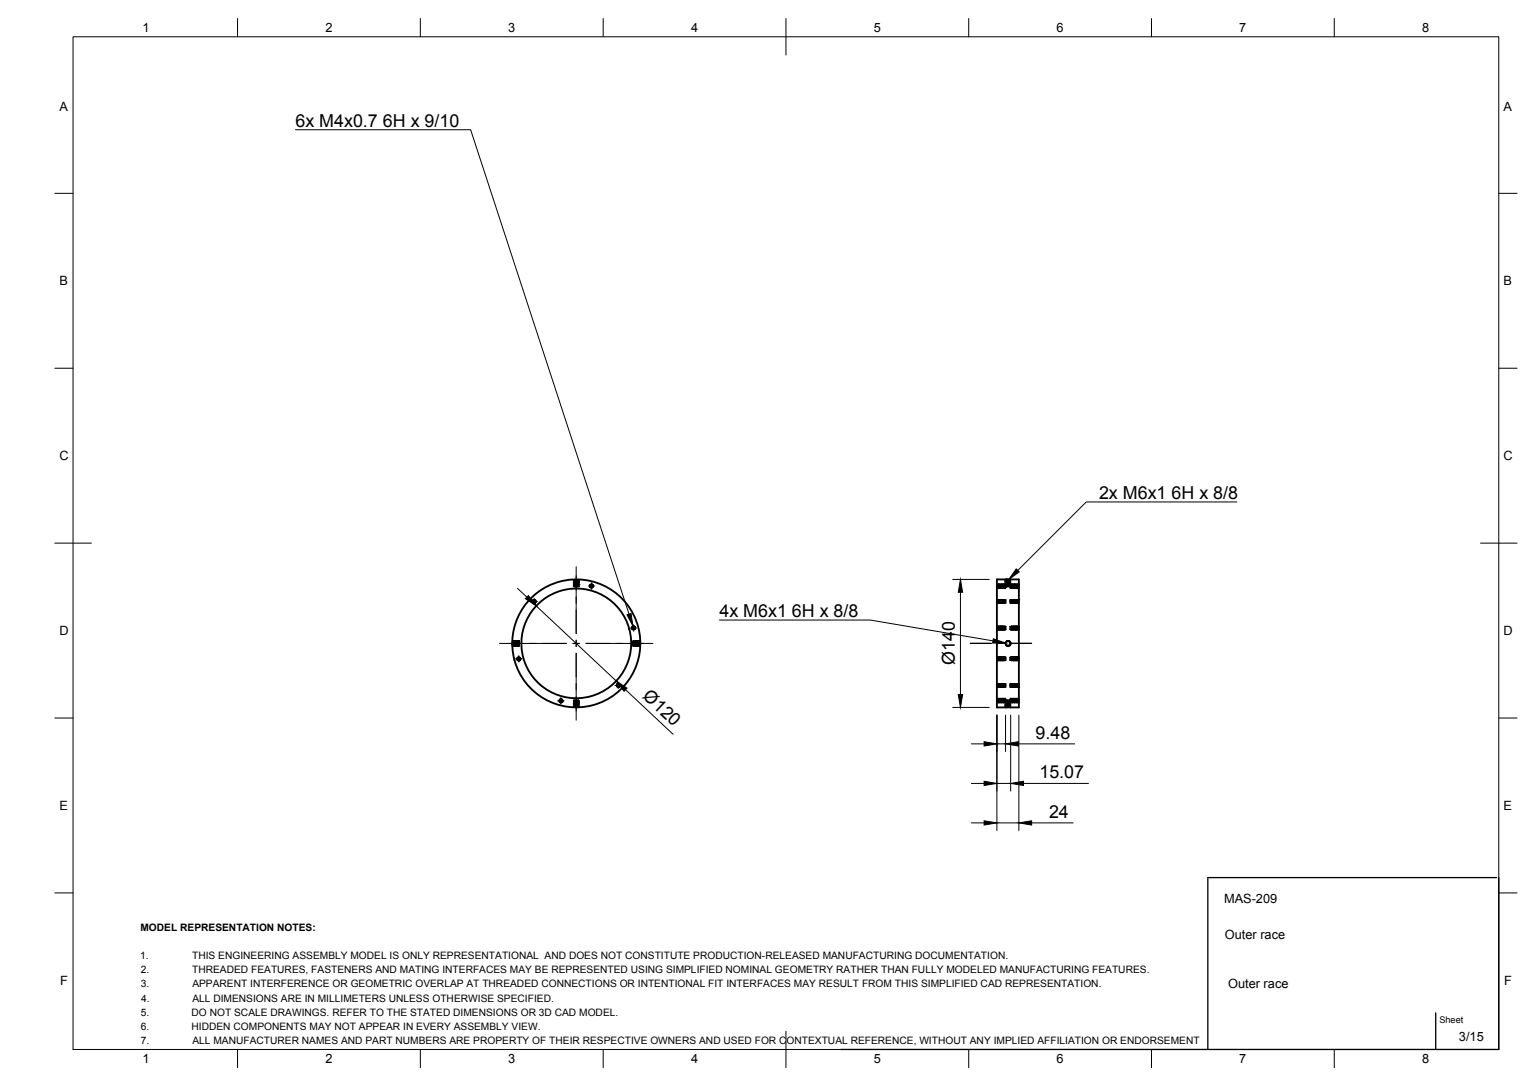
ISO-10303-21;
HEADER;
/* Generated by software containing ST-Developer
 * from STEP Tools, Inc. (www.steptools.com) 
 */

FILE_DESCRIPTION(
/* description */ ('Independent bearing-supported roller-ramp one-way clutch. Six logarit
hmic ramps with plain solid rollers, sprung guided plungers, native Co
il variants, removable shared keepers, rounded parallel key, shaft wit
h complete retaining lips, bronze journal/thrust support and bolted co
vers. Native rotor, roller planar/spin and plunger joints permit manua
l geometric engaged/released inspection. Automatic frictional torque s
witching/contact dynamics are not simulated; no capacity, hardness, fi
t, lubrication, speed, force or life rating. External input driver/cou
pling/anchors outside assembly.'),
/* implementation_level */ '2;1');

FILE_NAME(
/* name */ 'Outer race.step',
/* time_stamp */ '2026-11-08T07:04:38-08:00',
/* author */ (''),
/* organization */ (''),
/* preprocessor_version */ 'ST-DEVELOPER v20.2',
/* originating_system */ 'Autodesk Translation Framework v15.17.0.0',
/* authorisation */ '');

FILE_SCHEMA (('AUTOMOTIVE_DESIGN { 1 0 10303 214 3 1 1 }'));
ENDSEC;

DATA;
#10=MECHANICAL_DESIGN_GEOMETRIC_PRESENTATION_REPRESENTATION('',(#300),#99526);
#268=SHAPE_REPRESENTATION_RELATIONSHIP('SRR','None',#99625,#284);
#284=ADVANCED_BREP_SHAPE_REPRESENTATION('',(#316),#99510);
#300=STYLED_ITEM('',(#99714),#316);
#316=MANIFOLD_SOLID_BREP('Body1',#18270);
#332=FACE_BOUND('',#2130,.T.);
#333=FACE_BOUND('',#2131,.T.);
#334=FACE_BOUND('',#2132,.T.);
#335=FACE_BOUND('',#2133,.T.);
#336=FACE_BOUND('',#2135,.T.);
#337=FACE_BOUND('',#2136,.T.);
#338=FACE_BOUND('',#2137,.T.);
#339=FACE_BOUND('',#2138,.T.);
#340=FACE_BOUND('',#2139,.T.);
#341=FACE_BOUND('',#2140,.T.);
#342=FACE_BOUND('',#2141,.T.);
#343=FACE_BOUND('',#2143,.T.);
#344=FACE_BOUND('',#2144,.T.);
#345=FACE_BOUND('',#2145,.T.);
#346=FACE_BOUND('',#2146,.T.);
#347=FACE_BOUND('',#2147,.T.);
#348=FACE_BOUND('',#2148,.T.);
#349=FACE_BOUND('',#2149,.T.);
#440=PLANE('',#18901);
#441=PLANE('',#18903);
#442=PLANE('',#18905);
#443=PLANE('',#18908);
#444=PLANE('',#18909);
#445=PLANE('',#18912);
#446=PLANE('',#18915);
#447=PLANE('',#18918);
#448=PLANE('',#18921);
#449=PLANE('',#18924);
#450=PLANE('',#18925);
#451=PLANE('',#18926);
#452=PLANE('',#18927);
#453=PLANE('',#18928);
#454=PLANE('',#18929);
#455=PLANE('',#18932);
#456=PLANE('',#18935);
#457=PLANE('',#18938);
#458=PLANE('',#18941);
#459=PLANE('',#18944);
#460=PLANE('',#18945);
#461=PLANE('',#18946);
#462=PLANE('',#18947);
#463=PLANE('',#18948);
#464=PLANE('',#18949);
#465=PLANE('',#18952);
#466=PLANE('',#18953);
#467=PLANE('',#18956);
#468=PLANE('',#18963);
#469=PLANE('',#18964);
#614=B_SPLINE_SURFACE_WITH_KNOTS('',3,3,((#36513,#36514,#36515,#36516,#36517,
#36518,#36519,#36520,#36521,#36522,#36523,#36524,#36525,#36526,#36527,#36528,
#36529,#36530,#36531,#36532,#36533,#36534,#36535,#36536,#36537,#36538,#36539,
#36540,#36541,#36542,#36543,#36544,#36545,#36546,#36547,#36548,#36549,#36550,
#36551,#36552,#36553,#36554,#36555,#36556,#36557,#36558,#36559,#36560,#36561,
#36562,#36563,#36564,#36565,#36566,#36567,#36568),(#36569,#36570,#36571,
#36572,#36573,#36574,#36575,#36576,#36577,#36578,#36579,#36580,#36581,#36582,
#36583,#36584,#36585,#36586,#36587,#36588,#36589,#36590,#36591,#36592,#36593,
#36594,#36595,#36596,#36597,#36598,#36599,#36600,#36601,#36602,#36603,#36604,
#36605,#36606,#36607,#36608,#36609,#36610,#36611,#36612,#36613,#36614,#36615,
#36616,#36617,#36618,#36619,#36620,#36621,#36622,#36623,#36624),(#36625,
#36626,#36627,#36628,#36629,#36630,#36631,#36632,#36633,#36634,#36635,#36636,
#36637,#36638,#36639,#36640,#36641,#36642,#36643,#36644,#36645,#36646,#36647,
#36648,#36649,#36650,#36651,#36652,#36653,#36654,#36655,#36656,#36657,#36658,
#36659,#36660,#36661,#36662,#36663,#36664,#36665,#36666,#36667,#36668,#36669,
#36670,#36671,#36672,#36673,#36674,#36675,#36676,#36677,#36678,#36679,#36680),
(#36681,#36682,#36683,#36684,#36685,#36686,#36687,#36688,#36689,#36690,
#36691,#36692,#36693,#36694,#36695,#36696,#36697,#36698,#36699,#36700,#36701,
#36702,#36703,#36704,#36705,#36706,#36707,#36708,#36709,#36710,#36711,#36712,
#36713,#36714,#36715,#36716,#36717,#36718,#36719,#36720,#36721,#36722,#36723,
#36724,#36725,#36726,#36727,#36728,#36729,#36730,#36731,#36732,#36733,#36734,
#36735,#36736)),.UNSPECIFIED.,.F.,.F.,.F.,(4,4),(4,1,1,1,1,1,1,1,1,1,1,
1,1,1,1,1,1,1,1,1,1,1,1,1,1,1,1,1,1,1,1,1,1,1,1,1,1,1,1,1,1,1,1,1,1,1,1,
1,1,1,1,1,1,4),(0.,0.0642013499338865),(12.0817516052311,13.0640094280149,
14.0462672507987,15.0285250735825,16.0107828963664,16.9930407191502,17.975298541934,
18.9575563647178,19.9398141875016,20.9220720102854,21.9043298330692,22.886587655853,
23.8688454786368,24.8511033014206,25.8333611242044,26.8156189469882,27.797876769772,
28.7801345925559,29.7623924153397,30.7446502381235,31.7269080609073,32.7091658836911,
33.6914237064749,34.6736815292587,35.6559393520425,36.6381971748263,37.6204549976101,
38.6027128203939,39.5849706431777,40.5672284659615,41.5494862887453,42.5317441115292,
43.514001934313,44.4962597570968,45.4785175798806,46.4607754026644,47.4430332254482,
48.425291048232,49.4075488710158,50.3898066937996,51.3720645165834,52.3543223393672,
53.336580162151,54.3188379849348,55.3010958077186,56.2833536305025,57.2656114532863,
58.2478692760701,59.2301270988539,60.2123849216377,61.1946427444215,62.1769005672053,
63.1591583899891,64.1414162127729),.UNSPECIFIED.);
#615=B_SPLINE_SURFACE_WITH_KNOTS('',3,3,((#36890,#36891,#36892,#36893,#36894,
#36895,#36896,#36897,#36898,#36899,#36900,#36901,#36902,#36903,#36904,#36905,
#36906,#36907,#36908,#36909,#36910,#36911,#36912,#36913,#36914,#36915,#36916,
#36917,#36918,#36919,#36920,#36921,#36922,#36923,#36924,#36925,#36926,#36927,
#36928,#36929,#36930,#36931,#36932,#36933,#36934,#36935,#36936,#36937,#36938,
#36939,#36940,#36941,#36942,#36943,#36944,#36945),(#36946,#36947,#36948,
#36949,#36950,#36951,#36952,#36953,#36954,#36955,#36956,#36957,#36958,#36959,
#36960,#36961,#36962,#36963,#36964,#36965,#36966,#36967,#36968,#36969,#36970,
#36971,#36972,#36973,#36974,#36975,#36976,#36977,#36978,#36979,#36980,#36981,
#36982,#36983,#36984,#36985,#36986,#36987,#36988,#36989,#36990,#36991,#36992,
#36993,#36994,#36995,#36996,#36997,#36998,#36999,#37000,#37001),(#37002,
#37003,#37004,#37005,#37006,#37007,#37008,#37009,#37010,#37011,#37012,#37013,
#37014,#37015,#37016,#37017,#37018,#37019,#37020,#37021,#37022,#37023,#37024,
#37025,#37026,#37027,#37028,#37029,#37030,#37031,#37032,#37033,#37034,#37035,
#37036,#37037,#37038,#37039,#37040,#37041,#37042,#37043,#37044,#37045,#37046,
#37047,#37048,#37049,#37050,#37051,#37052,#37053,#37054,#37055,#37056,#37057),
(#37058,#37059,#37060,#37061,#37062,#37063,#37064,#37065,#37066,#37067,
#37068,#37069,#37070,#37071,#37072,#37073,#37074,#37075,#37076,#37077,#37078,
#37079,#37080,#37081,#37082,#37083,#37084,#37085,#37086,#37087,#37088,#37089,
#37090,#37091,#37092,#37093,#37094,#37095,#37096,#37097,#37098,#37099,#37100,
#37101,#37102,#37103,#37104,#37105,#37106,#37107,#37108,#37109,#37110,#37111,
#37112,#37113)),.UNSPECIFIED.,.F.,.F.,.F.,(4,4),(4,1,1,1,1,1,1,1,1,1,1,
1,1,1,1,1,1,1,1,1,1,1,1,1,1,1,1,1,1,1,1,1,1,1,1,1,1,1,1,1,1,1,1,1,1,1,1,
1,1,1,1,1,1,4),(0.,0.0642013499338865),(14.4348810643014,15.4206536381342,
16.4064262119669,17.3921987857997,18.3779713596324,19.3637439334652,20.3495165072979,
21.3352890811306,22.3210616549634,23.3068342287961,24.2926068026289,25.2783793764616,
26.2641519502944,27.2499245241271,28.2356970979599,29.2214696717926,30.2072422456253,
31.1930148194581,32.1787873932908,33.1645599671236,34.1503325409563,35.1361051147891,
36.1218776886218,37.1076502624546,38.0934228362873,39.07919541012,40.0649679839528,
41.0507405577855,42.0365131316183,43.022285705451,44.0080582792838,44.9938308531165,
45.9796034269493,46.965376000782,47.9511485746147,48.9369211484475,49.9226937222802,
50.908466296113,51.8942388699457,52.8800114437785,53.8657840176112,54.851556591444,
55.8373291652767,56.8231017391094,57.8088743129422,58.7946468867749,59.7804194606077,
60.7661920344404,61.7519646082732,62.7377371821059,63.7235097559387,64.7092823297714,
65.6950549036041,66.6808274774369),.UNSPECIFIED.);
#616=B_SPLINE_SURFACE_WITH_KNOTS('',3,3,((#37247,#37248,#37249,#37250,#37251,
#37252,#37253,#37254,#37255,#37256,#37257,#37258,#37259,#37260,#37261,#37262,
#37263,#37264,#37265,#37266,#37267,#37268,#37269,#37270,#37271,#37272,#37273,
#37274,#37275,#37276,#37277,#37278,#37279,#37280,#37281,#37282,#37283,#37284,
#37285,#37286,#37287,#37288,#37289,#37290,#37291,#37292,#37293,#37294,#37295,
#37296,#37297,#37298,#37299,#37300,#37301,#37302),(#37303,#37304,#37305,
#37306,#37307,#37308,#37309,#37310,#37311,#37312,#37313,#37314,#37315,#37316,
#37317,#37318,#37319,#37320,#37321,#37322,#37323,#37324,#37325,#37326,#37327,
#37328,#37329,#37330,#37331,#37332,#37333,#37334,#37335,#37336,#37337,#37338,
#37339,#37340,#37341,#37342,#37343,#37344,#37345,#37346,#37347,#37348,#37349,
#37350,#37351,#37352,#37353,#37354,#37355,#37356,#37357,#37358),(#37359,
#37360,#37361,#37362,#37363,#37364,#37365,#37366,#37367,#37368,#37369,#37370,
#37371,#37372,#37373,#37374,#37375,#37376,#37377,#37378,#37379,#37380,#37381,
#37382,#37383,#37384,#37385,#37386,#37387,#37388,#37389,#37390,#37391,#37392,
#37393,#37394,#37395,#37396,#37397,#37398,#37399,#37400,#37401,#37402,#37403,
#37404,#37405,#37406,#37407,#37408,#37409,#37410,#37411,#37412,#37413,#37414),
(#37415,#37416,#37417,#37418,#37419,#37420,#37421,#37422,#37423,#37424,
#37425,#37426,#37427,#37428,#37429,#37430,#37431,#37432,#37433,#37434,#37435,
#37436,#37437,#37438,#37439,#37440,#37441,#37442,#37443,#37444,#37445,#37446,
#37447,#37448,#37449,#37450,#37451,#37452,#37453,#37454,#37455,#37456,#37457,
#37458,#37459,#37460,#37461,#37462,#37463,#37464,#37465,#37466,#37467,#37468,
#37469,#37470)),.UNSPECIFIED.,.F.,.F.,.F.,(4,4),(4,1,1,1,1,1,1,1,1,1,1,
1,1,1,1,1,1,1,1,1,1,1,1,1,1,1,1,1,1,1,1,1,1,1,1,1,1,1,1,1,1,1,1,1,1,1,1,
1,1,1,1,1,1,4),(0.,0.0642013499338865),(12.0817516052313,13.0640094280151,
14.046267250799,15.0285250735828,16.0107828963666,16.9930407191504,17.9752985419342,
18.957556364718,19.9398141875018,20.9220720102856,21.9043298330694,22.8865876558532,
23.868845478637,24.8511033014208,25.8333611242046,26.8156189469884,27.7978767697722,
28.780134592556,29.7623924153398,30.7446502381237,31.7269080609075,32.7091658836913,
33.6914237064751,34.6736815292589,35.6559393520427,36.6381971748265,37.6204549976103,
38.6027128203941,39.5849706431779,40.5672284659617,41.5494862887455,42.5317441115293,
43.5140019343131,44.4962597570969,45.4785175798807,46.4607754026645,47.4430332254484,
48.4252910482322,49.407548871016,50.3898066937998,51.3720645165836,52.3543223393674,
53.3365801621512,54.318837984935,55.3010958077188,56.2833536305026,57.2656114532864,
58.2478692760702,59.230127098854,60.2123849216378,61.1946427444216,62.1769005672054,
63.1591583899892,64.1414162127731),.UNSPECIFIED.);
#617=B_SPLINE_SURFACE_WITH_KNOTS('',3,3,((#37624,#37625,#37626,#37627,#37628,
#37629,#37630,#37631,#37632,#37633,#37634,#37635,#37636,#37637,#37638,#37639,
#37640,#37641,#37642,#37643,#37644,#37645,#37646,#37647,#37648,#37649,#37650,
#37651,#37652,#37653,#37654,#37655,#37656,#37657,#37658,#37659,#37660,#37661,
#37662,#37663,#37664,#37665,#37666,#37667,#37668,#37669,#37670,#37671,#37672,
#37673,#37674,#37675,#37676,#37677,#37678,#37679),(#37680,#37681,#37682,
#37683,#37684,#37685,#37686,#37687,#37688,#37689,#37690,#37691,#37692,#37693,
#37694,#37695,#37696,#37697,#37698,#37699,#37700,#37701,#37702,#37703,#37704,
#37705,#37706,#37707,#37708,#37709,#37710,#37711,#37712,#37713,#37714,#37715,
#37716,#37717,#37718,#37719,#37720,#37721,#37722,#37723,#37724,#37725,#37726,
#37727,#37728,#37729,#37730,#37731,#37732,#37733,#37734,#37735),(#37736,
#37737,#37738,#37739,#37740,#37741,#37742,#37743,#37744,#37745,#37746,#37747,
#37748,#37749,#37750,#37751,#37752,#37753,#37754,#37755,#37756,#37757,#37758,
#37759,#37760,#37761,#37762,#37763,#37764,#37765,#37766,#37767,#37768,#37769,
#37770,#37771,#37772,#37773,#37774,#37775,#37776,#37777,#37778,#37779,#37780,
#37781,#37782,#37783,#37784,#37785,#37786,#37787,#37788,#37789,#37790,#37791),
(#37792,#37793,#37794,#37795,#37796,#37797,#37798,#37799,#37800,#37801,
#37802,#37803,#37804,#37805,#37806,#37807,#37808,#37809,#37810,#37811,#37812,
#37813,#37814,#37815,#37816,#37817,#37818,#37819,#37820,#37821,#37822,#37823,
#37824,#37825,#37826,#37827,#37828,#37829,#37830,#37831,#37832,#37833,#37834,
#37835,#37836,#37837,#37838,#37839,#37840,#37841,#37842,#37843,#37844,#37845,
#37846,#37847)),.UNSPECIFIED.,.F.,.F.,.F.,(4,4),(4,1,1,1,1,1,1,1,1,1,1,
1,1,1,1,1,1,1,1,1,1,1,1,1,1,1,1,1,1,1,1,1,1,1,1,1,1,1,1,1,1,1,1,1,1,1,1,
1,1,1,1,1,1,4),(0.,0.0642013499338865),(14.4348810643015,15.4206536381343,
16.406426211967,17.3921987857997,18.3779713596325,19.3637439334652,20.349516507298,
21.3352890811307,22.3210616549635,23.3068342287962,24.292606802629,25.2783793764617,
26.2641519502944,27.2499245241272,28.2356970979599,29.2214696717927,30.2072422456254,
31.1930148194582,32.1787873932909,33.1645599671237,34.1503325409564,35.1361051147891,
36.1218776886219,37.1076502624546,38.0934228362874,39.0791954101201,40.0649679839529,
41.0507405577856,42.0365131316183,43.0222857054511,44.0080582792838,44.9938308531166,
45.9796034269493,46.9653760007821,47.9511485746148,48.9369211484476,49.9226937222803,
50.908466296113,51.8942388699458,52.8800114437785,53.8657840176113,54.851556591444,
55.8373291652768,56.8231017391095,57.8088743129423,58.794646886775,59.7804194606078,
60.7661920344405,61.7519646082732,62.737737182106,63.7235097559387,64.7092823297715,
65.6950549036042,66.680827477437),.UNSPECIFIED.);
#618=B_SPLINE_SURFACE_WITH_KNOTS('',3,3,((#37981,#37982,#37983,#37984,#37985,
#37986,#37987,#37988,#37989,#37990,#37991,#37992,#37993,#37994,#37995,#37996,
#37997,#37998,#37999,#38000,#38001,#38002,#38003,#38004,#38005,#38006,#38007,
#38008,#38009,#38010,#38011,#38012,#38013,#38014,#38015,#38016,#38017,#38018,
#38019,#38020,#38021,#38022,#38023,#38024,#38025,#38026,#38027,#38028,#38029,
#38030,#38031,#38032,#38033,#38034,#38035,#38036),(#38037,#38038,#38039,
#38040,#38041,#38042,#38043,#38044,#38045,#38046,#38047,#38048,#38049,#38050,
#38051,#38052,#38053,#38054,#38055,#38056,#38057,#38058,#38059,#38060,#38061,
#38062,#38063,#38064,#38065,#38066,#38067,#38068,#38069,#38070,#38071,#38072,
#38073,#38074,#38075,#38076,#38077,#38078,#38079,#38080,#38081,#38082,#38083,
#38084,#38085,#38086,#38087,#38088,#38089,#38090,#38091,#38092),(#38093,
#38094,#38095,#38096,#38097,#38098,#38099,#38100,#38101,#38102,#38103,#38104,
#38105,#38106,#38107,#38108,#38109,#38110,#38111,#38112,#38113,#38114,#38115,
#38116,#38117,#38118,#38119,#38120,#38121,#38122,#38123,#38124,#38125,#38126,
#38127,#38128,#38129,#38130,#38131,#38132,#38133,#38134,#38135,#38136,#38137,
#38138,#38139,#38140,#38141,#38142,#38143,#38144,#38145,#38146,#38147,#38148),
(#38149,#38150,#38151,#38152,#38153,#38154,#38155,#38156,#38157,#38158,
#38159,#38160,#38161,#38162,#38163,#38164,#38165,#38166,#38167,#38168,#38169,
#38170,#38171,#38172,#38173,#38174,#38175,#38176,#38177,#38178,#38179,#38180,
#38181,#38182,#38183,#38184,#38185,#38186,#38187,#38188,#38189,#38190,#38191,
#38192,#38193,#38194,#38195,#38196,#38197,#38198,#38199,#38200,#38201,#38202,
#38203,#38204)),.UNSPECIFIED.,.F.,.F.,.F.,(4,4),(4,1,1,1,1,1,1,1,1,1,1,
1,1,1,1,1,1,1,1,1,1,1,1,1,1,1,1,1,1,1,1,1,1,1,1,1,1,1,1,1,1,1,1,1,1,1,1,
1,1,1,1,1,1,4),(0.,0.0642013499338865),(12.0817516052311,13.0640094280149,
14.0462672507987,15.0285250735825,16.0107828963663,16.9930407191502,17.975298541934,
18.9575563647178,19.9398141875016,20.9220720102854,21.9043298330692,22.886587655853,
23.8688454786368,24.8511033014206,25.8333611242044,26.8156189469882,27.797876769772,
28.7801345925558,29.7623924153396,30.7446502381234,31.7269080609072,32.709165883691,
33.6914237064749,34.6736815292587,35.6559393520425,36.6381971748263,37.6204549976101,
38.6027128203939,39.5849706431777,40.5672284659615,41.5494862887453,42.5317441115291,
43.5140019343129,44.4962597570967,45.4785175798805,46.4607754026643,47.4430332254481,
48.4252910482319,49.4075488710157,50.3898066937996,51.3720645165834,52.3543223393672,
53.336580162151,54.3188379849348,55.3010958077186,56.2833536305024,57.2656114532862,
58.24786927607,59.2301270988538,60.2123849216376,61.1946427444214,62.1769005672052,
63.159158389989,64.1414162127728),.UNSPECIFIED.);
#619=B_SPLINE_SURFACE_WITH_KNOTS('',3,3,((#38358,#38359,#38360,#38361,#38362,
#38363,#38364,#38365,#38366,#38367,#38368,#38369,#38370,#38371,#38372,#38373,
#38374,#38375,#38376,#38377,#38378,#38379,#38380,#38381,#38382,#38383,#38384,
#38385,#38386,#38387,#38388,#38389,#38390,#38391,#38392,#38393,#38394,#38395,
#38396,#38397,#38398,#38399,#38400,#38401,#38402,#38403,#38404,#38405,#38406,
#38407,#38408,#38409,#38410,#38411,#38412,#38413),(#38414,#38415,#38416,
#38417,#38418,#38419,#38420,#38421,#38422,#38423,#38424,#38425,#38426,#38427,
#38428,#38429,#38430,#38431,#38432,#38433,#38434,#38435,#38436,#38437,#38438,
#38439,#38440,#38441,#38442,#38443,#38444,#38445,#38446,#38447,#38448,#38449,
#38450,#38451,#38452,#38453,#38454,#38455,#38456,#38457,#38458,#38459,#38460,
#38461,#38462,#38463,#38464,#38465,#38466,#38467,#38468,#38469),(#38470,
#38471,#38472,#38473,#38474,#38475,#38476,#38477,#38478,#38479,#38480,#38481,
#38482,#38483,#38484,#38485,#38486,#38487,#38488,#38489,#38490,#38491,#38492,
#38493,#38494,#38495,#38496,#38497,#38498,#38499,#38500,#38501,#38502,#38503,
#38504,#38505,#38506,#38507,#38508,#38509,#38510,#38511,#38512,#38513,#38514,
#38515,#38516,#38517,#38518,#38519,#38520,#38521,#38522,#38523,#38524,#38525),
(#38526,#38527,#38528,#38529,#38530,#38531,#38532,#38533,#38534,#38535,
#38536,#38537,#38538,#38539,#38540,#38541,#38542,#38543,#38544,#38545,#38546,
#38547,#38548,#38549,#38550,#38551,#38552,#38553,#38554,#38555,#38556,#38557,
#38558,#38559,#38560,#38561,#38562,#38563,#38564,#38565,#38566,#38567,#38568,
#38569,#38570,#38571,#38572,#38573,#38574,#38575,#38576,#38577,#38578,#38579,
#38580,#38581)),.UNSPECIFIED.,.F.,.F.,.F.,(4,4),(4,1,1,1,1,1,1,1,1,1,1,
1,1,1,1,1,1,1,1,1,1,1,1,1,1,1,1,1,1,1,1,1,1,1,1,1,1,1,1,1,1,1,1,1,1,1,1,
1,1,1,1,1,1,4),(0.,0.0642013499338865),(14.4348810643012,15.420653638134,
16.4064262119667,17.3921987857995,18.3779713596322,19.363743933465,20.3495165072977,
21.3352890811305,22.3210616549632,23.3068342287959,24.2926068026287,25.2783793764614,
26.2641519502942,27.2499245241269,28.2356970979597,29.2214696717924,30.2072422456252,
31.1930148194579,32.1787873932907,33.1645599671234,34.1503325409562,35.1361051147889,
36.1218776886216,37.1076502624544,38.0934228362871,39.0791954101199,40.0649679839526,
41.0507405577854,42.0365131316181,43.0222857054509,44.0080582792836,44.9938308531164,
45.9796034269491,46.9653760007819,47.9511485746146,48.9369211484474,49.9226937222801,
50.9084662961128,51.8942388699456,52.8800114437783,53.8657840176111,54.8515565914438,
55.8373291652766,56.8231017391093,57.8088743129421,58.7946468867748,59.7804194606076,
60.7661920344403,61.751964608273,62.7377371821058,63.7235097559385,64.7092823297713,
65.695054903604,66.6808274774368),.UNSPECIFIED.);
#620=B_SPLINE_SURFACE_WITH_KNOTS('',3,3,((#38721,#38722,#38723,#38724,#38725,
#38726,#38727,#38728,#38729,#38730,#38731,#38732,#38733,#38734,#38735,#38736,
#38737,#38738,#38739,#38740,#38741,#38742,#38743,#38744,#38745,#38746,#38747,
#38748,#38749,#38750,#38751,#38752,#38753,#38754,#38755,#38756,#38757,#38758,
#38759,#38760,#38761,#38762,#38763,#38764,#38765,#38766,#38767,#38768,#38769,
#38770,#38771,#38772,#38773,#38774,#38775,#38776),(#38777,#38778,#38779,
#38780,#38781,#38782,#38783,#38784,#38785,#38786,#38787,#38788,#38789,#38790,
#38791,#38792,#38793,#38794,#38795,#38796,#38797,#38798,#38799,#38800,#38801,
#38802,#38803,#38804,#38805,#38806,#38807,#38808,#38809,#38810,#38811,#38812,
#38813,#38814,#38815,#38816,#38817,#38818,#38819,#38820,#38821,#38822,#38823,
#38824,#38825,#38826,#38827,#38828,#38829,#38830,#38831,#38832),(#38833,
#38834,#38835,#38836,#38837,#38838,#38839,#38840,#38841,#38842,#38843,#38844,
#38845,#38846,#38847,#38848,#38849,#38850,#38851,#38852,#38853,#38854,#38855,
#38856,#38857,#38858,#38859,#38860,#38861,#38862,#38863,#38864,#38865,#38866,
#38867,#38868,#38869,#38870,#38871,#38872,#38873,#38874,#38875,#38876,#38877,
#38878,#38879,#38880,#38881,#38882,#38883,#38884,#38885,#38886,#38887,#38888),
(#38889,#38890,#38891,#38892,#38893,#38894,#38895,#38896,#38897,#38898,
#38899,#38900,#38901,#38902,#38903,#38904,#38905,#38906,#38907,#38908,#38909,
#38910,#38911,#38912,#38913,#38914,#38915,#38916,#38917,#38918,#38919,#38920,
#38921,#38922,#38923,#38924,#38925,#38926,#38927,#38928,#38929,#38930,#38931,
#38932,#38933,#38934,#38935,#38936,#38937,#38938,#38939,#38940,#38941,#38942,
#38943,#38944)),.UNSPECIFIED.,.F.,.F.,.F.,(4,4),(4,1,1,1,1,1,1,1,1,1,1,
1,1,1,1,1,1,1,1,1,1,1,1,1,1,1,1,1,1,1,1,1,1,1,1,1,1,1,1,1,1,1,1,1,1,1,1,
1,1,1,1,1,1,4),(0.,0.0642013499338865),(12.0817516052311,13.0640094280149,
14.0462672507987,15.0285250735825,16.0107828963663,16.9930407191501,17.9752985419339,
18.9575563647177,19.9398141875016,20.9220720102854,21.9043298330692,22.886587655853,
23.8688454786368,24.8511033014206,25.8333611242044,26.8156189469882,27.797876769772,
28.7801345925558,29.7623924153396,30.7446502381234,31.7269080609072,32.709165883691,
33.6914237064748,34.6736815292587,35.6559393520425,36.6381971748263,37.6204549976101,
38.6027128203939,39.5849706431777,40.5672284659615,41.5494862887453,42.5317441115291,
43.5140019343129,44.4962597570967,45.4785175798805,46.4607754026643,47.4430332254481,
48.4252910482319,49.4075488710157,50.3898066937995,51.3720645165834,52.3543223393672,
53.336580162151,54.3188379849348,55.3010958077186,56.2833536305024,57.2656114532862,
58.24786927607,59.2301270988538,60.2123849216376,61.1946427444214,62.1769005672052,
63.159158389989,64.1414162127728),.UNSPECIFIED.);
#621=B_SPLINE_SURFACE_WITH_KNOTS('',3,3,((#39098,#39099,#39100,#39101,#39102,
#39103,#39104,#39105,#39106,#39107,#39108,#39109,#39110,#39111,#39112,#39113,
#39114,#39115,#39116,#39117,#39118,#39119,#39120,#39121,#39122,#39123,#39124,
#39125,#39126,#39127,#39128,#39129,#39130,#39131,#39132,#39133,#39134,#39135,
#39136,#39137,#39138,#39139,#39140,#39141,#39142,#39143,#39144,#39145,#39146,
#39147,#39148,#39149,#39150,#39151,#39152,#39153),(#39154,#39155,#39156,
#39157,#39158,#39159,#39160,#39161,#39162,#39163,#39164,#39165,#39166,#39167,
#39168,#39169,#39170,#39171,#39172,#39173,#39174,#39175,#39176,#39177,#39178,
#39179,#39180,#39181,#39182,#39183,#39184,#39185,#39186,#39187,#39188,#39189,
#39190,#39191,#39192,#39193,#39194,#39195,#39196,#39197,#39198,#39199,#39200,
#39201,#39202,#39203,#39204,#39205,#39206,#39207,#39208,#39209),(#39210,
#39211,#39212,#39213,#39214,#39215,#39216,#39217,#39218,#39219,#39220,#39221,
#39222,#39223,#39224,#39225,#39226,#39227,#39228,#39229,#39230,#39231,#39232,
#39233,#39234,#39235,#39236,#39237,#39238,#39239,#39240,#39241,#39242,#39243,
#39244,#39245,#39246,#39247,#39248,#39249,#39250,#39251,#39252,#39253,#39254,
#39255,#39256,#39257,#39258,#39259,#39260,#39261,#39262,#39263,#39264,#39265),
(#39266,#39267,#39268,#39269,#39270,#39271,#39272,#39273,#39274,#39275,
#39276,#39277,#39278,#39279,#39280,#39281,#39282,#39283,#39284,#39285,#39286,
#39287,#39288,#39289,#39290,#39291,#39292,#39293,#39294,#39295,#39296,#39297,
#39298,#39299,#39300,#39301,#39302,#39303,#39304,#39305,#39306,#39307,#39308,
#39309,#39310,#39311,#39312,#39313,#39314,#39315,#39316,#39317,#39318,#39319,
#39320,#39321)),.UNSPECIFIED.,.F.,.F.,.F.,(4,4),(4,1,1,1,1,1,1,1,1,1,1,
1,1,1,1,1,1,1,1,1,1,1,1,1,1,1,1,1,1,1,1,1,1,1,1,1,1,1,1,1,1,1,1,1,1,1,1,
1,1,1,1,1,1,4),(0.,0.0642013499338865),(14.4348810643014,15.4206536381342,
16.4064262119669,17.3921987857997,18.3779713596324,19.3637439334652,20.3495165072979,
21.3352890811306,22.3210616549634,23.3068342287961,24.2926068026289,25.2783793764616,
26.2641519502944,27.2499245241271,28.2356970979599,29.2214696717926,30.2072422456253,
31.1930148194581,32.1787873932908,33.1645599671236,34.1503325409563,35.1361051147891,
36.1218776886218,37.1076502624545,38.0934228362873,39.07919541012,40.0649679839528,
41.0507405577855,42.0365131316183,43.022285705451,44.0080582792838,44.9938308531165,
45.9796034269492,46.965376000782,47.9511485746147,48.9369211484475,49.9226937222802,
50.908466296113,51.8942388699457,52.8800114437785,53.8657840176112,54.8515565914439,
55.8373291652767,56.8231017391094,57.8088743129422,58.7946468867749,59.7804194606077,
60.7661920344404,61.7519646082732,62.7377371821059,63.7235097559386,64.7092823297714,
65.6950549036041,66.6808274774369),.UNSPECIFIED.);
#622=B_SPLINE_SURFACE_WITH_KNOTS('',3,3,((#39653,#39654,#39655,#39656,#39657,
#39658,#39659,#39660,#39661,#39662,#39663,#39664,#39665,#39666,#39667,#39668,
#39669,#39670,#39671,#39672,#39673,#39674,#39675,#39676,#39677,#39678,#39679,
#39680,#39681,#39682,#39683,#39684,#39685,#39686,#39687,#39688,#39689,#39690,
#39691,#39692,#39693,#39694,#39695,#39696,#39697,#39698,#39699,#39700,#39701,
#39702,#39703,#39704,#39705,#39706,#39707,#39708,#39709,#39710,#39711,#39712,
#39713,#39714,#39715,#39716,#39717,#39718,#39719,#39720,#39721,#39722,#39723,
#39724,#39725,#39726,#39727,#39728,#39729,#39730,#39731,#39732,#39733,#39734,
#39735,#39736,#39737,#39738),(#39739,#39740,#39741,#39742,#39743,#39744,
#39745,#39746,#39747,#39748,#39749,#39750,#39751,#39752,#39753,#39754,#39755,
#39756,#39757,#39758,#39759,#39760,#39761,#39762,#39763,#39764,#39765,#39766,
#39767,#39768,#39769,#39770,#39771,#39772,#39773,#39774,#39775,#39776,#39777,
#39778,#39779,#39780,#39781,#39782,#39783,#39784,#39785,#39786,#39787,#39788,
#39789,#39790,#39791,#39792,#39793,#39794,#39795,#39796,#39797,#39798,#39799,
#39800,#39801,#39802,#39803,#39804,#39805,#39806,#39807,#39808,#39809,#39810,
#39811,#39812,#39813,#39814,#39815,#39816,#39817,#39818,#39819,#39820,#39821,
#39822,#39823,#39824),(#39825,#39826,#39827,#39828,#39829,#39830,#39831,
#39832,#39833,#39834,#39835,#39836,#39837,#39838,#39839,#39840,#39841,#39842,
#39843,#39844,#39845,#39846,#39847,#39848,#39849,#39850,#39851,#39852,#39853,
#39854,#39855,#39856,#39857,#39858,#39859,#39860,#39861,#39862,#39863,#39864,
#39865,#39866,#39867,#39868,#39869,#39870,#39871,#39872,#39873,#39874,#39875,
#39876,#39877,#39878,#39879,#39880,#39881,#39882,#39883,#39884,#39885,#39886,
#39887,#39888,#39889,#39890,#39891,#39892,#39893,#39894,#39895,#39896,#39897,
#39898,#39899,#39900,#39901,#39902,#39903,#39904,#39905,#39906,#39907,#39908,
#39909,#39910),(#39911,#39912,#39913,#39914,#39915,#39916,#39917,#39918,
#39919,#39920,#39921,#39922,#39923,#39924,#39925,#39926,#39927,#39928,#39929,
#39930,#39931,#39932,#39933,#39934,#39935,#39936,#39937,#39938,#39939,#39940,
#39941,#39942,#39943,#39944,#39945,#39946,#39947,#39948,#39949,#39950,#39951,
#39952,#39953,#39954,#39955,#39956,#39957,#39958,#39959,#39960,#39961,#39962,
#39963,#39964,#39965,#39966,#39967,#39968,#39969,#39970,#39971,#39972,#39973,
#39974,#39975,#39976,#39977,#39978,#39979,#39980,#39981,#39982,#39983,#39984,
#39985,#39986,#39987,#39988,#39989,#39990,#39991,#39992,#39993,#39994,#39995,
#39996)),.UNSPECIFIED.,.F.,.F.,.F.,(4,4),(4,1,1,1,1,1,1,1,1,1,1,1,1,1,1,
1,1,1,1,1,1,1,1,1,1,1,1,1,1,1,1,1,1,1,1,1,1,1,1,1,1,1,1,1,1,1,1,1,1,1,1,
1,1,1,1,1,1,1,1,1,1,1,1,1,1,1,1,1,1,1,1,1,1,1,1,1,1,1,1,1,1,1,1,4),(0.,
0.0448889834294934),(11.8615800042567,12.8591513772396,13.8567227502225,
14.8542941232055,15.8518654961884,16.8494368691713,17.8470082421543,18.8445796151372,
19.8421509881201,20.8397223611031,21.837293734086,22.8348651070689,23.8324364800519,
24.8300078530348,25.8275792260177,26.8251505990007,27.8227219719836,28.8202933449665,
29.8178647179495,30.8154360909324,31.8130074639153,32.8105788368983,33.8081502098812,
34.8057215828641,35.803292955847,36.80086432883,37.7984357018129,38.7960070747958,
39.7935784477788,40.7911498207617,41.7887211937446,42.7862925667276,43.7838639397105,
44.7814353126934,45.7790066856764,46.7765780586593,47.7741494316422,48.7717208046252,
49.7692921776081,50.766863550591,51.764434923574,52.7620062965569,53.7595776695398,
54.7571490425228,55.7547204155057,56.7522917884886,57.7498631614716,58.7474345344545,
59.7450059074374,60.7425772804204,61.7401486534033,62.7377200263862,63.7352913993692,
64.7328627723521,65.730434145335,66.728005518318,67.7255768913009,68.7231482642838,
69.7207196372668,70.7182910102497,71.7158623832326,72.7134337562156,73.7110051291985,
74.7085765021814,75.7061478751643,76.7037192481473,77.7012906211302,78.6988619941132,
79.6964333670961,80.694004740079,81.691576113062,82.6891474860449,83.6867188590278,
84.6842902320108,85.6818616049937,86.6794329779766,87.6770043509595,88.6745757239425,
89.6721470969254,90.6697184699083,91.6672898428913,92.6648612158742,93.6624325888571,
94.6600039618401),.UNSPECIFIED.);
#623=B_SPLINE_SURFACE_WITH_KNOTS('',3,3,((#40104,#40105,#40106,#40107,#40108,
#40109,#40110,#40111,#40112,#40113,#40114,#40115,#40116,#40117,#40118,#40119,
#40120,#40121,#40122,#40123,#40124,#40125,#40126,#40127,#40128,#40129,#40130,
#40131,#40132,#40133,#40134,#40135,#40136,#40137,#40138,#40139,#40140,#40141,
#40142,#40143,#40144,#40145,#40146,#40147,#40148,#40149,#40150,#40151,#40152,
#40153,#40154,#40155,#40156,#40157,#40158,#40159,#40160,#40161,#40162,#40163,
#40164,#40165,#40166,#40167,#40168,#40169,#40170,#40171,#40172,#40173,#40174,
#40175,#40176,#40177,#40178,#40179,#40180,#40181,#40182,#40183,#40184,#40185,
#40186,#40187,#40188,#40189),(#40190,#40191,#40192,#40193,#40194,#40195,
#40196,#40197,#40198,#40199,#40200,#40201,#40202,#40203,#40204,#40205,#40206,
#40207,#40208,#40209,#40210,#40211,#40212,#40213,#40214,#40215,#40216,#40217,
#40218,#40219,#40220,#40221,#40222,#40223,#40224,#40225,#40226,#40227,#40228,
#40229,#40230,#40231,#40232,#40233,#40234,#40235,#40236,#40237,#40238,#40239,
#40240,#40241,#40242,#40243,#40244,#40245,#40246,#40247,#40248,#40249,#40250,
#40251,#40252,#40253,#40254,#40255,#40256,#40257,#40258,#40259,#40260,#40261,
#40262,#40263,#40264,#40265,#40266,#40267,#40268,#40269,#40270,#40271,#40272,
#40273,#40274,#40275),(#40276,#40277,#40278,#40279,#40280,#40281,#40282,
#40283,#40284,#40285,#40286,#40287,#40288,#40289,#40290,#40291,#40292,#40293,
#40294,#40295,#40296,#40297,#40298,#40299,#40300,#40301,#40302,#40303,#40304,
#40305,#40306,#40307,#40308,#40309,#40310,#40311,#40312,#40313,#40314,#40315,
#40316,#40317,#40318,#40319,#40320,#40321,#40322,#40323,#40324,#40325,#40326,
#40327,#40328,#40329,#40330,#40331,#40332,#40333,#40334,#40335,#40336,#40337,
#40338,#40339,#40340,#40341,#40342,#40343,#40344,#40345,#40346,#40347,#40348,
#40349,#40350,#40351,#40352,#40353,#40354,#40355,#40356,#40357,#40358,#40359,
#40360,#40361),(#40362,#40363,#40364,#40365,#40366,#40367,#40368,#40369,
#40370,#40371,#40372,#40373,#40374,#40375,#40376,#40377,#40378,#40379,#40380,
#40381,#40382,#40383,#40384,#40385,#40386,#40387,#40388,#40389,#40390,#40391,
#40392,#40393,#40394,#40395,#40396,#40397,#40398,#40399,#40400,#40401,#40402,
#40403,#40404,#40405,#40406,#40407,#40408,#40409,#40410,#40411,#40412,#40413,
#40414,#40415,#40416,#40417,#40418,#40419,#40420,#40421,#40422,#40423,#40424,
#40425,#40426,#40427,#40428,#40429,#40430,#40431,#40432,#40433,#40434,#40435,
#40436,#40437,#40438,#40439,#40440,#40441,#40442,#40443,#40444,#40445,#40446,
#40447)),.UNSPECIFIED.,.F.,.F.,.F.,(4,4),(4,1,1,1,1,1,1,1,1,1,1,1,1,1,1,
1,1,1,1,1,1,1,1,1,1,1,1,1,1,1,1,1,1,1,1,1,1,1,1,1,1,1,1,1,1,1,1,1,1,1,1,
1,1,1,1,1,1,1,1,1,1,1,1,1,1,1,1,1,1,1,1,1,1,1,1,1,1,1,1,1,1,1,1,4),(0.,
0.0448889834294934),(14.3981410127769,15.3957123857598,16.3932837587428,
17.3908551317257,18.3884265047086,19.3859978776916,20.3835692506745,21.3811406236574,
22.3787119966404,23.3762833696233,24.3738547426062,25.3714261155892,26.3689974885721,
27.366568861555,28.364140234538,29.3617116075209,30.3592829805038,31.3568543534868,
32.3544257264697,33.3519970994526,34.3495684724356,35.3471398454185,36.3447112184014,
37.3422825913844,38.3398539643673,39.3374253373502,40.3349967103332,41.3325680833161,
42.330139456299,43.327710829282,44.3252822022649,45.3228535752478,46.3204249482308,
47.3179963212137,48.3155676941966,49.3131390671795,50.3107104401625,51.3082818131454,
52.3058531861283,53.3034245591113,54.3009959320942,55.2985673050771,56.2961386780601,
57.293710051043,58.2912814240259,59.2888527970089,60.2864241699918,61.2839955429747,
62.2815669159577,63.2791382889406,64.2767096619235,65.2742810349065,66.2718524078894,
67.2694237808723,68.2669951538553,69.2645665268382,70.2621378998211,71.2597092728041,
72.257280645787,73.2548520187699,74.2524233917529,75.2499947647358,76.2475661377187,
77.2451375107017,78.2427088836846,79.2402802566675,80.2378516296505,81.2354230026334,
82.2329943756163,83.2305657485992,84.2281371215822,85.2257084945651,86.2232798675481,
87.220851240531,88.2184226135139,89.2159939864968,90.2135653594798,91.2111367324627,
92.2087081054457,93.2062794784286,94.2038508514115,95.2014222243944,96.1989935973774,
97.1965649703603),.UNSPECIFIED.);
#624=B_SPLINE_SURFACE_WITH_KNOTS('',3,3,((#40752,#40753,#40754,#40755,#40756,
#40757,#40758,#40759,#40760,#40761,#40762,#40763,#40764,#40765,#40766,#40767,
#40768,#40769,#40770,#40771,#40772,#40773,#40774,#40775,#40776,#40777,#40778,
#40779,#40780,#40781,#40782,#40783,#40784,#40785,#40786,#40787,#40788,#40789,
#40790,#40791,#40792,#40793,#40794,#40795,#40796,#40797,#40798,#40799,#40800,
#40801,#40802,#40803,#40804,#40805,#40806,#40807,#40808,#40809,#40810,#40811,
#40812,#40813,#40814,#40815,#40816,#40817,#40818,#40819,#40820,#40821,#40822,
#40823,#40824,#40825,#40826,#40827,#40828,#40829,#40830,#40831,#40832,#40833,
#40834,#40835,#40836,#40837),(#40838,#40839,#40840,#40841,#40842,#40843,
#40844,#40845,#40846,#40847,#40848,#40849,#40850,#40851,#40852,#40853,#40854,
#40855,#40856,#40857,#40858,#40859,#40860,#40861,#40862,#40863,#40864,#40865,
#40866,#40867,#40868,#40869,#40870,#40871,#40872,#40873,#40874,#40875,#40876,
#40877,#40878,#40879,#40880,#40881,#40882,#40883,#40884,#40885,#40886,#40887,
#40888,#40889,#40890,#40891,#40892,#40893,#40894,#40895,#40896,#40897,#40898,
#40899,#40900,#40901,#40902,#40903,#40904,#40905,#40906,#40907,#40908,#40909,
#40910,#40911,#40912,#40913,#40914,#40915,#40916,#40917,#40918,#40919,#40920,
#40921,#40922,#40923),(#40924,#40925,#40926,#40927,#40928,#40929,#40930,
#40931,#40932,#40933,#40934,#40935,#40936,#40937,#40938,#40939,#40940,#40941,
#40942,#40943,#40944,#40945,#40946,#40947,#40948,#40949,#40950,#40951,#40952,
#40953,#40954,#40955,#40956,#40957,#40958,#40959,#40960,#40961,#40962,#40963,
#40964,#40965,#40966,#40967,#40968,#40969,#40970,#40971,#40972,#40973,#40974,
#40975,#40976,#40977,#40978,#40979,#40980,#40981,#40982,#40983,#40984,#40985,
#40986,#40987,#40988,#40989,#40990,#40991,#40992,#40993,#40994,#40995,#40996,
#40997,#40998,#40999,#41000,#41001,#41002,#41003,#41004,#41005,#41006,#41007,
#41008,#41009),(#41010,#41011,#41012,#41013,#41014,#41015,#41016,#41017,
#41018,#41019,#41020,#41021,#41022,#41023,#41024,#41025,#41026,#41027,#41028,
#41029,#41030,#41031,#41032,#41033,#41034,#41035,#41036,#41037,#41038,#41039,
#41040,#41041,#41042,#41043,#41044,#41045,#41046,#41047,#41048,#41049,#41050,
#41051,#41052,#41053,#41054,#41055,#41056,#41057,#41058,#41059,#41060,#41061,
#41062,#41063,#41064,#41065,#41066,#41067,#41068,#41069,#41070,#41071,#41072,
#41073,#41074,#41075,#41076,#41077,#41078,#41079,#41080,#41081,#41082,#41083,
#41084,#41085,#41086,#41087,#41088,#41089,#41090,#41091,#41092,#41093,#41094,
#41095)),.UNSPECIFIED.,.F.,.F.,.F.,(4,4),(4,1,1,1,1,1,1,1,1,1,1,1,1,1,1,
1,1,1,1,1,1,1,1,1,1,1,1,1,1,1,1,1,1,1,1,1,1,1,1,1,1,1,1,1,1,1,1,1,1,1,1,
1,1,1,1,1,1,1,1,1,1,1,1,1,1,1,1,1,1,1,1,1,1,1,1,1,1,1,1,1,1,1,1,4),(0.,
0.0448889834294934),(11.8615800042567,12.8591513772396,13.8567227502225,
14.8542941232055,15.8518654961884,16.8494368691713,17.8470082421543,18.8445796151372,
19.8421509881201,20.8397223611031,21.837293734086,22.8348651070689,23.8324364800519,
24.8300078530348,25.8275792260177,26.8251505990007,27.8227219719836,28.8202933449665,
29.8178647179495,30.8154360909324,31.8130074639153,32.8105788368983,33.8081502098812,
34.8057215828641,35.803292955847,36.80086432883,37.7984357018129,38.7960070747959,
39.7935784477788,40.7911498207617,41.7887211937446,42.7862925667276,43.7838639397105,
44.7814353126934,45.7790066856764,46.7765780586593,47.7741494316422,48.7717208046252,
49.7692921776081,50.766863550591,51.764434923574,52.7620062965569,53.7595776695398,
54.7571490425228,55.7547204155057,56.7522917884886,57.7498631614716,58.7474345344545,
59.7450059074374,60.7425772804204,61.7401486534033,62.7377200263862,63.7352913993692,
64.7328627723521,65.730434145335,66.728005518318,67.7255768913009,68.7231482642838,
69.7207196372668,70.7182910102497,71.7158623832326,72.7134337562156,73.7110051291985,
74.7085765021814,75.7061478751644,76.7037192481473,77.7012906211302,78.6988619941132,
79.6964333670961,80.694004740079,81.691576113062,82.6891474860449,83.6867188590278,
84.6842902320108,85.6818616049937,86.6794329779766,87.6770043509595,88.6745757239425,
89.6721470969254,90.6697184699083,91.6672898428913,92.6648612158742,93.6624325888571,
94.6600039618401),.UNSPECIFIED.);
#625=B_SPLINE_SURFACE_WITH_KNOTS('',3,3,((#41203,#41204,#41205,#41206,#41207,
#41208,#41209,#41210,#41211,#41212,#41213,#41214,#41215,#41216,#41217,#41218,
#41219,#41220,#41221,#41222,#41223,#41224,#41225,#41226,#41227,#41228,#41229,
#41230,#41231,#41232,#41233,#41234,#41235,#41236,#41237,#41238,#41239,#41240,
#41241,#41242,#41243,#41244,#41245,#41246,#41247,#41248,#41249,#41250,#41251,
#41252,#41253,#41254,#41255,#41256,#41257,#41258,#41259,#41260,#41261,#41262,
#41263,#41264,#41265,#41266,#41267,#41268,#41269,#41270,#41271,#41272,#41273,
#41274,#41275,#41276,#41277,#41278,#41279,#41280,#41281,#41282,#41283,#41284,
#41285,#41286,#41287,#41288),(#41289,#41290,#41291,#41292,#41293,#41294,
#41295,#41296,#41297,#41298,#41299,#41300,#41301,#41302,#41303,#41304,#41305,
#41306,#41307,#41308,#41309,#41310,#41311,#41312,#41313,#41314,#41315,#41316,
#41317,#41318,#41319,#41320,#41321,#41322,#41323,#41324,#41325,#41326,#41327,
#41328,#41329,#41330,#41331,#41332,#41333,#41334,#41335,#41336,#41337,#41338,
#41339,#41340,#41341,#41342,#41343,#41344,#41345,#41346,#41347,#41348,#41349,
#41350,#41351,#41352,#41353,#41354,#41355,#41356,#41357,#41358,#41359,#41360,
#41361,#41362,#41363,#41364,#41365,#41366,#41367,#41368,#41369,#41370,#41371,
#41372,#41373,#41374),(#41375,#41376,#41377,#41378,#41379,#41380,#41381,
#41382,#41383,#41384,#41385,#41386,#41387,#41388,#41389,#41390,#41391,#41392,
#41393,#41394,#41395,#41396,#41397,#41398,#41399,#41400,#41401,#41402,#41403,
#41404,#41405,#41406,#41407,#41408,#41409,#41410,#41411,#41412,#41413,#41414,
#41415,#41416,#41417,#41418,#41419,#41420,#41421,#41422,#41423,#41424,#41425,
#41426,#41427,#41428,#41429,#41430,#41431,#41432,#41433,#41434,#41435,#41436,
#41437,#41438,#41439,#41440,#41441,#41442,#41443,#41444,#41445,#41446,#41447,
#41448,#41449,#41450,#41451,#41452,#41453,#41454,#41455,#41456,#41457,#41458,
#41459,#41460),(#41461,#41462,#41463,#41464,#41465,#41466,#41467,#41468,
#41469,#41470,#41471,#41472,#41473,#41474,#41475,#41476,#41477,#41478,#41479,
#41480,#41481,#41482,#41483,#41484,#41485,#41486,#41487,#41488,#41489,#41490,
#41491,#41492,#41493,#41494,#41495,#41496,#41497,#41498,#41499,#41500,#41501,
#41502,#41503,#41504,#41505,#41506,#41507,#41508,#41509,#41510,#41511,#41512,
#41513,#41514,#41515,#41516,#41517,#41518,#41519,#41520,#41521,#41522,#41523,
#41524,#41525,#41526,#41527,#41528,#41529,#41530,#41531,#41532,#41533,#41534,
#41535,#41536,#41537,#41538,#41539,#41540,#41541,#41542,#41543,#41544,#41545,
#41546)),.UNSPECIFIED.,.F.,.F.,.F.,(4,4),(4,1,1,1,1,1,1,1,1,1,1,1,1,1,1,
1,1,1,1,1,1,1,1,1,1,1,1,1,1,1,1,1,1,1,1,1,1,1,1,1,1,1,1,1,1,1,1,1,1,1,1,
1,1,1,1,1,1,1,1,1,1,1,1,1,1,1,1,1,1,1,1,1,1,1,1,1,1,1,1,1,1,1,1,4),(0.,
0.0448889834294934),(14.3981410127769,15.3957123857599,16.3932837587428,
17.3908551317257,18.3884265047086,19.3859978776916,20.3835692506745,21.3811406236574,
22.3787119966404,23.3762833696233,24.3738547426062,25.3714261155892,26.3689974885721,
27.366568861555,28.364140234538,29.3617116075209,30.3592829805038,31.3568543534868,
32.3544257264697,33.3519970994526,34.3495684724356,35.3471398454185,36.3447112184014,
37.3422825913844,38.3398539643673,39.3374253373502,40.3349967103332,41.3325680833161,
42.330139456299,43.327710829282,44.3252822022649,45.3228535752478,46.3204249482308,
47.3179963212137,48.3155676941966,49.3131390671796,50.3107104401625,51.3082818131454,
52.3058531861284,53.3034245591113,54.3009959320942,55.2985673050772,56.2961386780601,
57.293710051043,58.291281424026,59.2888527970089,60.2864241699918,61.2839955429748,
62.2815669159577,63.2791382889406,64.2767096619235,65.2742810349065,66.2718524078894,
67.2694237808723,68.2669951538553,69.2645665268382,70.2621378998211,71.2597092728041,
72.257280645787,73.25485201877,74.2524233917529,75.2499947647358,76.2475661377187,
77.2451375107017,78.2427088836846,79.2402802566675,80.2378516296505,81.2354230026334,
82.2329943756163,83.2305657485993,84.2281371215822,85.2257084945651,86.2232798675481,
87.220851240531,88.2184226135139,89.2159939864969,90.2135653594798,91.2111367324627,
92.2087081054457,93.2062794784286,94.2038508514115,95.2014222243945,96.1989935973774,
97.1965649703603),.UNSPECIFIED.);
#626=B_SPLINE_SURFACE_WITH_KNOTS('',3,3,((#41851,#41852,#41853,#41854,#41855,
#41856,#41857,#41858,#41859,#41860,#41861,#41862,#41863,#41864,#41865,#41866,
#41867,#41868,#41869,#41870,#41871,#41872,#41873,#41874,#41875,#41876,#41877,
#41878,#41879,#41880,#41881,#41882,#41883,#41884,#41885,#41886,#41887,#41888,
#41889,#41890,#41891,#41892,#41893,#41894,#41895,#41896,#41897,#41898,#41899,
#41900,#41901,#41902,#41903,#41904,#41905,#41906,#41907,#41908,#41909,#41910,
#41911,#41912,#41913,#41914,#41915,#41916,#41917,#41918,#41919,#41920,#41921,
#41922,#41923,#41924,#41925,#41926,#41927,#41928,#41929,#41930,#41931,#41932,
#41933,#41934,#41935,#41936),(#41937,#41938,#41939,#41940,#41941,#41942,
#41943,#41944,#41945,#41946,#41947,#41948,#41949,#41950,#41951,#41952,#41953,
#41954,#41955,#41956,#41957,#41958,#41959,#41960,#41961,#41962,#41963,#41964,
#41965,#41966,#41967,#41968,#41969,#41970,#41971,#41972,#41973,#41974,#41975,
#41976,#41977,#41978,#41979,#41980,#41981,#41982,#41983,#41984,#41985,#41986,
#41987,#41988,#41989,#41990,#41991,#41992,#41993,#41994,#41995,#41996,#41997,
#41998,#41999,#42000,#42001,#42002,#42003,#42004,#42005,#42006,#42007,#42008,
#42009,#42010,#42011,#42012,#42013,#42014,#42015,#42016,#42017,#42018,#42019,
#42020,#42021,#42022),(#42023,#42024,#42025,#42026,#42027,#42028,#42029,
#42030,#42031,#42032,#42033,#42034,#42035,#42036,#42037,#42038,#42039,#42040,
#42041,#42042,#42043,#42044,#42045,#42046,#42047,#42048,#42049,#42050,#42051,
#42052,#42053,#42054,#42055,#42056,#42057,#42058,#42059,#42060,#42061,#42062,
#42063,#42064,#42065,#42066,#42067,#42068,#42069,#42070,#42071,#42072,#42073,
#42074,#42075,#42076,#42077,#42078,#42079,#42080,#42081,#42082,#42083,#42084,
#42085,#42086,#42087,#42088,#42089,#42090,#42091,#42092,#42093,#42094,#42095,
#42096,#42097,#42098,#42099,#42100,#42101,#42102,#42103,#42104,#42105,#42106,
#42107,#42108),(#42109,#42110,#42111,#42112,#42113,#42114,#42115,#42116,
#42117,#42118,#42119,#42120,#42121,#42122,#42123,#42124,#42125,#42126,#42127,
#42128,#42129,#42130,#42131,#42132,#42133,#42134,#42135,#42136,#42137,#42138,
#42139,#42140,#42141,#42142,#42143,#42144,#42145,#42146,#42147,#42148,#42149,
#42150,#42151,#42152,#42153,#42154,#42155,#42156,#42157,#42158,#42159,#42160,
#42161,#42162,#42163,#42164,#42165,#42166,#42167,#42168,#42169,#42170,#42171,
#42172,#42173,#42174,#42175,#42176,#42177,#42178,#42179,#42180,#42181,#42182,
#42183,#42184,#42185,#42186,#42187,#42188,#42189,#42190,#42191,#42192,#42193,
#42194)),.UNSPECIFIED.,.F.,.F.,.F.,(4,4),(4,1,1,1,1,1,1,1,1,1,1,1,1,1,1,
1,1,1,1,1,1,1,1,1,1,1,1,1,1,1,1,1,1,1,1,1,1,1,1,1,1,1,1,1,1,1,1,1,1,1,1,
1,1,1,1,1,1,1,1,1,1,1,1,1,1,1,1,1,1,1,1,1,1,1,1,1,1,1,1,1,1,1,1,4),(0.,
0.0448889834294934),(11.8615800042567,12.8591513772396,13.8567227502225,
14.8542941232055,15.8518654961884,16.8494368691713,17.8470082421543,18.8445796151372,
19.8421509881201,20.8397223611031,21.837293734086,22.8348651070689,23.8324364800519,
24.8300078530348,25.8275792260177,26.8251505990007,27.8227219719836,28.8202933449665,
29.8178647179495,30.8154360909324,31.8130074639153,32.8105788368983,33.8081502098812,
34.8057215828641,35.8032929558471,36.80086432883,37.7984357018129,38.7960070747959,
39.7935784477788,40.7911498207617,41.7887211937447,42.7862925667276,43.7838639397105,
44.7814353126935,45.7790066856764,46.7765780586593,47.7741494316423,48.7717208046252,
49.7692921776081,50.7668635505911,51.764434923574,52.7620062965569,53.7595776695399,
54.7571490425228,55.7547204155057,56.7522917884886,57.7498631614716,58.7474345344545,
59.7450059074374,60.7425772804204,61.7401486534033,62.7377200263862,63.7352913993692,
64.7328627723521,65.730434145335,66.728005518318,67.7255768913009,68.7231482642838,
69.7207196372668,70.7182910102497,71.7158623832326,72.7134337562156,73.7110051291985,
74.7085765021814,75.7061478751644,76.7037192481473,77.7012906211302,78.6988619941132,
79.6964333670961,80.694004740079,81.691576113062,82.6891474860449,83.6867188590278,
84.6842902320108,85.6818616049937,86.6794329779766,87.6770043509596,88.6745757239425,
89.6721470969254,90.6697184699084,91.6672898428913,92.6648612158742,93.6624325888572,
94.6600039618401),.UNSPECIFIED.);
#627=B_SPLINE_SURFACE_WITH_KNOTS('',3,3,((#42302,#42303,#42304,#42305,#42306,
#42307,#42308,#42309,#42310,#42311,#42312,#42313,#42314,#42315,#42316,#42317,
#42318,#42319,#42320,#42321,#42322,#42323,#42324,#42325,#42326,#42327,#42328,
#42329,#42330,#42331,#42332,#42333,#42334,#42335,#42336,#42337,#42338,#42339,
#42340,#42341,#42342,#42343,#42344,#42345,#42346,#42347,#42348,#42349,#42350,
#42351,#42352,#42353,#42354,#42355,#42356,#42357,#42358,#42359,#42360,#42361,
#42362,#42363,#42364,#42365,#42366,#42367,#42368,#42369,#42370,#42371,#42372,
#42373,#42374,#42375,#42376,#42377,#42378,#42379,#42380,#42381,#42382,#42383,
#42384,#42385,#42386,#42387),(#42388,#42389,#42390,#42391,#42392,#42393,
#42394,#42395,#42396,#42397,#42398,#42399,#42400,#42401,#42402,#42403,#42404,
#42405,#42406,#42407,#42408,#42409,#42410,#42411,#42412,#42413,#42414,#42415,
#42416,#42417,#42418,#42419,#42420,#42421,#42422,#42423,#42424,#42425,#42426,
#42427,#42428,#42429,#42430,#42431,#42432,#42433,#42434,#42435,#42436,#42437,
#42438,#42439,#42440,#42441,#42442,#42443,#42444,#42445,#42446,#42447,#42448,
#42449,#42450,#42451,#42452,#42453,#42454,#42455,#42456,#42457,#42458,#42459,
#42460,#42461,#42462,#42463,#42464,#42465,#42466,#42467,#42468,#42469,#42470,
#42471,#42472,#42473),(#42474,#42475,#42476,#42477,#42478,#42479,#42480,
#42481,#42482,#42483,#42484,#42485,#42486,#42487,#42488,#42489,#42490,#42491,
#42492,#42493,#42494,#42495,#42496,#42497,#42498,#42499,#42500,#42501,#42502,
#42503,#42504,#42505,#42506,#42507,#42508,#42509,#42510,#42511,#42512,#42513,
#42514,#42515,#42516,#42517,#42518,#42519,#42520,#42521,#42522,#42523,#42524,
#42525,#42526,#42527,#42528,#42529,#42530,#42531,#42532,#42533,#42534,#42535,
#42536,#42537,#42538,#42539,#42540,#42541,#42542,#42543,#42544,#42545,#42546,
#42547,#42548,#42549,#42550,#42551,#42552,#42553,#42554,#42555,#42556,#42557,
#42558,#42559),(#42560,#42561,#42562,#42563,#42564,#42565,#42566,#42567,
#42568,#42569,#42570,#42571,#42572,#42573,#42574,#42575,#42576,#42577,#42578,
#42579,#42580,#42581,#42582,#42583,#42584,#42585,#42586,#42587,#42588,#42589,
#42590,#42591,#42592,#42593,#42594,#42595,#42596,#42597,#42598,#42599,#42600,
#42601,#42602,#42603,#42604,#42605,#42606,#42607,#42608,#42609,#42610,#42611,
#42612,#42613,#42614,#42615,#42616,#42617,#42618,#42619,#42620,#42621,#42622,
#42623,#42624,#42625,#42626,#42627,#42628,#42629,#42630,#42631,#42632,#42633,
#42634,#42635,#42636,#42637,#42638,#42639,#42640,#42641,#42642,#42643,#42644,
#42645)),.UNSPECIFIED.,.F.,.F.,.F.,(4,4),(4,1,1,1,1,1,1,1,1,1,1,1,1,1,1,
1,1,1,1,1,1,1,1,1,1,1,1,1,1,1,1,1,1,1,1,1,1,1,1,1,1,1,1,1,1,1,1,1,1,1,1,
1,1,1,1,1,1,1,1,1,1,1,1,1,1,1,1,1,1,1,1,1,1,1,1,1,1,1,1,1,1,1,1,4),(0.,
0.0448889834294934),(14.3981410127769,15.3957123857599,16.3932837587428,
17.3908551317257,18.3884265047087,19.3859978776916,20.3835692506745,21.3811406236575,
22.3787119966404,23.3762833696233,24.3738547426063,25.3714261155892,26.3689974885721,
27.3665688615551,28.364140234538,29.3617116075209,30.3592829805038,31.3568543534868,
32.3544257264697,33.3519970994526,34.3495684724356,35.3471398454185,36.3447112184014,
37.3422825913844,38.3398539643673,39.3374253373502,40.3349967103332,41.3325680833161,
42.330139456299,43.327710829282,44.3252822022649,45.3228535752478,46.3204249482308,
47.3179963212137,48.3155676941966,49.3131390671796,50.3107104401625,51.3082818131454,
52.3058531861284,53.3034245591113,54.3009959320942,55.2985673050772,56.2961386780601,
57.293710051043,58.291281424026,59.2888527970089,60.2864241699918,61.2839955429748,
62.2815669159577,63.2791382889406,64.2767096619236,65.2742810349065,66.2718524078894,
67.2694237808724,68.2669951538553,69.2645665268382,70.2621378998212,71.2597092728041,
72.257280645787,73.25485201877,74.2524233917529,75.2499947647358,76.2475661377187,
77.2451375107017,78.2427088836846,79.2402802566675,80.2378516296505,81.2354230026334,
82.2329943756163,83.2305657485993,84.2281371215822,85.2257084945651,86.2232798675481,
87.220851240531,88.2184226135139,89.2159939864969,90.2135653594798,91.2111367324627,
92.2087081054457,93.2062794784286,94.2038508514115,95.2014222243945,96.1989935973774,
97.1965649703603),.UNSPECIFIED.);
#628=B_SPLINE_SURFACE_WITH_KNOTS('',3,3,((#42950,#42951,#42952,#42953,#42954,
#42955,#42956,#42957,#42958,#42959,#42960,#42961,#42962,#42963,#42964,#42965,
#42966,#42967,#42968,#42969,#42970,#42971,#42972,#42973,#42974,#42975,#42976,
#42977,#42978,#42979,#42980,#42981,#42982,#42983,#42984,#42985,#42986,#42987,
#42988,#42989,#42990,#42991,#42992,#42993,#42994,#42995,#42996,#42997,#42998,
#42999,#43000,#43001,#43002,#43003,#43004,#43005,#43006,#43007,#43008,#43009,
#43010,#43011,#43012,#43013,#43014,#43015,#43016,#43017,#43018,#43019,#43020,
#43021,#43022,#43023,#43024,#43025,#43026,#43027,#43028,#43029,#43030,#43031,
#43032,#43033,#43034,#43035),(#43036,#43037,#43038,#43039,#43040,#43041,
#43042,#43043,#43044,#43045,#43046,#43047,#43048,#43049,#43050,#43051,#43052,
#43053,#43054,#43055,#43056,#43057,#43058,#43059,#43060,#43061,#43062,#43063,
#43064,#43065,#43066,#43067,#43068,#43069,#43070,#43071,#43072,#43073,#43074,
#43075,#43076,#43077,#43078,#43079,#43080,#43081,#43082,#43083,#43084,#43085,
#43086,#43087,#43088,#43089,#43090,#43091,#43092,#43093,#43094,#43095,#43096,
#43097,#43098,#43099,#43100,#43101,#43102,#43103,#43104,#43105,#43106,#43107,
#43108,#43109,#43110,#43111,#43112,#43113,#43114,#43115,#43116,#43117,#43118,
#43119,#43120,#43121),(#43122,#43123,#43124,#43125,#43126,#43127,#43128,
#43129,#43130,#43131,#43132,#43133,#43134,#43135,#43136,#43137,#43138,#43139,
#43140,#43141,#43142,#43143,#43144,#43145,#43146,#43147,#43148,#43149,#43150,
#43151,#43152,#43153,#43154,#43155,#43156,#43157,#43158,#43159,#43160,#43161,
#43162,#43163,#43164,#43165,#43166,#43167,#43168,#43169,#43170,#43171,#43172,
#43173,#43174,#43175,#43176,#43177,#43178,#43179,#43180,#43181,#43182,#43183,
#43184,#43185,#43186,#43187,#43188,#43189,#43190,#43191,#43192,#43193,#43194,
#43195,#43196,#43197,#43198,#43199,#43200,#43201,#43202,#43203,#43204,#43205,
#43206,#43207),(#43208,#43209,#43210,#43211,#43212,#43213,#43214,#43215,
#43216,#43217,#43218,#43219,#43220,#43221,#43222,#43223,#43224,#43225,#43226,
#43227,#43228,#43229,#43230,#43231,#43232,#43233,#43234,#43235,#43236,#43237,
#43238,#43239,#43240,#43241,#43242,#43243,#43244,#43245,#43246,#43247,#43248,
#43249,#43250,#43251,#43252,#43253,#43254,#43255,#43256,#43257,#43258,#43259,
#43260,#43261,#43262,#43263,#43264,#43265,#43266,#43267,#43268,#43269,#43270,
#43271,#43272,#43273,#43274,#43275,#43276,#43277,#43278,#43279,#43280,#43281,
#43282,#43283,#43284,#43285,#43286,#43287,#43288,#43289,#43290,#43291,#43292,
#43293)),.UNSPECIFIED.,.F.,.F.,.F.,(4,4),(4,1,1,1,1,1,1,1,1,1,1,1,1,1,1,
1,1,1,1,1,1,1,1,1,1,1,1,1,1,1,1,1,1,1,1,1,1,1,1,1,1,1,1,1,1,1,1,1,1,1,1,
1,1,1,1,1,1,1,1,1,1,1,1,1,1,1,1,1,1,1,1,1,1,1,1,1,1,1,1,1,1,1,1,4),(0.,
0.0448889834294934),(11.8615800042567,12.8591513772396,13.8567227502225,
14.8542941232055,15.8518654961884,16.8494368691713,17.8470082421543,18.8445796151372,
19.8421509881201,20.8397223611031,21.837293734086,22.8348651070689,23.8324364800519,
24.8300078530348,25.8275792260177,26.8251505990007,27.8227219719836,28.8202933449665,
29.8178647179495,30.8154360909324,31.8130074639153,32.8105788368983,33.8081502098812,
34.8057215828641,35.8032929558471,36.80086432883,37.7984357018129,38.7960070747959,
39.7935784477788,40.7911498207617,41.7887211937447,42.7862925667276,43.7838639397105,
44.7814353126935,45.7790066856764,46.7765780586593,47.7741494316423,48.7717208046252,
49.7692921776081,50.7668635505911,51.764434923574,52.7620062965569,53.7595776695399,
54.7571490425228,55.7547204155057,56.7522917884886,57.7498631614716,58.7474345344545,
59.7450059074374,60.7425772804204,61.7401486534033,62.7377200263862,63.7352913993692,
64.7328627723521,65.730434145335,66.728005518318,67.7255768913009,68.7231482642838,
69.7207196372668,70.7182910102497,71.7158623832326,72.7134337562156,73.7110051291985,
74.7085765021814,75.7061478751644,76.7037192481473,77.7012906211302,78.6988619941132,
79.6964333670961,80.694004740079,81.691576113062,82.6891474860449,83.6867188590278,
84.6842902320108,85.6818616049937,86.6794329779766,87.6770043509596,88.6745757239425,
89.6721470969254,90.6697184699084,91.6672898428913,92.6648612158742,93.6624325888572,
94.6600039618401),.UNSPECIFIED.);
#629=B_SPLINE_SURFACE_WITH_KNOTS('',3,3,((#43401,#43402,#43403,#43404,#43405,
#43406,#43407,#43408,#43409,#43410,#43411,#43412,#43413,#43414,#43415,#43416,
#43417,#43418,#43419,#43420,#43421,#43422,#43423,#43424,#43425,#43426,#43427,
#43428,#43429,#43430,#43431,#43432,#43433,#43434,#43435,#43436,#43437,#43438,
#43439,#43440,#43441,#43442,#43443,#43444,#43445,#43446,#43447,#43448,#43449,
#43450,#43451,#43452,#43453,#43454,#43455,#43456,#43457,#43458,#43459,#43460,
#43461,#43462,#43463,#43464,#43465,#43466,#43467,#43468,#43469,#43470,#43471,
#43472,#43473,#43474,#43475,#43476,#43477,#43478,#43479,#43480,#43481,#43482,
#43483,#43484,#43485,#43486),(#43487,#43488,#43489,#43490,#43491,#43492,
#43493,#43494,#43495,#43496,#43497,#43498,#43499,#43500,#43501,#43502,#43503,
#43504,#43505,#43506,#43507,#43508,#43509,#43510,#43511,#43512,#43513,#43514,
#43515,#43516,#43517,#43518,#43519,#43520,#43521,#43522,#43523,#43524,#43525,
#43526,#43527,#43528,#43529,#43530,#43531,#43532,#43533,#43534,#43535,#43536,
#43537,#43538,#43539,#43540,#43541,#43542,#43543,#43544,#43545,#43546,#43547,
#43548,#43549,#43550,#43551,#43552,#43553,#43554,#43555,#43556,#43557,#43558,
#43559,#43560,#43561,#43562,#43563,#43564,#43565,#43566,#43567,#43568,#43569,
#43570,#43571,#43572),(#43573,#43574,#43575,#43576,#43577,#43578,#43579,
#43580,#43581,#43582,#43583,#43584,#43585,#43586,#43587,#43588,#43589,#43590,
#43591,#43592,#43593,#43594,#43595,#43596,#43597,#43598,#43599,#43600,#43601,
#43602,#43603,#43604,#43605,#43606,#43607,#43608,#43609,#43610,#43611,#43612,
#43613,#43614,#43615,#43616,#43617,#43618,#43619,#43620,#43621,#43622,#43623,
#43624,#43625,#43626,#43627,#43628,#43629,#43630,#43631,#43632,#43633,#43634,
#43635,#43636,#43637,#43638,#43639,#43640,#43641,#43642,#43643,#43644,#43645,
#43646,#43647,#43648,#43649,#43650,#43651,#43652,#43653,#43654,#43655,#43656,
#43657,#43658),(#43659,#43660,#43661,#43662,#43663,#43664,#43665,#43666,
#43667,#43668,#43669,#43670,#43671,#43672,#43673,#43674,#43675,#43676,#43677,
#43678,#43679,#43680,#43681,#43682,#43683,#43684,#43685,#43686,#43687,#43688,
#43689,#43690,#43691,#43692,#43693,#43694,#43695,#43696,#43697,#43698,#43699,
#43700,#43701,#43702,#43703,#43704,#43705,#43706,#43707,#43708,#43709,#43710,
#43711,#43712,#43713,#43714,#43715,#43716,#43717,#43718,#43719,#43720,#43721,
#43722,#43723,#43724,#43725,#43726,#43727,#43728,#43729,#43730,#43731,#43732,
#43733,#43734,#43735,#43736,#43737,#43738,#43739,#43740,#43741,#43742,#43743,
#43744)),.UNSPECIFIED.,.F.,.F.,.F.,(4,4),(4,1,1,1,1,1,1,1,1,1,1,1,1,1,1,
1,1,1,1,1,1,1,1,1,1,1,1,1,1,1,1,1,1,1,1,1,1,1,1,1,1,1,1,1,1,1,1,1,1,1,1,
1,1,1,1,1,1,1,1,1,1,1,1,1,1,1,1,1,1,1,1,1,1,1,1,1,1,1,1,1,1,1,1,4),(0.,
0.0448889834294934),(14.3981410127769,15.3957123857599,16.3932837587428,
17.3908551317257,18.3884265047087,19.3859978776916,20.3835692506745,21.3811406236575,
22.3787119966404,23.3762833696233,24.3738547426063,25.3714261155892,26.3689974885721,
27.3665688615551,28.364140234538,29.3617116075209,30.3592829805038,31.3568543534868,
32.3544257264697,33.3519970994526,34.3495684724356,35.3471398454185,36.3447112184014,
37.3422825913844,38.3398539643673,39.3374253373502,40.3349967103332,41.3325680833161,
42.330139456299,43.327710829282,44.3252822022649,45.3228535752478,46.3204249482308,
47.3179963212137,48.3155676941966,49.3131390671796,50.3107104401625,51.3082818131454,
52.3058531861284,53.3034245591113,54.3009959320942,55.2985673050772,56.2961386780601,
57.293710051043,58.291281424026,59.2888527970089,60.2864241699918,61.2839955429748,
62.2815669159577,63.2791382889406,64.2767096619236,65.2742810349065,66.2718524078894,
67.2694237808724,68.2669951538553,69.2645665268382,70.2621378998212,71.2597092728041,
72.257280645787,73.25485201877,74.2524233917529,75.2499947647358,76.2475661377187,
77.2451375107017,78.2427088836846,79.2402802566675,80.2378516296505,81.2354230026334,
82.2329943756163,83.2305657485993,84.2281371215822,85.2257084945651,86.2232798675481,
87.220851240531,88.2184226135139,89.2159939864969,90.2135653594798,91.2111367324627,
92.2087081054457,93.2062794784286,94.2038508514115,95.2014222243945,96.1989935973774,
97.1965649703603),.UNSPECIFIED.);
#630=B_SPLINE_SURFACE_WITH_KNOTS('',3,3,((#44049,#44050,#44051,#44052,#44053,
#44054,#44055,#44056,#44057,#44058,#44059,#44060,#44061,#44062,#44063,#44064,
#44065,#44066,#44067,#44068,#44069,#44070,#44071,#44072,#44073,#44074,#44075,
#44076,#44077,#44078,#44079,#44080,#44081,#44082,#44083,#44084,#44085,#44086,
#44087,#44088,#44089,#44090,#44091,#44092,#44093,#44094,#44095,#44096,#44097,
#44098,#44099,#44100,#44101,#44102,#44103,#44104,#44105,#44106,#44107,#44108,
#44109,#44110,#44111,#44112,#44113,#44114,#44115,#44116,#44117,#44118,#44119,
#44120,#44121,#44122,#44123,#44124,#44125,#44126,#44127,#44128,#44129,#44130,
#44131,#44132,#44133,#44134),(#44135,#44136,#44137,#44138,#44139,#44140,
#44141,#44142,#44143,#44144,#44145,#44146,#44147,#44148,#44149,#44150,#44151,
#44152,#44153,#44154,#44155,#44156,#44157,#44158,#44159,#44160,#44161,#44162,
#44163,#44164,#44165,#44166,#44167,#44168,#44169,#44170,#44171,#44172,#44173,
#44174,#44175,#44176,#44177,#44178,#44179,#44180,#44181,#44182,#44183,#44184,
#44185,#44186,#44187,#44188,#44189,#44190,#44191,#44192,#44193,#44194,#44195,
#44196,#44197,#44198,#44199,#44200,#44201,#44202,#44203,#44204,#44205,#44206,
#44207,#44208,#44209,#44210,#44211,#44212,#44213,#44214,#44215,#44216,#44217,
#44218,#44219,#44220),(#44221,#44222,#44223,#44224,#44225,#44226,#44227,
#44228,#44229,#44230,#44231,#44232,#44233,#44234,#44235,#44236,#44237,#44238,
#44239,#44240,#44241,#44242,#44243,#44244,#44245,#44246,#44247,#44248,#44249,
#44250,#44251,#44252,#44253,#44254,#44255,#44256,#44257,#44258,#44259,#44260,
#44261,#44262,#44263,#44264,#44265,#44266,#44267,#44268,#44269,#44270,#44271,
#44272,#44273,#44274,#44275,#44276,#44277,#44278,#44279,#44280,#44281,#44282,
#44283,#44284,#44285,#44286,#44287,#44288,#44289,#44290,#44291,#44292,#44293,
#44294,#44295,#44296,#44297,#44298,#44299,#44300,#44301,#44302,#44303,#44304,
#44305,#44306),(#44307,#44308,#44309,#44310,#44311,#44312,#44313,#44314,
#44315,#44316,#44317,#44318,#44319,#44320,#44321,#44322,#44323,#44324,#44325,
#44326,#44327,#44328,#44329,#44330,#44331,#44332,#44333,#44334,#44335,#44336,
#44337,#44338,#44339,#44340,#44341,#44342,#44343,#44344,#44345,#44346,#44347,
#44348,#44349,#44350,#44351,#44352,#44353,#44354,#44355,#44356,#44357,#44358,
#44359,#44360,#44361,#44362,#44363,#44364,#44365,#44366,#44367,#44368,#44369,
#44370,#44371,#44372,#44373,#44374,#44375,#44376,#44377,#44378,#44379,#44380,
#44381,#44382,#44383,#44384,#44385,#44386,#44387,#44388,#44389,#44390,#44391,
#44392)),.UNSPECIFIED.,.F.,.F.,.F.,(4,4),(4,1,1,1,1,1,1,1,1,1,1,1,1,1,1,
1,1,1,1,1,1,1,1,1,1,1,1,1,1,1,1,1,1,1,1,1,1,1,1,1,1,1,1,1,1,1,1,1,1,1,1,
1,1,1,1,1,1,1,1,1,1,1,1,1,1,1,1,1,1,1,1,1,1,1,1,1,1,1,1,1,1,1,1,4),(0.,
0.0448889834294934),(11.8615800042567,12.8591513772396,13.8567227502225,
14.8542941232055,15.8518654961884,16.8494368691713,17.8470082421543,18.8445796151372,
19.8421509881201,20.8397223611031,21.837293734086,22.8348651070689,23.8324364800519,
24.8300078530348,25.8275792260177,26.8251505990007,27.8227219719836,28.8202933449665,
29.8178647179495,30.8154360909324,31.8130074639153,32.8105788368983,33.8081502098812,
34.8057215828641,35.8032929558471,36.80086432883,37.7984357018129,38.7960070747959,
39.7935784477788,40.7911498207617,41.7887211937447,42.7862925667276,43.7838639397105,
44.7814353126935,45.7790066856764,46.7765780586593,47.7741494316423,48.7717208046252,
49.7692921776081,50.7668635505911,51.764434923574,52.7620062965569,53.7595776695399,
54.7571490425228,55.7547204155057,56.7522917884886,57.7498631614716,58.7474345344545,
59.7450059074374,60.7425772804204,61.7401486534033,62.7377200263862,63.7352913993692,
64.7328627723521,65.7304341453351,66.728005518318,67.7255768913009,68.7231482642839,
69.7207196372668,70.7182910102497,71.7158623832326,72.7134337562156,73.7110051291985,
74.7085765021814,75.7061478751644,76.7037192481473,77.7012906211302,78.6988619941132,
79.6964333670961,80.694004740079,81.691576113062,82.6891474860449,83.6867188590278,
84.6842902320108,85.6818616049937,86.6794329779766,87.6770043509596,88.6745757239425,
89.6721470969254,90.6697184699084,91.6672898428913,92.6648612158742,93.6624325888572,
94.6600039618401),.UNSPECIFIED.);
#631=B_SPLINE_SURFACE_WITH_KNOTS('',3,3,((#44500,#44501,#44502,#44503,#44504,
#44505,#44506,#44507,#44508,#44509,#44510,#44511,#44512,#44513,#44514,#44515,
#44516,#44517,#44518,#44519,#44520,#44521,#44522,#44523,#44524,#44525,#44526,
#44527,#44528,#44529,#44530,#44531,#44532,#44533,#44534,#44535,#44536,#44537,
#44538,#44539,#44540,#44541,#44542,#44543,#44544,#44545,#44546,#44547,#44548,
#44549,#44550,#44551,#44552,#44553,#44554,#44555,#44556,#44557,#44558,#44559,
#44560,#44561,#44562,#44563,#44564,#44565,#44566,#44567,#44568,#44569,#44570,
#44571,#44572,#44573,#44574,#44575,#44576,#44577,#44578,#44579,#44580,#44581,
#44582,#44583,#44584,#44585),(#44586,#44587,#44588,#44589,#44590,#44591,
#44592,#44593,#44594,#44595,#44596,#44597,#44598,#44599,#44600,#44601,#44602,
#44603,#44604,#44605,#44606,#44607,#44608,#44609,#44610,#44611,#44612,#44613,
#44614,#44615,#44616,#44617,#44618,#44619,#44620,#44621,#44622,#44623,#44624,
#44625,#44626,#44627,#44628,#44629,#44630,#44631,#44632,#44633,#44634,#44635,
#44636,#44637,#44638,#44639,#44640,#44641,#44642,#44643,#44644,#44645,#44646,
#44647,#44648,#44649,#44650,#44651,#44652,#44653,#44654,#44655,#44656,#44657,
#44658,#44659,#44660,#44661,#44662,#44663,#44664,#44665,#44666,#44667,#44668,
#44669,#44670,#44671),(#44672,#44673,#44674,#44675,#44676,#44677,#44678,
#44679,#44680,#44681,#44682,#44683,#44684,#44685,#44686,#44687,#44688,#44689,
#44690,#44691,#44692,#44693,#44694,#44695,#44696,#44697,#44698,#44699,#44700,
#44701,#44702,#44703,#44704,#44705,#44706,#44707,#44708,#44709,#44710,#44711,
#44712,#44713,#44714,#44715,#44716,#44717,#44718,#44719,#44720,#44721,#44722,
#44723,#44724,#44725,#44726,#44727,#44728,#44729,#44730,#44731,#44732,#44733,
#44734,#44735,#44736,#44737,#44738,#44739,#44740,#44741,#44742,#44743,#44744,
#44745,#44746,#44747,#44748,#44749,#44750,#44751,#44752,#44753,#44754,#44755,
#44756,#44757),(#44758,#44759,#44760,#44761,#44762,#44763,#44764,#44765,
#44766,#44767,#44768,#44769,#44770,#44771,#44772,#44773,#44774,#44775,#44776,
#44777,#44778,#44779,#44780,#44781,#44782,#44783,#44784,#44785,#44786,#44787,
#44788,#44789,#44790,#44791,#44792,#44793,#44794,#44795,#44796,#44797,#44798,
#44799,#44800,#44801,#44802,#44803,#44804,#44805,#44806,#44807,#44808,#44809,
#44810,#44811,#44812,#44813,#44814,#44815,#44816,#44817,#44818,#44819,#44820,
#44821,#44822,#44823,#44824,#44825,#44826,#44827,#44828,#44829,#44830,#44831,
#44832,#44833,#44834,#44835,#44836,#44837,#44838,#44839,#44840,#44841,#44842,
#44843)),.UNSPECIFIED.,.F.,.F.,.F.,(4,4),(4,1,1,1,1,1,1,1,1,1,1,1,1,1,1,
1,1,1,1,1,1,1,1,1,1,1,1,1,1,1,1,1,1,1,1,1,1,1,1,1,1,1,1,1,1,1,1,1,1,1,1,
1,1,1,1,1,1,1,1,1,1,1,1,1,1,1,1,1,1,1,1,1,1,1,1,1,1,1,1,1,1,1,1,4),(0.,
0.0448889834294934),(14.3981410127769,15.3957123857599,16.3932837587428,
17.3908551317257,18.3884265047087,19.3859978776916,20.3835692506745,21.3811406236575,
22.3787119966404,23.3762833696233,24.3738547426063,25.3714261155892,26.3689974885721,
27.3665688615551,28.364140234538,29.3617116075209,30.3592829805038,31.3568543534868,
32.3544257264697,33.3519970994526,34.3495684724356,35.3471398454185,36.3447112184014,
37.3422825913844,38.3398539643673,39.3374253373502,40.3349967103332,41.3325680833161,
42.330139456299,43.327710829282,44.3252822022649,45.3228535752478,46.3204249482308,
47.3179963212137,48.3155676941966,49.3131390671796,50.3107104401625,51.3082818131454,
52.3058531861284,53.3034245591113,54.3009959320942,55.2985673050772,56.2961386780601,
57.293710051043,58.291281424026,59.2888527970089,60.2864241699918,61.2839955429748,
62.2815669159577,63.2791382889406,64.2767096619236,65.2742810349065,66.2718524078894,
67.2694237808724,68.2669951538553,69.2645665268382,70.2621378998212,71.2597092728041,
72.257280645787,73.25485201877,74.2524233917529,75.2499947647358,76.2475661377187,
77.2451375107017,78.2427088836846,79.2402802566675,80.2378516296505,81.2354230026334,
82.2329943756163,83.2305657485993,84.2281371215822,85.2257084945651,86.2232798675481,
87.220851240531,88.2184226135139,89.2159939864969,90.2135653594798,91.2111367324627,
92.2087081054457,93.2062794784286,94.2038508514115,95.2014222243945,96.1989935973774,
97.1965649703603),.UNSPECIFIED.);
#632=B_SPLINE_SURFACE_WITH_KNOTS('',3,3,((#45153,#45154,#45155,#45156,#45157,
#45158,#45159,#45160,#45161,#45162,#45163,#45164,#45165,#45166,#45167,#45168,
#45169,#45170,#45171,#45172,#45173,#45174,#45175,#45176,#45177,#45178,#45179,
#45180,#45181,#45182,#45183,#45184,#45185,#45186,#45187,#45188,#45189,#45190,
#45191,#45192,#45193,#45194,#45195,#45196,#45197,#45198,#45199,#45200,#45201,
#45202,#45203,#45204,#45205,#45206,#45207,#45208,#45209,#45210,#45211,#45212,
#45213,#45214,#45215,#45216,#45217,#45218,#45219,#45220,#45221,#45222,#45223,
#45224,#45225,#45226,#45227,#45228,#45229,#45230,#45231,#45232,#45233,#45234,
#45235,#45236,#45237,#45238),(#45239,#45240,#45241,#45242,#45243,#45244,
#45245,#45246,#45247,#45248,#45249,#45250,#45251,#45252,#45253,#45254,#45255,
#45256,#45257,#45258,#45259,#45260,#45261,#45262,#45263,#45264,#45265,#45266,
#45267,#45268,#45269,#45270,#45271,#45272,#45273,#45274,#45275,#45276,#45277,
#45278,#45279,#45280,#45281,#45282,#45283,#45284,#45285,#45286,#45287,#45288,
#45289,#45290,#45291,#45292,#45293,#45294,#45295,#45296,#45297,#45298,#45299,
#45300,#45301,#45302,#45303,#45304,#45305,#45306,#45307,#45308,#45309,#45310,
#45311,#45312,#45313,#45314,#45315,#45316,#45317,#45318,#45319,#45320,#45321,
#45322,#45323,#45324),(#45325,#45326,#45327,#45328,#45329,#45330,#45331,
#45332,#45333,#45334,#45335,#45336,#45337,#45338,#45339,#45340,#45341,#45342,
#45343,#45344,#45345,#45346,#45347,#45348,#45349,#45350,#45351,#45352,#45353,
#45354,#45355,#45356,#45357,#45358,#45359,#45360,#45361,#45362,#45363,#45364,
#45365,#45366,#45367,#45368,#45369,#45370,#45371,#45372,#45373,#45374,#45375,
#45376,#45377,#45378,#45379,#45380,#45381,#45382,#45383,#45384,#45385,#45386,
#45387,#45388,#45389,#45390,#45391,#45392,#45393,#45394,#45395,#45396,#45397,
#45398,#45399,#45400,#45401,#45402,#45403,#45404,#45405,#45406,#45407,#45408,
#45409,#45410),(#45411,#45412,#45413,#45414,#45415,#45416,#45417,#45418,
#45419,#45420,#45421,#45422,#45423,#45424,#45425,#45426,#45427,#45428,#45429,
#45430,#45431,#45432,#45433,#45434,#45435,#45436,#45437,#45438,#45439,#45440,
#45441,#45442,#45443,#45444,#45445,#45446,#45447,#45448,#45449,#45450,#45451,
#45452,#45453,#45454,#45455,#45456,#45457,#45458,#45459,#45460,#45461,#45462,
#45463,#45464,#45465,#45466,#45467,#45468,#45469,#45470,#45471,#45472,#45473,
#45474,#45475,#45476,#45477,#45478,#45479,#45480,#45481,#45482,#45483,#45484,
#45485,#45486,#45487,#45488,#45489,#45490,#45491,#45492,#45493,#45494,#45495,
#45496)),.UNSPECIFIED.,.F.,.F.,.F.,(4,4),(4,1,1,1,1,1,1,1,1,1,1,1,1,1,1,
1,1,1,1,1,1,1,1,1,1,1,1,1,1,1,1,1,1,1,1,1,1,1,1,1,1,1,1,1,1,1,1,1,1,1,1,
1,1,1,1,1,1,1,1,1,1,1,1,1,1,1,1,1,1,1,1,1,1,1,1,1,1,1,1,1,1,1,1,4),(0.,
0.0448889834294934),(11.8615800042566,12.8591513772395,13.8567227502225,
14.8542941232054,15.8518654961883,16.8494368691713,17.8470082421542,18.8445796151371,
19.8421509881201,20.839722361103,21.8372937340859,22.8348651070689,23.8324364800518,
24.8300078530347,25.8275792260177,26.8251505990006,27.8227219719835,28.8202933449665,
29.8178647179494,30.8154360909323,31.8130074639152,32.8105788368982,33.8081502098811,
34.805721582864,35.803292955847,36.8008643288299,37.7984357018128,38.7960070747958,
39.7935784477787,40.7911498207616,41.7887211937446,42.7862925667275,43.7838639397104,
44.7814353126934,45.7790066856763,46.7765780586592,47.7741494316422,48.7717208046251,
49.769292177608,50.766863550591,51.7644349235739,52.7620062965568,53.7595776695398,
54.7571490425227,55.7547204155056,56.7522917884886,57.7498631614715,58.7474345344544,
59.7450059074374,60.7425772804203,61.7401486534032,62.7377200263862,63.7352913993691,
64.732862772352,65.730434145335,66.7280055183179,67.7255768913008,68.7231482642838,
69.7207196372667,70.7182910102496,71.7158623832325,72.7134337562155,73.7110051291984,
74.7085765021813,75.7061478751643,76.7037192481472,77.7012906211301,78.6988619941131,
79.696433367096,80.6940047400789,81.6915761130619,82.6891474860448,83.6867188590277,
84.6842902320107,85.6818616049936,86.6794329779765,87.6770043509595,88.6745757239424,
89.6721470969253,90.6697184699083,91.6672898428912,92.6648612158741,93.6624325888571,
94.66000396184),.UNSPECIFIED.);
#633=B_SPLINE_SURFACE_WITH_KNOTS('',3,3,((#45604,#45605,#45606,#45607,#45608,
#45609,#45610,#45611,#45612,#45613,#45614,#45615,#45616,#45617,#45618,#45619,
#45620,#45621,#45622,#45623,#45624,#45625,#45626,#45627,#45628,#45629,#45630,
#45631,#45632,#45633,#45634,#45635,#45636,#45637,#45638,#45639,#45640,#45641,
#45642,#45643,#45644,#45645,#45646,#45647,#45648,#45649,#45650,#45651,#45652,
#45653,#45654,#45655,#45656,#45657,#45658,#45659,#45660,#45661,#45662,#45663,
#45664,#45665,#45666,#45667,#45668,#45669,#45670,#45671,#45672,#45673,#45674,
#45675,#45676,#45677,#45678,#45679,#45680,#45681,#45682,#45683,#45684,#45685,
#45686,#45687,#45688,#45689),(#45690,#45691,#45692,#45693,#45694,#45695,
#45696,#45697,#45698,#45699,#45700,#45701,#45702,#45703,#45704,#45705,#45706,
#45707,#45708,#45709,#45710,#45711,#45712,#45713,#45714,#45715,#45716,#45717,
#45718,#45719,#45720,#45721,#45722,#45723,#45724,#45725,#45726,#45727,#45728,
#45729,#45730,#45731,#45732,#45733,#45734,#45735,#45736,#45737,#45738,#45739,
#45740,#45741,#45742,#45743,#45744,#45745,#45746,#45747,#45748,#45749,#45750,
#45751,#45752,#45753,#45754,#45755,#45756,#45757,#45758,#45759,#45760,#45761,
#45762,#45763,#45764,#45765,#45766,#45767,#45768,#45769,#45770,#45771,#45772,
#45773,#45774,#45775),(#45776,#45777,#45778,#45779,#45780,#45781,#45782,
#45783,#45784,#45785,#45786,#45787,#45788,#45789,#45790,#45791,#45792,#45793,
#45794,#45795,#45796,#45797,#45798,#45799,#45800,#45801,#45802,#45803,#45804,
#45805,#45806,#45807,#45808,#45809,#45810,#45811,#45812,#45813,#45814,#45815,
#45816,#45817,#45818,#45819,#45820,#45821,#45822,#45823,#45824,#45825,#45826,
#45827,#45828,#45829,#45830,#45831,#45832,#45833,#45834,#45835,#45836,#45837,
#45838,#45839,#45840,#45841,#45842,#45843,#45844,#45845,#45846,#45847,#45848,
#45849,#45850,#45851,#45852,#45853,#45854,#45855,#45856,#45857,#45858,#45859,
#45860,#45861),(#45862,#45863,#45864,#45865,#45866,#45867,#45868,#45869,
#45870,#45871,#45872,#45873,#45874,#45875,#45876,#45877,#45878,#45879,#45880,
#45881,#45882,#45883,#45884,#45885,#45886,#45887,#45888,#45889,#45890,#45891,
#45892,#45893,#45894,#45895,#45896,#45897,#45898,#45899,#45900,#45901,#45902,
#45903,#45904,#45905,#45906,#45907,#45908,#45909,#45910,#45911,#45912,#45913,
#45914,#45915,#45916,#45917,#45918,#45919,#45920,#45921,#45922,#45923,#45924,
#45925,#45926,#45927,#45928,#45929,#45930,#45931,#45932,#45933,#45934,#45935,
#45936,#45937,#45938,#45939,#45940,#45941,#45942,#45943,#45944,#45945,#45946,
#45947)),.UNSPECIFIED.,.F.,.F.,.F.,(4,4),(4,1,1,1,1,1,1,1,1,1,1,1,1,1,1,
1,1,1,1,1,1,1,1,1,1,1,1,1,1,1,1,1,1,1,1,1,1,1,1,1,1,1,1,1,1,1,1,1,1,1,1,
1,1,1,1,1,1,1,1,1,1,1,1,1,1,1,1,1,1,1,1,1,1,1,1,1,1,1,1,1,1,1,1,4),(0.,
0.0448889834294934),(14.3981410127769,15.3957123857598,16.3932837587427,
17.3908551317257,18.3884265047086,19.3859978776915,20.3835692506745,21.3811406236574,
22.3787119966403,23.3762833696233,24.3738547426062,25.3714261155891,26.3689974885721,
27.366568861555,28.3641402345379,29.3617116075208,30.3592829805038,31.3568543534867,
32.3544257264696,33.3519970994526,34.3495684724355,35.3471398454184,36.3447112184014,
37.3422825913843,38.3398539643672,39.3374253373502,40.3349967103331,41.332568083316,
42.330139456299,43.3277108292819,44.3252822022648,45.3228535752478,46.3204249482307,
47.3179963212136,48.3155676941966,49.3131390671795,50.3107104401624,51.3082818131454,
52.3058531861283,53.3034245591112,54.3009959320942,55.2985673050771,56.29613867806,
57.293710051043,58.2912814240259,59.2888527970088,60.2864241699918,61.2839955429747,
62.2815669159576,63.2791382889406,64.2767096619235,65.2742810349064,66.2718524078894,
67.2694237808723,68.2669951538552,69.2645665268382,70.2621378998211,71.259709272804,
72.2572806457869,73.2548520187699,74.2524233917528,75.2499947647357,76.2475661377187,
77.2451375107016,78.2427088836845,79.2402802566675,80.2378516296504,81.2354230026333,
82.2329943756163,83.2305657485992,84.2281371215821,85.2257084945651,86.223279867548,
87.2208512405309,88.2184226135139,89.2159939864968,90.2135653594797,91.2111367324627,
92.2087081054456,93.2062794784285,94.2038508514115,95.2014222243944,96.1989935973773,
97.1965649703603),.UNSPECIFIED.);
#634=B_SPLINE_SURFACE_WITH_KNOTS('',3,3,((#46252,#46253,#46254,#46255,#46256,
#46257,#46258,#46259,#46260,#46261,#46262,#46263,#46264,#46265,#46266,#46267,
#46268,#46269,#46270,#46271,#46272,#46273,#46274,#46275,#46276,#46277,#46278,
#46279,#46280,#46281,#46282,#46283,#46284,#46285,#46286,#46287,#46288,#46289,
#46290,#46291,#46292,#46293,#46294,#46295,#46296,#46297,#46298,#46299,#46300,
#46301,#46302,#46303,#46304,#46305,#46306,#46307,#46308,#46309,#46310,#46311,
#46312,#46313,#46314,#46315,#46316,#46317,#46318,#46319,#46320,#46321,#46322,
#46323,#46324,#46325,#46326,#46327,#46328,#46329,#46330,#46331,#46332,#46333,
#46334,#46335,#46336,#46337),(#46338,#46339,#46340,#46341,#46342,#46343,
#46344,#46345,#46346,#46347,#46348,#46349,#46350,#46351,#46352,#46353,#46354,
#46355,#46356,#46357,#46358,#46359,#46360,#46361,#46362,#46363,#46364,#46365,
#46366,#46367,#46368,#46369,#46370,#46371,#46372,#46373,#46374,#46375,#46376,
#46377,#46378,#46379,#46380,#46381,#46382,#46383,#46384,#46385,#46386,#46387,
#46388,#46389,#46390,#46391,#46392,#46393,#46394,#46395,#46396,#46397,#46398,
#46399,#46400,#46401,#46402,#46403,#46404,#46405,#46406,#46407,#46408,#46409,
#46410,#46411,#46412,#46413,#46414,#46415,#46416,#46417,#46418,#46419,#46420,
#46421,#46422,#46423),(#46424,#46425,#46426,#46427,#46428,#46429,#46430,
#46431,#46432,#46433,#46434,#46435,#46436,#46437,#46438,#46439,#46440,#46441,
#46442,#46443,#46444,#46445,#46446,#46447,#46448,#46449,#46450,#46451,#46452,
#46453,#46454,#46455,#46456,#46457,#46458,#46459,#46460,#46461,#46462,#46463,
#46464,#46465,#46466,#46467,#46468,#46469,#46470,#46471,#46472,#46473,#46474,
#46475,#46476,#46477,#46478,#46479,#46480,#46481,#46482,#46483,#46484,#46485,
#46486,#46487,#46488,#46489,#46490,#46491,#46492,#46493,#46494,#46495,#46496,
#46497,#46498,#46499,#46500,#46501,#46502,#46503,#46504,#46505,#46506,#46507,
#46508,#46509),(#46510,#46511,#46512,#46513,#46514,#46515,#46516,#46517,
#46518,#46519,#46520,#46521,#46522,#46523,#46524,#46525,#46526,#46527,#46528,
#46529,#46530,#46531,#46532,#46533,#46534,#46535,#46536,#46537,#46538,#46539,
#46540,#46541,#46542,#46543,#46544,#46545,#46546,#46547,#46548,#46549,#46550,
#46551,#46552,#46553,#46554,#46555,#46556,#46557,#46558,#46559,#46560,#46561,
#46562,#46563,#46564,#46565,#46566,#46567,#46568,#46569,#46570,#46571,#46572,
#46573,#46574,#46575,#46576,#46577,#46578,#46579,#46580,#46581,#46582,#46583,
#46584,#46585,#46586,#46587,#46588,#46589,#46590,#46591,#46592,#46593,#46594,
#46595)),.UNSPECIFIED.,.F.,.F.,.F.,(4,4),(4,1,1,1,1,1,1,1,1,1,1,1,1,1,1,
1,1,1,1,1,1,1,1,1,1,1,1,1,1,1,1,1,1,1,1,1,1,1,1,1,1,1,1,1,1,1,1,1,1,1,1,
1,1,1,1,1,1,1,1,1,1,1,1,1,1,1,1,1,1,1,1,1,1,1,1,1,1,1,1,1,1,1,1,4),(0.,
0.0448889834294934),(11.8615800042566,12.8591513772395,13.8567227502225,
14.8542941232054,15.8518654961883,16.8494368691713,17.8470082421542,18.8445796151371,
19.8421509881201,20.839722361103,21.8372937340859,22.8348651070689,23.8324364800518,
24.8300078530347,25.8275792260177,26.8251505990006,27.8227219719835,28.8202933449665,
29.8178647179494,30.8154360909323,31.8130074639152,32.8105788368982,33.8081502098811,
34.805721582864,35.803292955847,36.8008643288299,37.7984357018128,38.7960070747958,
39.7935784477787,40.7911498207616,41.7887211937446,42.7862925667275,43.7838639397104,
44.7814353126934,45.7790066856763,46.7765780586592,47.7741494316422,48.7717208046251,
49.769292177608,50.766863550591,51.7644349235739,52.7620062965568,53.7595776695398,
54.7571490425227,55.7547204155056,56.7522917884886,57.7498631614715,58.7474345344544,
59.7450059074374,60.7425772804203,61.7401486534032,62.7377200263862,63.7352913993691,
64.732862772352,65.730434145335,66.7280055183179,67.7255768913008,68.7231482642838,
69.7207196372667,70.7182910102496,71.7158623832325,72.7134337562155,73.7110051291984,
74.7085765021813,75.7061478751643,76.7037192481472,77.7012906211301,78.6988619941131,
79.696433367096,80.6940047400789,81.6915761130619,82.6891474860448,83.6867188590277,
84.6842902320107,85.6818616049936,86.6794329779765,87.6770043509595,88.6745757239424,
89.6721470969253,90.6697184699083,91.6672898428912,92.6648612158741,93.6624325888571,
94.66000396184),.UNSPECIFIED.);
#635=B_SPLINE_SURFACE_WITH_KNOTS('',3,3,((#46703,#46704,#46705,#46706,#46707,
#46708,#46709,#46710,#46711,#46712,#46713,#46714,#46715,#46716,#46717,#46718,
#46719,#46720,#46721,#46722,#46723,#46724,#46725,#46726,#46727,#46728,#46729,
#46730,#46731,#46732,#46733,#46734,#46735,#46736,#46737,#46738,#46739,#46740,
#46741,#46742,#46743,#46744,#46745,#46746,#46747,#46748,#46749,#46750,#46751,
#46752,#46753,#46754,#46755,#46756,#46757,#46758,#46759,#46760,#46761,#46762,
#46763,#46764,#46765,#46766,#46767,#46768,#46769,#46770,#46771,#46772,#46773,
#46774,#46775,#46776,#46777,#46778,#46779,#46780,#46781,#46782,#46783,#46784,
#46785,#46786,#46787,#46788),(#46789,#46790,#46791,#46792,#46793,#46794,
#46795,#46796,#46797,#46798,#46799,#46800,#46801,#46802,#46803,#46804,#46805,
#46806,#46807,#46808,#46809,#46810,#46811,#46812,#46813,#46814,#46815,#46816,
#46817,#46818,#46819,#46820,#46821,#46822,#46823,#46824,#46825,#46826,#46827,
#46828,#46829,#46830,#46831,#46832,#46833,#46834,#46835,#46836,#46837,#46838,
#46839,#46840,#46841,#46842,#46843,#46844,#46845,#46846,#46847,#46848,#46849,
#46850,#46851,#46852,#46853,#46854,#46855,#46856,#46857,#46858,#46859,#46860,
#46861,#46862,#46863,#46864,#46865,#46866,#46867,#46868,#46869,#46870,#46871,
#46872,#46873,#46874),(#46875,#46876,#46877,#46878,#46879,#46880,#46881,
#46882,#46883,#46884,#46885,#46886,#46887,#46888,#46889,#46890,#46891,#46892,
#46893,#46894,#46895,#46896,#46897,#46898,#46899,#46900,#46901,#46902,#46903,
#46904,#46905,#46906,#46907,#46908,#46909,#46910,#46911,#46912,#46913,#46914,
#46915,#46916,#46917,#46918,#46919,#46920,#46921,#46922,#46923,#46924,#46925,
#46926,#46927,#46928,#46929,#46930,#46931,#46932,#46933,#46934,#46935,#46936,
#46937,#46938,#46939,#46940,#46941,#46942,#46943,#46944,#46945,#46946,#46947,
#46948,#46949,#46950,#46951,#46952,#46953,#46954,#46955,#46956,#46957,#46958,
#46959,#46960),(#46961,#46962,#46963,#46964,#46965,#46966,#46967,#46968,
#46969,#46970,#46971,#46972,#46973,#46974,#46975,#46976,#46977,#46978,#46979,
#46980,#46981,#46982,#46983,#46984,#46985,#46986,#46987,#46988,#46989,#46990,
#46991,#46992,#46993,#46994,#46995,#46996,#46997,#46998,#46999,#47000,#47001,
#47002,#47003,#47004,#47005,#47006,#47007,#47008,#47009,#47010,#47011,#47012,
#47013,#47014,#47015,#47016,#47017,#47018,#47019,#47020,#47021,#47022,#47023,
#47024,#47025,#47026,#47027,#47028,#47029,#47030,#47031,#47032,#47033,#47034,
#47035,#47036,#47037,#47038,#47039,#47040,#47041,#47042,#47043,#47044,#47045,
#47046)),.UNSPECIFIED.,.F.,.F.,.F.,(4,4),(4,1,1,1,1,1,1,1,1,1,1,1,1,1,1,
1,1,1,1,1,1,1,1,1,1,1,1,1,1,1,1,1,1,1,1,1,1,1,1,1,1,1,1,1,1,1,1,1,1,1,1,
1,1,1,1,1,1,1,1,1,1,1,1,1,1,1,1,1,1,1,1,1,1,1,1,1,1,1,1,1,1,1,1,4),(0.,
0.0448889834294934),(14.3981410127769,15.3957123857598,16.3932837587427,
17.3908551317257,18.3884265047086,19.3859978776915,20.3835692506745,21.3811406236574,
22.3787119966403,23.3762833696233,24.3738547426062,25.3714261155891,26.3689974885721,
27.366568861555,28.3641402345379,29.3617116075209,30.3592829805038,31.3568543534867,
32.3544257264696,33.3519970994526,34.3495684724355,35.3471398454184,36.3447112184014,
37.3422825913843,38.3398539643673,39.3374253373502,40.3349967103331,41.332568083316,
42.330139456299,43.3277108292819,44.3252822022648,45.3228535752478,46.3204249482307,
47.3179963212136,48.3155676941966,49.3131390671795,50.3107104401624,51.3082818131454,
52.3058531861283,53.3034245591112,54.3009959320942,55.2985673050771,56.29613867806,
57.293710051043,58.2912814240259,59.2888527970088,60.2864241699918,61.2839955429747,
62.2815669159576,63.2791382889406,64.2767096619235,65.2742810349064,66.2718524078894,
67.2694237808723,68.2669951538552,69.2645665268382,70.2621378998211,71.259709272804,
72.2572806457869,73.2548520187699,74.2524233917528,75.2499947647357,76.2475661377187,
77.2451375107016,78.2427088836845,79.2402802566675,80.2378516296504,81.2354230026333,
82.2329943756163,83.2305657485992,84.2281371215821,85.2257084945651,86.223279867548,
87.2208512405309,88.2184226135139,89.2159939864968,90.2135653594797,91.2111367324627,
92.2087081054456,93.2062794784285,94.2038508514115,95.2014222243944,96.1989935973773,
97.1965649703603),.UNSPECIFIED.);
#636=B_SPLINE_SURFACE_WITH_KNOTS('',3,3,((#47351,#47352,#47353,#47354,#47355,
#47356,#47357,#47358,#47359,#47360,#47361,#47362,#47363,#47364,#47365,#47366,
#47367,#47368,#47369,#47370,#47371,#47372,#47373,#47374,#47375,#47376,#47377,
#47378,#47379,#47380,#47381,#47382,#47383,#47384,#47385,#47386,#47387,#47388,
#47389,#47390,#47391,#47392,#47393,#47394,#47395,#47396,#47397,#47398,#47399,
#47400,#47401,#47402,#47403,#47404,#47405,#47406,#47407,#47408,#47409,#47410,
#47411,#47412,#47413,#47414,#47415,#47416,#47417,#47418,#47419,#47420,#47421,
#47422,#47423,#47424,#47425,#47426,#47427,#47428,#47429,#47430,#47431,#47432,
#47433,#47434,#47435,#47436),(#47437,#47438,#47439,#47440,#47441,#47442,
#47443,#47444,#47445,#47446,#47447,#47448,#47449,#47450,#47451,#47452,#47453,
#47454,#47455,#47456,#47457,#47458,#47459,#47460,#47461,#47462,#47463,#47464,
#47465,#47466,#47467,#47468,#47469,#47470,#47471,#47472,#47473,#47474,#47475,
#47476,#47477,#47478,#47479,#47480,#47481,#47482,#47483,#47484,#47485,#47486,
#47487,#47488,#47489,#47490,#47491,#47492,#47493,#47494,#47495,#47496,#47497,
#47498,#47499,#47500,#47501,#47502,#47503,#47504,#47505,#47506,#47507,#47508,
#47509,#47510,#47511,#47512,#47513,#47514,#47515,#47516,#47517,#47518,#47519,
#47520,#47521,#47522),(#47523,#47524,#47525,#47526,#47527,#47528,#47529,
#47530,#47531,#47532,#47533,#47534,#47535,#47536,#47537,#47538,#47539,#47540,
#47541,#47542,#47543,#47544,#47545,#47546,#47547,#47548,#47549,#47550,#47551,
#47552,#47553,#47554,#47555,#47556,#47557,#47558,#47559,#47560,#47561,#47562,
#47563,#47564,#47565,#47566,#47567,#47568,#47569,#47570,#47571,#47572,#47573,
#47574,#47575,#47576,#47577,#47578,#47579,#47580,#47581,#47582,#47583,#47584,
#47585,#47586,#47587,#47588,#47589,#47590,#47591,#47592,#47593,#47594,#47595,
#47596,#47597,#47598,#47599,#47600,#47601,#47602,#47603,#47604,#47605,#47606,
#47607,#47608),(#47609,#47610,#47611,#47612,#47613,#47614,#47615,#47616,
#47617,#47618,#47619,#47620,#47621,#47622,#47623,#47624,#47625,#47626,#47627,
#47628,#47629,#47630,#47631,#47632,#47633,#47634,#47635,#47636,#47637,#47638,
#47639,#47640,#47641,#47642,#47643,#47644,#47645,#47646,#47647,#47648,#47649,
#47650,#47651,#47652,#47653,#47654,#47655,#47656,#47657,#47658,#47659,#47660,
#47661,#47662,#47663,#47664,#47665,#47666,#47667,#47668,#47669,#47670,#47671,
#47672,#47673,#47674,#47675,#47676,#47677,#47678,#47679,#47680,#47681,#47682,
#47683,#47684,#47685,#47686,#47687,#47688,#47689,#47690,#47691,#47692,#47693,
#47694)),.UNSPECIFIED.,.F.,.F.,.F.,(4,4),(4,1,1,1,1,1,1,1,1,1,1,1,1,1,1,
1,1,1,1,1,1,1,1,1,1,1,1,1,1,1,1,1,1,1,1,1,1,1,1,1,1,1,1,1,1,1,1,1,1,1,1,
1,1,1,1,1,1,1,1,1,1,1,1,1,1,1,1,1,1,1,1,1,1,1,1,1,1,1,1,1,1,1,1,4),(0.,
0.0448889834294935),(11.8615800042566,12.8591513772396,13.8567227502225,
14.8542941232054,15.8518654961884,16.8494368691713,17.8470082421542,18.8445796151372,
19.8421509881201,20.839722361103,21.837293734086,22.8348651070689,23.8324364800518,
24.8300078530348,25.8275792260177,26.8251505990006,27.8227219719836,28.8202933449665,
29.8178647179494,30.8154360909324,31.8130074639153,32.8105788368982,33.8081502098811,
34.8057215828641,35.803292955847,36.80086432883,37.7984357018129,38.7960070747958,
39.7935784477787,40.7911498207617,41.7887211937446,42.7862925667275,43.7838639397105,
44.7814353126934,45.7790066856763,46.7765780586593,47.7741494316422,48.7717208046251,
49.7692921776081,50.766863550591,51.7644349235739,52.7620062965569,53.7595776695398,
54.7571490425227,55.7547204155057,56.7522917884886,57.7498631614715,58.7474345344545,
59.7450059074374,60.7425772804203,61.7401486534033,62.7377200263862,63.7352913993691,
64.7328627723521,65.730434145335,66.7280055183179,67.7255768913009,68.7231482642838,
69.7207196372667,70.7182910102497,71.7158623832326,72.7134337562155,73.7110051291985,
74.7085765021814,75.7061478751643,76.7037192481473,77.7012906211302,78.6988619941131,
79.696433367096,80.694004740079,81.6915761130619,82.6891474860448,83.6867188590278,
84.6842902320107,85.6818616049936,86.6794329779766,87.6770043509595,88.6745757239424,
89.6721470969254,90.6697184699083,91.6672898428912,92.6648612158742,93.6624325888571,
94.66000396184),.UNSPECIFIED.);
#637=B_SPLINE_SURFACE_WITH_KNOTS('',3,3,((#47802,#47803,#47804,#47805,#47806,
#47807,#47808,#47809,#47810,#47811,#47812,#47813,#47814,#47815,#47816,#47817,
#47818,#47819,#47820,#47821,#47822,#47823,#47824,#47825,#47826,#47827,#47828,
#47829,#47830,#47831,#47832,#47833,#47834,#47835,#47836,#47837,#47838,#47839,
#47840,#47841,#47842,#47843,#47844,#47845,#47846,#47847,#47848,#47849,#47850,
#47851,#47852,#47853,#47854,#47855,#47856,#47857,#47858,#47859,#47860,#47861,
#47862,#47863,#47864,#47865,#47866,#47867,#47868,#47869,#47870,#47871,#47872,
#47873,#47874,#47875,#47876,#47877,#47878,#47879,#47880,#47881,#47882,#47883,
#47884,#47885,#47886,#47887),(#47888,#47889,#47890,#47891,#47892,#47893,
#47894,#47895,#47896,#47897,#47898,#47899,#47900,#47901,#47902,#47903,#47904,
#47905,#47906,#47907,#47908,#47909,#47910,#47911,#47912,#47913,#47914,#47915,
#47916,#47917,#47918,#47919,#47920,#47921,#47922,#47923,#47924,#47925,#47926,
#47927,#47928,#47929,#47930,#47931,#47932,#47933,#47934,#47935,#47936,#47937,
#47938,#47939,#47940,#47941,#47942,#47943,#47944,#47945,#47946,#47947,#47948,
#47949,#47950,#47951,#47952,#47953,#47954,#47955,#47956,#47957,#47958,#47959,
#47960,#47961,#47962,#47963,#47964,#47965,#47966,#47967,#47968,#47969,#47970,
#47971,#47972,#47973),(#47974,#47975,#47976,#47977,#47978,#47979,#47980,
#47981,#47982,#47983,#47984,#47985,#47986,#47987,#47988,#47989,#47990,#47991,
#47992,#47993,#47994,#47995,#47996,#47997,#47998,#47999,#48000,#48001,#48002,
#48003,#48004,#48005,#48006,#48007,#48008,#48009,#48010,#48011,#48012,#48013,
#48014,#48015,#48016,#48017,#48018,#48019,#48020,#48021,#48022,#48023,#48024,
#48025,#48026,#48027,#48028,#48029,#48030,#48031,#48032,#48033,#48034,#48035,
#48036,#48037,#48038,#48039,#48040,#48041,#48042,#48043,#48044,#48045,#48046,
#48047,#48048,#48049,#48050,#48051,#48052,#48053,#48054,#48055,#48056,#48057,
#48058,#48059),(#48060,#48061,#48062,#48063,#48064,#48065,#48066,#48067,
#48068,#48069,#48070,#48071,#48072,#48073,#48074,#48075,#48076,#48077,#48078,
#48079,#48080,#48081,#48082,#48083,#48084,#48085,#48086,#48087,#48088,#48089,
#48090,#48091,#48092,#48093,#48094,#48095,#48096,#48097,#48098,#48099,#48100,
#48101,#48102,#48103,#48104,#48105,#48106,#48107,#48108,#48109,#48110,#48111,
#48112,#48113,#48114,#48115,#48116,#48117,#48118,#48119,#48120,#48121,#48122,
#48123,#48124,#48125,#48126,#48127,#48128,#48129,#48130,#48131,#48132,#48133,
#48134,#48135,#48136,#48137,#48138,#48139,#48140,#48141,#48142,#48143,#48144,
#48145)),.UNSPECIFIED.,.F.,.F.,.F.,(4,4),(4,1,1,1,1,1,1,1,1,1,1,1,1,1,1,
1,1,1,1,1,1,1,1,1,1,1,1,1,1,1,1,1,1,1,1,1,1,1,1,1,1,1,1,1,1,1,1,1,1,1,1,
1,1,1,1,1,1,1,1,1,1,1,1,1,1,1,1,1,1,1,1,1,1,1,1,1,1,1,1,1,1,1,1,4),(0.,
0.0448889834294935),(14.3981410127769,15.3957123857598,16.3932837587428,
17.3908551317257,18.3884265047086,19.3859978776916,20.3835692506745,21.3811406236574,
22.3787119966404,23.3762833696233,24.3738547426062,25.3714261155892,26.3689974885721,
27.366568861555,28.364140234538,29.3617116075209,30.3592829805038,31.3568543534868,
32.3544257264697,33.3519970994526,34.3495684724355,35.3471398454185,36.3447112184014,
37.3422825913843,38.3398539643673,39.3374253373502,40.3349967103332,41.3325680833161,
42.330139456299,43.3277108292819,44.3252822022649,45.3228535752478,46.3204249482307,
47.3179963212137,48.3155676941966,49.3131390671795,50.3107104401625,51.3082818131454,
52.3058531861283,53.3034245591113,54.3009959320942,55.2985673050771,56.2961386780601,
57.293710051043,58.2912814240259,59.2888527970089,60.2864241699918,61.2839955429747,
62.2815669159577,63.2791382889406,64.2767096619235,65.2742810349065,66.2718524078894,
67.2694237808723,68.2669951538553,69.2645665268382,70.2621378998211,71.2597092728041,
72.257280645787,73.2548520187699,74.2524233917529,75.2499947647358,76.2475661377187,
77.2451375107017,78.2427088836846,79.2402802566675,80.2378516296505,81.2354230026334,
82.2329943756163,83.2305657485992,84.2281371215822,85.2257084945651,86.223279867548,
87.220851240531,88.2184226135139,89.2159939864968,90.2135653594798,91.2111367324627,
92.2087081054456,93.2062794784286,94.2038508514115,95.2014222243944,96.1989935973774,
97.1965649703603),.UNSPECIFIED.);
#638=B_SPLINE_SURFACE_WITH_KNOTS('',3,3,((#48450,#48451,#48452,#48453,#48454,
#48455,#48456,#48457,#48458,#48459,#48460,#48461,#48462,#48463,#48464,#48465,
#48466,#48467,#48468,#48469,#48470,#48471,#48472,#48473,#48474,#48475,#48476,
#48477,#48478,#48479,#48480,#48481,#48482,#48483,#48484,#48485,#48486,#48487,
#48488,#48489,#48490,#48491,#48492,#48493,#48494,#48495,#48496,#48497,#48498,
#48499,#48500,#48501,#48502,#48503,#48504,#48505,#48506,#48507,#48508,#48509,
#48510,#48511,#48512,#48513,#48514,#48515,#48516,#48517,#48518,#48519,#48520,
#48521,#48522,#48523,#48524,#48525,#48526,#48527,#48528,#48529,#48530,#48531,
#48532,#48533,#48534,#48535),(#48536,#48537,#48538,#48539,#48540,#48541,
#48542,#48543,#48544,#48545,#48546,#48547,#48548,#48549,#48550,#48551,#48552,
#48553,#48554,#48555,#48556,#48557,#48558,#48559,#48560,#48561,#48562,#48563,
#48564,#48565,#48566,#48567,#48568,#48569,#48570,#48571,#48572,#48573,#48574,
#48575,#48576,#48577,#48578,#48579,#48580,#48581,#48582,#48583,#48584,#48585,
#48586,#48587,#48588,#48589,#48590,#48591,#48592,#48593,#48594,#48595,#48596,
#48597,#48598,#48599,#48600,#48601,#48602,#48603,#48604,#48605,#48606,#48607,
#48608,#48609,#48610,#48611,#48612,#48613,#48614,#48615,#48616,#48617,#48618,
#48619,#48620,#48621),(#48622,#48623,#48624,#48625,#48626,#48627,#48628,
#48629,#48630,#48631,#48632,#48633,#48634,#48635,#48636,#48637,#48638,#48639,
#48640,#48641,#48642,#48643,#48644,#48645,#48646,#48647,#48648,#48649,#48650,
#48651,#48652,#48653,#48654,#48655,#48656,#48657,#48658,#48659,#48660,#48661,
#48662,#48663,#48664,#48665,#48666,#48667,#48668,#48669,#48670,#48671,#48672,
#48673,#48674,#48675,#48676,#48677,#48678,#48679,#48680,#48681,#48682,#48683,
#48684,#48685,#48686,#48687,#48688,#48689,#48690,#48691,#48692,#48693,#48694,
#48695,#48696,#48697,#48698,#48699,#48700,#48701,#48702,#48703,#48704,#48705,
#48706,#48707),(#48708,#48709,#48710,#48711,#48712,#48713,#48714,#48715,
#48716,#48717,#48718,#48719,#48720,#48721,#48722,#48723,#48724,#48725,#48726,
#48727,#48728,#48729,#48730,#48731,#48732,#48733,#48734,#48735,#48736,#48737,
#48738,#48739,#48740,#48741,#48742,#48743,#48744,#48745,#48746,#48747,#48748,
#48749,#48750,#48751,#48752,#48753,#48754,#48755,#48756,#48757,#48758,#48759,
#48760,#48761,#48762,#48763,#48764,#48765,#48766,#48767,#48768,#48769,#48770,
#48771,#48772,#48773,#48774,#48775,#48776,#48777,#48778,#48779,#48780,#48781,
#48782,#48783,#48784,#48785,#48786,#48787,#48788,#48789,#48790,#48791,#48792,
#48793)),.UNSPECIFIED.,.F.,.F.,.F.,(4,4),(4,1,1,1,1,1,1,1,1,1,1,1,1,1,1,
1,1,1,1,1,1,1,1,1,1,1,1,1,1,1,1,1,1,1,1,1,1,1,1,1,1,1,1,1,1,1,1,1,1,1,1,
1,1,1,1,1,1,1,1,1,1,1,1,1,1,1,1,1,1,1,1,1,1,1,1,1,1,1,1,1,1,1,1,4),(0.,
0.0448889834294934),(11.8615800042566,12.8591513772395,13.8567227502225,
14.8542941232054,15.8518654961883,16.8494368691713,17.8470082421542,18.8445796151371,
19.8421509881201,20.839722361103,21.8372937340859,22.8348651070689,23.8324364800518,
24.8300078530347,25.8275792260177,26.8251505990006,27.8227219719835,28.8202933449664,
29.8178647179494,30.8154360909323,31.8130074639152,32.8105788368982,33.8081502098811,
34.805721582864,35.803292955847,36.8008643288299,37.7984357018128,38.7960070747958,
39.7935784477787,40.7911498207616,41.7887211937446,42.7862925667275,43.7838639397104,
44.7814353126934,45.7790066856763,46.7765780586592,47.7741494316422,48.7717208046251,
49.769292177608,50.766863550591,51.7644349235739,52.7620062965568,53.7595776695398,
54.7571490425227,55.7547204155056,56.7522917884886,57.7498631614715,58.7474345344544,
59.7450059074374,60.7425772804203,61.7401486534032,62.7377200263862,63.7352913993691,
64.732862772352,65.730434145335,66.7280055183179,67.7255768913008,68.7231482642838,
69.7207196372667,70.7182910102496,71.7158623832325,72.7134337562155,73.7110051291984,
74.7085765021813,75.7061478751643,76.7037192481472,77.7012906211301,78.6988619941131,
79.696433367096,80.6940047400789,81.6915761130619,82.6891474860448,83.6867188590277,
84.6842902320107,85.6818616049936,86.6794329779765,87.6770043509595,88.6745757239424,
89.6721470969253,90.6697184699083,91.6672898428912,92.6648612158741,93.6624325888571,
94.66000396184),.UNSPECIFIED.);
#639=B_SPLINE_SURFACE_WITH_KNOTS('',3,3,((#48901,#48902,#48903,#48904,#48905,
#48906,#48907,#48908,#48909,#48910,#48911,#48912,#48913,#48914,#48915,#48916,
#48917,#48918,#48919,#48920,#48921,#48922,#48923,#48924,#48925,#48926,#48927,
#48928,#48929,#48930,#48931,#48932,#48933,#48934,#48935,#48936,#48937,#48938,
#48939,#48940,#48941,#48942,#48943,#48944,#48945,#48946,#48947,#48948,#48949,
#48950,#48951,#48952,#48953,#48954,#48955,#48956,#48957,#48958,#48959,#48960,
#48961,#48962,#48963,#48964,#48965,#48966,#48967,#48968,#48969,#48970,#48971,
#48972,#48973,#48974,#48975,#48976,#48977,#48978,#48979,#48980,#48981,#48982,
#48983,#48984,#48985,#48986),(#48987,#48988,#48989,#48990,#48991,#48992,
#48993,#48994,#48995,#48996,#48997,#48998,#48999,#49000,#49001,#49002,#49003,
#49004,#49005,#49006,#49007,#49008,#49009,#49010,#49011,#49012,#49013,#49014,
#49015,#49016,#49017,#49018,#49019,#49020,#49021,#49022,#49023,#49024,#49025,
#49026,#49027,#49028,#49029,#49030,#49031,#49032,#49033,#49034,#49035,#49036,
#49037,#49038,#49039,#49040,#49041,#49042,#49043,#49044,#49045,#49046,#49047,
#49048,#49049,#49050,#49051,#49052,#49053,#49054,#49055,#49056,#49057,#49058,
#49059,#49060,#49061,#49062,#49063,#49064,#49065,#49066,#49067,#49068,#49069,
#49070,#49071,#49072),(#49073,#49074,#49075,#49076,#49077,#49078,#49079,
#49080,#49081,#49082,#49083,#49084,#49085,#49086,#49087,#49088,#49089,#49090,
#49091,#49092,#49093,#49094,#49095,#49096,#49097,#49098,#49099,#49100,#49101,
#49102,#49103,#49104,#49105,#49106,#49107,#49108,#49109,#49110,#49111,#49112,
#49113,#49114,#49115,#49116,#49117,#49118,#49119,#49120,#49121,#49122,#49123,
#49124,#49125,#49126,#49127,#49128,#49129,#49130,#49131,#49132,#49133,#49134,
#49135,#49136,#49137,#49138,#49139,#49140,#49141,#49142,#49143,#49144,#49145,
#49146,#49147,#49148,#49149,#49150,#49151,#49152,#49153,#49154,#49155,#49156,
#49157,#49158),(#49159,#49160,#49161,#49162,#49163,#49164,#49165,#49166,
#49167,#49168,#49169,#49170,#49171,#49172,#49173,#49174,#49175,#49176,#49177,
#49178,#49179,#49180,#49181,#49182,#49183,#49184,#49185,#49186,#49187,#49188,
#49189,#49190,#49191,#49192,#49193,#49194,#49195,#49196,#49197,#49198,#49199,
#49200,#49201,#49202,#49203,#49204,#49205,#49206,#49207,#49208,#49209,#49210,
#49211,#49212,#49213,#49214,#49215,#49216,#49217,#49218,#49219,#49220,#49221,
#49222,#49223,#49224,#49225,#49226,#49227,#49228,#49229,#49230,#49231,#49232,
#49233,#49234,#49235,#49236,#49237,#49238,#49239,#49240,#49241,#49242,#49243,
#49244)),.UNSPECIFIED.,.F.,.F.,.F.,(4,4),(4,1,1,1,1,1,1,1,1,1,1,1,1,1,1,
1,1,1,1,1,1,1,1,1,1,1,1,1,1,1,1,1,1,1,1,1,1,1,1,1,1,1,1,1,1,1,1,1,1,1,1,
1,1,1,1,1,1,1,1,1,1,1,1,1,1,1,1,1,1,1,1,1,1,1,1,1,1,1,1,1,1,1,1,4),(0.,
0.0448889834294934),(14.3981410127769,15.3957123857598,16.3932837587427,
17.3908551317257,18.3884265047086,19.3859978776915,20.3835692506745,21.3811406236574,
22.3787119966403,23.3762833696233,24.3738547426062,25.3714261155891,26.3689974885721,
27.366568861555,28.3641402345379,29.3617116075209,30.3592829805038,31.3568543534867,
32.3544257264696,33.3519970994526,34.3495684724355,35.3471398454184,36.3447112184014,
37.3422825913843,38.3398539643673,39.3374253373502,40.3349967103331,41.332568083316,
42.330139456299,43.3277108292819,44.3252822022648,45.3228535752478,46.3204249482307,
47.3179963212136,48.3155676941966,49.3131390671795,50.3107104401624,51.3082818131454,
52.3058531861283,53.3034245591112,54.3009959320942,55.2985673050771,56.29613867806,
57.293710051043,58.2912814240259,59.2888527970088,60.2864241699918,61.2839955429747,
62.2815669159576,63.2791382889406,64.2767096619235,65.2742810349064,66.2718524078894,
67.2694237808723,68.2669951538552,69.2645665268382,70.2621378998211,71.259709272804,
72.2572806457869,73.2548520187699,74.2524233917528,75.2499947647357,76.2475661377187,
77.2451375107016,78.2427088836845,79.2402802566675,80.2378516296504,81.2354230026333,
82.2329943756163,83.2305657485992,84.2281371215821,85.2257084945651,86.223279867548,
87.2208512405309,88.2184226135139,89.2159939864968,90.2135653594797,91.2111367324627,
92.2087081054456,93.2062794784285,94.2038508514115,95.2014222243944,96.1989935973773,
97.1965649703603),.UNSPECIFIED.);
#640=B_SPLINE_SURFACE_WITH_KNOTS('',3,3,((#49549,#49550,#49551,#49552,#49553,
#49554,#49555,#49556,#49557,#49558,#49559,#49560,#49561,#49562,#49563,#49564,
#49565,#49566,#49567,#49568,#49569,#49570,#49571,#49572,#49573,#49574,#49575,
#49576,#49577,#49578,#49579,#49580,#49581,#49582,#49583,#49584,#49585,#49586,
#49587,#49588,#49589,#49590,#49591,#49592,#49593,#49594,#49595,#49596,#49597,
#49598,#49599,#49600,#49601,#49602,#49603,#49604,#49605,#49606,#49607,#49608,
#49609,#49610,#49611,#49612,#49613,#49614,#49615,#49616,#49617,#49618,#49619,
#49620,#49621,#49622,#49623,#49624,#49625,#49626,#49627,#49628,#49629,#49630,
#49631,#49632,#49633,#49634),(#49635,#49636,#49637,#49638,#49639,#49640,
#49641,#49642,#49643,#49644,#49645,#49646,#49647,#49648,#49649,#49650,#49651,
#49652,#49653,#49654,#49655,#49656,#49657,#49658,#49659,#49660,#49661,#49662,
#49663,#49664,#49665,#49666,#49667,#49668,#49669,#49670,#49671,#49672,#49673,
#49674,#49675,#49676,#49677,#49678,#49679,#49680,#49681,#49682,#49683,#49684,
#49685,#49686,#49687,#49688,#49689,#49690,#49691,#49692,#49693,#49694,#49695,
#49696,#49697,#49698,#49699,#49700,#49701,#49702,#49703,#49704,#49705,#49706,
#49707,#49708,#49709,#49710,#49711,#49712,#49713,#49714,#49715,#49716,#49717,
#49718,#49719,#49720),(#49721,#49722,#49723,#49724,#49725,#49726,#49727,
#49728,#49729,#49730,#49731,#49732,#49733,#49734,#49735,#49736,#49737,#49738,
#49739,#49740,#49741,#49742,#49743,#49744,#49745,#49746,#49747,#49748,#49749,
#49750,#49751,#49752,#49753,#49754,#49755,#49756,#49757,#49758,#49759,#49760,
#49761,#49762,#49763,#49764,#49765,#49766,#49767,#49768,#49769,#49770,#49771,
#49772,#49773,#49774,#49775,#49776,#49777,#49778,#49779,#49780,#49781,#49782,
#49783,#49784,#49785,#49786,#49787,#49788,#49789,#49790,#49791,#49792,#49793,
#49794,#49795,#49796,#49797,#49798,#49799,#49800,#49801,#49802,#49803,#49804,
#49805,#49806),(#49807,#49808,#49809,#49810,#49811,#49812,#49813,#49814,
#49815,#49816,#49817,#49818,#49819,#49820,#49821,#49822,#49823,#49824,#49825,
#49826,#49827,#49828,#49829,#49830,#49831,#49832,#49833,#49834,#49835,#49836,
#49837,#49838,#49839,#49840,#49841,#49842,#49843,#49844,#49845,#49846,#49847,
#49848,#49849,#49850,#49851,#49852,#49853,#49854,#49855,#49856,#49857,#49858,
#49859,#49860,#49861,#49862,#49863,#49864,#49865,#49866,#49867,#49868,#49869,
#49870,#49871,#49872,#49873,#49874,#49875,#49876,#49877,#49878,#49879,#49880,
#49881,#49882,#49883,#49884,#49885,#49886,#49887,#49888,#49889,#49890,#49891,
#49892)),.UNSPECIFIED.,.F.,.F.,.F.,(4,4),(4,1,1,1,1,1,1,1,1,1,1,1,1,1,1,
1,1,1,1,1,1,1,1,1,1,1,1,1,1,1,1,1,1,1,1,1,1,1,1,1,1,1,1,1,1,1,1,1,1,1,1,
1,1,1,1,1,1,1,1,1,1,1,1,1,1,1,1,1,1,1,1,1,1,1,1,1,1,1,1,1,1,1,1,4),(0.,
0.0448889834294934),(11.8615800042566,12.8591513772395,13.8567227502225,
14.8542941232054,15.8518654961883,16.8494368691713,17.8470082421542,18.8445796151371,
19.8421509881201,20.839722361103,21.8372937340859,22.8348651070689,23.8324364800518,
24.8300078530347,25.8275792260177,26.8251505990006,27.8227219719835,28.8202933449665,
29.8178647179494,30.8154360909323,31.8130074639152,32.8105788368982,33.8081502098811,
34.805721582864,35.803292955847,36.8008643288299,37.7984357018128,38.7960070747958,
39.7935784477787,40.7911498207616,41.7887211937446,42.7862925667275,43.7838639397104,
44.7814353126934,45.7790066856763,46.7765780586592,47.7741494316422,48.7717208046251,
49.769292177608,50.766863550591,51.7644349235739,52.7620062965568,53.7595776695398,
54.7571490425227,55.7547204155056,56.7522917884886,57.7498631614715,58.7474345344544,
59.7450059074374,60.7425772804203,61.7401486534032,62.7377200263862,63.7352913993691,
64.732862772352,65.730434145335,66.7280055183179,67.7255768913008,68.7231482642838,
69.7207196372667,70.7182910102496,71.7158623832325,72.7134337562155,73.7110051291984,
74.7085765021813,75.7061478751643,76.7037192481472,77.7012906211301,78.6988619941131,
79.696433367096,80.6940047400789,81.6915761130619,82.6891474860448,83.6867188590277,
84.6842902320107,85.6818616049936,86.6794329779765,87.6770043509595,88.6745757239424,
89.6721470969253,90.6697184699083,91.6672898428912,92.6648612158741,93.6624325888571,
94.66000396184),.UNSPECIFIED.);
#641=B_SPLINE_SURFACE_WITH_KNOTS('',3,3,((#50000,#50001,#50002,#50003,#50004,
#50005,#50006,#50007,#50008,#50009,#50010,#50011,#50012,#50013,#50014,#50015,
#50016,#50017,#50018,#50019,#50020,#50021,#50022,#50023,#50024,#50025,#50026,
#50027,#50028,#50029,#50030,#50031,#50032,#50033,#50034,#50035,#50036,#50037,
#50038,#50039,#50040,#50041,#50042,#50043,#50044,#50045,#50046,#50047,#50048,
#50049,#50050,#50051,#50052,#50053,#50054,#50055,#50056,#50057,#50058,#50059,
#50060,#50061,#50062,#50063,#50064,#50065,#50066,#50067,#50068,#50069,#50070,
#50071,#50072,#50073,#50074,#50075,#50076,#50077,#50078,#50079,#50080,#50081,
#50082,#50083,#50084,#50085),(#50086,#50087,#50088,#50089,#50090,#50091,
#50092,#50093,#50094,#50095,#50096,#50097,#50098,#50099,#50100,#50101,#50102,
#50103,#50104,#50105,#50106,#50107,#50108,#50109,#50110,#50111,#50112,#50113,
#50114,#50115,#50116,#50117,#50118,#50119,#50120,#50121,#50122,#50123,#50124,
#50125,#50126,#50127,#50128,#50129,#50130,#50131,#50132,#50133,#50134,#50135,
#50136,#50137,#50138,#50139,#50140,#50141,#50142,#50143,#50144,#50145,#50146,
#50147,#50148,#50149,#50150,#50151,#50152,#50153,#50154,#50155,#50156,#50157,
#50158,#50159,#50160,#50161,#50162,#50163,#50164,#50165,#50166,#50167,#50168,
#50169,#50170,#50171),(#50172,#50173,#50174,#50175,#50176,#50177,#50178,
#50179,#50180,#50181,#50182,#50183,#50184,#50185,#50186,#50187,#50188,#50189,
#50190,#50191,#50192,#50193,#50194,#50195,#50196,#50197,#50198,#50199,#50200,
#50201,#50202,#50203,#50204,#50205,#50206,#50207,#50208,#50209,#50210,#50211,
#50212,#50213,#50214,#50215,#50216,#50217,#50218,#50219,#50220,#50221,#50222,
#50223,#50224,#50225,#50226,#50227,#50228,#50229,#50230,#50231,#50232,#50233,
#50234,#50235,#50236,#50237,#50238,#50239,#50240,#50241,#50242,#50243,#50244,
#50245,#50246,#50247,#50248,#50249,#50250,#50251,#50252,#50253,#50254,#50255,
#50256,#50257),(#50258,#50259,#50260,#50261,#50262,#50263,#50264,#50265,
#50266,#50267,#50268,#50269,#50270,#50271,#50272,#50273,#50274,#50275,#50276,
#50277,#50278,#50279,#50280,#50281,#50282,#50283,#50284,#50285,#50286,#50287,
#50288,#50289,#50290,#50291,#50292,#50293,#50294,#50295,#50296,#50297,#50298,
#50299,#50300,#50301,#50302,#50303,#50304,#50305,#50306,#50307,#50308,#50309,
#50310,#50311,#50312,#50313,#50314,#50315,#50316,#50317,#50318,#50319,#50320,
#50321,#50322,#50323,#50324,#50325,#50326,#50327,#50328,#50329,#50330,#50331,
#50332,#50333,#50334,#50335,#50336,#50337,#50338,#50339,#50340,#50341,#50342,
#50343)),.UNSPECIFIED.,.F.,.F.,.F.,(4,4),(4,1,1,1,1,1,1,1,1,1,1,1,1,1,1,
1,1,1,1,1,1,1,1,1,1,1,1,1,1,1,1,1,1,1,1,1,1,1,1,1,1,1,1,1,1,1,1,1,1,1,1,
1,1,1,1,1,1,1,1,1,1,1,1,1,1,1,1,1,1,1,1,1,1,1,1,1,1,1,1,1,1,1,1,4),(0.,
0.0448889834294934),(14.3981410127769,15.3957123857598,16.3932837587427,
17.3908551317257,18.3884265047086,19.3859978776915,20.3835692506745,21.3811406236574,
22.3787119966403,23.3762833696233,24.3738547426062,25.3714261155891,26.3689974885721,
27.366568861555,28.3641402345379,29.3617116075209,30.3592829805038,31.3568543534867,
32.3544257264696,33.3519970994526,34.3495684724355,35.3471398454184,36.3447112184014,
37.3422825913843,38.3398539643672,39.3374253373502,40.3349967103331,41.332568083316,
42.330139456299,43.3277108292819,44.3252822022648,45.3228535752478,46.3204249482307,
47.3179963212136,48.3155676941966,49.3131390671795,50.3107104401624,51.3082818131454,
52.3058531861283,53.3034245591112,54.3009959320942,55.2985673050771,56.29613867806,
57.293710051043,58.2912814240259,59.2888527970088,60.2864241699918,61.2839955429747,
62.2815669159576,63.2791382889406,64.2767096619235,65.2742810349064,66.2718524078894,
67.2694237808723,68.2669951538552,69.2645665268382,70.2621378998211,71.259709272804,
72.2572806457869,73.2548520187699,74.2524233917528,75.2499947647357,76.2475661377187,
77.2451375107016,78.2427088836845,79.2402802566675,80.2378516296504,81.2354230026333,
82.2329943756163,83.2305657485992,84.2281371215821,85.2257084945651,86.223279867548,
87.2208512405309,88.2184226135139,89.2159939864968,90.2135653594797,91.2111367324627,
92.2087081054456,93.2062794784285,94.2038508514115,95.2014222243944,96.1989935973773,
97.1965649703603),.UNSPECIFIED.);
#642=B_SPLINE_SURFACE_WITH_KNOTS('',3,3,((#50653,#50654,#50655,#50656,#50657,
#50658,#50659,#50660,#50661,#50662,#50663,#50664,#50665,#50666,#50667,#50668,
#50669,#50670,#50671,#50672,#50673,#50674,#50675,#50676,#50677,#50678,#50679,
#50680,#50681,#50682,#50683,#50684,#50685,#50686,#50687,#50688,#50689,#50690,
#50691,#50692,#50693,#50694,#50695,#50696,#50697,#50698,#50699,#50700,#50701,
#50702,#50703,#50704,#50705,#50706,#50707,#50708,#50709,#50710,#50711,#50712,
#50713,#50714,#50715,#50716,#50717,#50718,#50719,#50720,#50721,#50722,#50723,
#50724,#50725,#50726,#50727,#50728,#50729,#50730,#50731,#50732,#50733,#50734,
#50735,#50736,#50737,#50738),(#50739,#50740,#50741,#50742,#50743,#50744,
#50745,#50746,#50747,#50748,#50749,#50750,#50751,#50752,#50753,#50754,#50755,
#50756,#50757,#50758,#50759,#50760,#50761,#50762,#50763,#50764,#50765,#50766,
#50767,#50768,#50769,#50770,#50771,#50772,#50773,#50774,#50775,#50776,#50777,
#50778,#50779,#50780,#50781,#50782,#50783,#50784,#50785,#50786,#50787,#50788,
#50789,#50790,#50791,#50792,#50793,#50794,#50795,#50796,#50797,#50798,#50799,
#50800,#50801,#50802,#50803,#50804,#50805,#50806,#50807,#50808,#50809,#50810,
#50811,#50812,#50813,#50814,#50815,#50816,#50817,#50818,#50819,#50820,#50821,
#50822,#50823,#50824),(#50825,#50826,#50827,#50828,#50829,#50830,#50831,
#50832,#50833,#50834,#50835,#50836,#50837,#50838,#50839,#50840,#50841,#50842,
#50843,#50844,#50845,#50846,#50847,#50848,#50849,#50850,#50851,#50852,#50853,
#50854,#50855,#50856,#50857,#50858,#50859,#50860,#50861,#50862,#50863,#50864,
#50865,#50866,#50867,#50868,#50869,#50870,#50871,#50872,#50873,#50874,#50875,
#50876,#50877,#50878,#50879,#50880,#50881,#50882,#50883,#50884,#50885,#50886,
#50887,#50888,#50889,#50890,#50891,#50892,#50893,#50894,#50895,#50896,#50897,
#50898,#50899,#50900,#50901,#50902,#50903,#50904,#50905,#50906,#50907,#50908,
#50909,#50910),(#50911,#50912,#50913,#50914,#50915,#50916,#50917,#50918,
#50919,#50920,#50921,#50922,#50923,#50924,#50925,#50926,#50927,#50928,#50929,
#50930,#50931,#50932,#50933,#50934,#50935,#50936,#50937,#50938,#50939,#50940,
#50941,#50942,#50943,#50944,#50945,#50946,#50947,#50948,#50949,#50950,#50951,
#50952,#50953,#50954,#50955,#50956,#50957,#50958,#50959,#50960,#50961,#50962,
#50963,#50964,#50965,#50966,#50967,#50968,#50969,#50970,#50971,#50972,#50973,
#50974,#50975,#50976,#50977,#50978,#50979,#50980,#50981,#50982,#50983,#50984,
#50985,#50986,#50987,#50988,#50989,#50990,#50991,#50992,#50993,#50994,#50995,
#50996)),.UNSPECIFIED.,.F.,.F.,.F.,(4,4),(4,1,1,1,1,1,1,1,1,1,1,1,1,1,1,
1,1,1,1,1,1,1,1,1,1,1,1,1,1,1,1,1,1,1,1,1,1,1,1,1,1,1,1,1,1,1,1,1,1,1,1,
1,1,1,1,1,1,1,1,1,1,1,1,1,1,1,1,1,1,1,1,1,1,1,1,1,1,1,1,1,1,1,1,4),(0.,
0.0448889834294934),(11.8615800042567,12.8591513772396,13.8567227502225,
14.8542941232055,15.8518654961884,16.8494368691713,17.8470082421543,18.8445796151372,
19.8421509881201,20.8397223611031,21.837293734086,22.8348651070689,23.8324364800519,
24.8300078530348,25.8275792260177,26.8251505990007,27.8227219719836,28.8202933449665,
29.8178647179495,30.8154360909324,31.8130074639153,32.8105788368983,33.8081502098812,
34.8057215828641,35.8032929558471,36.80086432883,37.7984357018129,38.7960070747959,
39.7935784477788,40.7911498207617,41.7887211937447,42.7862925667276,43.7838639397105,
44.7814353126935,45.7790066856764,46.7765780586593,47.7741494316423,48.7717208046252,
49.7692921776081,50.7668635505911,51.764434923574,52.7620062965569,53.7595776695399,
54.7571490425228,55.7547204155057,56.7522917884886,57.7498631614716,58.7474345344545,
59.7450059074374,60.7425772804204,61.7401486534033,62.7377200263862,63.7352913993692,
64.7328627723521,65.730434145335,66.728005518318,67.7255768913009,68.7231482642838,
69.7207196372668,70.7182910102497,71.7158623832326,72.7134337562156,73.7110051291985,
74.7085765021814,75.7061478751644,76.7037192481473,77.7012906211302,78.6988619941132,
79.6964333670961,80.694004740079,81.691576113062,82.6891474860449,83.6867188590278,
84.6842902320108,85.6818616049937,86.6794329779766,87.6770043509596,88.6745757239425,
89.6721470969254,90.6697184699084,91.6672898428913,92.6648612158742,93.6624325888572,
94.6600039618401),.UNSPECIFIED.);
#643=B_SPLINE_SURFACE_WITH_KNOTS('',3,3,((#51104,#51105,#51106,#51107,#51108,
#51109,#51110,#51111,#51112,#51113,#51114,#51115,#51116,#51117,#51118,#51119,
#51120,#51121,#51122,#51123,#51124,#51125,#51126,#51127,#51128,#51129,#51130,
#51131,#51132,#51133,#51134,#51135,#51136,#51137,#51138,#51139,#51140,#51141,
#51142,#51143,#51144,#51145,#51146,#51147,#51148,#51149,#51150,#51151,#51152,
#51153,#51154,#51155,#51156,#51157,#51158,#51159,#51160,#51161,#51162,#51163,
#51164,#51165,#51166,#51167,#51168,#51169,#51170,#51171,#51172,#51173,#51174,
#51175,#51176,#51177,#51178,#51179,#51180,#51181,#51182,#51183,#51184,#51185,
#51186,#51187,#51188,#51189),(#51190,#51191,#51192,#51193,#51194,#51195,
#51196,#51197,#51198,#51199,#51200,#51201,#51202,#51203,#51204,#51205,#51206,
#51207,#51208,#51209,#51210,#51211,#51212,#51213,#51214,#51215,#51216,#51217,
#51218,#51219,#51220,#51221,#51222,#51223,#51224,#51225,#51226,#51227,#51228,
#51229,#51230,#51231,#51232,#51233,#51234,#51235,#51236,#51237,#51238,#51239,
#51240,#51241,#51242,#51243,#51244,#51245,#51246,#51247,#51248,#51249,#51250,
#51251,#51252,#51253,#51254,#51255,#51256,#51257,#51258,#51259,#51260,#51261,
#51262,#51263,#51264,#51265,#51266,#51267,#51268,#51269,#51270,#51271,#51272,
#51273,#51274,#51275),(#51276,#51277,#51278,#51279,#51280,#51281,#51282,
#51283,#51284,#51285,#51286,#51287,#51288,#51289,#51290,#51291,#51292,#51293,
#51294,#51295,#51296,#51297,#51298,#51299,#51300,#51301,#51302,#51303,#51304,
#51305,#51306,#51307,#51308,#51309,#51310,#51311,#51312,#51313,#51314,#51315,
#51316,#51317,#51318,#51319,#51320,#51321,#51322,#51323,#51324,#51325,#51326,
#51327,#51328,#51329,#51330,#51331,#51332,#51333,#51334,#51335,#51336,#51337,
#51338,#51339,#51340,#51341,#51342,#51343,#51344,#51345,#51346,#51347,#51348,
#51349,#51350,#51351,#51352,#51353,#51354,#51355,#51356,#51357,#51358,#51359,
#51360,#51361),(#51362,#51363,#51364,#51365,#51366,#51367,#51368,#51369,
#51370,#51371,#51372,#51373,#51374,#51375,#51376,#51377,#51378,#51379,#51380,
#51381,#51382,#51383,#51384,#51385,#51386,#51387,#51388,#51389,#51390,#51391,
#51392,#51393,#51394,#51395,#51396,#51397,#51398,#51399,#51400,#51401,#51402,
#51403,#51404,#51405,#51406,#51407,#51408,#51409,#51410,#51411,#51412,#51413,
#51414,#51415,#51416,#51417,#51418,#51419,#51420,#51421,#51422,#51423,#51424,
#51425,#51426,#51427,#51428,#51429,#51430,#51431,#51432,#51433,#51434,#51435,
#51436,#51437,#51438,#51439,#51440,#51441,#51442,#51443,#51444,#51445,#51446,
#51447)),.UNSPECIFIED.,.F.,.F.,.F.,(4,4),(4,1,1,1,1,1,1,1,1,1,1,1,1,1,1,
1,1,1,1,1,1,1,1,1,1,1,1,1,1,1,1,1,1,1,1,1,1,1,1,1,1,1,1,1,1,1,1,1,1,1,1,
1,1,1,1,1,1,1,1,1,1,1,1,1,1,1,1,1,1,1,1,1,1,1,1,1,1,1,1,1,1,1,1,4),(0.,
0.0448889834294934),(14.3981410127769,15.3957123857599,16.3932837587428,
17.3908551317257,18.3884265047087,19.3859978776916,20.3835692506745,21.3811406236575,
22.3787119966404,23.3762833696233,24.3738547426063,25.3714261155892,26.3689974885721,
27.3665688615551,28.364140234538,29.3617116075209,30.3592829805038,31.3568543534868,
32.3544257264697,33.3519970994526,34.3495684724356,35.3471398454185,36.3447112184014,
37.3422825913844,38.3398539643673,39.3374253373502,40.3349967103332,41.3325680833161,
42.330139456299,43.327710829282,44.3252822022649,45.3228535752478,46.3204249482308,
47.3179963212137,48.3155676941966,49.3131390671796,50.3107104401625,51.3082818131454,
52.3058531861284,53.3034245591113,54.3009959320942,55.2985673050772,56.2961386780601,
57.293710051043,58.291281424026,59.2888527970089,60.2864241699918,61.2839955429748,
62.2815669159577,63.2791382889406,64.2767096619236,65.2742810349065,66.2718524078894,
67.2694237808724,68.2669951538553,69.2645665268382,70.2621378998212,71.2597092728041,
72.257280645787,73.25485201877,74.2524233917529,75.2499947647358,76.2475661377187,
77.2451375107017,78.2427088836846,79.2402802566675,80.2378516296505,81.2354230026334,
82.2329943756163,83.2305657485993,84.2281371215822,85.2257084945651,86.2232798675481,
87.220851240531,88.2184226135139,89.2159939864969,90.2135653594798,91.2111367324627,
92.2087081054457,93.2062794784286,94.2038508514115,95.2014222243945,96.1989935973774,
97.1965649703603),.UNSPECIFIED.);
#644=B_SPLINE_SURFACE_WITH_KNOTS('',3,3,((#51753,#51754,#51755,#51756,#51757,
#51758,#51759,#51760,#51761,#51762,#51763,#51764,#51765,#51766,#51767,#51768,
#51769,#51770,#51771,#51772,#51773,#51774,#51775,#51776,#51777,#51778,#51779,
#51780,#51781,#51782,#51783,#51784,#51785,#51786,#51787,#51788,#51789,#51790,
#51791,#51792,#51793,#51794,#51795,#51796,#51797,#51798,#51799,#51800,#51801,
#51802,#51803,#51804,#51805,#51806,#51807,#51808,#51809,#51810,#51811,#51812,
#51813,#51814,#51815,#51816,#51817,#51818,#51819,#51820,#51821,#51822,#51823,
#51824,#51825,#51826,#51827,#51828,#51829,#51830,#51831,#51832,#51833,#51834,
#51835,#51836,#51837,#51838),(#51839,#51840,#51841,#51842,#51843,#51844,
#51845,#51846,#51847,#51848,#51849,#51850,#51851,#51852,#51853,#51854,#51855,
#51856,#51857,#51858,#51859,#51860,#51861,#51862,#51863,#51864,#51865,#51866,
#51867,#51868,#51869,#51870,#51871,#51872,#51873,#51874,#51875,#51876,#51877,
#51878,#51879,#51880,#51881,#51882,#51883,#51884,#51885,#51886,#51887,#51888,
#51889,#51890,#51891,#51892,#51893,#51894,#51895,#51896,#51897,#51898,#51899,
#51900,#51901,#51902,#51903,#51904,#51905,#51906,#51907,#51908,#51909,#51910,
#51911,#51912,#51913,#51914,#51915,#51916,#51917,#51918,#51919,#51920,#51921,
#51922,#51923,#51924),(#51925,#51926,#51927,#51928,#51929,#51930,#51931,
#51932,#51933,#51934,#51935,#51936,#51937,#51938,#51939,#51940,#51941,#51942,
#51943,#51944,#51945,#51946,#51947,#51948,#51949,#51950,#51951,#51952,#51953,
#51954,#51955,#51956,#51957,#51958,#51959,#51960,#51961,#51962,#51963,#51964,
#51965,#51966,#51967,#51968,#51969,#51970,#51971,#51972,#51973,#51974,#51975,
#51976,#51977,#51978,#51979,#51980,#51981,#51982,#51983,#51984,#51985,#51986,
#51987,#51988,#51989,#51990,#51991,#51992,#51993,#51994,#51995,#51996,#51997,
#51998,#51999,#52000,#52001,#52002,#52003,#52004,#52005,#52006,#52007,#52008,
#52009,#52010),(#52011,#52012,#52013,#52014,#52015,#52016,#52017,#52018,
#52019,#52020,#52021,#52022,#52023,#52024,#52025,#52026,#52027,#52028,#52029,
#52030,#52031,#52032,#52033,#52034,#52035,#52036,#52037,#52038,#52039,#52040,
#52041,#52042,#52043,#52044,#52045,#52046,#52047,#52048,#52049,#52050,#52051,
#52052,#52053,#52054,#52055,#52056,#52057,#52058,#52059,#52060,#52061,#52062,
#52063,#52064,#52065,#52066,#52067,#52068,#52069,#52070,#52071,#52072,#52073,
#52074,#52075,#52076,#52077,#52078,#52079,#52080,#52081,#52082,#52083,#52084,
#52085,#52086,#52087,#52088,#52089,#52090,#52091,#52092,#52093,#52094,#52095,
#52096)),.UNSPECIFIED.,.F.,.F.,.F.,(4,4),(4,1,1,1,1,1,1,1,1,1,1,1,1,1,1,
1,1,1,1,1,1,1,1,1,1,1,1,1,1,1,1,1,1,1,1,1,1,1,1,1,1,1,1,1,1,1,1,1,1,1,1,
1,1,1,1,1,1,1,1,1,1,1,1,1,1,1,1,1,1,1,1,1,1,1,1,1,1,1,1,1,1,1,1,4),(0.,
0.0448889834294935),(11.8615800042566,12.8591513772396,13.8567227502225,
14.8542941232054,15.8518654961884,16.8494368691713,17.8470082421542,18.8445796151372,
19.8421509881201,20.839722361103,21.837293734086,22.8348651070689,23.8324364800518,
24.8300078530348,25.8275792260177,26.8251505990006,27.8227219719836,28.8202933449665,
29.8178647179494,30.8154360909324,31.8130074639153,32.8105788368982,33.8081502098811,
34.8057215828641,35.803292955847,36.80086432883,37.7984357018129,38.7960070747958,
39.7935784477787,40.7911498207617,41.7887211937446,42.7862925667275,43.7838639397105,
44.7814353126934,45.7790066856763,46.7765780586593,47.7741494316422,48.7717208046251,
49.7692921776081,50.766863550591,51.7644349235739,52.7620062965569,53.7595776695398,
54.7571490425227,55.7547204155057,56.7522917884886,57.7498631614715,58.7474345344545,
59.7450059074374,60.7425772804203,61.7401486534033,62.7377200263862,63.7352913993691,
64.7328627723521,65.730434145335,66.7280055183179,67.7255768913009,68.7231482642838,
69.7207196372667,70.7182910102497,71.7158623832326,72.7134337562155,73.7110051291985,
74.7085765021814,75.7061478751643,76.7037192481473,77.7012906211302,78.6988619941131,
79.696433367096,80.694004740079,81.6915761130619,82.6891474860448,83.6867188590278,
84.6842902320107,85.6818616049936,86.6794329779766,87.6770043509595,88.6745757239424,
89.6721470969254,90.6697184699083,91.6672898428912,92.6648612158742,93.6624325888571,
94.66000396184),.UNSPECIFIED.);
#645=B_SPLINE_SURFACE_WITH_KNOTS('',3,3,((#52204,#52205,#52206,#52207,#52208,
#52209,#52210,#52211,#52212,#52213,#52214,#52215,#52216,#52217,#52218,#52219,
#52220,#52221,#52222,#52223,#52224,#52225,#52226,#52227,#52228,#52229,#52230,
#52231,#52232,#52233,#52234,#52235,#52236,#52237,#52238,#52239,#52240,#52241,
#52242,#52243,#52244,#52245,#52246,#52247,#52248,#52249,#52250,#52251,#52252,
#52253,#52254,#52255,#52256,#52257,#52258,#52259,#52260,#52261,#52262,#52263,
#52264,#52265,#52266,#52267,#52268,#52269,#52270,#52271,#52272,#52273,#52274,
#52275,#52276,#52277,#52278,#52279,#52280,#52281,#52282,#52283,#52284,#52285,
#52286,#52287,#52288,#52289),(#52290,#52291,#52292,#52293,#52294,#52295,
#52296,#52297,#52298,#52299,#52300,#52301,#52302,#52303,#52304,#52305,#52306,
#52307,#52308,#52309,#52310,#52311,#52312,#52313,#52314,#52315,#52316,#52317,
#52318,#52319,#52320,#52321,#52322,#52323,#52324,#52325,#52326,#52327,#52328,
#52329,#52330,#52331,#52332,#52333,#52334,#52335,#52336,#52337,#52338,#52339,
#52340,#52341,#52342,#52343,#52344,#52345,#52346,#52347,#52348,#52349,#52350,
#52351,#52352,#52353,#52354,#52355,#52356,#52357,#52358,#52359,#52360,#52361,
#52362,#52363,#52364,#52365,#52366,#52367,#52368,#52369,#52370,#52371,#52372,
#52373,#52374,#52375),(#52376,#52377,#52378,#52379,#52380,#52381,#52382,
#52383,#52384,#52385,#52386,#52387,#52388,#52389,#52390,#52391,#52392,#52393,
#52394,#52395,#52396,#52397,#52398,#52399,#52400,#52401,#52402,#52403,#52404,
#52405,#52406,#52407,#52408,#52409,#52410,#52411,#52412,#52413,#52414,#52415,
#52416,#52417,#52418,#52419,#52420,#52421,#52422,#52423,#52424,#52425,#52426,
#52427,#52428,#52429,#52430,#52431,#52432,#52433,#52434,#52435,#52436,#52437,
#52438,#52439,#52440,#52441,#52442,#52443,#52444,#52445,#52446,#52447,#52448,
#52449,#52450,#52451,#52452,#52453,#52454,#52455,#52456,#52457,#52458,#52459,
#52460,#52461),(#52462,#52463,#52464,#52465,#52466,#52467,#52468,#52469,
#52470,#52471,#52472,#52473,#52474,#52475,#52476,#52477,#52478,#52479,#52480,
#52481,#52482,#52483,#52484,#52485,#52486,#52487,#52488,#52489,#52490,#52491,
#52492,#52493,#52494,#52495,#52496,#52497,#52498,#52499,#52500,#52501,#52502,
#52503,#52504,#52505,#52506,#52507,#52508,#52509,#52510,#52511,#52512,#52513,
#52514,#52515,#52516,#52517,#52518,#52519,#52520,#52521,#52522,#52523,#52524,
#52525,#52526,#52527,#52528,#52529,#52530,#52531,#52532,#52533,#52534,#52535,
#52536,#52537,#52538,#52539,#52540,#52541,#52542,#52543,#52544,#52545,#52546,
#52547)),.UNSPECIFIED.,.F.,.F.,.F.,(4,4),(4,1,1,1,1,1,1,1,1,1,1,1,1,1,1,
1,1,1,1,1,1,1,1,1,1,1,1,1,1,1,1,1,1,1,1,1,1,1,1,1,1,1,1,1,1,1,1,1,1,1,1,
1,1,1,1,1,1,1,1,1,1,1,1,1,1,1,1,1,1,1,1,1,1,1,1,1,1,1,1,1,1,1,1,4),(0.,
0.0448889834294935),(14.3981410127769,15.3957123857598,16.3932837587428,
17.3908551317257,18.3884265047086,19.3859978776916,20.3835692506745,21.3811406236574,
22.3787119966404,23.3762833696233,24.3738547426062,25.3714261155892,26.3689974885721,
27.366568861555,28.364140234538,29.3617116075209,30.3592829805038,31.3568543534868,
32.3544257264697,33.3519970994526,34.3495684724355,35.3471398454185,36.3447112184014,
37.3422825913843,38.3398539643673,39.3374253373502,40.3349967103332,41.3325680833161,
42.330139456299,43.3277108292819,44.3252822022649,45.3228535752478,46.3204249482307,
47.3179963212137,48.3155676941966,49.3131390671795,50.3107104401625,51.3082818131454,
52.3058531861283,53.3034245591113,54.3009959320942,55.2985673050771,56.2961386780601,
57.293710051043,58.2912814240259,59.2888527970089,60.2864241699918,61.2839955429747,
62.2815669159577,63.2791382889406,64.2767096619235,65.2742810349065,66.2718524078894,
67.2694237808723,68.2669951538553,69.2645665268382,70.2621378998211,71.2597092728041,
72.257280645787,73.2548520187699,74.2524233917529,75.2499947647358,76.2475661377187,
77.2451375107017,78.2427088836846,79.2402802566675,80.2378516296505,81.2354230026334,
82.2329943756163,83.2305657485992,84.2281371215822,85.2257084945651,86.223279867548,
87.220851240531,88.2184226135139,89.2159939864968,90.2135653594798,91.2111367324627,
92.2087081054456,93.2062794784286,94.2038508514115,95.2014222243944,96.1989935973774,
97.1965649703603),.UNSPECIFIED.);
#675=FACE_OUTER_BOUND('',#1672,.T.);
#676=FACE_OUTER_BOUND('',#1673,.T.);
#677=FACE_OUTER_BOUND('',#1674,.T.);
#678=FACE_OUTER_BOUND('',#1675,.T.);
#679=FACE_OUTER_BOUND('',#1676,.T.);
#680=FACE_OUTER_BOUND('',#1677,.T.);
#681=FACE_OUTER_BOUND('',#1678,.T.);
#682=FACE_OUTER_BOUND('',#1679,.T.);
#683=FACE_OUTER_BOUND('',#1680,.T.);
#684=FACE_OUTER_BOUND('',#1681,.T.);
#685=FACE_OUTER_BOUND('',#1682,.T.);
#686=FACE_OUTER_BOUND('',#1683,.T.);
#687=FACE_OUTER_BOUND('',#1684,.T.);
#688=FACE_OUTER_BOUND('',#1685,.T.);
#689=FACE_OUTER_BOUND('',#1686,.T.);
#690=FACE_OUTER_BOUND('',#1687,.T.);
#691=FACE_OUTER_BOUND('',#1688,.T.);
#692=FACE_OUTER_BOUND('',#1689,.T.);
#693=FACE_OUTER_BOUND('',#1690,.T.);
#694=FACE_OUTER_BOUND('',#1691,.T.);
#695=FACE_OUTER_BOUND('',#1692,.T.);
#696=FACE_OUTER_BOUND('',#1693,.T.);
#697=FACE_OUTER_BOUND('',#1694,.T.);
#698=FACE_OUTER_BOUND('',#1695,.T.);
#699=FACE_OUTER_BOUND('',#1696,.T.);
#700=FACE_OUTER_BOUND('',#1697,.T.);
#701=FACE_OUTER_BOUND('',#1698,.T.);
#702=FACE_OUTER_BOUND('',#1699,.T.);
#703=FACE_OUTER_BOUND('',#1700,.T.);
#704=FACE_OUTER_BOUND('',#1701,.T.);
#705=FACE_OUTER_BOUND('',#1702,.T.);
#706=FACE_OUTER_BOUND('',#1703,.T.);
#707=FACE_OUTER_BOUND('',#1704,.T.);
#708=FACE_OUTER_BOUND('',#1705,.T.);
#709=FACE_OUTER_BOUND('',#1706,.T.);
#710=FACE_OUTER_BOUND('',#1707,.T.);
#711=FACE_OUTER_BOUND('',#1708,.T.);
#712=FACE_OUTER_BOUND('',#1709,.T.);
#713=FACE_OUTER_BOUND('',#1710,.T.);
#714=FACE_OUTER_BOUND('',#1711,.T.);
#715=FACE_OUTER_BOUND('',#1712,.T.);
#716=FACE_OUTER_BOUND('',#1713,.T.);
#717=FACE_OUTER_BOUND('',#1714,.T.);
#718=FACE_OUTER_BOUND('',#1715,.T.);
#719=FACE_OUTER_BOUND('',#1716,.T.);
#720=FACE_OUTER_BOUND('',#1717,.T.);
#721=FACE_OUTER_BOUND('',#1718,.T.);
#722=FACE_OUTER_BOUND('',#1719,.T.);
#723=FACE_OUTER_BOUND('',#1720,.T.);
#724=FACE_OUTER_BOUND('',#1721,.T.);
#725=FACE_OUTER_BOUND('',#1722,.T.);
#726=FACE_OUTER_BOUND('',#1723,.T.);
#727=FACE_OUTER_BOUND('',#1724,.T.);
#728=FACE_OUTER_BOUND('',#1725,.T.);
#729=FACE_OUTER_BOUND('',#1726,.T.);
#730=FACE_OUTER_BOUND('',#1727,.T.);
#731=FACE_OUTER_BOUND('',#1728,.T.);
#732=FACE_OUTER_BOUND('',#1729,.T.);
#733=FACE_OUTER_BOUND('',#1730,.T.);
#734=FACE_OUTER_BOUND('',#1731,.T.);
#735=FACE_OUTER_BOUND('',#1732,.T.);
#736=FACE_OUTER_BOUND('',#1733,.T.);
#737=FACE_OUTER_BOUND('',#1734,.T.);
#738=FACE_OUTER_BOUND('',#1735,.T.);
#739=FACE_OUTER_BOUND('',#1736,.T.);
#740=FACE_OUTER_BOUND('',#1737,.T.);
#741=FACE_OUTER_BOUND('',#1738,.T.);
#742=FACE_OUTER_BOUND('',#1739,.T.);
#743=FACE_OUTER_BOUND('',#1740,.T.);
#744=FACE_OUTER_BOUND('',#1741,.T.);
#745=FACE_OUTER_BOUND('',#1742,.T.);
#746=FACE_OUTER_BOUND('',#1743,.T.);
#747=FACE_OUTER_BOUND('',#1744,.T.);
#748=FACE_OUTER_BOUND('',#1745,.T.);
#749=FACE_OUTER_BOUND('',#1746,.T.);
#750=FACE_OUTER_BOUND('',#1747,.T.);
#751=FACE_OUTER_BOUND('',#1748,.T.);
#752=FACE_OUTER_BOUND('',#1749,.T.);
#753=FACE_OUTER_BOUND('',#1750,.T.);
#754=FACE_OUTER_BOUND('',#1751,.T.);
#755=FACE_OUTER_BOUND('',#1752,.T.);
#756=FACE_OUTER_BOUND('',#1753,.T.);
#757=FACE_OUTER_BOUND('',#1754,.T.);
#758=FACE_OUTER_BOUND('',#1755,.T.);
#759=FACE_OUTER_BOUND('',#1756,.T.);
#760=FACE_OUTER_BOUND('',#1757,.T.);
#761=FACE_OUTER_BOUND('',#1758,.T.);
#762=FACE_OUTER_BOUND('',#1759,.T.);
#763=FACE_OUTER_BOUND('',#1760,.T.);
#764=FACE_OUTER_BOUND('',#1761,.T.);
#765=FACE_OUTER_BOUND('',#1762,.T.);
#766=FACE_OUTER_BOUND('',#1763,.T.);
#767=FACE_OUTER_BOUND('',#1764,.T.);
#768=FACE_OUTER_BOUND('',#1765,.T.);
#769=FACE_OUTER_BOUND('',#1766,.T.);
#770=FACE_OUTER_BOUND('',#1767,.T.);
#771=FACE_OUTER_BOUND('',#1768,.T.);
#772=FACE_OUTER_BOUND('',#1769,.T.);
#773=FACE_OUTER_BOUND('',#1770,.T.);
#774=FACE_OUTER_BOUND('',#1771,.T.);
#775=FACE_OUTER_BOUND('',#1772,.T.);
#776=FACE_OUTER_BOUND('',#1773,.T.);
#777=FACE_OUTER_BOUND('',#1774,.T.);
#778=FACE_OUTER_BOUND('',#1775,.T.);
#779=FACE_OUTER_BOUND('',#1776,.T.);
#780=FACE_OUTER_BOUND('',#1777,.T.);
#781=FACE_OUTER_BOUND('',#1778,.T.);
#782=FACE_OUTER_BOUND('',#1779,.T.);
#783=FACE_OUTER_BOUND('',#1780,.T.);
#784=FACE_OUTER_BOUND('',#1781,.T.);
#785=FACE_OUTER_BOUND('',#1782,.T.);
#786=FACE_OUTER_BOUND('',#1783,.T.);
#787=FACE_OUTER_BOUND('',#1784,.T.);
#788=FACE_OUTER_BOUND('',#1785,.T.);
#789=FACE_OUTER_BOUND('',#1786,.T.);
#790=FACE_OUTER_BOUND('',#1787,.T.);
#791=FACE_OUTER_BOUND('',#1788,.T.);
#792=FACE_OUTER_BOUND('',#1789,.T.);
#793=FACE_OUTER_BOUND('',#1790,.T.);
#794=FACE_OUTER_BOUND('',#1791,.T.);
#795=FACE_OUTER_BOUND('',#1792,.T.);
#796=FACE_OUTER_BOUND('',#1793,.T.);
#797=FACE_OUTER_BOUND('',#1794,.T.);
#798=FACE_OUTER_BOUND('',#1795,.T.);
#799=FACE_OUTER_BOUND('',#1796,.T.);
#800=FACE_OUTER_BOUND('',#1797,.T.);
#801=FACE_OUTER_BOUND('',#1798,.T.);
#802=FACE_OUTER_BOUND('',#1799,.T.);
#803=FACE_OUTER_BOUND('',#1800,.T.);
#804=FACE_OUTER_BOUND('',#1801,.T.);
#805=FACE_OUTER_BOUND('',#1802,.T.);
#806=FACE_OUTER_BOUND('',#1803,.T.);
#807=FACE_OUTER_BOUND('',#1804,.T.);
#808=FACE_OUTER_BOUND('',#1805,.T.);
#809=FACE_OUTER_BOUND('',#1806,.T.);
#810=FACE_OUTER_BOUND('',#1807,.T.);
#811=FACE_OUTER_BOUND('',#1808,.T.);
#812=FACE_OUTER_BOUND('',#1809,.T.);
#813=FACE_OUTER_BOUND('',#1810,.T.);
#814=FACE_OUTER_BOUND('',#1811,.T.);
#815=FACE_OUTER_BOUND('',#1812,.T.);
#816=FACE_OUTER_BOUND('',#1813,.T.);
#817=FACE_OUTER_BOUND('',#1814,.T.);
#818=FACE_OUTER_BOUND('',#1815,.T.);
#819=FACE_OUTER_BOUND('',#1816,.T.);
#820=FACE_OUTER_BOUND('',#1817,.T.);
#821=FACE_OUTER_BOUND('',#1818,.T.);
#822=FACE_OUTER_BOUND('',#1819,.T.);
#823=FACE_OUTER_BOUND('',#1820,.T.);
#824=FACE_OUTER_BOUND('',#1821,.T.);
#825=FACE_OUTER_BOUND('',#1822,.T.);
#826=FACE_OUTER_BOUND('',#1823,.T.);
#827=FACE_OUTER_BOUND('',#1824,.T.);
#828=FACE_OUTER_BOUND('',#1825,.T.);
#829=FACE_OUTER_BOUND('',#1826,.T.);
#830=FACE_OUTER_BOUND('',#1827,.T.);
#831=FACE_OUTER_BOUND('',#1828,.T.);
#832=FACE_OUTER_BOUND('',#1829,.T.);
#833=FACE_OUTER_BOUND('',#1830,.T.);
#834=FACE_OUTER_BOUND('',#1831,.T.);
#835=FACE_OUTER_BOUND('',#1832,.T.);
#836=FACE_OUTER_BOUND('',#1833,.T.);
#837=FACE_OUTER_BOUND('',#1834,.T.);
#838=FACE_OUTER_BOUND('',#1835,.T.);
#839=FACE_OUTER_BOUND('',#1836,.T.);
#840=FACE_OUTER_BOUND('',#1837,.T.);
#841=FACE_OUTER_BOUND('',#1838,.T.);
#842=FACE_OUTER_BOUND('',#1839,.T.);
#843=FACE_OUTER_BOUND('',#1840,.T.);
#844=FACE_OUTER_BOUND('',#1841,.T.);
#845=FACE_OUTER_BOUND('',#1842,.T.);
#846=FACE_OUTER_BOUND('',#1843,.T.);
#847=FACE_OUTER_BOUND('',#1844,.T.);
#848=FACE_OUTER_BOUND('',#1845,.T.);
#849=FACE_OUTER_BOUND('',#1846,.T.);
#850=FACE_OUTER_BOUND('',#1847,.T.);
#851=FACE_OUTER_BOUND('',#1848,.T.);
#852=FACE_OUTER_BOUND('',#1849,.T.);
#853=FACE_OUTER_BOUND('',#1850,.T.);
#854=FACE_OUTER_BOUND('',#1851,.T.);
#855=FACE_OUTER_BOUND('',#1852,.T.);
#856=FACE_OUTER_BOUND('',#1853,.T.);
#857=FACE_OUTER_BOUND('',#1854,.T.);
#858=FACE_OUTER_BOUND('',#1855,.T.);
#859=FACE_OUTER_BOUND('',#1856,.T.);
#860=FACE_OUTER_BOUND('',#1857,.T.);
#861=FACE_OUTER_BOUND('',#1858,.T.);
#862=FACE_OUTER_BOUND('',#1859,.T.);
#863=FACE_OUTER_BOUND('',#1860,.T.);
#864=FACE_OUTER_BOUND('',#1861,.T.);
#865=FACE_OUTER_BOUND('',#1862,.T.);
#866=FACE_OUTER_BOUND('',#1863,.T.);
#867=FACE_OUTER_BOUND('',#1864,.T.);
#868=FACE_OUTER_BOUND('',#1865,.T.);
#869=FACE_OUTER_BOUND('',#1866,.T.);
#870=FACE_OUTER_BOUND('',#1867,.T.);
#871=FACE_OUTER_BOUND('',#1868,.T.);
#872=FACE_OUTER_BOUND('',#1869,.T.);
#873=FACE_OUTER_BOUND('',#1870,.T.);
#874=FACE_OUTER_BOUND('',#1871,.T.);
#875=FACE_OUTER_BOUND('',#1872,.T.);
#876=FACE_OUTER_BOUND('',#1873,.T.);
#877=FACE_OUTER_BOUND('',#1874,.T.);
#878=FACE_OUTER_BOUND('',#1875,.T.);
#879=FACE_OUTER_BOUND('',#1876,.T.);
#880=FACE_OUTER_BOUND('',#1877,.T.);
#881=FACE_OUTER_BOUND('',#1878,.T.);
#882=FACE_OUTER_BOUND('',#1879,.T.);
#883=FACE_OUTER_BOUND('',#1880,.T.);
#884=FACE_OUTER_BOUND('',#1881,.T.);
#885=FACE_OUTER_BOUND('',#1882,.T.);
#886=FACE_OUTER_BOUND('',#1883,.T.);
#887=FACE_OUTER_BOUND('',#1884,.T.);
#888=FACE_OUTER_BOUND('',#1885,.T.);
#889=FACE_OUTER_BOUND('',#1886,.T.);
#890=FACE_OUTER_BOUND('',#1887,.T.);
#891=FACE_OUTER_BOUND('',#1888,.T.);
#892=FACE_OUTER_BOUND('',#1889,.T.);
#893=FACE_OUTER_BOUND('',#1890,.T.);
#894=FACE_OUTER_BOUND('',#1891,.T.);
#895=FACE_OUTER_BOUND('',#1892,.T.);
#896=FACE_OUTER_BOUND('',#1893,.T.);
#897=FACE_OUTER_BOUND('',#1894,.T.);
#898=FACE_OUTER_BOUND('',#1895,.T.);
#899=FACE_OUTER_BOUND('',#1896,.T.);
#900=FACE_OUTER_BOUND('',#1897,.T.);
#901=FACE_OUTER_BOUND('',#1898,.T.);
#902=FACE_OUTER_BOUND('',#1899,.T.);
#903=FACE_OUTER_BOUND('',#1900,.T.);
#904=FACE_OUTER_BOUND('',#1901,.T.);
#905=FACE_OUTER_BOUND('',#1902,.T.);
#906=FACE_OUTER_BOUND('',#1903,.T.);
#907=FACE_OUTER_BOUND('',#1904,.T.);
#908=FACE_OUTER_BOUND('',#1905,.T.);
#909=FACE_OUTER_BOUND('',#1906,.T.);
#910=FACE_OUTER_BOUND('',#1907,.T.);
#911=FACE_OUTER_BOUND('',#1908,.T.);
#912=FACE_OUTER_BOUND('',#1909,.T.);
#913=FACE_OUTER_BOUND('',#1910,.T.);
#914=FACE_OUTER_BOUND('',#1911,.T.);
#915=FACE_OUTER_BOUND('',#1912,.T.);
#916=FACE_OUTER_BOUND('',#1913,.T.);
#917=FACE_OUTER_BOUND('',#1914,.T.);
#918=FACE_OUTER_BOUND('',#1915,.T.);
#919=FACE_OUTER_BOUND('',#1916,.T.);
#920=FACE_OUTER_BOUND('',#1917,.T.);
#921=FACE_OUTER_BOUND('',#1918,.T.);
#922=FACE_OUTER_BOUND('',#1919,.T.);
#923=FACE_OUTER_BOUND('',#1920,.T.);
#924=FACE_OUTER_BOUND('',#1921,.T.);
#925=FACE_OUTER_BOUND('',#1922,.T.);
#926=FACE_OUTER_BOUND('',#1923,.T.);
#927=FACE_OUTER_BOUND('',#1924,.T.);
#928=FACE_OUTER_BOUND('',#1925,.T.);
#929=FACE_OUTER_BOUND('',#1926,.T.);
#930=FACE_OUTER_BOUND('',#1927,.T.);
#931=FACE_OUTER_BOUND('',#1928,.T.);
#932=FACE_OUTER_BOUND('',#1929,.T.);
#933=FACE_OUTER_BOUND('',#1930,.T.);
#934=FACE_OUTER_BOUND('',#1931,.T.);
#935=FACE_OUTER_BOUND('',#1932,.T.);
#936=FACE_OUTER_BOUND('',#1933,.T.);
#937=FACE_OUTER_BOUND('',#1934,.T.);
#938=FACE_OUTER_BOUND('',#1935,.T.);
#939=FACE_OUTER_BOUND('',#1936,.T.);
#940=FACE_OUTER_BOUND('',#1937,.T.);
#941=FACE_OUTER_BOUND('',#1938,.T.);
#942=FACE_OUTER_BOUND('',#1939,.T.);
#943=FACE_OUTER_BOUND('',#1940,.T.);
#944=FACE_OUTER_BOUND('',#1941,.T.);
#945=FACE_OUTER_BOUND('',#1942,.T.);
#946=FACE_OUTER_BOUND('',#1943,.T.);
#947=FACE_OUTER_BOUND('',#1944,.T.);
#948=FACE_OUTER_BOUND('',#1945,.T.);
#949=FACE_OUTER_BOUND('',#1946,.T.);
#950=FACE_OUTER_BOUND('',#1947,.T.);
#951=FACE_OUTER_BOUND('',#1948,.T.);
#952=FACE_OUTER_BOUND('',#1949,.T.);
#953=FACE_OUTER_BOUND('',#1950,.T.);
#954=FACE_OUTER_BOUND('',#1951,.T.);
#955=FACE_OUTER_BOUND('',#1952,.T.);
#956=FACE_OUTER_BOUND('',#1953,.T.);
#957=FACE_OUTER_BOUND('',#1954,.T.);
#958=FACE_OUTER_BOUND('',#1955,.T.);
#959=FACE_OUTER_BOUND('',#1956,.T.);
#960=FACE_OUTER_BOUND('',#1957,.T.);
#961=FACE_OUTER_BOUND('',#1958,.T.);
#962=FACE_OUTER_BOUND('',#1959,.T.);
#963=FACE_OUTER_BOUND('',#1960,.T.);
#964=FACE_OUTER_BOUND('',#1961,.T.);
#965=FACE_OUTER_BOUND('',#1962,.T.);
#966=FACE_OUTER_BOUND('',#1963,.T.);
#967=FACE_OUTER_BOUND('',#1964,.T.);
#968=FACE_OUTER_BOUND('',#1965,.T.);
#969=FACE_OUTER_BOUND('',#1966,.T.);
#970=FACE_OUTER_BOUND('',#1967,.T.);
#971=FACE_OUTER_BOUND('',#1968,.T.);
#972=FACE_OUTER_BOUND('',#1969,.T.);
#973=FACE_OUTER_BOUND('',#1970,.T.);
#974=FACE_OUTER_BOUND('',#1971,.T.);
#975=FACE_OUTER_BOUND('',#1972,.T.);
#976=FACE_OUTER_BOUND('',#1973,.T.);
#977=FACE_OUTER_BOUND('',#1974,.T.);
#978=FACE_OUTER_BOUND('',#1975,.T.);
#979=FACE_OUTER_BOUND('',#1976,.T.);
#980=FACE_OUTER_BOUND('',#1977,.T.);
#981=FACE_OUTER_BOUND('',#1978,.T.);
#982=FACE_OUTER_BOUND('',#1979,.T.);
#983=FACE_OUTER_BOUND('',#1980,.T.);
#984=FACE_OUTER_BOUND('',#1981,.T.);
#985=FACE_OUTER_BOUND('',#1982,.T.);
#986=FACE_OUTER_BOUND('',#1983,.T.);
#987=FACE_OUTER_BOUND('',#1984,.T.);
#988=FACE_OUTER_BOUND('',#1985,.T.);
#989=FACE_OUTER_BOUND('',#1986,.T.);
#990=FACE_OUTER_BOUND('',#1987,.T.);
#991=FACE_OUTER_BOUND('',#1988,.T.);
#992=FACE_OUTER_BOUND('',#1989,.T.);
#993=FACE_OUTER_BOUND('',#1990,.T.);
#994=FACE_OUTER_BOUND('',#1991,.T.);
#995=FACE_OUTER_BOUND('',#1992,.T.);
#996=FACE_OUTER_BOUND('',#1993,.T.);
#997=FACE_OUTER_BOUND('',#1994,.T.);
#998=FACE_OUTER_BOUND('',#1995,.T.);
#999=FACE_OUTER_BOUND('',#1996,.T.);
#1000=FACE_OUTER_BOUND('',#1997,.T.);
#1001=FACE_OUTER_BOUND('',#1998,.T.);
#1002=FACE_OUTER_BOUND('',#1999,.T.);
#1003=FACE_OUTER_BOUND('',#2000,.T.);
#1004=FACE_OUTER_BOUND('',#2001,.T.);
#1005=FACE_OUTER_BOUND('',#2002,.T.);
#1006=FACE_OUTER_BOUND('',#2003,.T.);
#1007=FACE_OUTER_BOUND('',#2004,.T.);
#1008=FACE_OUTER_BOUND('',#2005,.T.);
#1009=FACE_OUTER_BOUND('',#2006,.T.);
#1010=FACE_OUTER_BOUND('',#2007,.T.);
#1011=FACE_OUTER_BOUND('',#2008,.T.);
#1012=FACE_OUTER_BOUND('',#2009,.T.);
#1013=FACE_OUTER_BOUND('',#2010,.T.);
#1014=FACE_OUTER_BOUND('',#2011,.T.);
#1015=FACE_OUTER_BOUND('',#2012,.T.);
#1016=FACE_OUTER_BOUND('',#2013,.T.);
#1017=FACE_OUTER_BOUND('',#2014,.T.);
#1018=FACE_OUTER_BOUND('',#2015,.T.);
#1019=FACE_OUTER_BOUND('',#2016,.T.);
#1020=FACE_OUTER_BOUND('',#2017,.T.);
#1021=FACE_OUTER_BOUND('',#2018,.T.);
#1022=FACE_OUTER_BOUND('',#2019,.T.);
#1023=FACE_OUTER_BOUND('',#2020,.T.);
#1024=FACE_OUTER_BOUND('',#2021,.T.);
#1025=FACE_OUTER_BOUND('',#2022,.T.);
#1026=FACE_OUTER_BOUND('',#2023,.T.);
#1027=FACE_OUTER_BOUND('',#2024,.T.);
#1028=FACE_OUTER_BOUND('',#2025,.T.);
#1029=FACE_OUTER_BOUND('',#2026,.T.);
#1030=FACE_OUTER_BOUND('',#2027,.T.);
#1031=FACE_OUTER_BOUND('',#2028,.T.);
#1032=FACE_OUTER_BOUND('',#2029,.T.);
#1033=FACE_OUTER_BOUND('',#2030,.T.);
#1034=FACE_OUTER_BOUND('',#2031,.T.);
#1035=FACE_OUTER_BOUND('',#2032,.T.);
#1036=FACE_OUTER_BOUND('',#2033,.T.);
#1037=FACE_OUTER_BOUND('',#2034,.T.);
#1038=FACE_OUTER_BOUND('',#2035,.T.);
#1039=FACE_OUTER_BOUND('',#2036,.T.);
#1040=FACE_OUTER_BOUND('',#2037,.T.);
#1041=FACE_OUTER_BOUND('',#2038,.T.);
#1042=FACE_OUTER_BOUND('',#2039,.T.);
#1043=FACE_OUTER_BOUND('',#2040,.T.);
#1044=FACE_OUTER_BOUND('',#2041,.T.);
#1045=FACE_OUTER_BOUND('',#2042,.T.);
#1046=FACE_OUTER_BOUND('',#2043,.T.);
#1047=FACE_OUTER_BOUND('',#2044,.T.);
#1048=FACE_OUTER_BOUND('',#2045,.T.);
#1049=FACE_OUTER_BOUND('',#2046,.T.);
#1050=FACE_OUTER_BOUND('',#2047,.T.);
#1051=FACE_OUTER_BOUND('',#2048,.T.);
#1052=FACE_OUTER_BOUND('',#2049,.T.);
#1053=FACE_OUTER_BOUND('',#2050,.T.);
#1054=FACE_OUTER_BOUND('',#2051,.T.);
#1055=FACE_OUTER_BOUND('',#2052,.T.);
#1056=FACE_OUTER_BOUND('',#2053,.T.);
#1057=FACE_OUTER_BOUND('',#2054,.T.);
#1058=FACE_OUTER_BOUND('',#2055,.T.);
#1059=FACE_OUTER_BOUND('',#2056,.T.);
#1060=FACE_OUTER_BOUND('',#2057,.T.);
#1061=FACE_OUTER_BOUND('',#2058,.T.);
#1062=FACE_OUTER_BOUND('',#2059,.T.);
#1063=FACE_OUTER_BOUND('',#2060,.T.);
#1064=FACE_OUTER_BOUND('',#2061,.T.);
#1065=FACE_OUTER_BOUND('',#2062,.T.);
#1066=FACE_OUTER_BOUND('',#2063,.T.);
#1067=FACE_OUTER_BOUND('',#2064,.T.);
#1068=FACE_OUTER_BOUND('',#2065,.T.);
#1069=FACE_OUTER_BOUND('',#2066,.T.);
#1070=FACE_OUTER_BOUND('',#2067,.T.);
#1071=FACE_OUTER_BOUND('',#2068,.T.);
#1072=FACE_OUTER_BOUND('',#2069,.T.);
#1073=FACE_OUTER_BOUND('',#2070,.T.);
#1074=FACE_OUTER_BOUND('',#2071,.T.);
#1075=FACE_OUTER_BOUND('',#2072,.T.);
#1076=FACE_OUTER_BOUND('',#2073,.T.);
#1077=FACE_OUTER_BOUND('',#2074,.T.);
#1078=FACE_OUTER_BOUND('',#2075,.T.);
#1079=FACE_OUTER_BOUND('',#2076,.T.);
#1080=FACE_OUTER_BOUND('',#2077,.T.);
#1081=FACE_OUTER_BOUND('',#2078,.T.);
#1082=FACE_OUTER_BOUND('',#2079,.T.);
#1083=FACE_OUTER_BOUND('',#2080,.T.);
#1084=FACE_OUTER_BOUND('',#2081,.T.);
#1085=FACE_OUTER_BOUND('',#2082,.T.);
#1086=FACE_OUTER_BOUND('',#2083,.T.);
#1087=FACE_OUTER_BOUND('',#2084,.T.);
#1088=FACE_OUTER_BOUND('',#2085,.T.);
#1089=FACE_OUTER_BOUND('',#2086,.T.);
#1090=FACE_OUTER_BOUND('',#2087,.T.);
#1091=FACE_OUTER_BOUND('',#2088,.T.);
#1092=FACE_OUTER_BOUND('',#2089,.T.);
#1093=FACE_OUTER_BOUND('',#2090,.T.);
#1094=FACE_OUTER_BOUND('',#2091,.T.);
#1095=FACE_OUTER_BOUND('',#2092,.T.);
#1096=FACE_OUTER_BOUND('',#2093,.T.);
#1097=FACE_OUTER_BOUND('',#2094,.T.);
#1098=FACE_OUTER_BOUND('',#2095,.T.);
#1099=FACE_OUTER_BOUND('',#2096,.T.);
#1100=FACE_OUTER_BOUND('',#2097,.T.);
#1101=FACE_OUTER_BOUND('',#2098,.T.);
#1102=FACE_OUTER_BOUND('',#2099,.T.);
#1103=FACE_OUTER_BOUND('',#2100,.T.);
#1104=FACE_OUTER_BOUND('',#2101,.T.);
#1105=FACE_OUTER_BOUND('',#2102,.T.);
#1106=FACE_OUTER_BOUND('',#2103,.T.);
#1107=FACE_OUTER_BOUND('',#2104,.T.);
#1108=FACE_OUTER_BOUND('',#2105,.T.);
#1109=FACE_OUTER_BOUND('',#2106,.T.);
#1110=FACE_OUTER_BOUND('',#2107,.T.);
#1111=FACE_OUTER_BOUND('',#2108,.T.);
#1112=FACE_OUTER_BOUND('',#2109,.T.);
#1113=FACE_OUTER_BOUND('',#2110,.T.);
#1114=FACE_OUTER_BOUND('',#2111,.T.);
#1115=FACE_OUTER_BOUND('',#2112,.T.);
#1116=FACE_OUTER_BOUND('',#2113,.T.);
#1117=FACE_OUTER_BOUND('',#2114,.T.);
#1118=FACE_OUTER_BOUND('',#2115,.T.);
#1119=FACE_OUTER_BOUND('',#2116,.T.);
#1120=FACE_OUTER_BOUND('',#2117,.T.);
#1121=FACE_OUTER_BOUND('',#2118,.T.);
#1122=FACE_OUTER_BOUND('',#2119,.T.);
#1123=FACE_OUTER_BOUND('',#2120,.T.);
#1124=FACE_OUTER_BOUND('',#2121,.T.);
#1125=FACE_OUTER_BOUND('',#2122,.T.);
#1126=FACE_OUTER_BOUND('',#2123,.T.);
#1127=FACE_OUTER_BOUND('',#2124,.T.);
#1128=FACE_OUTER_BOUND('',#2125,.T.);
#1129=FACE_OUTER_BOUND('',#2126,.T.);
#1130=FACE_OUTER_BOUND('',#2127,.T.);
#1131=FACE_OUTER_BOUND('',#2128,.T.);
#1132=FACE_OUTER_BOUND('',#2129,.T.);
#1133=FACE_OUTER_BOUND('',#2134,.T.);
#1134=FACE_OUTER_BOUND('',#2142,.T.);
#1672=EDGE_LOOP('',(#11018,#11019,#11020,#11021,#11022,#11023,#11024,#11025));
#1673=EDGE_LOOP('',(#11026,#11027,#11028,#11029));
#1674=EDGE_LOOP('',(#11030,#11031,#11032,#11033));
#1675=EDGE_LOOP('',(#11034,#11035,#11036,#11037));
#1676=EDGE_LOOP('',(#11038,#11039,#11040,#11041));
#1677=EDGE_LOOP('',(#11042,#11043,#11044,#11045));
#1678=EDGE_LOOP('',(#11046,#11047,#11048,#11049));
#1679=EDGE_LOOP('',(#11050,#11051,#11052,#11053));
#1680=EDGE_LOOP('',(#11054,#11055,#11056,#11057));
#1681=EDGE_LOOP('',(#11058,#11059,#11060,#11061));
#1682=EDGE_LOOP('',(#11062,#11063,#11064,#11065));
#1683=EDGE_LOOP('',(#11066,#11067,#11068,#11069));
#1684=EDGE_LOOP('',(#11070,#11071,#11072,#11073));
#1685=EDGE_LOOP('',(#11074,#11075,#11076,#11077));
#1686=EDGE_LOOP('',(#11078,#11079,#11080,#11081));
#1687=EDGE_LOOP('',(#11082,#11083,#11084,#11085));
#1688=EDGE_LOOP('',(#11086,#11087,#11088,#11089));
#1689=EDGE_LOOP('',(#11090,#11091,#11092,#11093));
#1690=EDGE_LOOP('',(#11094,#11095,#11096,#11097));
#1691=EDGE_LOOP('',(#11098,#11099,#11100,#11101));
#1692=EDGE_LOOP('',(#11102,#11103,#11104,#11105));
#1693=EDGE_LOOP('',(#11106,#11107,#11108,#11109));
#1694=EDGE_LOOP('',(#11110,#11111,#11112,#11113));
#1695=EDGE_LOOP('',(#11114,#11115,#11116,#11117));
#1696=EDGE_LOOP('',(#11118,#11119,#11120,#11121));
#1697=EDGE_LOOP('',(#11122,#11123,#11124,#11125,#11126,#11127,#11128,#11129));
#1698=EDGE_LOOP('',(#11130,#11131,#11132,#11133));
#1699=EDGE_LOOP('',(#11134,#11135,#11136,#11137));
#1700=EDGE_LOOP('',(#11138,#11139,#11140,#11141));
#1701=EDGE_LOOP('',(#11142,#11143,#11144,#11145));
#1702=EDGE_LOOP('',(#11146,#11147,#11148,#11149));
#1703=EDGE_LOOP('',(#11150,#11151,#11152,#11153));
#1704=EDGE_LOOP('',(#11154,#11155,#11156,#11157));
#1705=EDGE_LOOP('',(#11158,#11159,#11160,#11161));
#1706=EDGE_LOOP('',(#11162,#11163,#11164,#11165));
#1707=EDGE_LOOP('',(#11166,#11167,#11168,#11169));
#1708=EDGE_LOOP('',(#11170,#11171,#11172,#11173));
#1709=EDGE_LOOP('',(#11174,#11175,#11176,#11177));
#1710=EDGE_LOOP('',(#11178,#11179,#11180,#11181));
#1711=EDGE_LOOP('',(#11182,#11183,#11184,#11185));
#1712=EDGE_LOOP('',(#11186,#11187,#11188,#11189));
#1713=EDGE_LOOP('',(#11190,#11191,#11192,#11193));
#1714=EDGE_LOOP('',(#11194,#11195,#11196,#11197));
#1715=EDGE_LOOP('',(#11198,#11199,#11200,#11201));
#1716=EDGE_LOOP('',(#11202,#11203,#11204,#11205));
#1717=EDGE_LOOP('',(#11206,#11207,#11208,#11209));
#1718=EDGE_LOOP('',(#11210,#11211,#11212,#11213));
#1719=EDGE_LOOP('',(#11214,#11215,#11216,#11217));
#1720=EDGE_LOOP('',(#11218,#11219,#11220,#11221));
#1721=EDGE_LOOP('',(#11222,#11223,#11224,#11225));
#1722=EDGE_LOOP('',(#11226,#11227,#11228,#11229,#11230,#11231,#11232,#11233));
#1723=EDGE_LOOP('',(#11234,#11235,#11236,#11237));
#1724=EDGE_LOOP('',(#11238,#11239,#11240,#11241));
#1725=EDGE_LOOP('',(#11242,#11243,#11244,#11245));
#1726=EDGE_LOOP('',(#11246,#11247,#11248,#11249));
#1727=EDGE_LOOP('',(#11250,#11251,#11252,#11253));
#1728=EDGE_LOOP('',(#11254,#11255,#11256,#11257));
#1729=EDGE_LOOP('',(#11258,#11259,#11260,#11261));
#1730=EDGE_LOOP('',(#11262,#11263,#11264,#11265));
#1731=EDGE_LOOP('',(#11266,#11267,#11268,#11269));
#1732=EDGE_LOOP('',(#11270,#11271,#11272,#11273));
#1733=EDGE_LOOP('',(#11274,#11275,#11276,#11277));
#1734=EDGE_LOOP('',(#11278,#11279,#11280,#11281));
#1735=EDGE_LOOP('',(#11282,#11283,#11284,#11285));
#1736=EDGE_LOOP('',(#11286,#11287,#11288,#11289));
#1737=EDGE_LOOP('',(#11290,#11291,#11292,#11293));
#1738=EDGE_LOOP('',(#11294,#11295,#11296,#11297));
#1739=EDGE_LOOP('',(#11298,#11299,#11300,#11301));
#1740=EDGE_LOOP('',(#11302,#11303,#11304,#11305));
#1741=EDGE_LOOP('',(#11306,#11307,#11308,#11309));
#1742=EDGE_LOOP('',(#11310,#11311,#11312,#11313));
#1743=EDGE_LOOP('',(#11314,#11315,#11316,#11317));
#1744=EDGE_LOOP('',(#11318,#11319,#11320,#11321));
#1745=EDGE_LOOP('',(#11322,#11323,#11324,#11325));
#1746=EDGE_LOOP('',(#11326,#11327,#11328,#11329));
#1747=EDGE_LOOP('',(#11330,#11331,#11332,#11333,#11334,#11335,#11336,#11337));
#1748=EDGE_LOOP('',(#11338,#11339,#11340,#11341));
#1749=EDGE_LOOP('',(#11342,#11343,#11344,#11345));
#1750=EDGE_LOOP('',(#11346,#11347,#11348,#11349));
#1751=EDGE_LOOP('',(#11350,#11351,#11352,#11353));
#1752=EDGE_LOOP('',(#11354,#11355,#11356,#11357));
#1753=EDGE_LOOP('',(#11358,#11359,#11360,#11361));
#1754=EDGE_LOOP('',(#11362,#11363,#11364,#11365));
#1755=EDGE_LOOP('',(#11366,#11367,#11368,#11369));
#1756=EDGE_LOOP('',(#11370,#11371,#11372,#11373));
#1757=EDGE_LOOP('',(#11374,#11375,#11376,#11377));
#1758=EDGE_LOOP('',(#11378,#11379,#11380,#11381));
#1759=EDGE_LOOP('',(#11382,#11383,#11384,#11385));
#1760=EDGE_LOOP('',(#11386,#11387,#11388,#11389));
#1761=EDGE_LOOP('',(#11390,#11391,#11392,#11393));
#1762=EDGE_LOOP('',(#11394,#11395,#11396,#11397));
#1763=EDGE_LOOP('',(#11398,#11399,#11400,#11401));
#1764=EDGE_LOOP('',(#11402,#11403,#11404,#11405));
#1765=EDGE_LOOP('',(#11406,#11407,#11408,#11409));
#1766=EDGE_LOOP('',(#11410,#11411,#11412,#11413));
#1767=EDGE_LOOP('',(#11414,#11415,#11416,#11417));
#1768=EDGE_LOOP('',(#11418,#11419,#11420,#11421));
#1769=EDGE_LOOP('',(#11422,#11423,#11424,#11425));
#1770=EDGE_LOOP('',(#11426,#11427,#11428,#11429));
#1771=EDGE_LOOP('',(#11430,#11431,#11432,#11433));
#1772=EDGE_LOOP('',(#11434,#11435,#11436,#11437,#11438,#11439,#11440,#11441));
#1773=EDGE_LOOP('',(#11442,#11443,#11444,#11445));
#1774=EDGE_LOOP('',(#11446,#11447,#11448,#11449));
#1775=EDGE_LOOP('',(#11450,#11451,#11452,#11453));
#1776=EDGE_LOOP('',(#11454,#11455,#11456,#11457));
#1777=EDGE_LOOP('',(#11458,#11459,#11460,#11461));
#1778=EDGE_LOOP('',(#11462,#11463,#11464,#11465));
#1779=EDGE_LOOP('',(#11466,#11467,#11468,#11469));
#1780=EDGE_LOOP('',(#11470,#11471,#11472,#11473));
#1781=EDGE_LOOP('',(#11474,#11475,#11476,#11477));
#1782=EDGE_LOOP('',(#11478,#11479,#11480,#11481));
#1783=EDGE_LOOP('',(#11482,#11483,#11484,#11485));
#1784=EDGE_LOOP('',(#11486,#11487,#11488,#11489));
#1785=EDGE_LOOP('',(#11490,#11491,#11492,#11493));
#1786=EDGE_LOOP('',(#11494,#11495,#11496,#11497));
#1787=EDGE_LOOP('',(#11498,#11499,#11500,#11501));
#1788=EDGE_LOOP('',(#11502,#11503,#11504,#11505));
#1789=EDGE_LOOP('',(#11506,#11507,#11508,#11509));
#1790=EDGE_LOOP('',(#11510,#11511,#11512,#11513));
#1791=EDGE_LOOP('',(#11514,#11515,#11516,#11517));
#1792=EDGE_LOOP('',(#11518,#11519,#11520,#11521));
#1793=EDGE_LOOP('',(#11522,#11523,#11524,#11525));
#1794=EDGE_LOOP('',(#11526,#11527,#11528,#11529));
#1795=EDGE_LOOP('',(#11530,#11531,#11532,#11533));
#1796=EDGE_LOOP('',(#11534,#11535,#11536,#11537));
#1797=EDGE_LOOP('',(#11538,#11539,#11540,#11541,#11542,#11543,#11544,#11545));
#1798=EDGE_LOOP('',(#11546,#11547,#11548,#11549));
#1799=EDGE_LOOP('',(#11550,#11551,#11552,#11553));
#1800=EDGE_LOOP('',(#11554,#11555,#11556,#11557));
#1801=EDGE_LOOP('',(#11558,#11559,#11560,#11561));
#1802=EDGE_LOOP('',(#11562,#11563,#11564,#11565));
#1803=EDGE_LOOP('',(#11566,#11567,#11568,#11569));
#1804=EDGE_LOOP('',(#11570,#11571,#11572,#11573));
#1805=EDGE_LOOP('',(#11574,#11575,#11576,#11577));
#1806=EDGE_LOOP('',(#11578,#11579,#11580,#11581));
#1807=EDGE_LOOP('',(#11582,#11583,#11584,#11585));
#1808=EDGE_LOOP('',(#11586,#11587,#11588,#11589));
#1809=EDGE_LOOP('',(#11590,#11591,#11592,#11593));
#1810=EDGE_LOOP('',(#11594,#11595,#11596,#11597));
#1811=EDGE_LOOP('',(#11598,#11599,#11600,#11601));
#1812=EDGE_LOOP('',(#11602,#11603,#11604,#11605));
#1813=EDGE_LOOP('',(#11606,#11607,#11608,#11609));
#1814=EDGE_LOOP('',(#11610,#11611,#11612,#11613));
#1815=EDGE_LOOP('',(#11614,#11615,#11616,#11617));
#1816=EDGE_LOOP('',(#11618,#11619,#11620,#11621));
#1817=EDGE_LOOP('',(#11622,#11623,#11624,#11625));
#1818=EDGE_LOOP('',(#11626,#11627,#11628,#11629));
#1819=EDGE_LOOP('',(#11630,#11631,#11632,#11633));
#1820=EDGE_LOOP('',(#11634,#11635,#11636,#11637));
#1821=EDGE_LOOP('',(#11638,#11639,#11640,#11641));
#1822=EDGE_LOOP('',(#11642,#11643,#11644,#11645,#11646,#11647,#11648,#11649));
#1823=EDGE_LOOP('',(#11650,#11651,#11652,#11653));
#1824=EDGE_LOOP('',(#11654,#11655,#11656,#11657));
#1825=EDGE_LOOP('',(#11658,#11659,#11660,#11661));
#1826=EDGE_LOOP('',(#11662,#11663,#11664,#11665));
#1827=EDGE_LOOP('',(#11666,#11667,#11668,#11669));
#1828=EDGE_LOOP('',(#11670,#11671,#11672,#11673));
#1829=EDGE_LOOP('',(#11674,#11675,#11676,#11677));
#1830=EDGE_LOOP('',(#11678,#11679,#11680,#11681));
#1831=EDGE_LOOP('',(#11682,#11683,#11684,#11685));
#1832=EDGE_LOOP('',(#11686,#11687,#11688,#11689));
#1833=EDGE_LOOP('',(#11690,#11691,#11692,#11693));
#1834=EDGE_LOOP('',(#11694,#11695,#11696,#11697));
#1835=EDGE_LOOP('',(#11698,#11699,#11700,#11701));
#1836=EDGE_LOOP('',(#11702,#11703,#11704,#11705));
#1837=EDGE_LOOP('',(#11706,#11707,#11708,#11709));
#1838=EDGE_LOOP('',(#11710,#11711,#11712,#11713));
#1839=EDGE_LOOP('',(#11714,#11715,#11716,#11717));
#1840=EDGE_LOOP('',(#11718,#11719,#11720,#11721));
#1841=EDGE_LOOP('',(#11722,#11723,#11724,#11725));
#1842=EDGE_LOOP('',(#11726,#11727,#11728,#11729));
#1843=EDGE_LOOP('',(#11730,#11731,#11732,#11733));
#1844=EDGE_LOOP('',(#11734,#11735,#11736,#11737));
#1845=EDGE_LOOP('',(#11738,#11739,#11740,#11741));
#1846=EDGE_LOOP('',(#11742,#11743,#11744,#11745));
#1847=EDGE_LOOP('',(#11746,#11747,#11748,#11749,#11750,#11751,#11752,#11753));
#1848=EDGE_LOOP('',(#11754,#11755,#11756,#11757));
#1849=EDGE_LOOP('',(#11758,#11759,#11760,#11761));
#1850=EDGE_LOOP('',(#11762,#11763,#11764,#11765));
#1851=EDGE_LOOP('',(#11766,#11767,#11768,#11769));
#1852=EDGE_LOOP('',(#11770,#11771,#11772,#11773));
#1853=EDGE_LOOP('',(#11774,#11775,#11776,#11777));
#1854=EDGE_LOOP('',(#11778,#11779,#11780,#11781));
#1855=EDGE_LOOP('',(#11782,#11783,#11784,#11785));
#1856=EDGE_LOOP('',(#11786,#11787,#11788,#11789));
#1857=EDGE_LOOP('',(#11790,#11791,#11792,#11793));
#1858=EDGE_LOOP('',(#11794,#11795,#11796,#11797));
#1859=EDGE_LOOP('',(#11798,#11799,#11800,#11801));
#1860=EDGE_LOOP('',(#11802,#11803,#11804,#11805));
#1861=EDGE_LOOP('',(#11806,#11807,#11808,#11809));
#1862=EDGE_LOOP('',(#11810,#11811,#11812,#11813));
#1863=EDGE_LOOP('',(#11814,#11815,#11816,#11817));
#1864=EDGE_LOOP('',(#11818,#11819,#11820,#11821));
#1865=EDGE_LOOP('',(#11822,#11823,#11824,#11825));
#1866=EDGE_LOOP('',(#11826,#11827,#11828,#11829));
#1867=EDGE_LOOP('',(#11830,#11831,#11832,#11833));
#1868=EDGE_LOOP('',(#11834,#11835,#11836,#11837));
#1869=EDGE_LOOP('',(#11838,#11839,#11840,#11841));
#1870=EDGE_LOOP('',(#11842,#11843,#11844,#11845));
#1871=EDGE_LOOP('',(#11846,#11847,#11848,#11849));
#1872=EDGE_LOOP('',(#11850,#11851,#11852,#11853,#11854,#11855,#11856,#11857));
#1873=EDGE_LOOP('',(#11858,#11859,#11860,#11861));
#1874=EDGE_LOOP('',(#11862,#11863,#11864,#11865));
#1875=EDGE_LOOP('',(#11866,#11867,#11868,#11869));
#1876=EDGE_LOOP('',(#11870,#11871,#11872,#11873));
#1877=EDGE_LOOP('',(#11874,#11875,#11876,#11877));
#1878=EDGE_LOOP('',(#11878,#11879,#11880,#11881));
#1879=EDGE_LOOP('',(#11882,#11883,#11884,#11885));
#1880=EDGE_LOOP('',(#11886,#11887,#11888,#11889));
#1881=EDGE_LOOP('',(#11890,#11891,#11892,#11893));
#1882=EDGE_LOOP('',(#11894,#11895,#11896,#11897));
#1883=EDGE_LOOP('',(#11898,#11899,#11900,#11901));
#1884=EDGE_LOOP('',(#11902,#11903,#11904,#11905));
#1885=EDGE_LOOP('',(#11906,#11907,#11908,#11909));
#1886=EDGE_LOOP('',(#11910,#11911,#11912,#11913));
#1887=EDGE_LOOP('',(#11914,#11915,#11916,#11917));
#1888=EDGE_LOOP('',(#11918,#11919,#11920,#11921));
#1889=EDGE_LOOP('',(#11922,#11923,#11924,#11925));
#1890=EDGE_LOOP('',(#11926,#11927,#11928,#11929));
#1891=EDGE_LOOP('',(#11930,#11931,#11932,#11933));
#1892=EDGE_LOOP('',(#11934,#11935,#11936,#11937));
#1893=EDGE_LOOP('',(#11938,#11939,#11940,#11941));
#1894=EDGE_LOOP('',(#11942,#11943,#11944,#11945));
#1895=EDGE_LOOP('',(#11946,#11947,#11948,#11949));
#1896=EDGE_LOOP('',(#11950,#11951,#11952,#11953));
#1897=EDGE_LOOP('',(#11954,#11955,#11956,#11957,#11958,#11959,#11960,#11961));
#1898=EDGE_LOOP('',(#11962,#11963,#11964,#11965));
#1899=EDGE_LOOP('',(#11966,#11967,#11968,#11969));
#1900=EDGE_LOOP('',(#11970,#11971,#11972,#11973));
#1901=EDGE_LOOP('',(#11974,#11975,#11976,#11977));
#1902=EDGE_LOOP('',(#11978,#11979,#11980,#11981));
#1903=EDGE_LOOP('',(#11982,#11983,#11984,#11985));
#1904=EDGE_LOOP('',(#11986,#11987,#11988,#11989));
#1905=EDGE_LOOP('',(#11990,#11991,#11992,#11993));
#1906=EDGE_LOOP('',(#11994,#11995,#11996,#11997));
#1907=EDGE_LOOP('',(#11998,#11999,#12000,#12001));
#1908=EDGE_LOOP('',(#12002,#12003,#12004,#12005));
#1909=EDGE_LOOP('',(#12006,#12007,#12008,#12009));
#1910=EDGE_LOOP('',(#12010,#12011,#12012,#12013));
#1911=EDGE_LOOP('',(#12014,#12015,#12016,#12017));
#1912=EDGE_LOOP('',(#12018,#12019,#12020,#12021));
#1913=EDGE_LOOP('',(#12022,#12023,#12024,#12025));
#1914=EDGE_LOOP('',(#12026,#12027,#12028,#12029));
#1915=EDGE_LOOP('',(#12030,#12031,#12032,#12033));
#1916=EDGE_LOOP('',(#12034,#12035,#12036,#12037));
#1917=EDGE_LOOP('',(#12038,#12039,#12040,#12041));
#1918=EDGE_LOOP('',(#12042,#12043,#12044,#12045));
#1919=EDGE_LOOP('',(#12046,#12047,#12048,#12049));
#1920=EDGE_LOOP('',(#12050,#12051,#12052,#12053));
#1921=EDGE_LOOP('',(#12054,#12055,#12056,#12057));
#1922=EDGE_LOOP('',(#12058,#12059,#12060,#12061,#12062,#12063,#12064,#12065));
#1923=EDGE_LOOP('',(#12066,#12067,#12068,#12069));
#1924=EDGE_LOOP('',(#12070,#12071,#12072,#12073));
#1925=EDGE_LOOP('',(#12074,#12075,#12076,#12077));
#1926=EDGE_LOOP('',(#12078,#12079,#12080,#12081));
#1927=EDGE_LOOP('',(#12082,#12083,#12084,#12085));
#1928=EDGE_LOOP('',(#12086,#12087,#12088,#12089));
#1929=EDGE_LOOP('',(#12090,#12091,#12092,#12093));
#1930=EDGE_LOOP('',(#12094,#12095,#12096,#12097));
#1931=EDGE_LOOP('',(#12098,#12099,#12100,#12101));
#1932=EDGE_LOOP('',(#12102,#12103,#12104,#12105));
#1933=EDGE_LOOP('',(#12106,#12107,#12108,#12109));
#1934=EDGE_LOOP('',(#12110,#12111,#12112,#12113));
#1935=EDGE_LOOP('',(#12114,#12115,#12116,#12117));
#1936=EDGE_LOOP('',(#12118,#12119,#12120,#12121));
#1937=EDGE_LOOP('',(#12122,#12123,#12124,#12125));
#1938=EDGE_LOOP('',(#12126,#12127,#12128,#12129));
#1939=EDGE_LOOP('',(#12130,#12131,#12132,#12133));
#1940=EDGE_LOOP('',(#12134,#12135,#12136,#12137));
#1941=EDGE_LOOP('',(#12138,#12139,#12140,#12141));
#1942=EDGE_LOOP('',(#12142,#12143,#12144,#12145));
#1943=EDGE_LOOP('',(#12146,#12147,#12148,#12149));
#1944=EDGE_LOOP('',(#12150,#12151,#12152,#12153));
#1945=EDGE_LOOP('',(#12154,#12155,#12156,#12157));
#1946=EDGE_LOOP('',(#12158,#12159,#12160,#12161));
#1947=EDGE_LOOP('',(#12162,#12163,#12164,#12165,#12166,#12167,#12168,#12169));
#1948=EDGE_LOOP('',(#12170,#12171,#12172,#12173));
#1949=EDGE_LOOP('',(#12174,#12175,#12176,#12177));
#1950=EDGE_LOOP('',(#12178,#12179,#12180,#12181));
#1951=EDGE_LOOP('',(#12182,#12183,#12184,#12185));
#1952=EDGE_LOOP('',(#12186,#12187,#12188,#12189));
#1953=EDGE_LOOP('',(#12190,#12191,#12192,#12193));
#1954=EDGE_LOOP('',(#12194,#12195,#12196,#12197));
#1955=EDGE_LOOP('',(#12198,#12199,#12200,#12201));
#1956=EDGE_LOOP('',(#12202,#12203,#12204,#12205));
#1957=EDGE_LOOP('',(#12206,#12207,#12208,#12209));
#1958=EDGE_LOOP('',(#12210,#12211,#12212,#12213));
#1959=EDGE_LOOP('',(#12214,#12215,#12216,#12217));
#1960=EDGE_LOOP('',(#12218,#12219,#12220,#12221));
#1961=EDGE_LOOP('',(#12222,#12223,#12224,#12225));
#1962=EDGE_LOOP('',(#12226,#12227,#12228,#12229));
#1963=EDGE_LOOP('',(#12230,#12231,#12232,#12233));
#1964=EDGE_LOOP('',(#12234,#12235,#12236,#12237));
#1965=EDGE_LOOP('',(#12238,#12239,#12240,#12241));
#1966=EDGE_LOOP('',(#12242,#12243,#12244,#12245));
#1967=EDGE_LOOP('',(#12246,#12247,#12248,#12249));
#1968=EDGE_LOOP('',(#12250,#12251,#12252,#12253));
#1969=EDGE_LOOP('',(#12254,#12255,#12256,#12257));
#1970=EDGE_LOOP('',(#12258,#12259,#12260,#12261));
#1971=EDGE_LOOP('',(#12262,#12263,#12264,#12265));
#1972=EDGE_LOOP('',(#12266,#12267,#12268,#12269));
#1973=EDGE_LOOP('',(#12270,#12271,#12272,#12273));
#1974=EDGE_LOOP('',(#12274,#12275,#12276,#12277));
#1975=EDGE_LOOP('',(#12278,#12279,#12280,#12281));
#1976=EDGE_LOOP('',(#12282,#12283,#12284,#12285));
#1977=EDGE_LOOP('',(#12286,#12287,#12288,#12289));
#1978=EDGE_LOOP('',(#12290,#12291,#12292,#12293));
#1979=EDGE_LOOP('',(#12294,#12295,#12296,#12297));
#1980=EDGE_LOOP('',(#12298,#12299,#12300,#12301));
#1981=EDGE_LOOP('',(#12302,#12303,#12304,#12305));
#1982=EDGE_LOOP('',(#12306,#12307,#12308,#12309));
#1983=EDGE_LOOP('',(#12310,#12311,#12312,#12313));
#1984=EDGE_LOOP('',(#12314,#12315,#12316,#12317));
#1985=EDGE_LOOP('',(#12318,#12319,#12320,#12321));
#1986=EDGE_LOOP('',(#12322,#12323,#12324,#12325));
#1987=EDGE_LOOP('',(#12326,#12327,#12328,#12329,#12330));
#1988=EDGE_LOOP('',(#12331,#12332,#12333,#12334));
#1989=EDGE_LOOP('',(#12335,#12336,#12337,#12338));
#1990=EDGE_LOOP('',(#12339,#12340,#12341,#12342));
#1991=EDGE_LOOP('',(#12343,#12344,#12345,#12346));
#1992=EDGE_LOOP('',(#12347,#12348,#12349,#12350));
#1993=EDGE_LOOP('',(#12351,#12352,#12353,#12354));
#1994=EDGE_LOOP('',(#12355,#12356,#12357,#12358));
#1995=EDGE_LOOP('',(#12359,#12360,#12361,#12362));
#1996=EDGE_LOOP('',(#12363,#12364,#12365,#12366));
#1997=EDGE_LOOP('',(#12367,#12368,#12369,#12370));
#1998=EDGE_LOOP('',(#12371,#12372,#12373,#12374));
#1999=EDGE_LOOP('',(#12375,#12376,#12377,#12378));
#2000=EDGE_LOOP('',(#12379,#12380,#12381,#12382));
#2001=EDGE_LOOP('',(#12383,#12384,#12385,#12386));
#2002=EDGE_LOOP('',(#12387,#12388,#12389,#12390));
#2003=EDGE_LOOP('',(#12391,#12392,#12393,#12394));
#2004=EDGE_LOOP('',(#12395,#12396,#12397,#12398));
#2005=EDGE_LOOP('',(#12399,#12400,#12401,#12402));
#2006=EDGE_LOOP('',(#12403,#12404,#12405,#12406));
#2007=EDGE_LOOP('',(#12407,#12408,#12409,#12410));
#2008=EDGE_LOOP('',(#12411,#12412,#12413,#12414));
#2009=EDGE_LOOP('',(#12415,#12416,#12417,#12418));
#2010=EDGE_LOOP('',(#12419,#12420,#12421,#12422));
#2011=EDGE_LOOP('',(#12423,#12424,#12425,#12426));
#2012=EDGE_LOOP('',(#12427,#12428,#12429,#12430));
#2013=EDGE_LOOP('',(#12431,#12432,#12433,#12434));
#2014=EDGE_LOOP('',(#12435,#12436,#12437,#12438));
#2015=EDGE_LOOP('',(#12439,#12440,#12441,#12442));
#2016=EDGE_LOOP('',(#12443,#12444,#12445,#12446));
#2017=EDGE_LOOP('',(#12447,#12448,#12449,#12450));
#2018=EDGE_LOOP('',(#12451,#12452,#12453,#12454));
#2019=EDGE_LOOP('',(#12455,#12456,#12457,#12458,#12459));
#2020=EDGE_LOOP('',(#12460,#12461,#12462,#12463));
#2021=EDGE_LOOP('',(#12464,#12465,#12466,#12467));
#2022=EDGE_LOOP('',(#12468,#12469,#12470,#12471));
#2023=EDGE_LOOP('',(#12472,#12473,#12474,#12475));
#2024=EDGE_LOOP('',(#12476,#12477,#12478,#12479));
#2025=EDGE_LOOP('',(#12480,#12481,#12482,#12483));
#2026=EDGE_LOOP('',(#12484,#12485,#12486,#12487));
#2027=EDGE_LOOP('',(#12488,#12489,#12490,#12491,#12492));
#2028=EDGE_LOOP('',(#12493,#12494,#12495,#12496));
#2029=EDGE_LOOP('',(#12497,#12498,#12499,#12500));
#2030=EDGE_LOOP('',(#12501,#12502,#12503,#12504));
#2031=EDGE_LOOP('',(#12505,#12506,#12507,#12508));
#2032=EDGE_LOOP('',(#12509,#12510,#12511,#12512));
#2033=EDGE_LOOP('',(#12513,#12514,#12515,#12516));
#2034=EDGE_LOOP('',(#12517,#12518,#12519,#12520));
#2035=EDGE_LOOP('',(#12521,#12522,#12523,#12524,#12525));
#2036=EDGE_LOOP('',(#12526,#12527,#12528,#12529,#12530,#12531,#12532,#12533,
#12534,#12535,#12536,#12537,#12538,#12539,#12540,#12541,#12542,#12543,#12544,
#12545));
#2037=EDGE_LOOP('',(#12546,#12547,#12548,#12549));
#2038=EDGE_LOOP('',(#12550,#12551,#12552,#12553,#12554,#12555,#12556,#12557,
#12558,#12559,#12560,#12561,#12562,#12563,#12564,#12565,#12566,#12567,#12568,
#12569));
#2039=EDGE_LOOP('',(#12570,#12571,#12572,#12573,#12574,#12575,#12576,#12577,
#12578,#12579,#12580,#12581,#12582,#12583,#12584,#12585,#12586,#12587,#12588,
#12589));
#2040=EDGE_LOOP('',(#12590,#12591,#12592,#12593));
#2041=EDGE_LOOP('',(#12594,#12595,#12596,#12597,#12598,#12599,#12600,#12601,
#12602,#12603,#12604,#12605,#12606,#12607,#12608,#12609,#12610,#12611,#12612,
#12613));
#2042=EDGE_LOOP('',(#12614,#12615,#12616,#12617,#12618,#12619,#12620,#12621,
#12622,#12623,#12624,#12625,#12626,#12627,#12628,#12629,#12630,#12631,#12632,
#12633));
#2043=EDGE_LOOP('',(#12634,#12635,#12636,#12637));
#2044=EDGE_LOOP('',(#12638,#12639,#12640,#12641,#12642,#12643,#12644,#12645,
#12646,#12647,#12648,#12649,#12650,#12651,#12652,#12653,#12654,#12655,#12656,
#12657));
#2045=EDGE_LOOP('',(#12658,#12659,#12660,#12661));
#2046=EDGE_LOOP('',(#12662,#12663,#12664,#12665));
#2047=EDGE_LOOP('',(#12666,#12667,#12668,#12669));
#2048=EDGE_LOOP('',(#12670,#12671,#12672,#12673));
#2049=EDGE_LOOP('',(#12674,#12675,#12676,#12677));
#2050=EDGE_LOOP('',(#12678,#12679,#12680,#12681));
#2051=EDGE_LOOP('',(#12682,#12683,#12684,#12685,#12686,#12687,#12688,#12689,
#12690,#12691,#12692,#12693,#12694,#12695,#12696,#12697,#12698,#12699,#12700,
#12701));
#2052=EDGE_LOOP('',(#12702,#12703,#12704,#12705));
#2053=EDGE_LOOP('',(#12706,#12707,#12708,#12709,#12710,#12711,#12712,#12713,
#12714,#12715,#12716,#12717,#12718,#12719,#12720,#12721,#12722,#12723,#12724,
#12725));
#2054=EDGE_LOOP('',(#12726,#12727,#12728,#12729));
#2055=EDGE_LOOP('',(#12730,#12731,#12732,#12733));
#2056=EDGE_LOOP('',(#12734,#12735,#12736,#12737));
#2057=EDGE_LOOP('',(#12738,#12739,#12740,#12741));
#2058=EDGE_LOOP('',(#12742,#12743,#12744,#12745,#12746,#12747,#12748,#12749,
#12750,#12751,#12752,#12753,#12754,#12755,#12756,#12757,#12758,#12759,#12760,
#12761,#12762,#12763,#12764,#12765,#12766,#12767,#12768,#12769,#12770,#12771));
#2059=EDGE_LOOP('',(#12772,#12773,#12774,#12775,#12776,#12777,#12778,#12779,
#12780,#12781,#12782,#12783,#12784,#12785,#12786,#12787,#12788,#12789,#12790,
#12791,#12792,#12793,#12794,#12795,#12796,#12797,#12798,#12799,#12800));
#2060=EDGE_LOOP('',(#12801,#12802,#12803,#12804));
#2061=EDGE_LOOP('',(#12805,#12806,#12807,#12808));
#2062=EDGE_LOOP('',(#12809,#12810,#12811,#12812));
#2063=EDGE_LOOP('',(#12813,#12814,#12815,#12816,#12817,#12818,#12819,#12820,
#12821,#12822,#12823,#12824,#12825,#12826,#12827,#12828,#12829,#12830,#12831,
#12832,#12833,#12834,#12835,#12836,#12837,#12838,#12839,#12840,#12841,#12842));
#2064=EDGE_LOOP('',(#12843,#12844,#12845,#12846,#12847,#12848,#12849,#12850,
#12851,#12852,#12853,#12854,#12855,#12856,#12857,#12858,#12859,#12860,#12861,
#12862,#12863,#12864,#12865,#12866,#12867,#12868,#12869,#12870,#12871));
#2065=EDGE_LOOP('',(#12872,#12873,#12874,#12875));
#2066=EDGE_LOOP('',(#12876,#12877,#12878,#12879));
#2067=EDGE_LOOP('',(#12880,#12881,#12882,#12883));
#2068=EDGE_LOOP('',(#12884,#12885,#12886,#12887,#12888,#12889,#12890,#12891,
#12892,#12893,#12894,#12895,#12896,#12897,#12898,#12899,#12900,#12901,#12902,
#12903,#12904,#12905,#12906,#12907,#12908,#12909,#12910,#12911,#12912,#12913));
#2069=EDGE_LOOP('',(#12914,#12915,#12916,#12917,#12918,#12919,#12920,#12921,
#12922,#12923,#12924,#12925,#12926,#12927,#12928,#12929,#12930,#12931,#12932,
#12933,#12934,#12935,#12936,#12937,#12938,#12939,#12940,#12941,#12942));
#2070=EDGE_LOOP('',(#12943,#12944,#12945,#12946));
#2071=EDGE_LOOP('',(#12947,#12948,#12949,#12950));
#2072=EDGE_LOOP('',(#12951,#12952,#12953,#12954));
#2073=EDGE_LOOP('',(#12955,#12956,#12957,#12958,#12959,#12960,#12961,#12962,
#12963,#12964,#12965,#12966,#12967,#12968,#12969,#12970,#12971,#12972,#12973,
#12974,#12975,#12976,#12977,#12978,#12979,#12980,#12981,#12982,#12983,#12984));
#2074=EDGE_LOOP('',(#12985,#12986,#12987,#12988,#12989,#12990,#12991,#12992,
#12993,#12994,#12995,#12996,#12997,#12998,#12999,#13000,#13001,#13002,#13003,
#13004,#13005,#13006,#13007,#13008,#13009,#13010,#13011,#13012,#13013));
#2075=EDGE_LOOP('',(#13014,#13015,#13016,#13017));
#2076=EDGE_LOOP('',(#13018,#13019,#13020,#13021));
#2077=EDGE_LOOP('',(#13022,#13023,#13024,#13025));
#2078=EDGE_LOOP('',(#13026,#13027,#13028,#13029,#13030,#13031,#13032,#13033,
#13034,#13035,#13036,#13037,#13038,#13039,#13040,#13041,#13042,#13043,#13044,
#13045,#13046,#13047,#13048,#13049,#13050,#13051,#13052,#13053,#13054,#13055));
#2079=EDGE_LOOP('',(#13056,#13057,#13058,#13059,#13060,#13061,#13062,#13063,
#13064,#13065,#13066,#13067,#13068,#13069,#13070,#13071,#13072,#13073,#13074,
#13075,#13076,#13077,#13078,#13079,#13080,#13081,#13082,#13083,#13084));
#2080=EDGE_LOOP('',(#13085,#13086,#13087,#13088));
#2081=EDGE_LOOP('',(#13089));
#2082=EDGE_LOOP('',(#13090));
#2083=EDGE_LOOP('',(#13091));
#2084=EDGE_LOOP('',(#13092));
#2085=EDGE_LOOP('',(#13093));
#2086=EDGE_LOOP('',(#13094,#13095,#13096,#13097));
#2087=EDGE_LOOP('',(#13098,#13099,#13100,#13101));
#2088=EDGE_LOOP('',(#13102,#13103,#13104,#13105,#13106,#13107,#13108,#13109,
#13110,#13111,#13112,#13113,#13114,#13115,#13116,#13117,#13118,#13119,#13120,
#13121,#13122,#13123,#13124,#13125,#13126,#13127,#13128,#13129,#13130,#13131));
#2089=EDGE_LOOP('',(#13132,#13133,#13134,#13135,#13136,#13137,#13138,#13139,
#13140,#13141,#13142,#13143,#13144,#13145,#13146,#13147,#13148,#13149,#13150,
#13151,#13152,#13153,#13154,#13155,#13156,#13157,#13158,#13159,#13160));
#2090=EDGE_LOOP('',(#13161,#13162,#13163,#13164));
#2091=EDGE_LOOP('',(#13165,#13166,#13167,#13168));
#2092=EDGE_LOOP('',(#13169,#13170,#13171,#13172));
#2093=EDGE_LOOP('',(#13173,#13174,#13175,#13176,#13177,#13178,#13179,#13180,
#13181,#13182,#13183,#13184,#13185,#13186,#13187,#13188,#13189,#13190,#13191,
#13192,#13193,#13194,#13195,#13196,#13197,#13198,#13199,#13200,#13201,#13202));
#2094=EDGE_LOOP('',(#13203,#13204,#13205,#13206,#13207,#13208,#13209,#13210,
#13211,#13212,#13213,#13214,#13215,#13216,#13217,#13218,#13219,#13220,#13221,
#13222,#13223,#13224,#13225,#13226,#13227,#13228,#13229,#13230,#13231));
#2095=EDGE_LOOP('',(#13232,#13233,#13234,#13235));
#2096=EDGE_LOOP('',(#13236,#13237,#13238,#13239));
#2097=EDGE_LOOP('',(#13240,#13241,#13242,#13243));
#2098=EDGE_LOOP('',(#13244,#13245,#13246,#13247,#13248,#13249,#13250,#13251,
#13252,#13253,#13254,#13255,#13256,#13257,#13258,#13259,#13260,#13261,#13262,
#13263,#13264,#13265,#13266,#13267,#13268,#13269,#13270,#13271,#13272,#13273));
#2099=EDGE_LOOP('',(#13274,#13275,#13276,#13277,#13278,#13279,#13280,#13281,
#13282,#13283,#13284,#13285,#13286,#13287,#13288,#13289,#13290,#13291,#13292,
#13293,#13294,#13295,#13296,#13297,#13298,#13299,#13300,#13301,#13302));
#2100=EDGE_LOOP('',(#13303,#13304,#13305,#13306));
#2101=EDGE_LOOP('',(#13307,#13308,#13309,#13310));
#2102=EDGE_LOOP('',(#13311,#13312,#13313,#13314));
#2103=EDGE_LOOP('',(#13315,#13316,#13317,#13318,#13319,#13320,#13321,#13322,
#13323,#13324,#13325,#13326,#13327,#13328,#13329,#13330,#13331,#13332,#13333,
#13334,#13335,#13336,#13337,#13338,#13339,#13340,#13341,#13342,#13343,#13344));
#2104=EDGE_LOOP('',(#13345,#13346,#13347,#13348,#13349,#13350,#13351,#13352,
#13353,#13354,#13355,#13356,#13357,#13358,#13359,#13360,#13361,#13362,#13363,
#13364,#13365,#13366,#13367,#13368,#13369,#13370,#13371,#13372,#13373));
#2105=EDGE_LOOP('',(#13374,#13375,#13376,#13377));
#2106=EDGE_LOOP('',(#13378,#13379,#13380,#13381));
#2107=EDGE_LOOP('',(#13382,#13383,#13384,#13385));
#2108=EDGE_LOOP('',(#13386,#13387,#13388,#13389,#13390,#13391,#13392,#13393,
#13394,#13395,#13396,#13397,#13398,#13399,#13400,#13401,#13402,#13403,#13404,
#13405,#13406,#13407,#13408,#13409,#13410,#13411,#13412,#13413,#13414,#13415));
#2109=EDGE_LOOP('',(#13416,#13417,#13418,#13419,#13420,#13421,#13422,#13423,
#13424,#13425,#13426,#13427,#13428,#13429,#13430,#13431,#13432,#13433,#13434,
#13435,#13436,#13437,#13438,#13439,#13440,#13441,#13442,#13443,#13444));
#2110=EDGE_LOOP('',(#13445,#13446,#13447,#13448));
#2111=EDGE_LOOP('',(#13449));
#2112=EDGE_LOOP('',(#13450));
#2113=EDGE_LOOP('',(#13451));
#2114=EDGE_LOOP('',(#13452));
#2115=EDGE_LOOP('',(#13453));
#2116=EDGE_LOOP('',(#13454,#13455,#13456,#13457));
#2117=EDGE_LOOP('',(#13458,#13459,#13460,#13461));
#2118=EDGE_LOOP('',(#13462,#13463,#13464,#13465,#13466,#13467,#13468,#13469,
#13470,#13471,#13472,#13473,#13474,#13475,#13476,#13477,#13478,#13479,#13480,
#13481,#13482,#13483,#13484,#13485,#13486,#13487,#13488,#13489,#13490,#13491));
#2119=EDGE_LOOP('',(#13492,#13493,#13494,#13495,#13496,#13497,#13498,#13499,
#13500,#13501,#13502,#13503,#13504,#13505,#13506,#13507,#13508,#13509,#13510,
#13511,#13512,#13513,#13514,#13515,#13516,#13517,#13518,#13519,#13520));
#2120=EDGE_LOOP('',(#13521,#13522,#13523,#13524));
#2121=EDGE_LOOP('',(#13525));
#2122=EDGE_LOOP('',(#13526,#13527,#13528,#13529));
#2123=EDGE_LOOP('',(#13530,#13531,#13532,#13533));
#2124=EDGE_LOOP('',(#13534,#13535,#13536,#13537,#13538,#13539,#13540,#13541,
#13542,#13543,#13544,#13545,#13546,#13547,#13548,#13549,#13550,#13551,#13552,
#13553,#13554,#13555,#13556,#13557,#13558,#13559,#13560,#13561,#13562,#13563));
#2125=EDGE_LOOP('',(#13564,#13565,#13566,#13567,#13568,#13569,#13570,#13571,
#13572,#13573,#13574,#13575,#13576,#13577,#13578,#13579,#13580,#13581,#13582,
#13583,#13584,#13585,#13586,#13587,#13588,#13589,#13590,#13591,#13592));
#2126=EDGE_LOOP('',(#13593,#13594,#13595,#13596));
#2127=EDGE_LOOP('',(#13597));
#2128=EDGE_LOOP('',(#13598,#13599,#13600,#13601));
#2129=EDGE_LOOP('',(#13602,#13603,#13604,#13605));
#2130=EDGE_LOOP('',(#13606,#13607,#13608,#13609,#13610));
#2131=EDGE_LOOP('',(#13611,#13612,#13613,#13614,#13615));
#2132=EDGE_LOOP('',(#13616,#13617,#13618,#13619,#13620));
#2133=EDGE_LOOP('',(#13621,#13622,#13623,#13624,#13625));
#2134=EDGE_LOOP('',(#13626));
#2135=EDGE_LOOP('',(#13627,#13628,#13629,#13630));
#2136=EDGE_LOOP('',(#13631,#13632,#13633,#13634));
#2137=EDGE_LOOP('',(#13635,#13636,#13637,#13638));
#2138=EDGE_LOOP('',(#13639,#13640,#13641,#13642));
#2139=EDGE_LOOP('',(#13643,#13644,#13645,#13646));
#2140=EDGE_LOOP('',(#13647));
#2141=EDGE_LOOP('',(#13648,#13649,#13650,#13651));
#2142=EDGE_LOOP('',(#13652));
#2143=EDGE_LOOP('',(#13653,#13654,#13655,#13656));
#2144=EDGE_LOOP('',(#13657,#13658,#13659,#13660));
#2145=EDGE_LOOP('',(#13661,#13662,#13663,#13664));
#2146=EDGE_LOOP('',(#13665,#13666,#13667,#13668));
#2147=EDGE_LOOP('',(#13669,#13670,#13671,#13672));
#2148=EDGE_LOOP('',(#13673));
#2149=EDGE_LOOP('',(#13674,#13675,#13676,#13677));
#2777=CIRCLE('',#18466,1.666);
#2778=CIRCLE('',#18467,1.666);
#2779=CIRCLE('',#18479,1.666);
#2780=CIRCLE('',#18481,2.05475);
#2781=CIRCLE('',#18494,2.05475);
#2782=CIRCLE('',#18496,1.666);
#2783=CIRCLE('',#18497,1.666);
#2784=CIRCLE('',#18509,1.666);
#2785=CIRCLE('',#18511,2.05475);
#2786=CIRCLE('',#18524,2.05475);
#2787=CIRCLE('',#18526,1.666);
#2788=CIRCLE('',#18527,1.666);
#2789=CIRCLE('',#18539,1.666);
#2790=CIRCLE('',#18541,2.05475);
#2791=CIRCLE('',#18554,2.05475);
#2792=CIRCLE('',#18556,1.666);
#2793=CIRCLE('',#18557,1.666);
#2794=CIRCLE('',#18569,1.666);
#2795=CIRCLE('',#18571,2.05474999999998);
#2796=CIRCLE('',#18584,2.05474999999998);
#2797=CIRCLE('',#18586,1.666);
#2798=CIRCLE('',#18587,1.666);
#2799=CIRCLE('',#18599,1.666);
#2800=CIRCLE('',#18601,2.05475);
#2801=CIRCLE('',#18614,2.05475);
#2802=CIRCLE('',#18616,1.666);
#2803=CIRCLE('',#18617,1.666);
#2804=CIRCLE('',#18629,1.666);
#2805=CIRCLE('',#18631,2.05474999999998);
#2806=CIRCLE('',#18644,2.05474999999998);
#2807=CIRCLE('',#18646,1.666);
#2808=CIRCLE('',#18647,1.666);
#2809=CIRCLE('',#18659,1.666);
#2810=CIRCLE('',#18661,2.05474999999998);
#2811=CIRCLE('',#18674,2.05474999999998);
#2812=CIRCLE('',#18676,1.666);
#2813=CIRCLE('',#18677,1.666);
#2814=CIRCLE('',#18689,1.666);
#2815=CIRCLE('',#18691,2.05475000000002);
#2816=CIRCLE('',#18704,2.05475000000002);
#2817=CIRCLE('',#18706,1.666);
#2818=CIRCLE('',#18707,1.666);
#2819=CIRCLE('',#18719,1.666);
#2820=CIRCLE('',#18721,2.05474999999998);
#2821=CIRCLE('',#18734,2.05474999999998);
#2822=CIRCLE('',#18736,1.666);
#2823=CIRCLE('',#18737,1.666);
#2824=CIRCLE('',#18749,1.666);
#2825=CIRCLE('',#18751,2.05475);
#2826=CIRCLE('',#18764,2.05475);
#2827=CIRCLE('',#18766,1.666);
#2828=CIRCLE('',#18767,1.666);
#2829=CIRCLE('',#18779,1.666);
#2830=CIRCLE('',#18781,2.05474999999999);
#2831=CIRCLE('',#18794,2.05474999999999);
#2832=CIRCLE('',#18796,1.666);
#2833=CIRCLE('',#18797,1.666);
#2834=CIRCLE('',#18809,1.666);
#2835=CIRCLE('',#18811,2.05475);
#2836=CIRCLE('',#18824,2.05475);
#2837=CIRCLE('',#18826,2.5175);
#2838=CIRCLE('',#18835,3.07350000000007);
#2839=CIRCLE('',#18844,2.5175);
#2840=CIRCLE('',#18853,2.5175);
#2841=CIRCLE('',#18862,2.5175);
#2842=CIRCLE('',#18871,3.07350000000007);
#2843=CIRCLE('',#18880,3.07350000000007);
#2844=CIRCLE('',#18889,3.07350000000007);
#2845=CIRCLE('',#18958,60.);
#2846=CIRCLE('',#18959,60.);
#2847=CIRCLE('',#18961,70.);
#2848=CIRCLE('',#18962,70.);
#3113=B_SPLINE_CURVE_WITH_KNOTS('',3,(#23382,#23383,#23384,#23385,#23386,
#23387,#23388,#23389,#23390,#23391,#23392,#23393,#23394,#23395,#23396,#23397,
#23398,#23399,#23400,#23401,#23402,#23403),.UNSPECIFIED.,.F.,.F.,(4,3,3,
3,3,3,3,4),(76.708045941327,76.8129957196858,77.8105670926687,78.8081384656517,
79.8057098386346,80.8032812116175,81.8008525846005,82.7984239575834),
 .UNSPECIFIED.);
#3114=B_SPLINE_CURVE_WITH_KNOTS('',3,(#23407,#23408,#23409,#23410,#23411,
#23412,#23413),.UNSPECIFIED.,.F.,.F.,(4,3,4),(-80.7838110923089,-79.8057098386346,
-79.2446069498474),.UNSPECIFIED.);
#3115=B_SPLINE_CURVE_WITH_KNOTS('',3,(#23417,#23418,#23419,#23420,#23421,
#23422,#23423,#23424,#23425,#23426,#23427,#23428,#23429,#23430,#23431,#23432,
#23433,#23434,#23435,#23436,#23437,#23438),.UNSPECIFIED.,.F.,.F.,(4,3,3,
3,3,3,3,4),(-79.2446069498474,-78.8081384656517,-77.8105670926687,-76.8129957196858,
-75.8154243467029,-74.8178529737199,-73.820281600737,-72.9614216426678),
 .UNSPECIFIED.);
#3116=B_SPLINE_CURVE_WITH_KNOTS('',3,(#23443,#23444,#23445,#23446,#23447,
#23448,#23449,#23450,#23451,#23452,#23453,#23454,#23455,#23456,#23457,#23458,
#23459,#23460,#23461,#23462,#23463,#23464),.UNSPECIFIED.,.F.,.F.,(4,3,3,
3,3,3,3,4),(70.4248606341474,70.8275674817882,71.8251388547711,72.8227102277541,
73.820281600737,74.8178529737199,75.8154243467029,76.708045941327),
 .UNSPECIFIED.);
#3117=B_SPLINE_CURVE_WITH_KNOTS('',3,(#23465,#23466,#23467,#23468,#23469,
#23470,#23471,#23472,#23473,#23474,#23475,#23476,#23477,#23478,#23479,#23480,
#23481,#23482,#23483,#23484,#23485,#23486,#23487,#23488,#23489),
 .UNSPECIFIED.,.F.,.F.,(4,3,3,3,3,3,3,3,4),(-72.9614216426678,-72.8227102277541,
-71.8251388547712,-70.8275674817882,-69.8299961088053,-68.8324247358223,
-67.8348533628394,-66.8372819898565,-66.6782363354882),.UNSPECIFIED.);
#3118=B_SPLINE_CURVE_WITH_KNOTS('',3,(#23494,#23495,#23496,#23497,#23498,
#23499,#23500,#23501,#23502,#23503,#23504,#23505,#23506,#23507,#23508,#23509,
#23510,#23511,#23512,#23513,#23514,#23515),.UNSPECIFIED.,.F.,.F.,(4,3,3,
3,3,3,3,4),(64.1416753269678,64.8421392438906,65.8397106168735,66.8372819898565,
67.8348533628394,68.8324247358223,69.8299961088053,70.4248606341474),
 .UNSPECIFIED.);
#3119=B_SPLINE_CURVE_WITH_KNOTS('',3,(#23516,#23517,#23518,#23519,#23520,
#23521,#23522,#23523,#23524,#23525,#23526,#23527,#23528,#23529,#23530,#23531,
#23532,#23533,#23534,#23535,#23536,#23537),.UNSPECIFIED.,.F.,.F.,(4,3,3,
3,3,3,3,4),(-66.6782363354882,-65.8397106168735,-64.8421392438906,-63.8445678709077,
-62.8469964979248,-61.8494251249418,-60.8518537519589,-60.3950510283086),
 .UNSPECIFIED.);
#3120=B_SPLINE_CURVE_WITH_KNOTS('',3,(#23542,#23543,#23544,#23545,#23546,
#23547,#23548,#23549,#23550,#23551,#23552,#23553,#23554,#23555,#23556,#23557,
#23558,#23559,#23560,#23561,#23562,#23563),.UNSPECIFIED.,.F.,.F.,(4,3,3,
3,3,3,3,4),(57.8584900197882,58.856711005993,59.854282378976,60.8518537519589,
61.8494251249418,62.8469964979247,63.8445678709077,64.1416753269678),
 .UNSPECIFIED.);
#3121=B_SPLINE_CURVE_WITH_KNOTS('',3,(#23564,#23565,#23566,#23567,#23568,
#23569,#23570,#23571,#23572,#23573,#23574,#23575,#23576,#23577,#23578,#23579,
#23580,#23581,#23582,#23583,#23584,#23585),.UNSPECIFIED.,.F.,.F.,(4,3,3,
3,3,3,3,4),(-60.3950510283086,-59.854282378976,-58.856711005993,-57.8591396330101,
-56.8615682600271,-55.8639968870442,-54.8664255140613,-54.111865721129),
 .UNSPECIFIED.);
#3122=B_SPLINE_CURVE_WITH_KNOTS('',3,(#23590,#23591,#23592,#23593,#23594,
#23595,#23596,#23597,#23598,#23599,#23600,#23601,#23602,#23603,#23604,#23605,
#23606,#23607,#23608,#23609,#23610,#23611),.UNSPECIFIED.,.F.,.F.,(4,3,3,
3,3,3,3,4),(51.5753047126087,51.8737113951125,52.8712827680954,53.8688541410784,
54.8664255140613,55.8639968870442,56.8615682600272,57.8584900197882),
 .UNSPECIFIED.);
#3123=B_SPLINE_CURVE_WITH_KNOTS('',3,(#23612,#23613,#23614,#23615,#23616,
#23617,#23618,#23619,#23620,#23621,#23622,#23623,#23624,#23625,#23626,#23627,
#23628,#23629,#23630,#23631,#23632,#23633,#23634,#23635,#23636),
 .UNSPECIFIED.,.F.,.F.,(4,3,3,3,3,3,3,3,4),(-54.111865721129,-53.8688541410783,
-52.8712827680954,-51.8737113951125,-50.8761400221296,-49.8785686491466,
-48.8809972761637,-47.8834259031808,-47.8286804139494),.UNSPECIFIED.);
#3124=B_SPLINE_CURVE_WITH_KNOTS('',3,(#23641,#23642,#23643,#23644,#23645,
#23646,#23647,#23648,#23649,#23650,#23651,#23652,#23653,#23654,#23655,#23656,
#23657,#23658,#23659,#23660,#23661,#23662),.UNSPECIFIED.,.F.,.F.,(4,3,3,
3,3,3,3,4),(45.2921194054291,45.8882831572149,46.8858545301978,47.8834259031808,
48.8809972761637,49.8785686491466,50.8761400221296,51.5753047126087),
 .UNSPECIFIED.);
#3125=B_SPLINE_CURVE_WITH_KNOTS('',3,(#23663,#23664,#23665,#23666,#23667,
#23668,#23669,#23670,#23671,#23672,#23673,#23674,#23675,#23676,#23677,#23678,
#23679,#23680,#23681,#23682,#23683,#23684),.UNSPECIFIED.,.F.,.F.,(4,3,3,
3,3,3,3,4),(-47.8286804139494,-46.8858545301978,-45.8882831572149,-44.890711784232,
-43.893140411249,-42.8955690382661,-41.8979976652832,-41.5454951067698),
 .UNSPECIFIED.);
#3126=B_SPLINE_CURVE_WITH_KNOTS('',3,(#23689,#23690,#23691,#23692,#23693,
#23694,#23695,#23696,#23697,#23698,#23699,#23700,#23701,#23702,#23703,#23704,
#23705,#23706,#23707,#23708,#23709,#23710),.UNSPECIFIED.,.F.,.F.,(4,3,3,
3,3,3,3,4),(39.0089340982495,39.9028549193173,40.9004262923002,41.8979976652832,
42.8955690382661,43.893140411249,44.890711784232,45.2921194054291),
 .UNSPECIFIED.);
#3127=B_SPLINE_CURVE_WITH_KNOTS('',3,(#23711,#23712,#23713,#23714,#23715,
#23716,#23717,#23718,#23719,#23720,#23721,#23722,#23723,#23724,#23725,#23726,
#23727,#23728,#23729,#23730,#23731,#23732),.UNSPECIFIED.,.F.,.F.,(4,3,3,
3,3,3,3,4),(-41.5454951067698,-40.9004262923002,-39.9028549193173,-38.9052835463344,
-37.9077121733514,-36.9101408003685,-35.9125694273856,-35.2623097995902),
 .UNSPECIFIED.);
#3128=B_SPLINE_CURVE_WITH_KNOTS('',3,(#23737,#23738,#23739,#23740,#23741,
#23742,#23743,#23744,#23745,#23746,#23747,#23748,#23749,#23750,#23751,#23752,
#23753,#23754,#23755,#23756,#23757,#23758,#23759,#23760,#23761),
 .UNSPECIFIED.,.F.,.F.,(4,3,3,3,3,3,3,3,4),(32.7257487910699,32.9198553084368,
33.9174266814197,34.9149980544026,35.9125694273856,36.9101408003685,37.9077121733514,
38.9052835463344,39.0089340982495),.UNSPECIFIED.);
#3129=B_SPLINE_CURVE_WITH_KNOTS('',3,(#23762,#23763,#23764,#23765,#23766,
#23767,#23768,#23769,#23770,#23771,#23772,#23773,#23774,#23775,#23776,#23777,
#23778,#23779,#23780,#23781,#23782,#23783),.UNSPECIFIED.,.F.,.F.,(4,3,3,
3,3,3,3,4),(-35.2623097995902,-34.9149980544026,-33.9174266814197,-32.9198553084368,
-31.9222839354538,-30.9247125624709,-29.927141189488,-28.9791244924106),
 .UNSPECIFIED.);
#3130=B_SPLINE_CURVE_WITH_KNOTS('',3,(#23788,#23789,#23790,#23791,#23792,
#23793,#23794,#23795,#23796,#23797,#23798,#23799,#23800,#23801,#23802,#23803,
#23804,#23805,#23806,#23807,#23808,#23809),.UNSPECIFIED.,.F.,.F.,(4,3,3,
3,3,3,3,4),(26.4425634838903,26.9344270705392,27.9319984435221,28.929569816505,
29.927141189488,30.9247125624709,31.9222839354538,32.7257487910699),
 .UNSPECIFIED.);
#3131=B_SPLINE_CURVE_WITH_KNOTS('',3,(#23810,#23811,#23812,#23813,#23814,
#23815,#23816,#23817,#23818,#23819,#23820,#23821,#23822,#23823,#23824,#23825,
#23826,#23827,#23828,#23829,#23830,#23831,#23832,#23833,#23834),
 .UNSPECIFIED.,.F.,.F.,(4,3,3,3,3,3,3,3,4),(-28.9791244924106,-28.929569816505,
-27.9319984435221,-26.9344270705392,-25.9368556975563,-24.9392843245733,
-23.9417129515904,-22.9441415786074,-22.695939185231),.UNSPECIFIED.);
#3132=B_SPLINE_CURVE_WITH_KNOTS('',3,(#23839,#23840,#23841,#23842,#23843,
#23844,#23845,#23846,#23847,#23848,#23849,#23850,#23851,#23852,#23853,#23854,
#23855,#23856,#23857,#23858,#23859,#23860),.UNSPECIFIED.,.F.,.F.,(4,3,3,
3,3,3,3,4),(20.1593781767107,20.9489988326416,21.9465702056245,22.9441415786074,
23.9417129515904,24.9392843245733,25.9368556975563,26.4425634838903),
 .UNSPECIFIED.);
#3133=B_SPLINE_CURVE_WITH_KNOTS('',3,(#23861,#23862,#23863,#23864,#23865,
#23866,#23867,#23868,#23869,#23870,#23871,#23872,#23873,#23874,#23875,#23876,
#23877,#23878,#23879,#23880,#23881,#23882),.UNSPECIFIED.,.F.,.F.,(4,3,3,
3,3,3,3,4),(-22.695939185231,-21.9465702056245,-20.9489988326416,-19.9514274596586,
-18.9538560866757,-17.9562847136928,-16.9587133407099,-16.4127538780514),
 .UNSPECIFIED.);
#3134=B_SPLINE_CURVE_WITH_KNOTS('',3,(#23887,#23888,#23889,#23890,#23891,
#23892,#23893,#23894,#23895,#23896,#23897,#23898,#23899,#23900,#23901,#23902,
#23903,#23904,#23905,#23906,#23907,#23908,#23909,#23910,#23911),
 .UNSPECIFIED.,.F.,.F.,(4,3,3,3,3,3,3,3,4),(13.8761928695311,13.9659992217611,
14.963570594744,15.9611419677269,16.9587133407099,17.9562847136928,18.9538560866757,
19.9514274596586,20.1593781767107),.UNSPECIFIED.);
#3135=B_SPLINE_CURVE_WITH_KNOTS('',3,(#23912,#23913,#23914,#23915,#23916,
#23917,#23918,#23919,#23920,#23921,#23922,#23923,#23924,#23925,#23926,#23927,
#23928,#23929,#23930,#23931,#23932,#23933),.UNSPECIFIED.,.F.,.F.,(4,3,3,
3,3,3,3,4),(-16.4127538780514,-15.9611419677269,-14.963570594744,-13.9659992217611,
-12.9684278487781,-11.9708564757952,-10.9732851028123,-10.1295685708719),
 .UNSPECIFIED.);
#3136=B_SPLINE_CURVE_WITH_KNOTS('',3,(#23939,#23940,#23941,#23942,#23943,
#23944,#23945,#23946,#23947,#23948,#23949,#23950,#23951),.UNSPECIFIED.,
 .F.,.F.,(4,3,3,3,4),(-3.84638326369226,-2.9927141189488,-1.99514274596587,
-0.997571372982933,0.),.UNSPECIFIED.);
#3137=B_SPLINE_CURVE_WITH_KNOTS('',3,(#23954,#23955,#23956,#23957,#23958,
#23959,#23960,#23961,#23962,#23963,#23964,#23965,#23966,#23967,#23968,#23969,
#23970,#23971,#23972),.UNSPECIFIED.,.F.,.F.,(4,3,3,3,3,3,4),(2.01461286527445,
2.9927141189488,3.99028549193173,4.98785686491466,5.9854282378976,6.98299961088053,
7.59300756235153),.UNSPECIFIED.);
#3138=B_SPLINE_CURVE_WITH_KNOTS('',3,(#23978,#23979,#23980,#23981,#23982,
#23983,#23984),.UNSPECIFIED.,.F.,.F.,(4,1,1,1,4),(91.106186954104,91.6672898428912,
92.6648612158742,93.6624325888571,94.66000396184),.UNSPECIFIED.);
#3139=B_SPLINE_CURVE_WITH_KNOTS('',3,(#23987,#23988,#23989,#23990,#23991,
#23992,#23993,#23994),.UNSPECIFIED.,.F.,.F.,(4,1,1,1,1,4),(91.106186954104,
91.2111367324627,92.2087081054456,93.2062794784286,94.2038508514115,95.1819521050858),
 .UNSPECIFIED.);
#3140=B_SPLINE_CURVE_WITH_KNOTS('',3,(#23999,#24000,#24001,#24002,#24003,
#24004,#24005,#24006,#24007,#24008),.UNSPECIFIED.,.F.,.F.,(4,1,1,1,1,1,
1,4),(84.8230016469244,85.6818616049936,86.6794329779766,87.6770043509595,
88.6745757239424,89.6721470969254,90.6697184699083,91.106186954104),
 .UNSPECIFIED.);
#3141=B_SPLINE_CURVE_WITH_KNOTS('',3,(#24009,#24010,#24011,#24012,#24013,
#24014,#24015,#24016,#24017,#24018),.UNSPECIFIED.,.F.,.F.,(4,1,1,1,1,1,
1,4),(84.8230016469244,85.2257084945651,86.223279867548,87.220851240531,
88.2184226135139,89.2159939864968,90.2135653594798,91.106186954104),
 .UNSPECIFIED.);
#3142=B_SPLINE_CURVE_WITH_KNOTS('',3,(#24023,#24024,#24025,#24026,#24027,
#24028,#24029,#24030,#24031,#24032,#24033),.UNSPECIFIED.,.F.,.F.,(4,1,1,
1,1,1,1,1,4),(78.5398163397448,78.6988619941131,79.696433367096,80.694004740079,
81.6915761130619,82.6891474860448,83.6867188590278,84.6842902320107,84.8230016469244),
 .UNSPECIFIED.);
#3143=B_SPLINE_CURVE_WITH_KNOTS('',3,(#24034,#24035,#24036,#24037,#24038,
#24039,#24040,#24041,#24042,#24043),.UNSPECIFIED.,.F.,.F.,(4,1,1,1,1,1,
1,4),(78.5398163397448,79.2402802566675,80.2378516296505,81.2354230026334,
82.2329943756163,83.2305657485992,84.2281371215822,84.8230016469244),
 .UNSPECIFIED.);
#3144=B_SPLINE_CURVE_WITH_KNOTS('',3,(#24048,#24049,#24050,#24051,#24052,
#24053,#24054,#24055,#24056,#24057),.UNSPECIFIED.,.F.,.F.,(4,1,1,1,1,1,
1,4),(72.2566310325652,72.7134337562155,73.7110051291985,74.7085765021814,
75.7061478751643,76.7037192481473,77.7012906211302,78.5398163397448),
 .UNSPECIFIED.);
#3145=B_SPLINE_CURVE_WITH_KNOTS('',3,(#24058,#24059,#24060,#24061,#24062,
#24063,#24064,#24065,#24066,#24067,#24068),.UNSPECIFIED.,.F.,.F.,(4,1,1,
1,1,1,1,1,4),(72.2566310325652,72.257280645787,73.2548520187699,74.2524233917529,
75.2499947647358,76.2475661377187,77.2451375107017,78.2427088836846,78.5398163397448),
 .UNSPECIFIED.);
#3146=B_SPLINE_CURVE_WITH_KNOTS('',3,(#24073,#24074,#24075,#24076,#24077,
#24078,#24079,#24080,#24081,#24082),.UNSPECIFIED.,.F.,.F.,(4,1,1,1,1,1,
1,4),(65.9734457253856,66.7280055183179,67.7255768913009,68.7231482642838,
69.7207196372667,70.7182910102497,71.7158623832326,72.2566310325652),
 .UNSPECIFIED.);
#3147=B_SPLINE_CURVE_WITH_KNOTS('',3,(#24083,#24084,#24085,#24086,#24087,
#24088,#24089,#24090,#24091,#24092),.UNSPECIFIED.,.F.,.F.,(4,1,1,1,1,1,
1,4),(65.9734457253856,66.2718524078894,67.2694237808723,68.2669951538553,
69.2645665268382,70.2621378998211,71.2597092728041,72.2566310325652),
 .UNSPECIFIED.);
#3148=B_SPLINE_CURVE_WITH_KNOTS('',3,(#24097,#24098,#24099,#24100,#24101,
#24102,#24103,#24104,#24105,#24106,#24107),.UNSPECIFIED.,.F.,.F.,(4,1,1,
1,1,1,1,1,4),(59.690260418206,59.7450059074374,60.7425772804203,61.7401486534033,
62.7377200263862,63.7352913993691,64.7328627723521,65.730434145335,65.9734457253856),
 .UNSPECIFIED.);
#3149=B_SPLINE_CURVE_WITH_KNOTS('',3,(#24108,#24109,#24110,#24111,#24112,
#24113,#24114,#24115,#24116,#24117),.UNSPECIFIED.,.F.,.F.,(4,1,1,1,1,1,
1,4),(59.690260418206,60.2864241699918,61.2839955429747,62.2815669159577,
63.2791382889406,64.2767096619235,65.2742810349065,65.9734457253856),
 .UNSPECIFIED.);
#3150=B_SPLINE_CURVE_WITH_KNOTS('',3,(#24122,#24123,#24124,#24125,#24126,
#24127,#24128,#24129,#24130,#24131),.UNSPECIFIED.,.F.,.F.,(4,1,1,1,1,1,
1,4),(53.4070751110264,53.7595776695398,54.7571490425227,55.7547204155057,
56.7522917884886,57.7498631614715,58.7474345344545,59.690260418206),
 .UNSPECIFIED.);
#3151=B_SPLINE_CURVE_WITH_KNOTS('',3,(#24132,#24133,#24134,#24135,#24136,
#24137,#24138,#24139,#24140,#24141),.UNSPECIFIED.,.F.,.F.,(4,1,1,1,1,1,
1,4),(53.4070751110264,54.3009959320942,55.2985673050771,56.2961386780601,
57.293710051043,58.2912814240259,59.2888527970089,59.690260418206),
 .UNSPECIFIED.);
#3152=B_SPLINE_CURVE_WITH_KNOTS('',3,(#24146,#24147,#24148,#24149,#24150,
#24151,#24152,#24153,#24154,#24155),.UNSPECIFIED.,.F.,.F.,(4,1,1,1,1,1,
1,4),(47.1238898038468,47.7741494316422,48.7717208046251,49.7692921776081,
50.766863550591,51.7644349235739,52.7620062965569,53.4070751110264),
 .UNSPECIFIED.);
#3153=B_SPLINE_CURVE_WITH_KNOTS('',3,(#24156,#24157,#24158,#24159,#24160,
#24161,#24162,#24163,#24164,#24165,#24166),.UNSPECIFIED.,.F.,.F.,(4,1,1,
1,1,1,1,1,4),(47.1238898038468,47.3179963212137,48.3155676941966,49.3131390671795,
50.3107104401625,51.3082818131454,52.3058531861283,53.3034245591113,53.4070751110264),
 .UNSPECIFIED.);
#3154=B_SPLINE_CURVE_WITH_KNOTS('',3,(#24171,#24172,#24173,#24174,#24175,
#24176,#24177,#24178,#24179,#24180),.UNSPECIFIED.,.F.,.F.,(4,1,1,1,1,1,
1,4),(40.8407044966673,41.7887211937446,42.7862925667275,43.7838639397105,
44.7814353126934,45.7790066856763,46.7765780586593,47.1238898038468),
 .UNSPECIFIED.);
#3155=B_SPLINE_CURVE_WITH_KNOTS('',3,(#24181,#24182,#24183,#24184,#24185,
#24186,#24187,#24188,#24189,#24190),.UNSPECIFIED.,.F.,.F.,(4,1,1,1,1,1,
1,4),(40.8407044966673,41.3325680833161,42.330139456299,43.3277108292819,
44.3252822022649,45.3228535752478,46.3204249482307,47.1238898038468),
 .UNSPECIFIED.);
#3156=B_SPLINE_CURVE_WITH_KNOTS('',3,(#24195,#24196,#24197,#24198,#24199,
#24200,#24201,#24202,#24203,#24204,#24205),.UNSPECIFIED.,.F.,.F.,(4,1,1,
1,1,1,1,1,4),(34.5575191894876,34.8057215828641,35.803292955847,36.80086432883,
37.7984357018129,38.7960070747958,39.7935784477787,40.7911498207617,40.8407044966673),
 .UNSPECIFIED.);
#3157=B_SPLINE_CURVE_WITH_KNOTS('',3,(#24206,#24207,#24208,#24209,#24210,
#24211,#24212,#24213,#24214,#24215),.UNSPECIFIED.,.F.,.F.,(4,1,1,1,1,1,
1,4),(34.5575191894876,35.3471398454185,36.3447112184014,37.3422825913843,
38.3398539643673,39.3374253373502,40.3349967103332,40.8407044966673),
 .UNSPECIFIED.);
#3158=B_SPLINE_CURVE_WITH_KNOTS('',3,(#24220,#24221,#24222,#24223,#24224,
#24225,#24226,#24227,#24228,#24229),.UNSPECIFIED.,.F.,.F.,(4,1,1,1,1,1,
1,4),(28.2743338823081,28.8202933449665,29.8178647179494,30.8154360909324,
31.8130074639153,32.8105788368982,33.8081502098811,34.5575191894876),
 .UNSPECIFIED.);
#3159=B_SPLINE_CURVE_WITH_KNOTS('',3,(#24230,#24231,#24232,#24233,#24234,
#24235,#24236,#24237,#24238,#24239,#24240),.UNSPECIFIED.,.F.,.F.,(4,1,1,
1,1,1,1,1,4),(28.2743338823081,28.364140234538,29.3617116075209,30.3592829805038,
31.3568543534868,32.3544257264697,33.3519970994526,34.3495684724355,34.5575191894876),
 .UNSPECIFIED.);
#3160=B_SPLINE_CURVE_WITH_KNOTS('',3,(#24245,#24246,#24247,#24248,#24249,
#24250,#24251,#24252,#24253,#24254),.UNSPECIFIED.,.F.,.F.,(4,1,1,1,1,1,
1,4),(21.9911485751285,22.8348651070689,23.8324364800518,24.8300078530348,
25.8275792260177,26.8251505990006,27.8227219719836,28.2743338823081),
 .UNSPECIFIED.);
#3161=B_SPLINE_CURVE_WITH_KNOTS('',3,(#24255,#24256,#24257,#24258,#24259,
#24260,#24261,#24262,#24263,#24264),.UNSPECIFIED.,.F.,.F.,(4,1,1,1,1,1,
1,4),(21.9911485751285,22.3787119966404,23.3762833696233,24.3738547426062,
25.3714261155892,26.3689974885721,27.366568861555,28.2743338823081),
 .UNSPECIFIED.);
#3162=B_SPLINE_CURVE_WITH_KNOTS('',3,(#24270,#24271,#24272,#24273,#24274),
 .UNSPECIFIED.,.F.,.F.,(4,1,4),(14.3981410127769,15.3957123857598,15.7079632679489),
 .UNSPECIFIED.);
#3163=B_SPLINE_CURVE_WITH_KNOTS('',3,(#24277,#24278,#24279,#24280,#24281),
 .UNSPECIFIED.,.F.,.F.,(4,1,4),(13.8761928695311,14.8542941232054,15.7079632679489),
 .UNSPECIFIED.);
#3164=B_SPLINE_CURVE_WITH_KNOTS('',3,(#24287,#24288,#24289,#24290,#24291,
#24292,#24293,#24294,#24295,#24296,#24297,#24298,#24299,#24300,#24301,#24302,
#24303,#24304,#24305,#24306,#24307,#24308),.UNSPECIFIED.,.F.,.F.,(4,3,3,
3,3,3,3,4),(76.708045941327,76.8129957196858,77.8105670926687,78.8081384656517,
79.8057098386346,80.8032812116175,81.8008525846005,82.7984239575834),
 .UNSPECIFIED.);
#3165=B_SPLINE_CURVE_WITH_KNOTS('',3,(#24312,#24313,#24314,#24315,#24316,
#24317,#24318),.UNSPECIFIED.,.F.,.F.,(4,3,4),(-80.783811092309,-79.8057098386346,
-79.2446069498473),.UNSPECIFIED.);
#3166=B_SPLINE_CURVE_WITH_KNOTS('',3,(#24322,#24323,#24324,#24325,#24326,
#24327,#24328,#24329,#24330,#24331,#24332,#24333,#24334,#24335,#24336,#24337,
#24338,#24339,#24340,#24341,#24342,#24343),.UNSPECIFIED.,.F.,.F.,(4,3,3,
3,3,3,3,4),(-79.2446069498473,-78.8081384656517,-77.8105670926687,-76.8129957196858,
-75.8154243467029,-74.81785297372,-73.820281600737,-72.9614216426677),
 .UNSPECIFIED.);
#3167=B_SPLINE_CURVE_WITH_KNOTS('',3,(#24348,#24349,#24350,#24351,#24352,
#24353,#24354,#24355,#24356,#24357,#24358,#24359,#24360,#24361,#24362,#24363,
#24364,#24365,#24366,#24367,#24368,#24369),.UNSPECIFIED.,.F.,.F.,(4,3,3,
3,3,3,3,4),(70.4248606341474,70.8275674817882,71.8251388547712,72.8227102277541,
73.820281600737,74.81785297372,75.8154243467029,76.708045941327),
 .UNSPECIFIED.);
#3168=B_SPLINE_CURVE_WITH_KNOTS('',3,(#24370,#24371,#24372,#24373,#24374,
#24375,#24376,#24377,#24378,#24379,#24380,#24381,#24382,#24383,#24384,#24385,
#24386,#24387,#24388,#24389,#24390,#24391,#24392,#24393,#24394),
 .UNSPECIFIED.,.F.,.F.,(4,3,3,3,3,3,3,3,4),(-72.9614216426677,-72.8227102277541,
-71.8251388547712,-70.8275674817882,-69.8299961088053,-68.8324247358224,
-67.8348533628394,-66.8372819898565,-66.6782363354881),.UNSPECIFIED.);
#3169=B_SPLINE_CURVE_WITH_KNOTS('',3,(#24399,#24400,#24401,#24402,#24403,
#24404,#24405,#24406,#24407,#24408,#24409,#24410,#24411,#24412,#24413,#24414,
#24415,#24416,#24417,#24418,#24419,#24420),.UNSPECIFIED.,.F.,.F.,(4,3,3,
3,3,3,3,4),(64.1416753269678,64.8421392438906,65.8397106168735,66.8372819898565,
67.8348533628394,68.8324247358223,69.8299961088053,70.4248606341474),
 .UNSPECIFIED.);
#3170=B_SPLINE_CURVE_WITH_KNOTS('',3,(#24421,#24422,#24423,#24424,#24425,
#24426,#24427,#24428,#24429,#24430,#24431,#24432,#24433,#24434,#24435,#24436,
#24437,#24438,#24439,#24440,#24441,#24442),.UNSPECIFIED.,.F.,.F.,(4,3,3,
3,3,3,3,4),(-66.6782363354881,-65.8397106168736,-64.8421392438906,-63.8445678709077,
-62.8469964979248,-61.8494251249418,-60.8518537519589,-60.3950510283085),
 .UNSPECIFIED.);
#3171=B_SPLINE_CURVE_WITH_KNOTS('',3,(#24447,#24448,#24449,#24450,#24451,
#24452,#24453,#24454,#24455,#24456,#24457,#24458,#24459,#24460,#24461,#24462,
#24463,#24464,#24465,#24466,#24467,#24468),.UNSPECIFIED.,.F.,.F.,(4,3,3,
3,3,3,3,4),(57.8584900197882,58.856711005993,59.854282378976,60.8518537519589,
61.8494251249418,62.8469964979248,63.8445678709077,64.1416753269678),
 .UNSPECIFIED.);
#3172=B_SPLINE_CURVE_WITH_KNOTS('',3,(#24469,#24470,#24471,#24472,#24473,
#24474,#24475,#24476,#24477,#24478,#24479,#24480,#24481,#24482,#24483,#24484,
#24485,#24486,#24487,#24488,#24489,#24490),.UNSPECIFIED.,.F.,.F.,(4,3,3,
3,3,3,3,4),(-60.3950510283085,-59.854282378976,-58.856711005993,-57.8591396330101,
-56.8615682600271,-55.8639968870442,-54.8664255140613,-54.111865721129),
 .UNSPECIFIED.);
#3173=B_SPLINE_CURVE_WITH_KNOTS('',3,(#24495,#24496,#24497,#24498,#24499,
#24500,#24501,#24502,#24503,#24504,#24505,#24506,#24507,#24508,#24509,#24510,
#24511,#24512,#24513,#24514,#24515,#24516),.UNSPECIFIED.,.F.,.F.,(4,3,3,
3,3,3,3,4),(51.5753047126087,51.8737113951125,52.8712827680954,53.8688541410784,
54.8664255140613,55.8639968870442,56.8615682600272,57.8584900197882),
 .UNSPECIFIED.);
#3174=B_SPLINE_CURVE_WITH_KNOTS('',3,(#24517,#24518,#24519,#24520,#24521,
#24522,#24523,#24524,#24525,#24526,#24527,#24528,#24529,#24530,#24531,#24532,
#24533,#24534,#24535,#24536,#24537,#24538,#24539,#24540,#24541),
 .UNSPECIFIED.,.F.,.F.,(4,3,3,3,3,3,3,3,4),(-54.111865721129,-53.8688541410784,
-52.8712827680954,-51.8737113951125,-50.8761400221296,-49.8785686491466,
-48.8809972761637,-47.8834259031808,-47.8286804139494),.UNSPECIFIED.);
#3175=B_SPLINE_CURVE_WITH_KNOTS('',3,(#24546,#24547,#24548,#24549,#24550,
#24551,#24552,#24553,#24554,#24555,#24556,#24557,#24558,#24559,#24560,#24561,
#24562,#24563,#24564,#24565,#24566,#24567),.UNSPECIFIED.,.F.,.F.,(4,3,3,
3,3,3,3,4),(45.2921194054291,45.8882831572149,46.8858545301978,47.8834259031808,
48.8809972761637,49.8785686491466,50.8761400221296,51.5753047126087),
 .UNSPECIFIED.);
#3176=B_SPLINE_CURVE_WITH_KNOTS('',3,(#24568,#24569,#24570,#24571,#24572,
#24573,#24574,#24575,#24576,#24577,#24578,#24579,#24580,#24581,#24582,#24583,
#24584,#24585,#24586,#24587,#24588,#24589),.UNSPECIFIED.,.F.,.F.,(4,3,3,
3,3,3,3,4),(-47.8286804139494,-46.8858545301978,-45.8882831572149,-44.890711784232,
-43.893140411249,-42.8955690382661,-41.8979976652832,-41.5454951067698),
 .UNSPECIFIED.);
#3177=B_SPLINE_CURVE_WITH_KNOTS('',3,(#24594,#24595,#24596,#24597,#24598,
#24599,#24600,#24601,#24602,#24603,#24604,#24605,#24606,#24607,#24608,#24609,
#24610,#24611,#24612,#24613,#24614,#24615),.UNSPECIFIED.,.F.,.F.,(4,3,3,
3,3,3,3,4),(39.0089340982495,39.9028549193173,40.9004262923002,41.8979976652832,
42.8955690382661,43.893140411249,44.890711784232,45.2921194054291),
 .UNSPECIFIED.);
#3178=B_SPLINE_CURVE_WITH_KNOTS('',3,(#24616,#24617,#24618,#24619,#24620,
#24621,#24622,#24623,#24624,#24625,#24626,#24627,#24628,#24629,#24630,#24631,
#24632,#24633,#24634,#24635,#24636,#24637),.UNSPECIFIED.,.F.,.F.,(4,3,3,
3,3,3,3,4),(-41.5454951067698,-40.9004262923002,-39.9028549193173,-38.9052835463344,
-37.9077121733514,-36.9101408003685,-35.9125694273856,-35.2623097995902),
 .UNSPECIFIED.);
#3179=B_SPLINE_CURVE_WITH_KNOTS('',3,(#24642,#24643,#24644,#24645,#24646,
#24647,#24648,#24649,#24650,#24651,#24652,#24653,#24654,#24655,#24656,#24657,
#24658,#24659,#24660,#24661,#24662,#24663,#24664,#24665,#24666),
 .UNSPECIFIED.,.F.,.F.,(4,3,3,3,3,3,3,3,4),(32.7257487910699,32.9198553084368,
33.9174266814197,34.9149980544026,35.9125694273856,36.9101408003685,37.9077121733514,
38.9052835463344,39.0089340982495),.UNSPECIFIED.);
#3180=B_SPLINE_CURVE_WITH_KNOTS('',3,(#24667,#24668,#24669,#24670,#24671,
#24672,#24673,#24674,#24675,#24676,#24677,#24678,#24679,#24680,#24681,#24682,
#24683,#24684,#24685,#24686,#24687,#24688),.UNSPECIFIED.,.F.,.F.,(4,3,3,
3,3,3,3,4),(-35.2623097995902,-34.9149980544027,-33.9174266814197,-32.9198553084368,
-31.9222839354538,-30.9247125624709,-29.927141189488,-28.9791244924106),
 .UNSPECIFIED.);
#3181=B_SPLINE_CURVE_WITH_KNOTS('',3,(#24693,#24694,#24695,#24696,#24697,
#24698,#24699,#24700,#24701,#24702,#24703,#24704,#24705,#24706,#24707,#24708,
#24709,#24710,#24711,#24712,#24713,#24714),.UNSPECIFIED.,.F.,.F.,(4,3,3,
3,3,3,3,4),(26.4425634838903,26.9344270705392,27.9319984435221,28.929569816505,
29.927141189488,30.9247125624709,31.9222839354538,32.7257487910699),
 .UNSPECIFIED.);
#3182=B_SPLINE_CURVE_WITH_KNOTS('',3,(#24715,#24716,#24717,#24718,#24719,
#24720,#24721,#24722,#24723,#24724,#24725,#24726,#24727,#24728,#24729,#24730,
#24731,#24732,#24733,#24734,#24735,#24736,#24737,#24738,#24739),
 .UNSPECIFIED.,.F.,.F.,(4,3,3,3,3,3,3,3,4),(-28.9791244924106,-28.929569816505,
-27.9319984435221,-26.9344270705392,-25.9368556975562,-24.9392843245733,
-23.9417129515904,-22.9441415786075,-22.695939185231),.UNSPECIFIED.);
#3183=B_SPLINE_CURVE_WITH_KNOTS('',3,(#24744,#24745,#24746,#24747,#24748,
#24749,#24750,#24751,#24752,#24753,#24754,#24755,#24756,#24757,#24758,#24759,
#24760,#24761,#24762,#24763,#24764,#24765),.UNSPECIFIED.,.F.,.F.,(4,3,3,
3,3,3,3,4),(20.1593781767107,20.9489988326416,21.9465702056245,22.9441415786075,
23.9417129515904,24.9392843245733,25.9368556975563,26.4425634838903),
 .UNSPECIFIED.);
#3184=B_SPLINE_CURVE_WITH_KNOTS('',3,(#24766,#24767,#24768,#24769,#24770,
#24771,#24772,#24773,#24774,#24775,#24776,#24777,#24778,#24779,#24780,#24781,
#24782,#24783,#24784,#24785,#24786,#24787),.UNSPECIFIED.,.F.,.F.,(4,3,3,
3,3,3,3,4),(-22.695939185231,-21.9465702056245,-20.9489988326416,-19.9514274596587,
-18.9538560866757,-17.9562847136928,-16.9587133407099,-16.4127538780514),
 .UNSPECIFIED.);
#3185=B_SPLINE_CURVE_WITH_KNOTS('',3,(#24792,#24793,#24794,#24795,#24796,
#24797,#24798,#24799,#24800,#24801,#24802,#24803,#24804,#24805,#24806,#24807,
#24808,#24809,#24810,#24811,#24812,#24813,#24814,#24815,#24816),
 .UNSPECIFIED.,.F.,.F.,(4,3,3,3,3,3,3,3,4),(13.8761928695311,13.9659992217611,
14.963570594744,15.9611419677269,16.9587133407099,17.9562847136928,18.9538560866757,
19.9514274596586,20.1593781767107),.UNSPECIFIED.);
#3186=B_SPLINE_CURVE_WITH_KNOTS('',3,(#24817,#24818,#24819,#24820,#24821,
#24822,#24823,#24824,#24825,#24826,#24827,#24828,#24829,#24830,#24831,#24832,
#24833,#24834,#24835,#24836,#24837,#24838),.UNSPECIFIED.,.F.,.F.,(4,3,3,
3,3,3,3,4),(-16.4127538780514,-15.9611419677269,-14.963570594744,-13.9659992217611,
-12.9684278487781,-11.9708564757952,-10.9732851028123,-10.1295685708718),
 .UNSPECIFIED.);
#3187=B_SPLINE_CURVE_WITH_KNOTS('',3,(#24844,#24845,#24846,#24847,#24848,
#24849,#24850,#24851,#24852,#24853,#24854,#24855,#24856),.UNSPECIFIED.,
 .F.,.F.,(4,3,3,3,4),(-3.84638326369223,-2.9927141189488,-1.99514274596586,
-0.997571372982929,0.),.UNSPECIFIED.);
#3188=B_SPLINE_CURVE_WITH_KNOTS('',3,(#24859,#24860,#24861,#24862,#24863,
#24864,#24865,#24866,#24867,#24868,#24869,#24870,#24871,#24872,#24873,#24874,
#24875,#24876,#24877),.UNSPECIFIED.,.F.,.F.,(4,3,3,3,3,3,4),(2.01461286527443,
2.9927141189488,3.99028549193173,4.98785686491467,5.9854282378976,6.98299961088053,
7.59300756235153),.UNSPECIFIED.);
#3189=B_SPLINE_CURVE_WITH_KNOTS('',3,(#24883,#24884,#24885,#24886,#24887,
#24888,#24889),.UNSPECIFIED.,.F.,.F.,(4,1,1,1,4),(91.106186954104,91.6672898428913,
92.6648612158742,93.6624325888572,94.6600039618401),.UNSPECIFIED.);
#3190=B_SPLINE_CURVE_WITH_KNOTS('',3,(#24892,#24893,#24894,#24895,#24896,
#24897,#24898,#24899),.UNSPECIFIED.,.F.,.F.,(4,1,1,1,1,4),(91.106186954104,
91.2111367324627,92.2087081054457,93.2062794784286,94.2038508514115,95.1819521050859),
 .UNSPECIFIED.);
#3191=B_SPLINE_CURVE_WITH_KNOTS('',3,(#24904,#24905,#24906,#24907,#24908,
#24909,#24910,#24911,#24912,#24913),.UNSPECIFIED.,.F.,.F.,(4,1,1,1,1,1,
1,4),(84.8230016469244,85.6818616049937,86.6794329779766,87.6770043509596,
88.6745757239425,89.6721470969254,90.6697184699084,91.106186954104),
 .UNSPECIFIED.);
#3192=B_SPLINE_CURVE_WITH_KNOTS('',3,(#24914,#24915,#24916,#24917,#24918,
#24919,#24920,#24921,#24922,#24923),.UNSPECIFIED.,.F.,.F.,(4,1,1,1,1,1,
1,4),(84.8230016469244,85.2257084945651,86.2232798675481,87.220851240531,
88.2184226135139,89.2159939864969,90.2135653594798,91.106186954104),
 .UNSPECIFIED.);
#3193=B_SPLINE_CURVE_WITH_KNOTS('',3,(#24928,#24929,#24930,#24931,#24932,
#24933,#24934,#24935,#24936,#24937,#24938),.UNSPECIFIED.,.F.,.F.,(4,1,1,
1,1,1,1,1,4),(78.5398163397448,78.6988619941132,79.6964333670961,80.694004740079,
81.691576113062,82.6891474860449,83.6867188590278,84.6842902320108,84.8230016469244),
 .UNSPECIFIED.);
#3194=B_SPLINE_CURVE_WITH_KNOTS('',3,(#24939,#24940,#24941,#24942,#24943,
#24944,#24945,#24946,#24947,#24948),.UNSPECIFIED.,.F.,.F.,(4,1,1,1,1,1,
1,4),(78.5398163397448,79.2402802566675,80.2378516296505,81.2354230026334,
82.2329943756163,83.2305657485993,84.2281371215822,84.8230016469244),
 .UNSPECIFIED.);
#3195=B_SPLINE_CURVE_WITH_KNOTS('',3,(#24953,#24954,#24955,#24956,#24957,
#24958,#24959,#24960,#24961,#24962),.UNSPECIFIED.,.F.,.F.,(4,1,1,1,1,1,
1,4),(72.2566310325652,72.7134337562156,73.7110051291985,74.7085765021814,
75.7061478751644,76.7037192481473,77.7012906211302,78.5398163397448),
 .UNSPECIFIED.);
#3196=B_SPLINE_CURVE_WITH_KNOTS('',3,(#24963,#24964,#24965,#24966,#24967,
#24968,#24969,#24970,#24971,#24972,#24973),.UNSPECIFIED.,.F.,.F.,(4,1,1,
1,1,1,1,1,4),(72.2566310325652,72.257280645787,73.25485201877,74.2524233917529,
75.2499947647358,76.2475661377187,77.2451375107017,78.2427088836846,78.5398163397448),
 .UNSPECIFIED.);
#3197=B_SPLINE_CURVE_WITH_KNOTS('',3,(#24978,#24979,#24980,#24981,#24982,
#24983,#24984,#24985,#24986,#24987),.UNSPECIFIED.,.F.,.F.,(4,1,1,1,1,1,
1,4),(65.9734457253856,66.728005518318,67.7255768913009,68.7231482642838,
69.7207196372668,70.7182910102497,71.7158623832326,72.2566310325652),
 .UNSPECIFIED.);
#3198=B_SPLINE_CURVE_WITH_KNOTS('',3,(#24988,#24989,#24990,#24991,#24992,
#24993,#24994,#24995,#24996,#24997),.UNSPECIFIED.,.F.,.F.,(4,1,1,1,1,1,
1,4),(65.9734457253856,66.2718524078894,67.2694237808724,68.2669951538553,
69.2645665268382,70.2621378998212,71.2597092728041,72.2566310325652),
 .UNSPECIFIED.);
#3199=B_SPLINE_CURVE_WITH_KNOTS('',3,(#25002,#25003,#25004,#25005,#25006,
#25007,#25008,#25009,#25010,#25011,#25012),.UNSPECIFIED.,.F.,.F.,(4,1,1,
1,1,1,1,1,4),(59.690260418206,59.7450059074374,60.7425772804204,61.7401486534033,
62.7377200263862,63.7352913993692,64.7328627723521,65.730434145335,65.9734457253856),
 .UNSPECIFIED.);
#3200=B_SPLINE_CURVE_WITH_KNOTS('',3,(#25013,#25014,#25015,#25016,#25017,
#25018,#25019,#25020,#25021,#25022),.UNSPECIFIED.,.F.,.F.,(4,1,1,1,1,1,
1,4),(59.690260418206,60.2864241699918,61.2839955429748,62.2815669159577,
63.2791382889406,64.2767096619236,65.2742810349065,65.9734457253856),
 .UNSPECIFIED.);
#3201=B_SPLINE_CURVE_WITH_KNOTS('',3,(#25027,#25028,#25029,#25030,#25031,
#25032,#25033,#25034,#25035,#25036),.UNSPECIFIED.,.F.,.F.,(4,1,1,1,1,1,
1,4),(53.4070751110264,53.7595776695399,54.7571490425228,55.7547204155057,
56.7522917884886,57.7498631614716,58.7474345344545,59.690260418206),
 .UNSPECIFIED.);
#3202=B_SPLINE_CURVE_WITH_KNOTS('',3,(#25037,#25038,#25039,#25040,#25041,
#25042,#25043,#25044,#25045,#25046),.UNSPECIFIED.,.F.,.F.,(4,1,1,1,1,1,
1,4),(53.4070751110264,54.3009959320942,55.2985673050772,56.2961386780601,
57.293710051043,58.291281424026,59.2888527970089,59.690260418206),
 .UNSPECIFIED.);
#3203=B_SPLINE_CURVE_WITH_KNOTS('',3,(#25051,#25052,#25053,#25054,#25055,
#25056,#25057,#25058,#25059,#25060),.UNSPECIFIED.,.F.,.F.,(4,1,1,1,1,1,
1,4),(47.1238898038468,47.7741494316423,48.7717208046252,49.7692921776081,
50.7668635505911,51.764434923574,52.7620062965569,53.4070751110264),
 .UNSPECIFIED.);
#3204=B_SPLINE_CURVE_WITH_KNOTS('',3,(#25061,#25062,#25063,#25064,#25065,
#25066,#25067,#25068,#25069,#25070,#25071),.UNSPECIFIED.,.F.,.F.,(4,1,1,
1,1,1,1,1,4),(47.1238898038468,47.3179963212137,48.3155676941966,49.3131390671796,
50.3107104401625,51.3082818131454,52.3058531861284,53.3034245591113,53.4070751110264),
 .UNSPECIFIED.);
#3205=B_SPLINE_CURVE_WITH_KNOTS('',3,(#25076,#25077,#25078,#25079,#25080,
#25081,#25082,#25083,#25084,#25085),.UNSPECIFIED.,.F.,.F.,(4,1,1,1,1,1,
1,4),(40.8407044966673,41.7887211937447,42.7862925667276,43.7838639397105,
44.7814353126935,45.7790066856764,46.7765780586593,47.1238898038468),
 .UNSPECIFIED.);
#3206=B_SPLINE_CURVE_WITH_KNOTS('',3,(#25086,#25087,#25088,#25089,#25090,
#25091,#25092,#25093,#25094,#25095),.UNSPECIFIED.,.F.,.F.,(4,1,1,1,1,1,
1,4),(40.8407044966673,41.3325680833161,42.330139456299,43.327710829282,
44.3252822022649,45.3228535752478,46.3204249482308,47.1238898038468),
 .UNSPECIFIED.);
#3207=B_SPLINE_CURVE_WITH_KNOTS('',3,(#25100,#25101,#25102,#25103,#25104,
#25105,#25106,#25107,#25108,#25109,#25110),.UNSPECIFIED.,.F.,.F.,(4,1,1,
1,1,1,1,1,4),(34.5575191894876,34.8057215828641,35.8032929558471,36.80086432883,
37.7984357018129,38.7960070747959,39.7935784477788,40.7911498207617,40.8407044966673),
 .UNSPECIFIED.);
#3208=B_SPLINE_CURVE_WITH_KNOTS('',3,(#25111,#25112,#25113,#25114,#25115,
#25116,#25117,#25118,#25119,#25120),.UNSPECIFIED.,.F.,.F.,(4,1,1,1,1,1,
1,4),(34.5575191894876,35.3471398454185,36.3447112184014,37.3422825913844,
38.3398539643673,39.3374253373502,40.3349967103332,40.8407044966673),
 .UNSPECIFIED.);
#3209=B_SPLINE_CURVE_WITH_KNOTS('',3,(#25125,#25126,#25127,#25128,#25129,
#25130,#25131,#25132,#25133,#25134),.UNSPECIFIED.,.F.,.F.,(4,1,1,1,1,1,
1,4),(28.2743338823081,28.8202933449665,29.8178647179495,30.8154360909324,
31.8130074639153,32.8105788368983,33.8081502098812,34.5575191894876),
 .UNSPECIFIED.);
#3210=B_SPLINE_CURVE_WITH_KNOTS('',3,(#25135,#25136,#25137,#25138,#25139,
#25140,#25141,#25142,#25143,#25144,#25145),.UNSPECIFIED.,.F.,.F.,(4,1,1,
1,1,1,1,1,4),(28.2743338823081,28.364140234538,29.3617116075209,30.3592829805038,
31.3568543534868,32.3544257264697,33.3519970994526,34.3495684724356,34.5575191894876),
 .UNSPECIFIED.);
#3211=B_SPLINE_CURVE_WITH_KNOTS('',3,(#25150,#25151,#25152,#25153,#25154,
#25155,#25156,#25157,#25158,#25159),.UNSPECIFIED.,.F.,.F.,(4,1,1,1,1,1,
1,4),(21.9911485751285,22.8348651070689,23.8324364800519,24.8300078530348,
25.8275792260177,26.8251505990007,27.8227219719836,28.2743338823081),
 .UNSPECIFIED.);
#3212=B_SPLINE_CURVE_WITH_KNOTS('',3,(#25160,#25161,#25162,#25163,#25164,
#25165,#25166,#25167,#25168,#25169),.UNSPECIFIED.,.F.,.F.,(4,1,1,1,1,1,
1,4),(21.9911485751285,22.3787119966404,23.3762833696233,24.3738547426063,
25.3714261155892,26.3689974885721,27.3665688615551,28.2743338823081),
 .UNSPECIFIED.);
#3213=B_SPLINE_CURVE_WITH_KNOTS('',3,(#25175,#25176,#25177,#25178,#25179),
 .UNSPECIFIED.,.F.,.F.,(4,1,4),(14.3981410127769,15.3957123857599,15.7079632679489),
 .UNSPECIFIED.);
#3214=B_SPLINE_CURVE_WITH_KNOTS('',3,(#25182,#25183,#25184,#25185,#25186),
 .UNSPECIFIED.,.F.,.F.,(4,1,4),(13.8761928695311,14.8542941232055,15.7079632679489),
 .UNSPECIFIED.);
#3215=B_SPLINE_CURVE_WITH_KNOTS('',3,(#25192,#25193,#25194,#25195,#25196,
#25197,#25198,#25199,#25200,#25201,#25202,#25203,#25204,#25205,#25206,#25207,
#25208,#25209,#25210,#25211,#25212,#25213),.UNSPECIFIED.,.F.,.F.,(4,3,3,
3,3,3,3,4),(76.7080459413271,76.8129957196858,77.8105670926687,78.8081384656517,
79.8057098386346,80.8032812116175,81.8008525846005,82.7984239575834),
 .UNSPECIFIED.);
#3216=B_SPLINE_CURVE_WITH_KNOTS('',3,(#25217,#25218,#25219,#25220,#25221,
#25222,#25223),.UNSPECIFIED.,.F.,.F.,(4,3,4),(-80.783811092309,-79.8057098386346,
-79.2446069498474),.UNSPECIFIED.);
#3217=B_SPLINE_CURVE_WITH_KNOTS('',3,(#25227,#25228,#25229,#25230,#25231,
#25232,#25233,#25234,#25235,#25236,#25237,#25238,#25239,#25240,#25241,#25242,
#25243,#25244,#25245,#25246,#25247,#25248),.UNSPECIFIED.,.F.,.F.,(4,3,3,
3,3,3,3,4),(-79.2446069498474,-78.8081384656517,-77.8105670926687,-76.8129957196858,
-75.8154243467029,-74.8178529737199,-73.820281600737,-72.9614216426678),
 .UNSPECIFIED.);
#3218=B_SPLINE_CURVE_WITH_KNOTS('',3,(#25253,#25254,#25255,#25256,#25257,
#25258,#25259,#25260,#25261,#25262,#25263,#25264,#25265,#25266,#25267,#25268,
#25269,#25270,#25271,#25272,#25273,#25274),.UNSPECIFIED.,.F.,.F.,(4,3,3,
3,3,3,3,4),(70.4248606341475,70.8275674817882,71.8251388547711,72.8227102277541,
73.820281600737,74.8178529737199,75.8154243467029,76.7080459413271),
 .UNSPECIFIED.);
#3219=B_SPLINE_CURVE_WITH_KNOTS('',3,(#25275,#25276,#25277,#25278,#25279,
#25280,#25281,#25282,#25283,#25284,#25285,#25286,#25287,#25288,#25289,#25290,
#25291,#25292,#25293,#25294,#25295,#25296,#25297,#25298,#25299),
 .UNSPECIFIED.,.F.,.F.,(4,3,3,3,3,3,3,3,4),(-72.9614216426678,-72.8227102277541,
-71.8251388547711,-70.8275674817882,-69.8299961088053,-68.8324247358223,
-67.8348533628394,-66.8372819898565,-66.6782363354882),.UNSPECIFIED.);
#3220=B_SPLINE_CURVE_WITH_KNOTS('',3,(#25304,#25305,#25306,#25307,#25308,
#25309,#25310,#25311,#25312,#25313,#25314,#25315,#25316,#25317,#25318,#25319,
#25320,#25321,#25322,#25323,#25324,#25325),.UNSPECIFIED.,.F.,.F.,(4,3,3,
3,3,3,3,4),(64.1416753269679,64.8421392438906,65.8397106168735,66.8372819898565,
67.8348533628394,68.8324247358223,69.8299961088053,70.4248606341475),
 .UNSPECIFIED.);
#3221=B_SPLINE_CURVE_WITH_KNOTS('',3,(#25326,#25327,#25328,#25329,#25330,
#25331,#25332,#25333,#25334,#25335,#25336,#25337,#25338,#25339,#25340,#25341,
#25342,#25343,#25344,#25345,#25346,#25347),.UNSPECIFIED.,.F.,.F.,(4,3,3,
3,3,3,3,4),(-66.6782363354882,-65.8397106168736,-64.8421392438906,-63.8445678709077,
-62.8469964979247,-61.8494251249418,-60.8518537519589,-60.3950510283086),
 .UNSPECIFIED.);
#3222=B_SPLINE_CURVE_WITH_KNOTS('',3,(#25352,#25353,#25354,#25355,#25356,
#25357,#25358,#25359,#25360,#25361,#25362,#25363,#25364,#25365,#25366,#25367,
#25368,#25369,#25370,#25371,#25372,#25373),.UNSPECIFIED.,.F.,.F.,(4,3,3,
3,3,3,3,4),(57.8584900197883,58.856711005993,59.854282378976,60.8518537519589,
61.8494251249418,62.8469964979248,63.8445678709077,64.1416753269679),
 .UNSPECIFIED.);
#3223=B_SPLINE_CURVE_WITH_KNOTS('',3,(#25374,#25375,#25376,#25377,#25378,
#25379,#25380,#25381,#25382,#25383,#25384,#25385,#25386,#25387,#25388,#25389,
#25390,#25391,#25392,#25393,#25394,#25395),.UNSPECIFIED.,.F.,.F.,(4,3,3,
3,3,3,3,4),(-60.3950510283086,-59.854282378976,-58.856711005993,-57.8591396330101,
-56.8615682600272,-55.8639968870442,-54.8664255140613,-54.111865721129),
 .UNSPECIFIED.);
#3224=B_SPLINE_CURVE_WITH_KNOTS('',3,(#25400,#25401,#25402,#25403,#25404,
#25405,#25406,#25407,#25408,#25409,#25410,#25411,#25412,#25413,#25414,#25415,
#25416,#25417,#25418,#25419,#25420,#25421),.UNSPECIFIED.,.F.,.F.,(4,3,3,
3,3,3,3,4),(51.5753047126087,51.8737113951125,52.8712827680954,53.8688541410784,
54.8664255140613,55.8639968870442,56.8615682600272,57.8584900197883),
 .UNSPECIFIED.);
#3225=B_SPLINE_CURVE_WITH_KNOTS('',3,(#25422,#25423,#25424,#25425,#25426,
#25427,#25428,#25429,#25430,#25431,#25432,#25433,#25434,#25435,#25436,#25437,
#25438,#25439,#25440,#25441,#25442,#25443,#25444,#25445,#25446),
 .UNSPECIFIED.,.F.,.F.,(4,3,3,3,3,3,3,3,4),(-54.111865721129,-53.8688541410784,
-52.8712827680954,-51.8737113951125,-50.8761400221296,-49.8785686491466,
-48.8809972761637,-47.8834259031808,-47.8286804139494),.UNSPECIFIED.);
#3226=B_SPLINE_CURVE_WITH_KNOTS('',3,(#25451,#25452,#25453,#25454,#25455,
#25456,#25457,#25458,#25459,#25460,#25461,#25462,#25463,#25464,#25465,#25466,
#25467,#25468,#25469,#25470,#25471,#25472),.UNSPECIFIED.,.F.,.F.,(4,3,3,
3,3,3,3,4),(45.2921194054291,45.8882831572149,46.8858545301978,47.8834259031808,
48.8809972761637,49.8785686491466,50.8761400221296,51.5753047126087),
 .UNSPECIFIED.);
#3227=B_SPLINE_CURVE_WITH_KNOTS('',3,(#25473,#25474,#25475,#25476,#25477,
#25478,#25479,#25480,#25481,#25482,#25483,#25484,#25485,#25486,#25487,#25488,
#25489,#25490,#25491,#25492,#25493,#25494),.UNSPECIFIED.,.F.,.F.,(4,3,3,
3,3,3,3,4),(-47.8286804139494,-46.8858545301978,-45.8882831572149,-44.890711784232,
-43.893140411249,-42.8955690382661,-41.8979976652832,-41.5454951067698),
 .UNSPECIFIED.);
#3228=B_SPLINE_CURVE_WITH_KNOTS('',3,(#25499,#25500,#25501,#25502,#25503,
#25504,#25505,#25506,#25507,#25508,#25509,#25510,#25511,#25512,#25513,#25514,
#25515,#25516,#25517,#25518,#25519,#25520),.UNSPECIFIED.,.F.,.F.,(4,3,3,
3,3,3,3,4),(39.0089340982495,39.9028549193173,40.9004262923002,41.8979976652832,
42.8955690382661,43.893140411249,44.890711784232,45.2921194054291),
 .UNSPECIFIED.);
#3229=B_SPLINE_CURVE_WITH_KNOTS('',3,(#25521,#25522,#25523,#25524,#25525,
#25526,#25527,#25528,#25529,#25530,#25531,#25532,#25533,#25534,#25535,#25536,
#25537,#25538,#25539,#25540,#25541,#25542),.UNSPECIFIED.,.F.,.F.,(4,3,3,
3,3,3,3,4),(-41.5454951067698,-40.9004262923002,-39.9028549193173,-38.9052835463344,
-37.9077121733514,-36.9101408003685,-35.9125694273856,-35.2623097995902),
 .UNSPECIFIED.);
#3230=B_SPLINE_CURVE_WITH_KNOTS('',3,(#25547,#25548,#25549,#25550,#25551,
#25552,#25553,#25554,#25555,#25556,#25557,#25558,#25559,#25560,#25561,#25562,
#25563,#25564,#25565,#25566,#25567,#25568,#25569,#25570,#25571),
 .UNSPECIFIED.,.F.,.F.,(4,3,3,3,3,3,3,3,4),(32.7257487910699,32.9198553084368,
33.9174266814197,34.9149980544026,35.9125694273856,36.9101408003685,37.9077121733514,
38.9052835463344,39.0089340982495),.UNSPECIFIED.);
#3231=B_SPLINE_CURVE_WITH_KNOTS('',3,(#25572,#25573,#25574,#25575,#25576,
#25577,#25578,#25579,#25580,#25581,#25582,#25583,#25584,#25585,#25586,#25587,
#25588,#25589,#25590,#25591,#25592,#25593),.UNSPECIFIED.,.F.,.F.,(4,3,3,
3,3,3,3,4),(-35.2623097995902,-34.9149980544026,-33.9174266814197,-32.9198553084368,
-31.9222839354538,-30.9247125624709,-29.927141189488,-28.9791244924107),
 .UNSPECIFIED.);
#3232=B_SPLINE_CURVE_WITH_KNOTS('',3,(#25598,#25599,#25600,#25601,#25602,
#25603,#25604,#25605,#25606,#25607,#25608,#25609,#25610,#25611,#25612,#25613,
#25614,#25615,#25616,#25617,#25618,#25619),.UNSPECIFIED.,.F.,.F.,(4,3,3,
3,3,3,3,4),(26.4425634838903,26.9344270705392,27.9319984435221,28.9295698165051,
29.927141189488,30.9247125624709,31.9222839354538,32.7257487910699),
 .UNSPECIFIED.);
#3233=B_SPLINE_CURVE_WITH_KNOTS('',3,(#25620,#25621,#25622,#25623,#25624,
#25625,#25626,#25627,#25628,#25629,#25630,#25631,#25632,#25633,#25634,#25635,
#25636,#25637,#25638,#25639,#25640,#25641,#25642,#25643,#25644),
 .UNSPECIFIED.,.F.,.F.,(4,3,3,3,3,3,3,3,4),(-28.9791244924107,-28.929569816505,
-27.9319984435221,-26.9344270705392,-25.9368556975563,-24.9392843245733,
-23.9417129515904,-22.9441415786074,-22.6959391852311),.UNSPECIFIED.);
#3234=B_SPLINE_CURVE_WITH_KNOTS('',3,(#25649,#25650,#25651,#25652,#25653,
#25654,#25655,#25656,#25657,#25658,#25659,#25660,#25661,#25662,#25663,#25664,
#25665,#25666,#25667,#25668,#25669,#25670),.UNSPECIFIED.,.F.,.F.,(4,3,3,
3,3,3,3,4),(20.1593781767108,20.9489988326416,21.9465702056245,22.9441415786075,
23.9417129515904,24.9392843245733,25.9368556975563,26.4425634838903),
 .UNSPECIFIED.);
#3235=B_SPLINE_CURVE_WITH_KNOTS('',3,(#25671,#25672,#25673,#25674,#25675,
#25676,#25677,#25678,#25679,#25680,#25681,#25682,#25683,#25684,#25685,#25686,
#25687,#25688,#25689,#25690,#25691,#25692),.UNSPECIFIED.,.F.,.F.,(4,3,3,
3,3,3,3,4),(-22.6959391852311,-21.9465702056245,-20.9489988326416,-19.9514274596586,
-18.9538560866757,-17.9562847136928,-16.9587133407099,-16.4127538780515),
 .UNSPECIFIED.);
#3236=B_SPLINE_CURVE_WITH_KNOTS('',3,(#25697,#25698,#25699,#25700,#25701,
#25702,#25703,#25704,#25705,#25706,#25707,#25708,#25709,#25710,#25711,#25712,
#25713,#25714,#25715,#25716,#25717,#25718,#25719,#25720,#25721),
 .UNSPECIFIED.,.F.,.F.,(4,3,3,3,3,3,3,3,4),(13.8761928695312,13.9659992217611,
14.963570594744,15.9611419677269,16.9587133407099,17.9562847136928,18.9538560866757,
19.9514274596587,20.1593781767108),.UNSPECIFIED.);
#3237=B_SPLINE_CURVE_WITH_KNOTS('',3,(#25722,#25723,#25724,#25725,#25726,
#25727,#25728,#25729,#25730,#25731,#25732,#25733,#25734,#25735,#25736,#25737,
#25738,#25739,#25740,#25741,#25742,#25743),.UNSPECIFIED.,.F.,.F.,(4,3,3,
3,3,3,3,4),(-16.4127538780515,-15.9611419677269,-14.963570594744,-13.9659992217611,
-12.9684278487781,-11.9708564757952,-10.9732851028123,-10.1295685708719),
 .UNSPECIFIED.);
#3238=B_SPLINE_CURVE_WITH_KNOTS('',3,(#25749,#25750,#25751,#25752,#25753,
#25754,#25755,#25756,#25757,#25758,#25759,#25760,#25761),.UNSPECIFIED.,
 .F.,.F.,(4,3,3,3,4),(-3.8463832636923,-2.9927141189488,-1.99514274596586,
-0.997571372982932,0.),.UNSPECIFIED.);
#3239=B_SPLINE_CURVE_WITH_KNOTS('',3,(#25764,#25765,#25766,#25767,#25768,
#25769,#25770,#25771,#25772,#25773,#25774,#25775,#25776,#25777,#25778,#25779,
#25780,#25781,#25782),.UNSPECIFIED.,.F.,.F.,(4,3,3,3,3,3,4),(2.01461286527445,
2.9927141189488,3.99028549193173,4.98785686491466,5.98542823789759,6.98299961088053,
7.59300756235161),.UNSPECIFIED.);
#3240=B_SPLINE_CURVE_WITH_KNOTS('',3,(#25788,#25789,#25790,#25791,#25792,
#25793,#25794),.UNSPECIFIED.,.F.,.F.,(4,1,1,1,4),(91.106186954104,91.6672898428912,
92.6648612158741,93.6624325888571,94.66000396184),.UNSPECIFIED.);
#3241=B_SPLINE_CURVE_WITH_KNOTS('',3,(#25797,#25798,#25799,#25800,#25801,
#25802,#25803,#25804),.UNSPECIFIED.,.F.,.F.,(4,1,1,1,1,4),(91.106186954104,
91.2111367324627,92.2087081054456,93.2062794784285,94.2038508514115,95.1819521050858),
 .UNSPECIFIED.);
#3242=B_SPLINE_CURVE_WITH_KNOTS('',3,(#25809,#25810,#25811,#25812,#25813,
#25814,#25815,#25816,#25817,#25818),.UNSPECIFIED.,.F.,.F.,(4,1,1,1,1,1,
1,4),(84.8230016469244,85.6818616049936,86.6794329779765,87.6770043509595,
88.6745757239424,89.6721470969253,90.6697184699083,91.106186954104),
 .UNSPECIFIED.);
#3243=B_SPLINE_CURVE_WITH_KNOTS('',3,(#25819,#25820,#25821,#25822,#25823,
#25824,#25825,#25826,#25827,#25828),.UNSPECIFIED.,.F.,.F.,(4,1,1,1,1,1,
1,4),(84.8230016469244,85.2257084945651,86.223279867548,87.2208512405309,
88.2184226135139,89.2159939864968,90.2135653594797,91.106186954104),
 .UNSPECIFIED.);
#3244=B_SPLINE_CURVE_WITH_KNOTS('',3,(#25833,#25834,#25835,#25836,#25837,
#25838,#25839,#25840,#25841,#25842,#25843),.UNSPECIFIED.,.F.,.F.,(4,1,1,
1,1,1,1,1,4),(78.5398163397448,78.6988619941131,79.696433367096,80.6940047400789,
81.6915761130619,82.6891474860448,83.6867188590277,84.6842902320107,84.8230016469244),
 .UNSPECIFIED.);
#3245=B_SPLINE_CURVE_WITH_KNOTS('',3,(#25844,#25845,#25846,#25847,#25848,
#25849,#25850,#25851,#25852,#25853),.UNSPECIFIED.,.F.,.F.,(4,1,1,1,1,1,
1,4),(78.5398163397448,79.2402802566675,80.2378516296504,81.2354230026333,
82.2329943756163,83.2305657485992,84.2281371215821,84.8230016469244),
 .UNSPECIFIED.);
#3246=B_SPLINE_CURVE_WITH_KNOTS('',3,(#25858,#25859,#25860,#25861,#25862,
#25863,#25864,#25865,#25866,#25867),.UNSPECIFIED.,.F.,.F.,(4,1,1,1,1,1,
1,4),(72.2566310325652,72.7134337562155,73.7110051291984,74.7085765021813,
75.7061478751643,76.7037192481472,77.7012906211301,78.5398163397448),
 .UNSPECIFIED.);
#3247=B_SPLINE_CURVE_WITH_KNOTS('',3,(#25868,#25869,#25870,#25871,#25872,
#25873,#25874,#25875,#25876,#25877,#25878),.UNSPECIFIED.,.F.,.F.,(4,1,1,
1,1,1,1,1,4),(72.2566310325652,72.2572806457869,73.2548520187699,74.2524233917528,
75.2499947647357,76.2475661377187,77.2451375107016,78.2427088836845,78.5398163397448),
 .UNSPECIFIED.);
#3248=B_SPLINE_CURVE_WITH_KNOTS('',3,(#25883,#25884,#25885,#25886,#25887,
#25888,#25889,#25890,#25891,#25892),.UNSPECIFIED.,.F.,.F.,(4,1,1,1,1,1,
1,4),(65.9734457253856,66.7280055183179,67.7255768913008,68.7231482642838,
69.7207196372667,70.7182910102496,71.7158623832325,72.2566310325652),
 .UNSPECIFIED.);
#3249=B_SPLINE_CURVE_WITH_KNOTS('',3,(#25893,#25894,#25895,#25896,#25897,
#25898,#25899,#25900,#25901,#25902),.UNSPECIFIED.,.F.,.F.,(4,1,1,1,1,1,
1,4),(65.9734457253856,66.2718524078894,67.2694237808723,68.2669951538552,
69.2645665268382,70.2621378998211,71.259709272804,72.2566310325652),
 .UNSPECIFIED.);
#3250=B_SPLINE_CURVE_WITH_KNOTS('',3,(#25907,#25908,#25909,#25910,#25911,
#25912,#25913,#25914,#25915,#25916,#25917),.UNSPECIFIED.,.F.,.F.,(4,1,1,
1,1,1,1,1,4),(59.690260418206,59.7450059074374,60.7425772804203,61.7401486534032,
62.7377200263862,63.7352913993691,64.732862772352,65.730434145335,65.9734457253856),
 .UNSPECIFIED.);
#3251=B_SPLINE_CURVE_WITH_KNOTS('',3,(#25918,#25919,#25920,#25921,#25922,
#25923,#25924,#25925,#25926,#25927),.UNSPECIFIED.,.F.,.F.,(4,1,1,1,1,1,
1,4),(59.690260418206,60.2864241699918,61.2839955429747,62.2815669159576,
63.2791382889406,64.2767096619235,65.2742810349064,65.9734457253856),
 .UNSPECIFIED.);
#3252=B_SPLINE_CURVE_WITH_KNOTS('',3,(#25932,#25933,#25934,#25935,#25936,
#25937,#25938,#25939,#25940,#25941),.UNSPECIFIED.,.F.,.F.,(4,1,1,1,1,1,
1,4),(53.4070751110264,53.7595776695398,54.7571490425227,55.7547204155056,
56.7522917884886,57.7498631614715,58.7474345344544,59.690260418206),
 .UNSPECIFIED.);
#3253=B_SPLINE_CURVE_WITH_KNOTS('',3,(#25942,#25943,#25944,#25945,#25946,
#25947,#25948,#25949,#25950,#25951),.UNSPECIFIED.,.F.,.F.,(4,1,1,1,1,1,
1,4),(53.4070751110264,54.3009959320942,55.2985673050771,56.29613867806,
57.293710051043,58.2912814240259,59.2888527970088,59.690260418206),
 .UNSPECIFIED.);
#3254=B_SPLINE_CURVE_WITH_KNOTS('',3,(#25956,#25957,#25958,#25959,#25960,
#25961,#25962,#25963,#25964,#25965),.UNSPECIFIED.,.F.,.F.,(4,1,1,1,1,1,
1,4),(47.1238898038468,47.7741494316422,48.7717208046251,49.769292177608,
50.766863550591,51.7644349235739,52.7620062965568,53.4070751110264),
 .UNSPECIFIED.);
#3255=B_SPLINE_CURVE_WITH_KNOTS('',3,(#25966,#25967,#25968,#25969,#25970,
#25971,#25972,#25973,#25974,#25975,#25976),.UNSPECIFIED.,.F.,.F.,(4,1,1,
1,1,1,1,1,4),(47.1238898038468,47.3179963212136,48.3155676941966,49.3131390671795,
50.3107104401624,51.3082818131454,52.3058531861283,53.3034245591112,53.4070751110264),
 .UNSPECIFIED.);
#3256=B_SPLINE_CURVE_WITH_KNOTS('',3,(#25981,#25982,#25983,#25984,#25985,
#25986,#25987,#25988,#25989,#25990),.UNSPECIFIED.,.F.,.F.,(4,1,1,1,1,1,
1,4),(40.8407044966673,41.7887211937446,42.7862925667275,43.7838639397104,
44.7814353126934,45.7790066856763,46.7765780586592,47.1238898038468),
 .UNSPECIFIED.);
#3257=B_SPLINE_CURVE_WITH_KNOTS('',3,(#25991,#25992,#25993,#25994,#25995,
#25996,#25997,#25998,#25999,#26000),.UNSPECIFIED.,.F.,.F.,(4,1,1,1,1,1,
1,4),(40.8407044966673,41.332568083316,42.330139456299,43.3277108292819,
44.3252822022648,45.3228535752478,46.3204249482307,47.1238898038468),
 .UNSPECIFIED.);
#3258=B_SPLINE_CURVE_WITH_KNOTS('',3,(#26005,#26006,#26007,#26008,#26009,
#26010,#26011,#26012,#26013,#26014,#26015),.UNSPECIFIED.,.F.,.F.,(4,1,1,
1,1,1,1,1,4),(34.5575191894876,34.805721582864,35.803292955847,36.8008643288299,
37.7984357018128,38.7960070747958,39.7935784477787,40.7911498207616,40.8407044966673),
 .UNSPECIFIED.);
#3259=B_SPLINE_CURVE_WITH_KNOTS('',3,(#26016,#26017,#26018,#26019,#26020,
#26021,#26022,#26023,#26024,#26025),.UNSPECIFIED.,.F.,.F.,(4,1,1,1,1,1,
1,4),(34.5575191894876,35.3471398454184,36.3447112184014,37.3422825913843,
38.3398539643672,39.3374253373502,40.3349967103331,40.8407044966673),
 .UNSPECIFIED.);
#3260=B_SPLINE_CURVE_WITH_KNOTS('',3,(#26030,#26031,#26032,#26033,#26034,
#26035,#26036,#26037,#26038,#26039),.UNSPECIFIED.,.F.,.F.,(4,1,1,1,1,1,
1,4),(28.2743338823081,28.8202933449665,29.8178647179494,30.8154360909323,
31.8130074639152,32.8105788368982,33.8081502098811,34.5575191894876),
 .UNSPECIFIED.);
#3261=B_SPLINE_CURVE_WITH_KNOTS('',3,(#26040,#26041,#26042,#26043,#26044,
#26045,#26046,#26047,#26048,#26049,#26050),.UNSPECIFIED.,.F.,.F.,(4,1,1,
1,1,1,1,1,4),(28.2743338823081,28.3641402345379,29.3617116075209,30.3592829805038,
31.3568543534867,32.3544257264696,33.3519970994526,34.3495684724355,34.5575191894876),
 .UNSPECIFIED.);
#3262=B_SPLINE_CURVE_WITH_KNOTS('',3,(#26055,#26056,#26057,#26058,#26059,
#26060,#26061,#26062,#26063,#26064),.UNSPECIFIED.,.F.,.F.,(4,1,1,1,1,1,
1,4),(21.9911485751285,22.8348651070689,23.8324364800518,24.8300078530347,
25.8275792260177,26.8251505990006,27.8227219719835,28.2743338823081),
 .UNSPECIFIED.);
#3263=B_SPLINE_CURVE_WITH_KNOTS('',3,(#26065,#26066,#26067,#26068,#26069,
#26070,#26071,#26072,#26073,#26074),.UNSPECIFIED.,.F.,.F.,(4,1,1,1,1,1,
1,4),(21.9911485751285,22.3787119966403,23.3762833696233,24.3738547426062,
25.3714261155891,26.3689974885721,27.366568861555,28.2743338823081),
 .UNSPECIFIED.);
#3264=B_SPLINE_CURVE_WITH_KNOTS('',3,(#26080,#26081,#26082,#26083,#26084),
 .UNSPECIFIED.,.F.,.F.,(4,1,4),(14.3981410127769,15.3957123857598,15.7079632679489),
 .UNSPECIFIED.);
#3265=B_SPLINE_CURVE_WITH_KNOTS('',3,(#26087,#26088,#26089,#26090,#26091),
 .UNSPECIFIED.,.F.,.F.,(4,1,4),(13.8761928695311,14.8542941232054,15.7079632679489),
 .UNSPECIFIED.);
#3266=B_SPLINE_CURVE_WITH_KNOTS('',3,(#26097,#26098,#26099,#26100,#26101,
#26102,#26103,#26104,#26105,#26106,#26107,#26108,#26109,#26110,#26111,#26112,
#26113,#26114,#26115,#26116,#26117,#26118),.UNSPECIFIED.,.F.,.F.,(4,3,3,
3,3,3,3,4),(76.7080459413271,76.8129957196858,77.8105670926687,78.8081384656517,
79.8057098386346,80.8032812116175,81.8008525846005,82.7984239575834),
 .UNSPECIFIED.);
#3267=B_SPLINE_CURVE_WITH_KNOTS('',3,(#26122,#26123,#26124,#26125,#26126,
#26127,#26128),.UNSPECIFIED.,.F.,.F.,(4,3,4),(-80.783811092309,-79.8057098386346,
-79.2446069498474),.UNSPECIFIED.);
#3268=B_SPLINE_CURVE_WITH_KNOTS('',3,(#26132,#26133,#26134,#26135,#26136,
#26137,#26138,#26139,#26140,#26141,#26142,#26143,#26144,#26145,#26146,#26147,
#26148,#26149,#26150,#26151,#26152,#26153),.UNSPECIFIED.,.F.,.F.,(4,3,3,
3,3,3,3,4),(-79.2446069498474,-78.8081384656517,-77.8105670926687,-76.8129957196858,
-75.8154243467029,-74.8178529737199,-73.820281600737,-72.9614216426678),
 .UNSPECIFIED.);
#3269=B_SPLINE_CURVE_WITH_KNOTS('',3,(#26158,#26159,#26160,#26161,#26162,
#26163,#26164,#26165,#26166,#26167,#26168,#26169,#26170,#26171,#26172,#26173,
#26174,#26175,#26176,#26177,#26178,#26179),.UNSPECIFIED.,.F.,.F.,(4,3,3,
3,3,3,3,4),(70.4248606341475,70.8275674817882,71.8251388547711,72.8227102277541,
73.820281600737,74.81785297372,75.8154243467029,76.7080459413271),
 .UNSPECIFIED.);
#3270=B_SPLINE_CURVE_WITH_KNOTS('',3,(#26180,#26181,#26182,#26183,#26184,
#26185,#26186,#26187,#26188,#26189,#26190,#26191,#26192,#26193,#26194,#26195,
#26196,#26197,#26198,#26199,#26200,#26201,#26202,#26203,#26204),
 .UNSPECIFIED.,.F.,.F.,(4,3,3,3,3,3,3,3,4),(-72.9614216426678,-72.8227102277541,
-71.8251388547711,-70.8275674817882,-69.8299961088053,-68.8324247358223,
-67.8348533628394,-66.8372819898565,-66.6782363354882),.UNSPECIFIED.);
#3271=B_SPLINE_CURVE_WITH_KNOTS('',3,(#26209,#26210,#26211,#26212,#26213,
#26214,#26215,#26216,#26217,#26218,#26219,#26220,#26221,#26222,#26223,#26224,
#26225,#26226,#26227,#26228,#26229,#26230),.UNSPECIFIED.,.F.,.F.,(4,3,3,
3,3,3,3,4),(64.1416753269679,64.8421392438906,65.8397106168735,66.8372819898565,
67.8348533628394,68.8324247358223,69.8299961088053,70.4248606341475),
 .UNSPECIFIED.);
#3272=B_SPLINE_CURVE_WITH_KNOTS('',3,(#26231,#26232,#26233,#26234,#26235,
#26236,#26237,#26238,#26239,#26240,#26241,#26242,#26243,#26244,#26245,#26246,
#26247,#26248,#26249,#26250,#26251,#26252),.UNSPECIFIED.,.F.,.F.,(4,3,3,
3,3,3,3,4),(-66.6782363354882,-65.8397106168736,-64.8421392438906,-63.8445678709077,
-62.8469964979248,-61.8494251249418,-60.8518537519589,-60.3950510283086),
 .UNSPECIFIED.);
#3273=B_SPLINE_CURVE_WITH_KNOTS('',3,(#26257,#26258,#26259,#26260,#26261,
#26262,#26263,#26264,#26265,#26266,#26267,#26268,#26269,#26270,#26271,#26272,
#26273,#26274,#26275,#26276,#26277,#26278),.UNSPECIFIED.,.F.,.F.,(4,3,3,
3,3,3,3,4),(57.8584900197883,58.856711005993,59.854282378976,60.8518537519589,
61.8494251249418,62.8469964979247,63.8445678709077,64.1416753269679),
 .UNSPECIFIED.);
#3274=B_SPLINE_CURVE_WITH_KNOTS('',3,(#26279,#26280,#26281,#26282,#26283,
#26284,#26285,#26286,#26287,#26288,#26289,#26290,#26291,#26292,#26293,#26294,
#26295,#26296,#26297,#26298,#26299,#26300),.UNSPECIFIED.,.F.,.F.,(4,3,3,
3,3,3,3,4),(-60.3950510283086,-59.854282378976,-58.856711005993,-57.8591396330101,
-56.8615682600272,-55.8639968870442,-54.8664255140613,-54.111865721129),
 .UNSPECIFIED.);
#3275=B_SPLINE_CURVE_WITH_KNOTS('',3,(#26305,#26306,#26307,#26308,#26309,
#26310,#26311,#26312,#26313,#26314,#26315,#26316,#26317,#26318,#26319,#26320,
#26321,#26322,#26323,#26324,#26325,#26326),.UNSPECIFIED.,.F.,.F.,(4,3,3,
3,3,3,3,4),(51.5753047126087,51.8737113951125,52.8712827680954,53.8688541410784,
54.8664255140613,55.8639968870442,56.8615682600272,57.8584900197883),
 .UNSPECIFIED.);
#3276=B_SPLINE_CURVE_WITH_KNOTS('',3,(#26327,#26328,#26329,#26330,#26331,
#26332,#26333,#26334,#26335,#26336,#26337,#26338,#26339,#26340,#26341,#26342,
#26343,#26344,#26345,#26346,#26347,#26348,#26349,#26350,#26351),
 .UNSPECIFIED.,.F.,.F.,(4,3,3,3,3,3,3,3,4),(-54.111865721129,-53.8688541410784,
-52.8712827680954,-51.8737113951125,-50.8761400221296,-49.8785686491466,
-48.8809972761637,-47.8834259031808,-47.8286804139494),.UNSPECIFIED.);
#3277=B_SPLINE_CURVE_WITH_KNOTS('',3,(#26356,#26357,#26358,#26359,#26360,
#26361,#26362,#26363,#26364,#26365,#26366,#26367,#26368,#26369,#26370,#26371,
#26372,#26373,#26374,#26375,#26376,#26377),.UNSPECIFIED.,.F.,.F.,(4,3,3,
3,3,3,3,4),(45.2921194054291,45.8882831572149,46.8858545301978,47.8834259031808,
48.8809972761637,49.8785686491466,50.8761400221296,51.5753047126087),
 .UNSPECIFIED.);
#3278=B_SPLINE_CURVE_WITH_KNOTS('',3,(#26378,#26379,#26380,#26381,#26382,
#26383,#26384,#26385,#26386,#26387,#26388,#26389,#26390,#26391,#26392,#26393,
#26394,#26395,#26396,#26397,#26398,#26399),.UNSPECIFIED.,.F.,.F.,(4,3,3,
3,3,3,3,4),(-47.8286804139494,-46.8858545301978,-45.8882831572149,-44.890711784232,
-43.893140411249,-42.8955690382661,-41.8979976652832,-41.5454951067698),
 .UNSPECIFIED.);
#3279=B_SPLINE_CURVE_WITH_KNOTS('',3,(#26404,#26405,#26406,#26407,#26408,
#26409,#26410,#26411,#26412,#26413,#26414,#26415,#26416,#26417,#26418,#26419,
#26420,#26421,#26422,#26423,#26424,#26425),.UNSPECIFIED.,.F.,.F.,(4,3,3,
3,3,3,3,4),(39.0089340982495,39.9028549193173,40.9004262923002,41.8979976652832,
42.8955690382661,43.893140411249,44.890711784232,45.2921194054291),
 .UNSPECIFIED.);
#3280=B_SPLINE_CURVE_WITH_KNOTS('',3,(#26426,#26427,#26428,#26429,#26430,
#26431,#26432,#26433,#26434,#26435,#26436,#26437,#26438,#26439,#26440,#26441,
#26442,#26443,#26444,#26445,#26446,#26447),.UNSPECIFIED.,.F.,.F.,(4,3,3,
3,3,3,3,4),(-41.5454951067698,-40.9004262923002,-39.9028549193173,-38.9052835463344,
-37.9077121733514,-36.9101408003685,-35.9125694273856,-35.2623097995902),
 .UNSPECIFIED.);
#3281=B_SPLINE_CURVE_WITH_KNOTS('',3,(#26452,#26453,#26454,#26455,#26456,
#26457,#26458,#26459,#26460,#26461,#26462,#26463,#26464,#26465,#26466,#26467,
#26468,#26469,#26470,#26471,#26472,#26473,#26474,#26475,#26476),
 .UNSPECIFIED.,.F.,.F.,(4,3,3,3,3,3,3,3,4),(32.7257487910699,32.9198553084368,
33.9174266814197,34.9149980544026,35.9125694273856,36.9101408003685,37.9077121733514,
38.9052835463344,39.0089340982495),.UNSPECIFIED.);
#3282=B_SPLINE_CURVE_WITH_KNOTS('',3,(#26477,#26478,#26479,#26480,#26481,
#26482,#26483,#26484,#26485,#26486,#26487,#26488,#26489,#26490,#26491,#26492,
#26493,#26494,#26495,#26496,#26497,#26498),.UNSPECIFIED.,.F.,.F.,(4,3,3,
3,3,3,3,4),(-35.2623097995902,-34.9149980544026,-33.9174266814197,-32.9198553084368,
-31.9222839354538,-30.9247125624709,-29.927141189488,-28.9791244924107),
 .UNSPECIFIED.);
#3283=B_SPLINE_CURVE_WITH_KNOTS('',3,(#26503,#26504,#26505,#26506,#26507,
#26508,#26509,#26510,#26511,#26512,#26513,#26514,#26515,#26516,#26517,#26518,
#26519,#26520,#26521,#26522,#26523,#26524),.UNSPECIFIED.,.F.,.F.,(4,3,3,
3,3,3,3,4),(26.4425634838903,26.9344270705392,27.9319984435221,28.929569816505,
29.927141189488,30.9247125624709,31.9222839354538,32.7257487910699),
 .UNSPECIFIED.);
#3284=B_SPLINE_CURVE_WITH_KNOTS('',3,(#26525,#26526,#26527,#26528,#26529,
#26530,#26531,#26532,#26533,#26534,#26535,#26536,#26537,#26538,#26539,#26540,
#26541,#26542,#26543,#26544,#26545,#26546,#26547,#26548,#26549),
 .UNSPECIFIED.,.F.,.F.,(4,3,3,3,3,3,3,3,4),(-28.9791244924107,-28.929569816505,
-27.9319984435221,-26.9344270705392,-25.9368556975563,-24.9392843245733,
-23.9417129515904,-22.9441415786074,-22.6959391852311),.UNSPECIFIED.);
#3285=B_SPLINE_CURVE_WITH_KNOTS('',3,(#26554,#26555,#26556,#26557,#26558,
#26559,#26560,#26561,#26562,#26563,#26564,#26565,#26566,#26567,#26568,#26569,
#26570,#26571,#26572,#26573,#26574,#26575),.UNSPECIFIED.,.F.,.F.,(4,3,3,
3,3,3,3,4),(20.1593781767108,20.9489988326416,21.9465702056245,22.9441415786074,
23.9417129515904,24.9392843245733,25.9368556975562,26.4425634838903),
 .UNSPECIFIED.);
#3286=B_SPLINE_CURVE_WITH_KNOTS('',3,(#26576,#26577,#26578,#26579,#26580,
#26581,#26582,#26583,#26584,#26585,#26586,#26587,#26588,#26589,#26590,#26591,
#26592,#26593,#26594,#26595,#26596,#26597),.UNSPECIFIED.,.F.,.F.,(4,3,3,
3,3,3,3,4),(-22.6959391852311,-21.9465702056245,-20.9489988326416,-19.9514274596586,
-18.9538560866757,-17.9562847136928,-16.9587133407099,-16.4127538780515),
 .UNSPECIFIED.);
#3287=B_SPLINE_CURVE_WITH_KNOTS('',3,(#26602,#26603,#26604,#26605,#26606,
#26607,#26608,#26609,#26610,#26611,#26612,#26613,#26614,#26615,#26616,#26617,
#26618,#26619,#26620,#26621,#26622,#26623,#26624,#26625,#26626),
 .UNSPECIFIED.,.F.,.F.,(4,3,3,3,3,3,3,3,4),(13.8761928695312,13.9659992217611,
14.963570594744,15.9611419677269,16.9587133407099,17.9562847136928,18.9538560866757,
19.9514274596587,20.1593781767108),.UNSPECIFIED.);
#3288=B_SPLINE_CURVE_WITH_KNOTS('',3,(#26627,#26628,#26629,#26630,#26631,
#26632,#26633,#26634,#26635,#26636,#26637,#26638,#26639,#26640,#26641,#26642,
#26643,#26644,#26645,#26646,#26647,#26648),.UNSPECIFIED.,.F.,.F.,(4,3,3,
3,3,3,3,4),(-16.4127538780515,-15.9611419677269,-14.963570594744,-13.9659992217611,
-12.9684278487781,-11.9708564757952,-10.9732851028123,-10.1295685708719),
 .UNSPECIFIED.);
#3289=B_SPLINE_CURVE_WITH_KNOTS('',3,(#26654,#26655,#26656,#26657,#26658,
#26659,#26660,#26661,#26662,#26663,#26664,#26665,#26666),.UNSPECIFIED.,
 .F.,.F.,(4,3,3,3,4),(-3.8463832636923,-2.99271411894879,-1.99514274596586,
-0.997571372982931,0.),.UNSPECIFIED.);
#3290=B_SPLINE_CURVE_WITH_KNOTS('',3,(#26669,#26670,#26671,#26672,#26673,
#26674,#26675,#26676,#26677,#26678,#26679,#26680,#26681,#26682,#26683,#26684,
#26685,#26686,#26687),.UNSPECIFIED.,.F.,.F.,(4,3,3,3,3,3,4),(2.01461286527429,
2.99271411894879,3.99028549193173,4.98785686491466,5.9854282378976,6.98299961088053,
7.59300756235157),.UNSPECIFIED.);
#3291=B_SPLINE_CURVE_WITH_KNOTS('',3,(#26693,#26694,#26695,#26696,#26697,
#26698,#26699),.UNSPECIFIED.,.F.,.F.,(4,1,1,1,4),(91.106186954104,91.6672898428912,
92.6648612158741,93.6624325888571,94.66000396184),.UNSPECIFIED.);
#3292=B_SPLINE_CURVE_WITH_KNOTS('',3,(#26702,#26703,#26704,#26705,#26706,
#26707,#26708,#26709),.UNSPECIFIED.,.F.,.F.,(4,1,1,1,1,4),(91.106186954104,
91.2111367324627,92.2087081054456,93.2062794784285,94.2038508514115,95.1819521050858),
 .UNSPECIFIED.);
#3293=B_SPLINE_CURVE_WITH_KNOTS('',3,(#26714,#26715,#26716,#26717,#26718,
#26719,#26720,#26721,#26722,#26723),.UNSPECIFIED.,.F.,.F.,(4,1,1,1,1,1,
1,4),(84.8230016469244,85.6818616049936,86.6794329779765,87.6770043509595,
88.6745757239424,89.6721470969253,90.6697184699083,91.106186954104),
 .UNSPECIFIED.);
#3294=B_SPLINE_CURVE_WITH_KNOTS('',3,(#26724,#26725,#26726,#26727,#26728,
#26729,#26730,#26731,#26732,#26733),.UNSPECIFIED.,.F.,.F.,(4,1,1,1,1,1,
1,4),(84.8230016469244,85.2257084945651,86.223279867548,87.2208512405309,
88.2184226135139,89.2159939864968,90.2135653594797,91.106186954104),
 .UNSPECIFIED.);
#3295=B_SPLINE_CURVE_WITH_KNOTS('',3,(#26738,#26739,#26740,#26741,#26742,
#26743,#26744,#26745,#26746,#26747,#26748),.UNSPECIFIED.,.F.,.F.,(4,1,1,
1,1,1,1,1,4),(78.5398163397448,78.6988619941131,79.696433367096,80.6940047400789,
81.6915761130619,82.6891474860448,83.6867188590277,84.6842902320107,84.8230016469244),
 .UNSPECIFIED.);
#3296=B_SPLINE_CURVE_WITH_KNOTS('',3,(#26749,#26750,#26751,#26752,#26753,
#26754,#26755,#26756,#26757,#26758),.UNSPECIFIED.,.F.,.F.,(4,1,1,1,1,1,
1,4),(78.5398163397448,79.2402802566675,80.2378516296504,81.2354230026333,
82.2329943756163,83.2305657485992,84.2281371215821,84.8230016469244),
 .UNSPECIFIED.);
#3297=B_SPLINE_CURVE_WITH_KNOTS('',3,(#26763,#26764,#26765,#26766,#26767,
#26768,#26769,#26770,#26771,#26772),.UNSPECIFIED.,.F.,.F.,(4,1,1,1,1,1,
1,4),(72.2566310325652,72.7134337562155,73.7110051291984,74.7085765021813,
75.7061478751643,76.7037192481472,77.7012906211301,78.5398163397448),
 .UNSPECIFIED.);
#3298=B_SPLINE_CURVE_WITH_KNOTS('',3,(#26773,#26774,#26775,#26776,#26777,
#26778,#26779,#26780,#26781,#26782,#26783),.UNSPECIFIED.,.F.,.F.,(4,1,1,
1,1,1,1,1,4),(72.2566310325652,72.2572806457869,73.2548520187699,74.2524233917528,
75.2499947647357,76.2475661377187,77.2451375107016,78.2427088836845,78.5398163397448),
 .UNSPECIFIED.);
#3299=B_SPLINE_CURVE_WITH_KNOTS('',3,(#26788,#26789,#26790,#26791,#26792,
#26793,#26794,#26795,#26796,#26797),.UNSPECIFIED.,.F.,.F.,(4,1,1,1,1,1,
1,4),(65.9734457253856,66.7280055183179,67.7255768913008,68.7231482642838,
69.7207196372667,70.7182910102496,71.7158623832325,72.2566310325652),
 .UNSPECIFIED.);
#3300=B_SPLINE_CURVE_WITH_KNOTS('',3,(#26798,#26799,#26800,#26801,#26802,
#26803,#26804,#26805,#26806,#26807),.UNSPECIFIED.,.F.,.F.,(4,1,1,1,1,1,
1,4),(65.9734457253856,66.2718524078894,67.2694237808723,68.2669951538552,
69.2645665268382,70.2621378998211,71.259709272804,72.2566310325652),
 .UNSPECIFIED.);
#3301=B_SPLINE_CURVE_WITH_KNOTS('',3,(#26812,#26813,#26814,#26815,#26816,
#26817,#26818,#26819,#26820,#26821,#26822),.UNSPECIFIED.,.F.,.F.,(4,1,1,
1,1,1,1,1,4),(59.690260418206,59.7450059074374,60.7425772804203,61.7401486534032,
62.7377200263862,63.7352913993691,64.732862772352,65.730434145335,65.9734457253856),
 .UNSPECIFIED.);
#3302=B_SPLINE_CURVE_WITH_KNOTS('',3,(#26823,#26824,#26825,#26826,#26827,
#26828,#26829,#26830,#26831,#26832),.UNSPECIFIED.,.F.,.F.,(4,1,1,1,1,1,
1,4),(59.690260418206,60.2864241699918,61.2839955429747,62.2815669159576,
63.2791382889406,64.2767096619235,65.2742810349064,65.9734457253856),
 .UNSPECIFIED.);
#3303=B_SPLINE_CURVE_WITH_KNOTS('',3,(#26837,#26838,#26839,#26840,#26841,
#26842,#26843,#26844,#26845,#26846),.UNSPECIFIED.,.F.,.F.,(4,1,1,1,1,1,
1,4),(53.4070751110264,53.7595776695398,54.7571490425227,55.7547204155056,
56.7522917884886,57.7498631614715,58.7474345344544,59.690260418206),
 .UNSPECIFIED.);
#3304=B_SPLINE_CURVE_WITH_KNOTS('',3,(#26847,#26848,#26849,#26850,#26851,
#26852,#26853,#26854,#26855,#26856),.UNSPECIFIED.,.F.,.F.,(4,1,1,1,1,1,
1,4),(53.4070751110264,54.3009959320942,55.2985673050771,56.29613867806,
57.293710051043,58.2912814240259,59.2888527970088,59.690260418206),
 .UNSPECIFIED.);
#3305=B_SPLINE_CURVE_WITH_KNOTS('',3,(#26861,#26862,#26863,#26864,#26865,
#26866,#26867,#26868,#26869,#26870),.UNSPECIFIED.,.F.,.F.,(4,1,1,1,1,1,
1,4),(47.1238898038469,47.7741494316422,48.7717208046251,49.769292177608,
50.766863550591,51.7644349235739,52.7620062965568,53.4070751110264),
 .UNSPECIFIED.);
#3306=B_SPLINE_CURVE_WITH_KNOTS('',3,(#26871,#26872,#26873,#26874,#26875,
#26876,#26877,#26878,#26879,#26880,#26881),.UNSPECIFIED.,.F.,.F.,(4,1,1,
1,1,1,1,1,4),(47.1238898038468,47.3179963212136,48.3155676941966,49.3131390671795,
50.3107104401624,51.3082818131454,52.3058531861283,53.3034245591112,53.4070751110264),
 .UNSPECIFIED.);
#3307=B_SPLINE_CURVE_WITH_KNOTS('',3,(#26886,#26887,#26888,#26889,#26890,
#26891,#26892,#26893,#26894,#26895),.UNSPECIFIED.,.F.,.F.,(4,1,1,1,1,1,
1,4),(40.8407044966673,41.7887211937446,42.7862925667275,43.7838639397104,
44.7814353126934,45.7790066856763,46.7765780586592,47.1238898038469),
 .UNSPECIFIED.);
#3308=B_SPLINE_CURVE_WITH_KNOTS('',3,(#26896,#26897,#26898,#26899,#26900,
#26901,#26902,#26903,#26904,#26905),.UNSPECIFIED.,.F.,.F.,(4,1,1,1,1,1,
1,4),(40.8407044966673,41.332568083316,42.330139456299,43.3277108292819,
44.3252822022648,45.3228535752478,46.3204249482307,47.1238898038468),
 .UNSPECIFIED.);
#3309=B_SPLINE_CURVE_WITH_KNOTS('',3,(#26910,#26911,#26912,#26913,#26914,
#26915,#26916,#26917,#26918,#26919,#26920),.UNSPECIFIED.,.F.,.F.,(4,1,1,
1,1,1,1,1,4),(34.5575191894877,34.805721582864,35.803292955847,36.8008643288299,
37.7984357018128,38.7960070747958,39.7935784477787,40.7911498207616,40.8407044966673),
 .UNSPECIFIED.);
#3310=B_SPLINE_CURVE_WITH_KNOTS('',3,(#26921,#26922,#26923,#26924,#26925,
#26926,#26927,#26928,#26929,#26930),.UNSPECIFIED.,.F.,.F.,(4,1,1,1,1,1,
1,4),(34.5575191894876,35.3471398454184,36.3447112184014,37.3422825913843,
38.3398539643673,39.3374253373502,40.3349967103331,40.8407044966673),
 .UNSPECIFIED.);
#3311=B_SPLINE_CURVE_WITH_KNOTS('',3,(#26935,#26936,#26937,#26938,#26939,
#26940,#26941,#26942,#26943,#26944),.UNSPECIFIED.,.F.,.F.,(4,1,1,1,1,1,
1,4),(28.2743338823081,28.8202933449664,29.8178647179494,30.8154360909323,
31.8130074639152,32.8105788368982,33.8081502098811,34.5575191894877),
 .UNSPECIFIED.);
#3312=B_SPLINE_CURVE_WITH_KNOTS('',3,(#26945,#26946,#26947,#26948,#26949,
#26950,#26951,#26952,#26953,#26954,#26955),.UNSPECIFIED.,.F.,.F.,(4,1,1,
1,1,1,1,1,4),(28.2743338823081,28.3641402345379,29.3617116075209,30.3592829805038,
31.3568543534867,32.3544257264696,33.3519970994526,34.3495684724355,34.5575191894876),
 .UNSPECIFIED.);
#3313=B_SPLINE_CURVE_WITH_KNOTS('',3,(#26960,#26961,#26962,#26963,#26964,
#26965,#26966,#26967,#26968,#26969),.UNSPECIFIED.,.F.,.F.,(4,1,1,1,1,1,
1,4),(21.9911485751285,22.8348651070689,23.8324364800518,24.8300078530347,
25.8275792260177,26.8251505990006,27.8227219719835,28.2743338823081),
 .UNSPECIFIED.);
#3314=B_SPLINE_CURVE_WITH_KNOTS('',3,(#26970,#26971,#26972,#26973,#26974,
#26975,#26976,#26977,#26978,#26979),.UNSPECIFIED.,.F.,.F.,(4,1,1,1,1,1,
1,4),(21.9911485751285,22.3787119966403,23.3762833696233,24.3738547426062,
25.3714261155891,26.3689974885721,27.366568861555,28.2743338823081),
 .UNSPECIFIED.);
#3315=B_SPLINE_CURVE_WITH_KNOTS('',3,(#26985,#26986,#26987,#26988,#26989),
 .UNSPECIFIED.,.F.,.F.,(4,1,4),(14.3981410127769,15.3957123857598,15.7079632679489),
 .UNSPECIFIED.);
#3316=B_SPLINE_CURVE_WITH_KNOTS('',3,(#26992,#26993,#26994,#26995,#26996),
 .UNSPECIFIED.,.F.,.F.,(4,1,4),(13.8761928695311,14.8542941232054,15.7079632679489),
 .UNSPECIFIED.);
#3317=B_SPLINE_CURVE_WITH_KNOTS('',3,(#27002,#27003,#27004,#27005,#27006,
#27007,#27008,#27009,#27010,#27011,#27012,#27013,#27014,#27015,#27016,#27017,
#27018,#27019,#27020,#27021,#27022,#27023),.UNSPECIFIED.,.F.,.F.,(4,3,3,
3,3,3,3,4),(76.708045941327,76.8129957196858,77.8105670926687,78.8081384656517,
79.8057098386346,80.8032812116175,81.8008525846005,82.7984239575834),
 .UNSPECIFIED.);
#3318=B_SPLINE_CURVE_WITH_KNOTS('',3,(#27027,#27028,#27029,#27030,#27031,
#27032,#27033),.UNSPECIFIED.,.F.,.F.,(4,3,4),(-80.7838110923089,-79.8057098386346,
-79.2446069498474),.UNSPECIFIED.);
#3319=B_SPLINE_CURVE_WITH_KNOTS('',3,(#27037,#27038,#27039,#27040,#27041,
#27042,#27043,#27044,#27045,#27046,#27047,#27048,#27049,#27050,#27051,#27052,
#27053,#27054,#27055,#27056,#27057,#27058),.UNSPECIFIED.,.F.,.F.,(4,3,3,
3,3,3,3,4),(-79.2446069498474,-78.8081384656517,-77.8105670926687,-76.8129957196858,
-75.8154243467029,-74.8178529737199,-73.820281600737,-72.9614216426678),
 .UNSPECIFIED.);
#3320=B_SPLINE_CURVE_WITH_KNOTS('',3,(#27063,#27064,#27065,#27066,#27067,
#27068,#27069,#27070,#27071,#27072,#27073,#27074,#27075,#27076,#27077,#27078,
#27079,#27080,#27081,#27082,#27083,#27084),.UNSPECIFIED.,.F.,.F.,(4,3,3,
3,3,3,3,4),(70.4248606341474,70.8275674817882,71.8251388547711,72.8227102277541,
73.820281600737,74.8178529737199,75.8154243467029,76.708045941327),
 .UNSPECIFIED.);
#3321=B_SPLINE_CURVE_WITH_KNOTS('',3,(#27085,#27086,#27087,#27088,#27089,
#27090,#27091,#27092,#27093,#27094,#27095,#27096,#27097,#27098,#27099,#27100,
#27101,#27102,#27103,#27104,#27105,#27106,#27107,#27108,#27109),
 .UNSPECIFIED.,.F.,.F.,(4,3,3,3,3,3,3,3,4),(-72.9614216426678,-72.8227102277541,
-71.8251388547712,-70.8275674817882,-69.8299961088053,-68.8324247358223,
-67.8348533628394,-66.8372819898565,-66.6782363354882),.UNSPECIFIED.);
#3322=B_SPLINE_CURVE_WITH_KNOTS('',3,(#27114,#27115,#27116,#27117,#27118,
#27119,#27120,#27121,#27122,#27123,#27124,#27125,#27126,#27127,#27128,#27129,
#27130,#27131,#27132,#27133,#27134,#27135),.UNSPECIFIED.,.F.,.F.,(4,3,3,
3,3,3,3,4),(64.1416753269678,64.8421392438906,65.8397106168735,66.8372819898565,
67.8348533628394,68.8324247358223,69.8299961088053,70.4248606341474),
 .UNSPECIFIED.);
#3323=B_SPLINE_CURVE_WITH_KNOTS('',3,(#27136,#27137,#27138,#27139,#27140,
#27141,#27142,#27143,#27144,#27145,#27146,#27147,#27148,#27149,#27150,#27151,
#27152,#27153,#27154,#27155,#27156,#27157),.UNSPECIFIED.,.F.,.F.,(4,3,3,
3,3,3,3,4),(-66.6782363354882,-65.8397106168735,-64.8421392438906,-63.8445678709077,
-62.8469964979248,-61.8494251249418,-60.8518537519589,-60.3950510283086),
 .UNSPECIFIED.);
#3324=B_SPLINE_CURVE_WITH_KNOTS('',3,(#27162,#27163,#27164,#27165,#27166,
#27167,#27168,#27169,#27170,#27171,#27172,#27173,#27174,#27175,#27176,#27177,
#27178,#27179,#27180,#27181,#27182,#27183),.UNSPECIFIED.,.F.,.F.,(4,3,3,
3,3,3,3,4),(57.8584900197882,58.856711005993,59.854282378976,60.8518537519589,
61.8494251249418,62.8469964979247,63.8445678709077,64.1416753269678),
 .UNSPECIFIED.);
#3325=B_SPLINE_CURVE_WITH_KNOTS('',3,(#27184,#27185,#27186,#27187,#27188,
#27189,#27190,#27191,#27192,#27193,#27194,#27195,#27196,#27197,#27198,#27199,
#27200,#27201,#27202,#27203,#27204,#27205),.UNSPECIFIED.,.F.,.F.,(4,3,3,
3,3,3,3,4),(-60.3950510283086,-59.854282378976,-58.856711005993,-57.8591396330101,
-56.8615682600271,-55.8639968870442,-54.8664255140613,-54.111865721129),
 .UNSPECIFIED.);
#3326=B_SPLINE_CURVE_WITH_KNOTS('',3,(#27210,#27211,#27212,#27213,#27214,
#27215,#27216,#27217,#27218,#27219,#27220,#27221,#27222,#27223,#27224,#27225,
#27226,#27227,#27228,#27229,#27230,#27231),.UNSPECIFIED.,.F.,.F.,(4,3,3,
3,3,3,3,4),(51.5753047126087,51.8737113951125,52.8712827680954,53.8688541410784,
54.8664255140613,55.8639968870442,56.8615682600272,57.8584900197882),
 .UNSPECIFIED.);
#3327=B_SPLINE_CURVE_WITH_KNOTS('',3,(#27232,#27233,#27234,#27235,#27236,
#27237,#27238,#27239,#27240,#27241,#27242,#27243,#27244,#27245,#27246,#27247,
#27248,#27249,#27250,#27251,#27252,#27253,#27254,#27255,#27256),
 .UNSPECIFIED.,.F.,.F.,(4,3,3,3,3,3,3,3,4),(-54.111865721129,-53.8688541410783,
-52.8712827680954,-51.8737113951125,-50.8761400221296,-49.8785686491466,
-48.8809972761637,-47.8834259031808,-47.8286804139494),.UNSPECIFIED.);
#3328=B_SPLINE_CURVE_WITH_KNOTS('',3,(#27261,#27262,#27263,#27264,#27265,
#27266,#27267,#27268,#27269,#27270,#27271,#27272,#27273,#27274,#27275,#27276,
#27277,#27278,#27279,#27280,#27281,#27282),.UNSPECIFIED.,.F.,.F.,(4,3,3,
3,3,3,3,4),(45.2921194054291,45.8882831572149,46.8858545301978,47.8834259031808,
48.8809972761637,49.8785686491466,50.8761400221296,51.5753047126087),
 .UNSPECIFIED.);
#3329=B_SPLINE_CURVE_WITH_KNOTS('',3,(#27283,#27284,#27285,#27286,#27287,
#27288,#27289,#27290,#27291,#27292,#27293,#27294,#27295,#27296,#27297,#27298,
#27299,#27300,#27301,#27302,#27303,#27304),.UNSPECIFIED.,.F.,.F.,(4,3,3,
3,3,3,3,4),(-47.8286804139494,-46.8858545301978,-45.8882831572149,-44.890711784232,
-43.893140411249,-42.8955690382661,-41.8979976652832,-41.5454951067698),
 .UNSPECIFIED.);
#3330=B_SPLINE_CURVE_WITH_KNOTS('',3,(#27309,#27310,#27311,#27312,#27313,
#27314,#27315,#27316,#27317,#27318,#27319,#27320,#27321,#27322,#27323,#27324,
#27325,#27326,#27327,#27328,#27329,#27330),.UNSPECIFIED.,.F.,.F.,(4,3,3,
3,3,3,3,4),(39.0089340982495,39.9028549193173,40.9004262923002,41.8979976652832,
42.8955690382661,43.893140411249,44.890711784232,45.2921194054291),
 .UNSPECIFIED.);
#3331=B_SPLINE_CURVE_WITH_KNOTS('',3,(#27331,#27332,#27333,#27334,#27335,
#27336,#27337,#27338,#27339,#27340,#27341,#27342,#27343,#27344,#27345,#27346,
#27347,#27348,#27349,#27350,#27351,#27352),.UNSPECIFIED.,.F.,.F.,(4,3,3,
3,3,3,3,4),(-41.5454951067698,-40.9004262923002,-39.9028549193173,-38.9052835463344,
-37.9077121733514,-36.9101408003685,-35.9125694273856,-35.2623097995902),
 .UNSPECIFIED.);
#3332=B_SPLINE_CURVE_WITH_KNOTS('',3,(#27357,#27358,#27359,#27360,#27361,
#27362,#27363,#27364,#27365,#27366,#27367,#27368,#27369,#27370,#27371,#27372,
#27373,#27374,#27375,#27376,#27377,#27378,#27379,#27380,#27381),
 .UNSPECIFIED.,.F.,.F.,(4,3,3,3,3,3,3,3,4),(32.7257487910699,32.9198553084368,
33.9174266814197,34.9149980544026,35.9125694273856,36.9101408003685,37.9077121733514,
38.9052835463344,39.0089340982495),.UNSPECIFIED.);
#3333=B_SPLINE_CURVE_WITH_KNOTS('',3,(#27382,#27383,#27384,#27385,#27386,
#27387,#27388,#27389,#27390,#27391,#27392,#27393,#27394,#27395,#27396,#27397,
#27398,#27399,#27400,#27401,#27402,#27403),.UNSPECIFIED.,.F.,.F.,(4,3,3,
3,3,3,3,4),(-35.2623097995902,-34.9149980544026,-33.9174266814197,-32.9198553084368,
-31.9222839354538,-30.9247125624709,-29.927141189488,-28.9791244924106),
 .UNSPECIFIED.);
#3334=B_SPLINE_CURVE_WITH_KNOTS('',3,(#27408,#27409,#27410,#27411,#27412,
#27413,#27414,#27415,#27416,#27417,#27418,#27419,#27420,#27421,#27422,#27423,
#27424,#27425,#27426,#27427,#27428,#27429),.UNSPECIFIED.,.F.,.F.,(4,3,3,
3,3,3,3,4),(26.4425634838903,26.9344270705392,27.9319984435221,28.929569816505,
29.927141189488,30.9247125624709,31.9222839354538,32.7257487910699),
 .UNSPECIFIED.);
#3335=B_SPLINE_CURVE_WITH_KNOTS('',3,(#27430,#27431,#27432,#27433,#27434,
#27435,#27436,#27437,#27438,#27439,#27440,#27441,#27442,#27443,#27444,#27445,
#27446,#27447,#27448,#27449,#27450,#27451,#27452,#27453,#27454),
 .UNSPECIFIED.,.F.,.F.,(4,3,3,3,3,3,3,3,4),(-28.9791244924106,-28.929569816505,
-27.9319984435221,-26.9344270705392,-25.9368556975563,-24.9392843245733,
-23.9417129515904,-22.9441415786074,-22.695939185231),.UNSPECIFIED.);
#3336=B_SPLINE_CURVE_WITH_KNOTS('',3,(#27459,#27460,#27461,#27462,#27463,
#27464,#27465,#27466,#27467,#27468,#27469,#27470,#27471,#27472,#27473,#27474,
#27475,#27476,#27477,#27478,#27479,#27480),.UNSPECIFIED.,.F.,.F.,(4,3,3,
3,3,3,3,4),(20.1593781767107,20.9489988326416,21.9465702056245,22.9441415786074,
23.9417129515904,24.9392843245733,25.9368556975563,26.4425634838903),
 .UNSPECIFIED.);
#3337=B_SPLINE_CURVE_WITH_KNOTS('',3,(#27481,#27482,#27483,#27484,#27485,
#27486,#27487,#27488,#27489,#27490,#27491,#27492,#27493,#27494,#27495,#27496,
#27497,#27498,#27499,#27500,#27501,#27502),.UNSPECIFIED.,.F.,.F.,(4,3,3,
3,3,3,3,4),(-22.695939185231,-21.9465702056245,-20.9489988326416,-19.9514274596586,
-18.9538560866757,-17.9562847136928,-16.9587133407099,-16.4127538780514),
 .UNSPECIFIED.);
#3338=B_SPLINE_CURVE_WITH_KNOTS('',3,(#27507,#27508,#27509,#27510,#27511,
#27512,#27513,#27514,#27515,#27516,#27517,#27518,#27519,#27520,#27521,#27522,
#27523,#27524,#27525,#27526,#27527,#27528,#27529,#27530,#27531),
 .UNSPECIFIED.,.F.,.F.,(4,3,3,3,3,3,3,3,4),(13.8761928695311,13.9659992217611,
14.963570594744,15.9611419677269,16.9587133407099,17.9562847136928,18.9538560866757,
19.9514274596586,20.1593781767107),.UNSPECIFIED.);
#3339=B_SPLINE_CURVE_WITH_KNOTS('',3,(#27532,#27533,#27534,#27535,#27536,
#27537,#27538,#27539,#27540,#27541,#27542,#27543,#27544,#27545,#27546,#27547,
#27548,#27549,#27550,#27551,#27552,#27553),.UNSPECIFIED.,.F.,.F.,(4,3,3,
3,3,3,3,4),(-16.4127538780514,-15.9611419677269,-14.963570594744,-13.9659992217611,
-12.9684278487781,-11.9708564757952,-10.9732851028123,-10.1295685708719),
 .UNSPECIFIED.);
#3340=B_SPLINE_CURVE_WITH_KNOTS('',3,(#27559,#27560,#27561,#27562,#27563,
#27564,#27565,#27566,#27567,#27568,#27569,#27570,#27571),.UNSPECIFIED.,
 .F.,.F.,(4,3,3,3,4),(-3.84638326369226,-2.9927141189488,-1.99514274596587,
-0.997571372982933,0.),.UNSPECIFIED.);
#3341=B_SPLINE_CURVE_WITH_KNOTS('',3,(#27574,#27575,#27576,#27577,#27578,
#27579,#27580,#27581,#27582,#27583,#27584,#27585,#27586,#27587,#27588,#27589,
#27590,#27591,#27592),.UNSPECIFIED.,.F.,.F.,(4,3,3,3,3,3,4),(2.01461286527445,
2.9927141189488,3.99028549193173,4.98785686491466,5.9854282378976,6.98299961088053,
7.59300756235153),.UNSPECIFIED.);
#3342=B_SPLINE_CURVE_WITH_KNOTS('',3,(#27598,#27599,#27600,#27601,#27602,
#27603,#27604),.UNSPECIFIED.,.F.,.F.,(4,1,1,1,4),(91.106186954104,91.6672898428912,
92.6648612158742,93.6624325888571,94.66000396184),.UNSPECIFIED.);
#3343=B_SPLINE_CURVE_WITH_KNOTS('',3,(#27607,#27608,#27609,#27610,#27611,
#27612,#27613,#27614),.UNSPECIFIED.,.F.,.F.,(4,1,1,1,1,4),(91.106186954104,
91.2111367324627,92.2087081054456,93.2062794784286,94.2038508514115,95.1819521050858),
 .UNSPECIFIED.);
#3344=B_SPLINE_CURVE_WITH_KNOTS('',3,(#27619,#27620,#27621,#27622,#27623,
#27624,#27625,#27626,#27627,#27628),.UNSPECIFIED.,.F.,.F.,(4,1,1,1,1,1,
1,4),(84.8230016469244,85.6818616049936,86.6794329779766,87.6770043509595,
88.6745757239424,89.6721470969254,90.6697184699083,91.106186954104),
 .UNSPECIFIED.);
#3345=B_SPLINE_CURVE_WITH_KNOTS('',3,(#27629,#27630,#27631,#27632,#27633,
#27634,#27635,#27636,#27637,#27638),.UNSPECIFIED.,.F.,.F.,(4,1,1,1,1,1,
1,4),(84.8230016469244,85.2257084945651,86.223279867548,87.220851240531,
88.2184226135139,89.2159939864968,90.2135653594798,91.106186954104),
 .UNSPECIFIED.);
#3346=B_SPLINE_CURVE_WITH_KNOTS('',3,(#27643,#27644,#27645,#27646,#27647,
#27648,#27649,#27650,#27651,#27652,#27653),.UNSPECIFIED.,.F.,.F.,(4,1,1,
1,1,1,1,1,4),(78.5398163397448,78.6988619941131,79.696433367096,80.694004740079,
81.6915761130619,82.6891474860448,83.6867188590278,84.6842902320107,84.8230016469244),
 .UNSPECIFIED.);
#3347=B_SPLINE_CURVE_WITH_KNOTS('',3,(#27654,#27655,#27656,#27657,#27658,
#27659,#27660,#27661,#27662,#27663),.UNSPECIFIED.,.F.,.F.,(4,1,1,1,1,1,
1,4),(78.5398163397448,79.2402802566675,80.2378516296505,81.2354230026334,
82.2329943756163,83.2305657485992,84.2281371215822,84.8230016469244),
 .UNSPECIFIED.);
#3348=B_SPLINE_CURVE_WITH_KNOTS('',3,(#27668,#27669,#27670,#27671,#27672,
#27673,#27674,#27675,#27676,#27677),.UNSPECIFIED.,.F.,.F.,(4,1,1,1,1,1,
1,4),(72.2566310325652,72.7134337562155,73.7110051291985,74.7085765021814,
75.7061478751643,76.7037192481473,77.7012906211302,78.5398163397448),
 .UNSPECIFIED.);
#3349=B_SPLINE_CURVE_WITH_KNOTS('',3,(#27678,#27679,#27680,#27681,#27682,
#27683,#27684,#27685,#27686,#27687,#27688),.UNSPECIFIED.,.F.,.F.,(4,1,1,
1,1,1,1,1,4),(72.2566310325652,72.257280645787,73.2548520187699,74.2524233917529,
75.2499947647358,76.2475661377187,77.2451375107017,78.2427088836846,78.5398163397448),
 .UNSPECIFIED.);
#3350=B_SPLINE_CURVE_WITH_KNOTS('',3,(#27693,#27694,#27695,#27696,#27697,
#27698,#27699,#27700,#27701,#27702),.UNSPECIFIED.,.F.,.F.,(4,1,1,1,1,1,
1,4),(65.9734457253856,66.7280055183179,67.7255768913009,68.7231482642838,
69.7207196372667,70.7182910102497,71.7158623832326,72.2566310325652),
 .UNSPECIFIED.);
#3351=B_SPLINE_CURVE_WITH_KNOTS('',3,(#27703,#27704,#27705,#27706,#27707,
#27708,#27709,#27710,#27711,#27712),.UNSPECIFIED.,.F.,.F.,(4,1,1,1,1,1,
1,4),(65.9734457253856,66.2718524078894,67.2694237808723,68.2669951538553,
69.2645665268382,70.2621378998211,71.2597092728041,72.2566310325652),
 .UNSPECIFIED.);
#3352=B_SPLINE_CURVE_WITH_KNOTS('',3,(#27717,#27718,#27719,#27720,#27721,
#27722,#27723,#27724,#27725,#27726,#27727),.UNSPECIFIED.,.F.,.F.,(4,1,1,
1,1,1,1,1,4),(59.690260418206,59.7450059074374,60.7425772804203,61.7401486534033,
62.7377200263862,63.7352913993691,64.7328627723521,65.730434145335,65.9734457253856),
 .UNSPECIFIED.);
#3353=B_SPLINE_CURVE_WITH_KNOTS('',3,(#27728,#27729,#27730,#27731,#27732,
#27733,#27734,#27735,#27736,#27737),.UNSPECIFIED.,.F.,.F.,(4,1,1,1,1,1,
1,4),(59.690260418206,60.2864241699918,61.2839955429747,62.2815669159577,
63.2791382889406,64.2767096619235,65.2742810349065,65.9734457253856),
 .UNSPECIFIED.);
#3354=B_SPLINE_CURVE_WITH_KNOTS('',3,(#27742,#27743,#27744,#27745,#27746,
#27747,#27748,#27749,#27750,#27751),.UNSPECIFIED.,.F.,.F.,(4,1,1,1,1,1,
1,4),(53.4070751110264,53.7595776695398,54.7571490425227,55.7547204155057,
56.7522917884886,57.7498631614715,58.7474345344545,59.690260418206),
 .UNSPECIFIED.);
#3355=B_SPLINE_CURVE_WITH_KNOTS('',3,(#27752,#27753,#27754,#27755,#27756,
#27757,#27758,#27759,#27760,#27761),.UNSPECIFIED.,.F.,.F.,(4,1,1,1,1,1,
1,4),(53.4070751110264,54.3009959320942,55.2985673050771,56.2961386780601,
57.293710051043,58.2912814240259,59.2888527970089,59.690260418206),
 .UNSPECIFIED.);
#3356=B_SPLINE_CURVE_WITH_KNOTS('',3,(#27766,#27767,#27768,#27769,#27770,
#27771,#27772,#27773,#27774,#27775),.UNSPECIFIED.,.F.,.F.,(4,1,1,1,1,1,
1,4),(47.1238898038468,47.7741494316422,48.7717208046251,49.7692921776081,
50.766863550591,51.7644349235739,52.7620062965569,53.4070751110264),
 .UNSPECIFIED.);
#3357=B_SPLINE_CURVE_WITH_KNOTS('',3,(#27776,#27777,#27778,#27779,#27780,
#27781,#27782,#27783,#27784,#27785,#27786),.UNSPECIFIED.,.F.,.F.,(4,1,1,
1,1,1,1,1,4),(47.1238898038468,47.3179963212137,48.3155676941966,49.3131390671795,
50.3107104401625,51.3082818131454,52.3058531861283,53.3034245591113,53.4070751110264),
 .UNSPECIFIED.);
#3358=B_SPLINE_CURVE_WITH_KNOTS('',3,(#27791,#27792,#27793,#27794,#27795,
#27796,#27797,#27798,#27799,#27800),.UNSPECIFIED.,.F.,.F.,(4,1,1,1,1,1,
1,4),(40.8407044966673,41.7887211937446,42.7862925667275,43.7838639397105,
44.7814353126934,45.7790066856763,46.7765780586593,47.1238898038468),
 .UNSPECIFIED.);
#3359=B_SPLINE_CURVE_WITH_KNOTS('',3,(#27801,#27802,#27803,#27804,#27805,
#27806,#27807,#27808,#27809,#27810),.UNSPECIFIED.,.F.,.F.,(4,1,1,1,1,1,
1,4),(40.8407044966673,41.3325680833161,42.330139456299,43.3277108292819,
44.3252822022649,45.3228535752478,46.3204249482307,47.1238898038468),
 .UNSPECIFIED.);
#3360=B_SPLINE_CURVE_WITH_KNOTS('',3,(#27815,#27816,#27817,#27818,#27819,
#27820,#27821,#27822,#27823,#27824,#27825),.UNSPECIFIED.,.F.,.F.,(4,1,1,
1,1,1,1,1,4),(34.5575191894876,34.8057215828641,35.803292955847,36.80086432883,
37.7984357018129,38.7960070747958,39.7935784477787,40.7911498207617,40.8407044966673),
 .UNSPECIFIED.);
#3361=B_SPLINE_CURVE_WITH_KNOTS('',3,(#27826,#27827,#27828,#27829,#27830,
#27831,#27832,#27833,#27834,#27835),.UNSPECIFIED.,.F.,.F.,(4,1,1,1,1,1,
1,4),(34.5575191894876,35.3471398454185,36.3447112184014,37.3422825913843,
38.3398539643673,39.3374253373502,40.3349967103332,40.8407044966673),
 .UNSPECIFIED.);
#3362=B_SPLINE_CURVE_WITH_KNOTS('',3,(#27840,#27841,#27842,#27843,#27844,
#27845,#27846,#27847,#27848,#27849),.UNSPECIFIED.,.F.,.F.,(4,1,1,1,1,1,
1,4),(28.2743338823081,28.8202933449665,29.8178647179494,30.8154360909324,
31.8130074639153,32.8105788368982,33.8081502098811,34.5575191894876),
 .UNSPECIFIED.);
#3363=B_SPLINE_CURVE_WITH_KNOTS('',3,(#27850,#27851,#27852,#27853,#27854,
#27855,#27856,#27857,#27858,#27859,#27860),.UNSPECIFIED.,.F.,.F.,(4,1,1,
1,1,1,1,1,4),(28.2743338823081,28.364140234538,29.3617116075209,30.3592829805038,
31.3568543534868,32.3544257264697,33.3519970994526,34.3495684724355,34.5575191894876),
 .UNSPECIFIED.);
#3364=B_SPLINE_CURVE_WITH_KNOTS('',3,(#27865,#27866,#27867,#27868,#27869,
#27870,#27871,#27872,#27873,#27874),.UNSPECIFIED.,.F.,.F.,(4,1,1,1,1,1,
1,4),(21.9911485751285,22.8348651070689,23.8324364800518,24.8300078530348,
25.8275792260177,26.8251505990006,27.8227219719836,28.2743338823081),
 .UNSPECIFIED.);
#3365=B_SPLINE_CURVE_WITH_KNOTS('',3,(#27875,#27876,#27877,#27878,#27879,
#27880,#27881,#27882,#27883,#27884),.UNSPECIFIED.,.F.,.F.,(4,1,1,1,1,1,
1,4),(21.9911485751285,22.3787119966404,23.3762833696233,24.3738547426062,
25.3714261155892,26.3689974885721,27.366568861555,28.2743338823081),
 .UNSPECIFIED.);
#3366=B_SPLINE_CURVE_WITH_KNOTS('',3,(#27890,#27891,#27892,#27893,#27894),
 .UNSPECIFIED.,.F.,.F.,(4,1,4),(14.3981410127769,15.3957123857598,15.7079632679489),
 .UNSPECIFIED.);
#3367=B_SPLINE_CURVE_WITH_KNOTS('',3,(#27897,#27898,#27899,#27900,#27901),
 .UNSPECIFIED.,.F.,.F.,(4,1,4),(13.8761928695311,14.8542941232054,15.7079632679489),
 .UNSPECIFIED.);
#3368=B_SPLINE_CURVE_WITH_KNOTS('',3,(#27907,#27908,#27909,#27910,#27911,
#27912,#27913,#27914,#27915,#27916,#27917,#27918,#27919,#27920,#27921,#27922,
#27923,#27924,#27925,#27926,#27927,#27928),.UNSPECIFIED.,.F.,.F.,(4,3,3,
3,3,3,3,4),(76.7080459413271,76.8129957196858,77.8105670926687,78.8081384656517,
79.8057098386346,80.8032812116175,81.8008525846005,82.7984239575834),
 .UNSPECIFIED.);
#3369=B_SPLINE_CURVE_WITH_KNOTS('',3,(#27932,#27933,#27934,#27935,#27936,
#27937,#27938),.UNSPECIFIED.,.F.,.F.,(4,3,4),(-80.7838110923091,-79.8057098386346,
-79.2446069498474),.UNSPECIFIED.);
#3370=B_SPLINE_CURVE_WITH_KNOTS('',3,(#27942,#27943,#27944,#27945,#27946,
#27947,#27948,#27949,#27950,#27951,#27952,#27953,#27954,#27955,#27956,#27957,
#27958,#27959,#27960,#27961,#27962,#27963),.UNSPECIFIED.,.F.,.F.,(4,3,3,
3,3,3,3,4),(-79.2446069498474,-78.8081384656517,-77.8105670926687,-76.8129957196858,
-75.8154243467029,-74.8178529737199,-73.820281600737,-72.9614216426678),
 .UNSPECIFIED.);
#3371=B_SPLINE_CURVE_WITH_KNOTS('',3,(#27968,#27969,#27970,#27971,#27972,
#27973,#27974,#27975,#27976,#27977,#27978,#27979,#27980,#27981,#27982,#27983,
#27984,#27985,#27986,#27987,#27988,#27989),.UNSPECIFIED.,.F.,.F.,(4,3,3,
3,3,3,3,4),(70.4248606341475,70.8275674817882,71.8251388547711,72.8227102277541,
73.820281600737,74.8178529737199,75.8154243467029,76.7080459413271),
 .UNSPECIFIED.);
#3372=B_SPLINE_CURVE_WITH_KNOTS('',3,(#27990,#27991,#27992,#27993,#27994,
#27995,#27996,#27997,#27998,#27999,#28000,#28001,#28002,#28003,#28004,#28005,
#28006,#28007,#28008,#28009,#28010,#28011,#28012,#28013,#28014),
 .UNSPECIFIED.,.F.,.F.,(4,3,3,3,3,3,3,3,4),(-72.9614216426678,-72.8227102277541,
-71.8251388547711,-70.8275674817882,-69.8299961088053,-68.8324247358223,
-67.8348533628394,-66.8372819898565,-66.6782363354882),.UNSPECIFIED.);
#3373=B_SPLINE_CURVE_WITH_KNOTS('',3,(#28019,#28020,#28021,#28022,#28023,
#28024,#28025,#28026,#28027,#28028,#28029,#28030,#28031,#28032,#28033,#28034,
#28035,#28036,#28037,#28038,#28039,#28040),.UNSPECIFIED.,.F.,.F.,(4,3,3,
3,3,3,3,4),(64.1416753269679,64.8421392438906,65.8397106168735,66.8372819898565,
67.8348533628394,68.8324247358223,69.8299961088053,70.4248606341475),
 .UNSPECIFIED.);
#3374=B_SPLINE_CURVE_WITH_KNOTS('',3,(#28041,#28042,#28043,#28044,#28045,
#28046,#28047,#28048,#28049,#28050,#28051,#28052,#28053,#28054,#28055,#28056,
#28057,#28058,#28059,#28060,#28061,#28062),.UNSPECIFIED.,.F.,.F.,(4,3,3,
3,3,3,3,4),(-66.6782363354882,-65.8397106168736,-64.8421392438906,-63.8445678709077,
-62.8469964979247,-61.8494251249418,-60.8518537519589,-60.3950510283086),
 .UNSPECIFIED.);
#3375=B_SPLINE_CURVE_WITH_KNOTS('',3,(#28067,#28068,#28069,#28070,#28071,
#28072,#28073,#28074,#28075,#28076,#28077,#28078,#28079,#28080,#28081,#28082,
#28083,#28084,#28085,#28086,#28087,#28088),.UNSPECIFIED.,.F.,.F.,(4,3,3,
3,3,3,3,4),(57.8584900197883,58.856711005993,59.854282378976,60.8518537519589,
61.8494251249418,62.8469964979247,63.8445678709077,64.1416753269679),
 .UNSPECIFIED.);
#3376=B_SPLINE_CURVE_WITH_KNOTS('',3,(#28089,#28090,#28091,#28092,#28093,
#28094,#28095,#28096,#28097,#28098,#28099,#28100,#28101,#28102,#28103,#28104,
#28105,#28106,#28107,#28108,#28109,#28110),.UNSPECIFIED.,.F.,.F.,(4,3,3,
3,3,3,3,4),(-60.3950510283086,-59.854282378976,-58.856711005993,-57.8591396330101,
-56.8615682600272,-55.8639968870442,-54.8664255140613,-54.111865721129),
 .UNSPECIFIED.);
#3377=B_SPLINE_CURVE_WITH_KNOTS('',3,(#28115,#28116,#28117,#28118,#28119,
#28120,#28121,#28122,#28123,#28124,#28125,#28126,#28127,#28128,#28129,#28130,
#28131,#28132,#28133,#28134,#28135,#28136),.UNSPECIFIED.,.F.,.F.,(4,3,3,
3,3,3,3,4),(51.5753047126087,51.8737113951125,52.8712827680954,53.8688541410784,
54.8664255140613,55.8639968870442,56.8615682600272,57.8584900197883),
 .UNSPECIFIED.);
#3378=B_SPLINE_CURVE_WITH_KNOTS('',3,(#28137,#28138,#28139,#28140,#28141,
#28142,#28143,#28144,#28145,#28146,#28147,#28148,#28149,#28150,#28151,#28152,
#28153,#28154,#28155,#28156,#28157,#28158,#28159,#28160,#28161),
 .UNSPECIFIED.,.F.,.F.,(4,3,3,3,3,3,3,3,4),(-54.111865721129,-53.8688541410784,
-52.8712827680954,-51.8737113951125,-50.8761400221296,-49.8785686491466,
-48.8809972761637,-47.8834259031808,-47.8286804139494),.UNSPECIFIED.);
#3379=B_SPLINE_CURVE_WITH_KNOTS('',3,(#28166,#28167,#28168,#28169,#28170,
#28171,#28172,#28173,#28174,#28175,#28176,#28177,#28178,#28179,#28180,#28181,
#28182,#28183,#28184,#28185,#28186,#28187),.UNSPECIFIED.,.F.,.F.,(4,3,3,
3,3,3,3,4),(45.2921194054291,45.8882831572149,46.8858545301978,47.8834259031808,
48.8809972761637,49.8785686491466,50.8761400221296,51.5753047126087),
 .UNSPECIFIED.);
#3380=B_SPLINE_CURVE_WITH_KNOTS('',3,(#28188,#28189,#28190,#28191,#28192,
#28193,#28194,#28195,#28196,#28197,#28198,#28199,#28200,#28201,#28202,#28203,
#28204,#28205,#28206,#28207,#28208,#28209),.UNSPECIFIED.,.F.,.F.,(4,3,3,
3,3,3,3,4),(-47.8286804139494,-46.8858545301978,-45.8882831572149,-44.890711784232,
-43.893140411249,-42.8955690382661,-41.8979976652832,-41.5454951067698),
 .UNSPECIFIED.);
#3381=B_SPLINE_CURVE_WITH_KNOTS('',3,(#28214,#28215,#28216,#28217,#28218,
#28219,#28220,#28221,#28222,#28223,#28224,#28225,#28226,#28227,#28228,#28229,
#28230,#28231,#28232,#28233,#28234,#28235),.UNSPECIFIED.,.F.,.F.,(4,3,3,
3,3,3,3,4),(39.0089340982495,39.9028549193173,40.9004262923002,41.8979976652832,
42.8955690382661,43.893140411249,44.890711784232,45.2921194054291),
 .UNSPECIFIED.);
#3382=B_SPLINE_CURVE_WITH_KNOTS('',3,(#28236,#28237,#28238,#28239,#28240,
#28241,#28242,#28243,#28244,#28245,#28246,#28247,#28248,#28249,#28250,#28251,
#28252,#28253,#28254,#28255,#28256,#28257),.UNSPECIFIED.,.F.,.F.,(4,3,3,
3,3,3,3,4),(-41.5454951067698,-40.9004262923002,-39.9028549193173,-38.9052835463344,
-37.9077121733514,-36.9101408003685,-35.9125694273856,-35.2623097995902),
 .UNSPECIFIED.);
#3383=B_SPLINE_CURVE_WITH_KNOTS('',3,(#28262,#28263,#28264,#28265,#28266,
#28267,#28268,#28269,#28270,#28271,#28272,#28273,#28274,#28275,#28276,#28277,
#28278,#28279,#28280,#28281,#28282,#28283,#28284,#28285,#28286),
 .UNSPECIFIED.,.F.,.F.,(4,3,3,3,3,3,3,3,4),(32.7257487910699,32.9198553084368,
33.9174266814197,34.9149980544026,35.9125694273856,36.9101408003685,37.9077121733514,
38.9052835463344,39.0089340982495),.UNSPECIFIED.);
#3384=B_SPLINE_CURVE_WITH_KNOTS('',3,(#28287,#28288,#28289,#28290,#28291,
#28292,#28293,#28294,#28295,#28296,#28297,#28298,#28299,#28300,#28301,#28302,
#28303,#28304,#28305,#28306,#28307,#28308),.UNSPECIFIED.,.F.,.F.,(4,3,3,
3,3,3,3,4),(-35.2623097995902,-34.9149980544026,-33.9174266814197,-32.9198553084368,
-31.9222839354538,-30.9247125624709,-29.927141189488,-28.9791244924107),
 .UNSPECIFIED.);
#3385=B_SPLINE_CURVE_WITH_KNOTS('',3,(#28313,#28314,#28315,#28316,#28317,
#28318,#28319,#28320,#28321,#28322,#28323,#28324,#28325,#28326,#28327,#28328,
#28329,#28330,#28331,#28332,#28333,#28334),.UNSPECIFIED.,.F.,.F.,(4,3,3,
3,3,3,3,4),(26.4425634838903,26.9344270705392,27.9319984435221,28.9295698165051,
29.927141189488,30.9247125624709,31.9222839354538,32.7257487910699),
 .UNSPECIFIED.);
#3386=B_SPLINE_CURVE_WITH_KNOTS('',3,(#28335,#28336,#28337,#28338,#28339,
#28340,#28341,#28342,#28343,#28344,#28345,#28346,#28347,#28348,#28349,#28350,
#28351,#28352,#28353,#28354,#28355,#28356,#28357,#28358,#28359),
 .UNSPECIFIED.,.F.,.F.,(4,3,3,3,3,3,3,3,4),(-28.9791244924107,-28.929569816505,
-27.9319984435221,-26.9344270705392,-25.9368556975563,-24.9392843245733,
-23.9417129515904,-22.9441415786074,-22.6959391852311),.UNSPECIFIED.);
#3387=B_SPLINE_CURVE_WITH_KNOTS('',3,(#28364,#28365,#28366,#28367,#28368,
#28369,#28370,#28371,#28372,#28373,#28374,#28375,#28376,#28377,#28378,#28379,
#28380,#28381,#28382,#28383,#28384,#28385),.UNSPECIFIED.,.F.,.F.,(4,3,3,
3,3,3,3,4),(20.1593781767108,20.9489988326416,21.9465702056245,22.9441415786075,
23.9417129515904,24.9392843245733,25.9368556975563,26.4425634838903),
 .UNSPECIFIED.);
#3388=B_SPLINE_CURVE_WITH_KNOTS('',3,(#28386,#28387,#28388,#28389,#28390,
#28391,#28392,#28393,#28394,#28395,#28396,#28397,#28398,#28399,#28400,#28401,
#28402,#28403,#28404,#28405,#28406,#28407),.UNSPECIFIED.,.F.,.F.,(4,3,3,
3,3,3,3,4),(-22.6959391852311,-21.9465702056245,-20.9489988326416,-19.9514274596586,
-18.9538560866757,-17.9562847136928,-16.9587133407099,-16.4127538780515),
 .UNSPECIFIED.);
#3389=B_SPLINE_CURVE_WITH_KNOTS('',3,(#28412,#28413,#28414,#28415,#28416,
#28417,#28418,#28419,#28420,#28421,#28422,#28423,#28424,#28425,#28426,#28427,
#28428,#28429,#28430,#28431,#28432,#28433,#28434,#28435,#28436),
 .UNSPECIFIED.,.F.,.F.,(4,3,3,3,3,3,3,3,4),(13.8761928695312,13.9659992217611,
14.963570594744,15.9611419677269,16.9587133407099,17.9562847136928,18.9538560866757,
19.9514274596587,20.1593781767108),.UNSPECIFIED.);
#3390=B_SPLINE_CURVE_WITH_KNOTS('',3,(#28437,#28438,#28439,#28440,#28441,
#28442,#28443,#28444,#28445,#28446,#28447,#28448,#28449,#28450,#28451,#28452,
#28453,#28454,#28455,#28456,#28457,#28458),.UNSPECIFIED.,.F.,.F.,(4,3,3,
3,3,3,3,4),(-16.4127538780515,-15.9611419677269,-14.963570594744,-13.9659992217611,
-12.9684278487781,-11.9708564757952,-10.9732851028123,-10.1295685708719),
 .UNSPECIFIED.);
#3391=B_SPLINE_CURVE_WITH_KNOTS('',3,(#28464,#28465,#28466,#28467,#28468,
#28469,#28470,#28471,#28472,#28473,#28474,#28475,#28476),.UNSPECIFIED.,
 .F.,.F.,(4,3,3,3,4),(-3.8463832636923,-2.9927141189488,-1.99514274596586,
-0.997571372982932,0.),.UNSPECIFIED.);
#3392=B_SPLINE_CURVE_WITH_KNOTS('',3,(#28479,#28480,#28481,#28482,#28483,
#28484,#28485,#28486,#28487,#28488,#28489,#28490,#28491,#28492,#28493,#28494,
#28495,#28496,#28497),.UNSPECIFIED.,.F.,.F.,(4,3,3,3,3,3,4),(2.01461286527437,
2.9927141189488,3.99028549193173,4.98785686491466,5.9854282378976,6.98299961088053,
7.59300756235157),.UNSPECIFIED.);
#3393=B_SPLINE_CURVE_WITH_KNOTS('',3,(#28503,#28504,#28505,#28506,#28507,
#28508,#28509),.UNSPECIFIED.,.F.,.F.,(4,1,1,1,4),(91.106186954104,91.6672898428912,
92.6648612158741,93.6624325888571,94.66000396184),.UNSPECIFIED.);
#3394=B_SPLINE_CURVE_WITH_KNOTS('',3,(#28512,#28513,#28514,#28515,#28516,
#28517,#28518,#28519),.UNSPECIFIED.,.F.,.F.,(4,1,1,1,1,4),(91.106186954104,
91.2111367324627,92.2087081054456,93.2062794784285,94.2038508514115,95.1819521050858),
 .UNSPECIFIED.);
#3395=B_SPLINE_CURVE_WITH_KNOTS('',3,(#28524,#28525,#28526,#28527,#28528,
#28529,#28530,#28531,#28532,#28533),.UNSPECIFIED.,.F.,.F.,(4,1,1,1,1,1,
1,4),(84.8230016469244,85.6818616049936,86.6794329779765,87.6770043509595,
88.6745757239424,89.6721470969253,90.6697184699083,91.106186954104),
 .UNSPECIFIED.);
#3396=B_SPLINE_CURVE_WITH_KNOTS('',3,(#28534,#28535,#28536,#28537,#28538,
#28539,#28540,#28541,#28542,#28543),.UNSPECIFIED.,.F.,.F.,(4,1,1,1,1,1,
1,4),(84.8230016469244,85.2257084945651,86.223279867548,87.2208512405309,
88.2184226135139,89.2159939864968,90.2135653594797,91.106186954104),
 .UNSPECIFIED.);
#3397=B_SPLINE_CURVE_WITH_KNOTS('',3,(#28548,#28549,#28550,#28551,#28552,
#28553,#28554,#28555,#28556,#28557,#28558),.UNSPECIFIED.,.F.,.F.,(4,1,1,
1,1,1,1,1,4),(78.5398163397448,78.6988619941131,79.696433367096,80.6940047400789,
81.6915761130619,82.6891474860448,83.6867188590277,84.6842902320107,84.8230016469244),
 .UNSPECIFIED.);
#3398=B_SPLINE_CURVE_WITH_KNOTS('',3,(#28559,#28560,#28561,#28562,#28563,
#28564,#28565,#28566,#28567,#28568),.UNSPECIFIED.,.F.,.F.,(4,1,1,1,1,1,
1,4),(78.5398163397448,79.2402802566675,80.2378516296504,81.2354230026333,
82.2329943756163,83.2305657485992,84.2281371215821,84.8230016469244),
 .UNSPECIFIED.);
#3399=B_SPLINE_CURVE_WITH_KNOTS('',3,(#28573,#28574,#28575,#28576,#28577,
#28578,#28579,#28580,#28581,#28582),.UNSPECIFIED.,.F.,.F.,(4,1,1,1,1,1,
1,4),(72.2566310325652,72.7134337562155,73.7110051291984,74.7085765021813,
75.7061478751643,76.7037192481472,77.7012906211301,78.5398163397448),
 .UNSPECIFIED.);
#3400=B_SPLINE_CURVE_WITH_KNOTS('',3,(#28583,#28584,#28585,#28586,#28587,
#28588,#28589,#28590,#28591,#28592,#28593),.UNSPECIFIED.,.F.,.F.,(4,1,1,
1,1,1,1,1,4),(72.2566310325652,72.2572806457869,73.2548520187699,74.2524233917528,
75.2499947647357,76.2475661377187,77.2451375107016,78.2427088836845,78.5398163397448),
 .UNSPECIFIED.);
#3401=B_SPLINE_CURVE_WITH_KNOTS('',3,(#28598,#28599,#28600,#28601,#28602,
#28603,#28604,#28605,#28606,#28607),.UNSPECIFIED.,.F.,.F.,(4,1,1,1,1,1,
1,4),(65.9734457253856,66.7280055183179,67.7255768913008,68.7231482642838,
69.7207196372667,70.7182910102496,71.7158623832325,72.2566310325652),
 .UNSPECIFIED.);
#3402=B_SPLINE_CURVE_WITH_KNOTS('',3,(#28608,#28609,#28610,#28611,#28612,
#28613,#28614,#28615,#28616,#28617),.UNSPECIFIED.,.F.,.F.,(4,1,1,1,1,1,
1,4),(65.9734457253856,66.2718524078894,67.2694237808723,68.2669951538552,
69.2645665268382,70.2621378998211,71.259709272804,72.2566310325652),
 .UNSPECIFIED.);
#3403=B_SPLINE_CURVE_WITH_KNOTS('',3,(#28622,#28623,#28624,#28625,#28626,
#28627,#28628,#28629,#28630,#28631,#28632),.UNSPECIFIED.,.F.,.F.,(4,1,1,
1,1,1,1,1,4),(59.690260418206,59.7450059074374,60.7425772804203,61.7401486534032,
62.7377200263862,63.7352913993691,64.732862772352,65.730434145335,65.9734457253856),
 .UNSPECIFIED.);
#3404=B_SPLINE_CURVE_WITH_KNOTS('',3,(#28633,#28634,#28635,#28636,#28637,
#28638,#28639,#28640,#28641,#28642),.UNSPECIFIED.,.F.,.F.,(4,1,1,1,1,1,
1,4),(59.690260418206,60.2864241699918,61.2839955429747,62.2815669159576,
63.2791382889406,64.2767096619235,65.2742810349064,65.9734457253856),
 .UNSPECIFIED.);
#3405=B_SPLINE_CURVE_WITH_KNOTS('',3,(#28647,#28648,#28649,#28650,#28651,
#28652,#28653,#28654,#28655,#28656),.UNSPECIFIED.,.F.,.F.,(4,1,1,1,1,1,
1,4),(53.4070751110264,53.7595776695398,54.7571490425227,55.7547204155056,
56.7522917884886,57.7498631614715,58.7474345344544,59.690260418206),
 .UNSPECIFIED.);
#3406=B_SPLINE_CURVE_WITH_KNOTS('',3,(#28657,#28658,#28659,#28660,#28661,
#28662,#28663,#28664,#28665,#28666),.UNSPECIFIED.,.F.,.F.,(4,1,1,1,1,1,
1,4),(53.4070751110264,54.3009959320942,55.2985673050771,56.29613867806,
57.293710051043,58.2912814240259,59.2888527970088,59.690260418206),
 .UNSPECIFIED.);
#3407=B_SPLINE_CURVE_WITH_KNOTS('',3,(#28671,#28672,#28673,#28674,#28675,
#28676,#28677,#28678,#28679,#28680),.UNSPECIFIED.,.F.,.F.,(4,1,1,1,1,1,
1,4),(47.1238898038469,47.7741494316422,48.7717208046251,49.769292177608,
50.766863550591,51.7644349235739,52.7620062965568,53.4070751110264),
 .UNSPECIFIED.);
#3408=B_SPLINE_CURVE_WITH_KNOTS('',3,(#28681,#28682,#28683,#28684,#28685,
#28686,#28687,#28688,#28689,#28690,#28691),.UNSPECIFIED.,.F.,.F.,(4,1,1,
1,1,1,1,1,4),(47.1238898038468,47.3179963212136,48.3155676941966,49.3131390671795,
50.3107104401624,51.3082818131454,52.3058531861283,53.3034245591112,53.4070751110264),
 .UNSPECIFIED.);
#3409=B_SPLINE_CURVE_WITH_KNOTS('',3,(#28696,#28697,#28698,#28699,#28700,
#28701,#28702,#28703,#28704,#28705),.UNSPECIFIED.,.F.,.F.,(4,1,1,1,1,1,
1,4),(40.8407044966673,41.7887211937446,42.7862925667275,43.7838639397104,
44.7814353126934,45.7790066856763,46.7765780586592,47.1238898038469),
 .UNSPECIFIED.);
#3410=B_SPLINE_CURVE_WITH_KNOTS('',3,(#28706,#28707,#28708,#28709,#28710,
#28711,#28712,#28713,#28714,#28715),.UNSPECIFIED.,.F.,.F.,(4,1,1,1,1,1,
1,4),(40.8407044966673,41.332568083316,42.330139456299,43.3277108292819,
44.3252822022648,45.3228535752478,46.3204249482307,47.1238898038468),
 .UNSPECIFIED.);
#3411=B_SPLINE_CURVE_WITH_KNOTS('',3,(#28720,#28721,#28722,#28723,#28724,
#28725,#28726,#28727,#28728,#28729,#28730),.UNSPECIFIED.,.F.,.F.,(4,1,1,
1,1,1,1,1,4),(34.5575191894877,34.805721582864,35.803292955847,36.8008643288299,
37.7984357018128,38.7960070747958,39.7935784477787,40.7911498207616,40.8407044966673),
 .UNSPECIFIED.);
#3412=B_SPLINE_CURVE_WITH_KNOTS('',3,(#28731,#28732,#28733,#28734,#28735,
#28736,#28737,#28738,#28739,#28740),.UNSPECIFIED.,.F.,.F.,(4,1,1,1,1,1,
1,4),(34.5575191894876,35.3471398454184,36.3447112184014,37.3422825913843,
38.3398539643673,39.3374253373502,40.3349967103331,40.8407044966673),
 .UNSPECIFIED.);
#3413=B_SPLINE_CURVE_WITH_KNOTS('',3,(#28745,#28746,#28747,#28748,#28749,
#28750,#28751,#28752,#28753,#28754),.UNSPECIFIED.,.F.,.F.,(4,1,1,1,1,1,
1,4),(28.2743338823081,28.8202933449665,29.8178647179494,30.8154360909323,
31.8130074639152,32.8105788368982,33.8081502098811,34.5575191894877),
 .UNSPECIFIED.);
#3414=B_SPLINE_CURVE_WITH_KNOTS('',3,(#28755,#28756,#28757,#28758,#28759,
#28760,#28761,#28762,#28763,#28764,#28765),.UNSPECIFIED.,.F.,.F.,(4,1,1,
1,1,1,1,1,4),(28.2743338823081,28.3641402345379,29.3617116075209,30.3592829805038,
31.3568543534867,32.3544257264696,33.3519970994526,34.3495684724355,34.5575191894876),
 .UNSPECIFIED.);
#3415=B_SPLINE_CURVE_WITH_KNOTS('',3,(#28770,#28771,#28772,#28773,#28774,
#28775,#28776,#28777,#28778,#28779),.UNSPECIFIED.,.F.,.F.,(4,1,1,1,1,1,
1,4),(21.9911485751285,22.8348651070689,23.8324364800518,24.8300078530347,
25.8275792260177,26.8251505990006,27.8227219719835,28.2743338823081),
 .UNSPECIFIED.);
#3416=B_SPLINE_CURVE_WITH_KNOTS('',3,(#28780,#28781,#28782,#28783,#28784,
#28785,#28786,#28787,#28788,#28789),.UNSPECIFIED.,.F.,.F.,(4,1,1,1,1,1,
1,4),(21.9911485751285,22.3787119966403,23.3762833696233,24.3738547426062,
25.3714261155891,26.3689974885721,27.366568861555,28.2743338823081),
 .UNSPECIFIED.);
#3417=B_SPLINE_CURVE_WITH_KNOTS('',3,(#28795,#28796,#28797,#28798,#28799),
 .UNSPECIFIED.,.F.,.F.,(4,1,4),(14.3981410127769,15.3957123857598,15.7079632679489),
 .UNSPECIFIED.);
#3418=B_SPLINE_CURVE_WITH_KNOTS('',3,(#28802,#28803,#28804,#28805,#28806),
 .UNSPECIFIED.,.F.,.F.,(4,1,4),(13.8761928695311,14.8542941232054,15.7079632679489),
 .UNSPECIFIED.);
#3419=B_SPLINE_CURVE_WITH_KNOTS('',3,(#28812,#28813,#28814,#28815,#28816,
#28817,#28818,#28819,#28820,#28821,#28822,#28823,#28824,#28825,#28826,#28827,
#28828,#28829,#28830,#28831,#28832,#28833),.UNSPECIFIED.,.F.,.F.,(4,3,3,
3,3,3,3,4),(76.7080459413271,76.8129957196858,77.8105670926687,78.8081384656517,
79.8057098386346,80.8032812116175,81.8008525846005,82.7984239575834),
 .UNSPECIFIED.);
#3420=B_SPLINE_CURVE_WITH_KNOTS('',3,(#28837,#28838,#28839,#28840,#28841,
#28842,#28843),.UNSPECIFIED.,.F.,.F.,(4,3,4),(-80.783811092309,-79.8057098386346,
-79.2446069498474),.UNSPECIFIED.);
#3421=B_SPLINE_CURVE_WITH_KNOTS('',3,(#28847,#28848,#28849,#28850,#28851,
#28852,#28853,#28854,#28855,#28856,#28857,#28858,#28859,#28860,#28861,#28862,
#28863,#28864,#28865,#28866,#28867,#28868),.UNSPECIFIED.,.F.,.F.,(4,3,3,
3,3,3,3,4),(-79.2446069498474,-78.8081384656517,-77.8105670926687,-76.8129957196858,
-75.8154243467029,-74.8178529737199,-73.820281600737,-72.9614216426678),
 .UNSPECIFIED.);
#3422=B_SPLINE_CURVE_WITH_KNOTS('',3,(#28873,#28874,#28875,#28876,#28877,
#28878,#28879,#28880,#28881,#28882,#28883,#28884,#28885,#28886,#28887,#28888,
#28889,#28890,#28891,#28892,#28893,#28894),.UNSPECIFIED.,.F.,.F.,(4,3,3,
3,3,3,3,4),(70.4248606341475,70.8275674817882,71.8251388547711,72.8227102277541,
73.820281600737,74.81785297372,75.8154243467029,76.7080459413271),
 .UNSPECIFIED.);
#3423=B_SPLINE_CURVE_WITH_KNOTS('',3,(#28895,#28896,#28897,#28898,#28899,
#28900,#28901,#28902,#28903,#28904,#28905,#28906,#28907,#28908,#28909,#28910,
#28911,#28912,#28913,#28914,#28915,#28916,#28917,#28918,#28919),
 .UNSPECIFIED.,.F.,.F.,(4,3,3,3,3,3,3,3,4),(-72.9614216426678,-72.8227102277541,
-71.8251388547711,-70.8275674817882,-69.8299961088053,-68.8324247358223,
-67.8348533628394,-66.8372819898565,-66.6782363354882),.UNSPECIFIED.);
#3424=B_SPLINE_CURVE_WITH_KNOTS('',3,(#28924,#28925,#28926,#28927,#28928,
#28929,#28930,#28931,#28932,#28933,#28934,#28935,#28936,#28937,#28938,#28939,
#28940,#28941,#28942,#28943,#28944,#28945),.UNSPECIFIED.,.F.,.F.,(4,3,3,
3,3,3,3,4),(64.1416753269679,64.8421392438906,65.8397106168735,66.8372819898565,
67.8348533628394,68.8324247358223,69.8299961088053,70.4248606341475),
 .UNSPECIFIED.);
#3425=B_SPLINE_CURVE_WITH_KNOTS('',3,(#28946,#28947,#28948,#28949,#28950,
#28951,#28952,#28953,#28954,#28955,#28956,#28957,#28958,#28959,#28960,#28961,
#28962,#28963,#28964,#28965,#28966,#28967),.UNSPECIFIED.,.F.,.F.,(4,3,3,
3,3,3,3,4),(-66.6782363354882,-65.8397106168736,-64.8421392438906,-63.8445678709077,
-62.8469964979247,-61.8494251249418,-60.8518537519589,-60.3950510283086),
 .UNSPECIFIED.);
#3426=B_SPLINE_CURVE_WITH_KNOTS('',3,(#28972,#28973,#28974,#28975,#28976,
#28977,#28978,#28979,#28980,#28981,#28982,#28983,#28984,#28985,#28986,#28987,
#28988,#28989,#28990,#28991,#28992,#28993),.UNSPECIFIED.,.F.,.F.,(4,3,3,
3,3,3,3,4),(57.8584900197883,58.856711005993,59.854282378976,60.8518537519589,
61.8494251249418,62.8469964979247,63.8445678709077,64.1416753269679),
 .UNSPECIFIED.);
#3427=B_SPLINE_CURVE_WITH_KNOTS('',3,(#28994,#28995,#28996,#28997,#28998,
#28999,#29000,#29001,#29002,#29003,#29004,#29005,#29006,#29007,#29008,#29009,
#29010,#29011,#29012,#29013,#29014,#29015),.UNSPECIFIED.,.F.,.F.,(4,3,3,
3,3,3,3,4),(-60.3950510283086,-59.854282378976,-58.856711005993,-57.8591396330101,
-56.8615682600271,-55.8639968870442,-54.8664255140613,-54.111865721129),
 .UNSPECIFIED.);
#3428=B_SPLINE_CURVE_WITH_KNOTS('',3,(#29020,#29021,#29022,#29023,#29024,
#29025,#29026,#29027,#29028,#29029,#29030,#29031,#29032,#29033,#29034,#29035,
#29036,#29037,#29038,#29039,#29040,#29041),.UNSPECIFIED.,.F.,.F.,(4,3,3,
3,3,3,3,4),(51.5753047126087,51.8737113951125,52.8712827680954,53.8688541410784,
54.8664255140613,55.8639968870442,56.8615682600272,57.8584900197883),
 .UNSPECIFIED.);
#3429=B_SPLINE_CURVE_WITH_KNOTS('',3,(#29042,#29043,#29044,#29045,#29046,
#29047,#29048,#29049,#29050,#29051,#29052,#29053,#29054,#29055,#29056,#29057,
#29058,#29059,#29060,#29061,#29062,#29063,#29064,#29065,#29066),
 .UNSPECIFIED.,.F.,.F.,(4,3,3,3,3,3,3,3,4),(-54.111865721129,-53.8688541410784,
-52.8712827680954,-51.8737113951125,-50.8761400221296,-49.8785686491466,
-48.8809972761637,-47.8834259031808,-47.8286804139494),.UNSPECIFIED.);
#3430=B_SPLINE_CURVE_WITH_KNOTS('',3,(#29071,#29072,#29073,#29074,#29075,
#29076,#29077,#29078,#29079,#29080,#29081,#29082,#29083,#29084,#29085,#29086,
#29087,#29088,#29089,#29090,#29091,#29092),.UNSPECIFIED.,.F.,.F.,(4,3,3,
3,3,3,3,4),(45.2921194054291,45.8882831572149,46.8858545301978,47.8834259031808,
48.8809972761637,49.8785686491466,50.8761400221296,51.5753047126087),
 .UNSPECIFIED.);
#3431=B_SPLINE_CURVE_WITH_KNOTS('',3,(#29093,#29094,#29095,#29096,#29097,
#29098,#29099,#29100,#29101,#29102,#29103,#29104,#29105,#29106,#29107,#29108,
#29109,#29110,#29111,#29112,#29113,#29114),.UNSPECIFIED.,.F.,.F.,(4,3,3,
3,3,3,3,4),(-47.8286804139494,-46.8858545301978,-45.8882831572149,-44.890711784232,
-43.893140411249,-42.8955690382661,-41.8979976652832,-41.5454951067698),
 .UNSPECIFIED.);
#3432=B_SPLINE_CURVE_WITH_KNOTS('',3,(#29119,#29120,#29121,#29122,#29123,
#29124,#29125,#29126,#29127,#29128,#29129,#29130,#29131,#29132,#29133,#29134,
#29135,#29136,#29137,#29138,#29139,#29140),.UNSPECIFIED.,.F.,.F.,(4,3,3,
3,3,3,3,4),(39.0089340982495,39.9028549193173,40.9004262923002,41.8979976652832,
42.8955690382661,43.893140411249,44.890711784232,45.2921194054291),
 .UNSPECIFIED.);
#3433=B_SPLINE_CURVE_WITH_KNOTS('',3,(#29141,#29142,#29143,#29144,#29145,
#29146,#29147,#29148,#29149,#29150,#29151,#29152,#29153,#29154,#29155,#29156,
#29157,#29158,#29159,#29160,#29161,#29162),.UNSPECIFIED.,.F.,.F.,(4,3,3,
3,3,3,3,4),(-41.5454951067698,-40.9004262923002,-39.9028549193173,-38.9052835463344,
-37.9077121733514,-36.9101408003685,-35.9125694273856,-35.2623097995902),
 .UNSPECIFIED.);
#3434=B_SPLINE_CURVE_WITH_KNOTS('',3,(#29167,#29168,#29169,#29170,#29171,
#29172,#29173,#29174,#29175,#29176,#29177,#29178,#29179,#29180,#29181,#29182,
#29183,#29184,#29185,#29186,#29187,#29188,#29189,#29190,#29191),
 .UNSPECIFIED.,.F.,.F.,(4,3,3,3,3,3,3,3,4),(32.7257487910699,32.9198553084368,
33.9174266814197,34.9149980544026,35.9125694273856,36.9101408003685,37.9077121733514,
38.9052835463344,39.0089340982495),.UNSPECIFIED.);
#3435=B_SPLINE_CURVE_WITH_KNOTS('',3,(#29192,#29193,#29194,#29195,#29196,
#29197,#29198,#29199,#29200,#29201,#29202,#29203,#29204,#29205,#29206,#29207,
#29208,#29209,#29210,#29211,#29212,#29213),.UNSPECIFIED.,.F.,.F.,(4,3,3,
3,3,3,3,4),(-35.2623097995902,-34.9149980544026,-33.9174266814197,-32.9198553084368,
-31.9222839354538,-30.9247125624709,-29.927141189488,-28.9791244924106),
 .UNSPECIFIED.);
#3436=B_SPLINE_CURVE_WITH_KNOTS('',3,(#29218,#29219,#29220,#29221,#29222,
#29223,#29224,#29225,#29226,#29227,#29228,#29229,#29230,#29231,#29232,#29233,
#29234,#29235,#29236,#29237,#29238,#29239),.UNSPECIFIED.,.F.,.F.,(4,3,3,
3,3,3,3,4),(26.4425634838903,26.9344270705392,27.9319984435221,28.929569816505,
29.927141189488,30.9247125624709,31.9222839354538,32.7257487910699),
 .UNSPECIFIED.);
#3437=B_SPLINE_CURVE_WITH_KNOTS('',3,(#29240,#29241,#29242,#29243,#29244,
#29245,#29246,#29247,#29248,#29249,#29250,#29251,#29252,#29253,#29254,#29255,
#29256,#29257,#29258,#29259,#29260,#29261,#29262,#29263,#29264),
 .UNSPECIFIED.,.F.,.F.,(4,3,3,3,3,3,3,3,4),(-28.9791244924106,-28.929569816505,
-27.9319984435221,-26.9344270705392,-25.9368556975562,-24.9392843245733,
-23.9417129515904,-22.9441415786074,-22.6959391852311),.UNSPECIFIED.);
#3438=B_SPLINE_CURVE_WITH_KNOTS('',3,(#29269,#29270,#29271,#29272,#29273,
#29274,#29275,#29276,#29277,#29278,#29279,#29280,#29281,#29282,#29283,#29284,
#29285,#29286,#29287,#29288,#29289,#29290),.UNSPECIFIED.,.F.,.F.,(4,3,3,
3,3,3,3,4),(20.1593781767108,20.9489988326416,21.9465702056245,22.9441415786074,
23.9417129515904,24.9392843245733,25.9368556975562,26.4425634838903),
 .UNSPECIFIED.);
#3439=B_SPLINE_CURVE_WITH_KNOTS('',3,(#29291,#29292,#29293,#29294,#29295,
#29296,#29297,#29298,#29299,#29300,#29301,#29302,#29303,#29304,#29305,#29306,
#29307,#29308,#29309,#29310,#29311,#29312),.UNSPECIFIED.,.F.,.F.,(4,3,3,
3,3,3,3,4),(-22.6959391852311,-21.9465702056245,-20.9489988326416,-19.9514274596586,
-18.9538560866757,-17.9562847136928,-16.9587133407098,-16.4127538780515),
 .UNSPECIFIED.);
#3440=B_SPLINE_CURVE_WITH_KNOTS('',3,(#29317,#29318,#29319,#29320,#29321,
#29322,#29323,#29324,#29325,#29326,#29327,#29328,#29329,#29330,#29331,#29332,
#29333,#29334,#29335,#29336,#29337,#29338,#29339,#29340,#29341),
 .UNSPECIFIED.,.F.,.F.,(4,3,3,3,3,3,3,3,4),(13.8761928695311,13.9659992217611,
14.963570594744,15.9611419677269,16.9587133407098,17.9562847136928,18.9538560866757,
19.9514274596586,20.1593781767108),.UNSPECIFIED.);
#3441=B_SPLINE_CURVE_WITH_KNOTS('',3,(#29342,#29343,#29344,#29345,#29346,
#29347,#29348,#29349,#29350,#29351,#29352,#29353,#29354,#29355,#29356,#29357,
#29358,#29359,#29360,#29361,#29362,#29363),.UNSPECIFIED.,.F.,.F.,(4,3,3,
3,3,3,3,4),(-16.4127538780515,-15.9611419677269,-14.963570594744,-13.9659992217611,
-12.9684278487781,-11.9708564757952,-10.9732851028123,-10.1295685708719),
 .UNSPECIFIED.);
#3442=B_SPLINE_CURVE_WITH_KNOTS('',3,(#29369,#29370,#29371,#29372,#29373,
#29374,#29375,#29376,#29377,#29378,#29379,#29380,#29381),.UNSPECIFIED.,
 .F.,.F.,(4,3,3,3,4),(-3.8463832636923,-2.99271411894879,-1.99514274596586,
-0.997571372982927,0.),.UNSPECIFIED.);
#3443=B_SPLINE_CURVE_WITH_KNOTS('',3,(#29384,#29385,#29386,#29387,#29388,
#29389,#29390,#29391,#29392,#29393,#29394,#29395,#29396,#29397,#29398,#29399,
#29400,#29401,#29402),.UNSPECIFIED.,.F.,.F.,(4,3,3,3,3,3,4),(2.01461286527433,
2.9927141189488,3.99028549193173,4.98785686491466,5.98542823789759,6.98299961088052,
7.59300756235157),.UNSPECIFIED.);
#3444=B_SPLINE_CURVE_WITH_KNOTS('',3,(#29408,#29409,#29410,#29411,#29412,
#29413,#29414),.UNSPECIFIED.,.F.,.F.,(4,1,1,1,4),(91.106186954104,91.6672898428912,
92.6648612158741,93.6624325888571,94.66000396184),.UNSPECIFIED.);
#3445=B_SPLINE_CURVE_WITH_KNOTS('',3,(#29417,#29418,#29419,#29420,#29421,
#29422,#29423,#29424),.UNSPECIFIED.,.F.,.F.,(4,1,1,1,1,4),(91.106186954104,
91.2111367324627,92.2087081054456,93.2062794784285,94.2038508514115,95.1819521050858),
 .UNSPECIFIED.);
#3446=B_SPLINE_CURVE_WITH_KNOTS('',3,(#29429,#29430,#29431,#29432,#29433,
#29434,#29435,#29436,#29437,#29438),.UNSPECIFIED.,.F.,.F.,(4,1,1,1,1,1,
1,4),(84.8230016469244,85.6818616049936,86.6794329779765,87.6770043509595,
88.6745757239424,89.6721470969253,90.6697184699083,91.106186954104),
 .UNSPECIFIED.);
#3447=B_SPLINE_CURVE_WITH_KNOTS('',3,(#29439,#29440,#29441,#29442,#29443,
#29444,#29445,#29446,#29447,#29448),.UNSPECIFIED.,.F.,.F.,(4,1,1,1,1,1,
1,4),(84.8230016469244,85.2257084945651,86.223279867548,87.2208512405309,
88.2184226135139,89.2159939864968,90.2135653594797,91.106186954104),
 .UNSPECIFIED.);
#3448=B_SPLINE_CURVE_WITH_KNOTS('',3,(#29453,#29454,#29455,#29456,#29457,
#29458,#29459,#29460,#29461,#29462,#29463),.UNSPECIFIED.,.F.,.F.,(4,1,1,
1,1,1,1,1,4),(78.5398163397448,78.6988619941131,79.696433367096,80.6940047400789,
81.6915761130619,82.6891474860448,83.6867188590277,84.6842902320107,84.8230016469244),
 .UNSPECIFIED.);
#3449=B_SPLINE_CURVE_WITH_KNOTS('',3,(#29464,#29465,#29466,#29467,#29468,
#29469,#29470,#29471,#29472,#29473),.UNSPECIFIED.,.F.,.F.,(4,1,1,1,1,1,
1,4),(78.5398163397448,79.2402802566675,80.2378516296504,81.2354230026333,
82.2329943756163,83.2305657485992,84.2281371215821,84.8230016469244),
 .UNSPECIFIED.);
#3450=B_SPLINE_CURVE_WITH_KNOTS('',3,(#29478,#29479,#29480,#29481,#29482,
#29483,#29484,#29485,#29486,#29487),.UNSPECIFIED.,.F.,.F.,(4,1,1,1,1,1,
1,4),(72.2566310325652,72.7134337562155,73.7110051291984,74.7085765021813,
75.7061478751643,76.7037192481472,77.7012906211301,78.5398163397448),
 .UNSPECIFIED.);
#3451=B_SPLINE_CURVE_WITH_KNOTS('',3,(#29488,#29489,#29490,#29491,#29492,
#29493,#29494,#29495,#29496,#29497,#29498),.UNSPECIFIED.,.F.,.F.,(4,1,1,
1,1,1,1,1,4),(72.2566310325652,72.2572806457869,73.2548520187699,74.2524233917528,
75.2499947647357,76.2475661377187,77.2451375107016,78.2427088836845,78.5398163397448),
 .UNSPECIFIED.);
#3452=B_SPLINE_CURVE_WITH_KNOTS('',3,(#29503,#29504,#29505,#29506,#29507,
#29508,#29509,#29510,#29511,#29512),.UNSPECIFIED.,.F.,.F.,(4,1,1,1,1,1,
1,4),(65.9734457253856,66.7280055183179,67.7255768913008,68.7231482642838,
69.7207196372667,70.7182910102496,71.7158623832325,72.2566310325652),
 .UNSPECIFIED.);
#3453=B_SPLINE_CURVE_WITH_KNOTS('',3,(#29513,#29514,#29515,#29516,#29517,
#29518,#29519,#29520,#29521,#29522),.UNSPECIFIED.,.F.,.F.,(4,1,1,1,1,1,
1,4),(65.9734457253856,66.2718524078894,67.2694237808723,68.2669951538552,
69.2645665268382,70.2621378998211,71.259709272804,72.2566310325652),
 .UNSPECIFIED.);
#3454=B_SPLINE_CURVE_WITH_KNOTS('',3,(#29527,#29528,#29529,#29530,#29531,
#29532,#29533,#29534,#29535,#29536,#29537),.UNSPECIFIED.,.F.,.F.,(4,1,1,
1,1,1,1,1,4),(59.690260418206,59.7450059074374,60.7425772804203,61.7401486534032,
62.7377200263862,63.7352913993691,64.732862772352,65.730434145335,65.9734457253856),
 .UNSPECIFIED.);
#3455=B_SPLINE_CURVE_WITH_KNOTS('',3,(#29538,#29539,#29540,#29541,#29542,
#29543,#29544,#29545,#29546,#29547),.UNSPECIFIED.,.F.,.F.,(4,1,1,1,1,1,
1,4),(59.690260418206,60.2864241699918,61.2839955429747,62.2815669159576,
63.2791382889406,64.2767096619235,65.2742810349064,65.9734457253856),
 .UNSPECIFIED.);
#3456=B_SPLINE_CURVE_WITH_KNOTS('',3,(#29552,#29553,#29554,#29555,#29556,
#29557,#29558,#29559,#29560,#29561),.UNSPECIFIED.,.F.,.F.,(4,1,1,1,1,1,
1,4),(53.4070751110265,53.7595776695398,54.7571490425227,55.7547204155056,
56.7522917884886,57.7498631614715,58.7474345344544,59.690260418206),
 .UNSPECIFIED.);
#3457=B_SPLINE_CURVE_WITH_KNOTS('',3,(#29562,#29563,#29564,#29565,#29566,
#29567,#29568,#29569,#29570,#29571),.UNSPECIFIED.,.F.,.F.,(4,1,1,1,1,1,
1,4),(53.4070751110264,54.3009959320942,55.2985673050771,56.29613867806,
57.293710051043,58.2912814240259,59.2888527970088,59.690260418206),
 .UNSPECIFIED.);
#3458=B_SPLINE_CURVE_WITH_KNOTS('',3,(#29576,#29577,#29578,#29579,#29580,
#29581,#29582,#29583,#29584,#29585),.UNSPECIFIED.,.F.,.F.,(4,1,1,1,1,1,
1,4),(47.1238898038469,47.7741494316422,48.7717208046251,49.769292177608,
50.766863550591,51.7644349235739,52.7620062965568,53.4070751110265),
 .UNSPECIFIED.);
#3459=B_SPLINE_CURVE_WITH_KNOTS('',3,(#29586,#29587,#29588,#29589,#29590,
#29591,#29592,#29593,#29594,#29595,#29596),.UNSPECIFIED.,.F.,.F.,(4,1,1,
1,1,1,1,1,4),(47.1238898038468,47.3179963212136,48.3155676941966,49.3131390671795,
50.3107104401624,51.3082818131454,52.3058531861283,53.3034245591112,53.4070751110264),
 .UNSPECIFIED.);
#3460=B_SPLINE_CURVE_WITH_KNOTS('',3,(#29601,#29602,#29603,#29604,#29605,
#29606,#29607,#29608,#29609,#29610),.UNSPECIFIED.,.F.,.F.,(4,1,1,1,1,1,
1,4),(40.8407044966673,41.7887211937446,42.7862925667275,43.7838639397104,
44.7814353126934,45.7790066856763,46.7765780586592,47.1238898038469),
 .UNSPECIFIED.);
#3461=B_SPLINE_CURVE_WITH_KNOTS('',3,(#29611,#29612,#29613,#29614,#29615,
#29616,#29617,#29618,#29619,#29620),.UNSPECIFIED.,.F.,.F.,(4,1,1,1,1,1,
1,4),(40.8407044966673,41.332568083316,42.330139456299,43.3277108292819,
44.3252822022648,45.3228535752478,46.3204249482307,47.1238898038468),
 .UNSPECIFIED.);
#3462=B_SPLINE_CURVE_WITH_KNOTS('',3,(#29625,#29626,#29627,#29628,#29629,
#29630,#29631,#29632,#29633,#29634,#29635),.UNSPECIFIED.,.F.,.F.,(4,1,1,
1,1,1,1,1,4),(34.5575191894877,34.805721582864,35.803292955847,36.8008643288299,
37.7984357018128,38.7960070747958,39.7935784477787,40.7911498207616,40.8407044966673),
 .UNSPECIFIED.);
#3463=B_SPLINE_CURVE_WITH_KNOTS('',3,(#29636,#29637,#29638,#29639,#29640,
#29641,#29642,#29643,#29644,#29645),.UNSPECIFIED.,.F.,.F.,(4,1,1,1,1,1,
1,4),(34.5575191894876,35.3471398454184,36.3447112184014,37.3422825913843,
38.3398539643672,39.3374253373502,40.3349967103331,40.8407044966673),
 .UNSPECIFIED.);
#3464=B_SPLINE_CURVE_WITH_KNOTS('',3,(#29650,#29651,#29652,#29653,#29654,
#29655,#29656,#29657,#29658,#29659),.UNSPECIFIED.,.F.,.F.,(4,1,1,1,1,1,
1,4),(28.2743338823081,28.8202933449665,29.8178647179494,30.8154360909323,
31.8130074639152,32.8105788368982,33.8081502098811,34.5575191894877),
 .UNSPECIFIED.);
#3465=B_SPLINE_CURVE_WITH_KNOTS('',3,(#29660,#29661,#29662,#29663,#29664,
#29665,#29666,#29667,#29668,#29669,#29670),.UNSPECIFIED.,.F.,.F.,(4,1,1,
1,1,1,1,1,4),(28.2743338823081,28.3641402345379,29.3617116075208,30.3592829805038,
31.3568543534867,32.3544257264696,33.3519970994526,34.3495684724355,34.5575191894876),
 .UNSPECIFIED.);
#3466=B_SPLINE_CURVE_WITH_KNOTS('',3,(#29675,#29676,#29677,#29678,#29679,
#29680,#29681,#29682,#29683,#29684),.UNSPECIFIED.,.F.,.F.,(4,1,1,1,1,1,
1,4),(21.9911485751285,22.8348651070689,23.8324364800518,24.8300078530347,
25.8275792260177,26.8251505990006,27.8227219719835,28.2743338823081),
 .UNSPECIFIED.);
#3467=B_SPLINE_CURVE_WITH_KNOTS('',3,(#29685,#29686,#29687,#29688,#29689,
#29690,#29691,#29692,#29693,#29694),.UNSPECIFIED.,.F.,.F.,(4,1,1,1,1,1,
1,4),(21.9911485751285,22.3787119966403,23.3762833696233,24.3738547426062,
25.3714261155891,26.3689974885721,27.366568861555,28.2743338823081),
 .UNSPECIFIED.);
#3468=B_SPLINE_CURVE_WITH_KNOTS('',3,(#29700,#29701,#29702,#29703,#29704),
 .UNSPECIFIED.,.F.,.F.,(4,1,4),(14.3981410127769,15.3957123857598,15.7079632679489),
 .UNSPECIFIED.);
#3469=B_SPLINE_CURVE_WITH_KNOTS('',3,(#29707,#29708,#29709,#29710,#29711),
 .UNSPECIFIED.,.F.,.F.,(4,1,4),(13.8761928695311,14.8542941232054,15.7079632679489),
 .UNSPECIFIED.);
#3470=B_SPLINE_CURVE_WITH_KNOTS('',3,(#29717,#29718,#29719,#29720,#29721,
#29722,#29723,#29724,#29725,#29726,#29727,#29728,#29729,#29730,#29731,#29732,
#29733,#29734,#29735,#29736,#29737,#29738),.UNSPECIFIED.,.F.,.F.,(4,3,3,
3,3,3,3,4),(76.708045941327,76.8129957196858,77.8105670926687,78.8081384656517,
79.8057098386346,80.8032812116175,81.8008525846005,82.7984239575834),
 .UNSPECIFIED.);
#3471=B_SPLINE_CURVE_WITH_KNOTS('',3,(#29742,#29743,#29744,#29745,#29746,
#29747,#29748),.UNSPECIFIED.,.F.,.F.,(4,3,4),(-80.7838110923089,-79.8057098386346,
-79.2446069498473),.UNSPECIFIED.);
#3472=B_SPLINE_CURVE_WITH_KNOTS('',3,(#29752,#29753,#29754,#29755,#29756,
#29757,#29758,#29759,#29760,#29761,#29762,#29763,#29764,#29765,#29766,#29767,
#29768,#29769,#29770,#29771,#29772,#29773),.UNSPECIFIED.,.F.,.F.,(4,3,3,
3,3,3,3,4),(-79.2446069498473,-78.8081384656517,-77.8105670926687,-76.8129957196858,
-75.8154243467029,-74.81785297372,-73.820281600737,-72.9614216426677),
 .UNSPECIFIED.);
#3473=B_SPLINE_CURVE_WITH_KNOTS('',3,(#29778,#29779,#29780,#29781,#29782,
#29783,#29784,#29785,#29786,#29787,#29788,#29789,#29790,#29791,#29792,#29793,
#29794,#29795,#29796,#29797,#29798,#29799),.UNSPECIFIED.,.F.,.F.,(4,3,3,
3,3,3,3,4),(70.4248606341474,70.8275674817882,71.8251388547712,72.8227102277541,
73.820281600737,74.81785297372,75.8154243467029,76.708045941327),
 .UNSPECIFIED.);
#3474=B_SPLINE_CURVE_WITH_KNOTS('',3,(#29800,#29801,#29802,#29803,#29804,
#29805,#29806,#29807,#29808,#29809,#29810,#29811,#29812,#29813,#29814,#29815,
#29816,#29817,#29818,#29819,#29820,#29821,#29822,#29823,#29824),
 .UNSPECIFIED.,.F.,.F.,(4,3,3,3,3,3,3,3,4),(-72.9614216426677,-72.8227102277541,
-71.8251388547711,-70.8275674817882,-69.8299961088053,-68.8324247358223,
-67.8348533628394,-66.8372819898565,-66.6782363354881),.UNSPECIFIED.);
#3475=B_SPLINE_CURVE_WITH_KNOTS('',3,(#29829,#29830,#29831,#29832,#29833,
#29834,#29835,#29836,#29837,#29838,#29839,#29840,#29841,#29842,#29843,#29844,
#29845,#29846,#29847,#29848,#29849,#29850),.UNSPECIFIED.,.F.,.F.,(4,3,3,
3,3,3,3,4),(64.1416753269678,64.8421392438906,65.8397106168735,66.8372819898565,
67.8348533628394,68.8324247358223,69.8299961088053,70.4248606341474),
 .UNSPECIFIED.);
#3476=B_SPLINE_CURVE_WITH_KNOTS('',3,(#29851,#29852,#29853,#29854,#29855,
#29856,#29857,#29858,#29859,#29860,#29861,#29862,#29863,#29864,#29865,#29866,
#29867,#29868,#29869,#29870,#29871,#29872),.UNSPECIFIED.,.F.,.F.,(4,3,3,
3,3,3,3,4),(-66.6782363354881,-65.8397106168735,-64.8421392438906,-63.8445678709077,
-62.8469964979248,-61.8494251249418,-60.8518537519589,-60.3950510283085),
 .UNSPECIFIED.);
#3477=B_SPLINE_CURVE_WITH_KNOTS('',3,(#29877,#29878,#29879,#29880,#29881,
#29882,#29883,#29884,#29885,#29886,#29887,#29888,#29889,#29890,#29891,#29892,
#29893,#29894,#29895,#29896,#29897,#29898),.UNSPECIFIED.,.F.,.F.,(4,3,3,
3,3,3,3,4),(57.8584900197882,58.856711005993,59.854282378976,60.8518537519589,
61.8494251249418,62.8469964979248,63.8445678709077,64.1416753269678),
 .UNSPECIFIED.);
#3478=B_SPLINE_CURVE_WITH_KNOTS('',3,(#29899,#29900,#29901,#29902,#29903,
#29904,#29905,#29906,#29907,#29908,#29909,#29910,#29911,#29912,#29913,#29914,
#29915,#29916,#29917,#29918,#29919,#29920),.UNSPECIFIED.,.F.,.F.,(4,3,3,
3,3,3,3,4),(-60.3950510283085,-59.854282378976,-58.856711005993,-57.8591396330101,
-56.8615682600272,-55.8639968870442,-54.8664255140613,-54.111865721129),
 .UNSPECIFIED.);
#3479=B_SPLINE_CURVE_WITH_KNOTS('',3,(#29925,#29926,#29927,#29928,#29929,
#29930,#29931,#29932,#29933,#29934,#29935,#29936,#29937,#29938,#29939,#29940,
#29941,#29942,#29943,#29944,#29945,#29946),.UNSPECIFIED.,.F.,.F.,(4,3,3,
3,3,3,3,4),(51.5753047126087,51.8737113951125,52.8712827680954,53.8688541410784,
54.8664255140613,55.8639968870442,56.8615682600272,57.8584900197882),
 .UNSPECIFIED.);
#3480=B_SPLINE_CURVE_WITH_KNOTS('',3,(#29947,#29948,#29949,#29950,#29951,
#29952,#29953,#29954,#29955,#29956,#29957,#29958,#29959,#29960,#29961,#29962,
#29963,#29964,#29965,#29966,#29967,#29968,#29969,#29970,#29971),
 .UNSPECIFIED.,.F.,.F.,(4,3,3,3,3,3,3,3,4),(-54.111865721129,-53.8688541410784,
-52.8712827680954,-51.8737113951125,-50.8761400221296,-49.8785686491466,
-48.8809972761637,-47.8834259031808,-47.8286804139494),.UNSPECIFIED.);
#3481=B_SPLINE_CURVE_WITH_KNOTS('',3,(#29976,#29977,#29978,#29979,#29980,
#29981,#29982,#29983,#29984,#29985,#29986,#29987,#29988,#29989,#29990,#29991,
#29992,#29993,#29994,#29995,#29996,#29997),.UNSPECIFIED.,.F.,.F.,(4,3,3,
3,3,3,3,4),(45.2921194054291,45.8882831572149,46.8858545301978,47.8834259031808,
48.8809972761637,49.8785686491466,50.8761400221296,51.5753047126087),
 .UNSPECIFIED.);
#3482=B_SPLINE_CURVE_WITH_KNOTS('',3,(#29998,#29999,#30000,#30001,#30002,
#30003,#30004,#30005,#30006,#30007,#30008,#30009,#30010,#30011,#30012,#30013,
#30014,#30015,#30016,#30017,#30018,#30019),.UNSPECIFIED.,.F.,.F.,(4,3,3,
3,3,3,3,4),(-47.8286804139494,-46.8858545301978,-45.8882831572149,-44.890711784232,
-43.893140411249,-42.8955690382661,-41.8979976652832,-41.5454951067698),
 .UNSPECIFIED.);
#3483=B_SPLINE_CURVE_WITH_KNOTS('',3,(#30024,#30025,#30026,#30027,#30028,
#30029,#30030,#30031,#30032,#30033,#30034,#30035,#30036,#30037,#30038,#30039,
#30040,#30041,#30042,#30043,#30044,#30045),.UNSPECIFIED.,.F.,.F.,(4,3,3,
3,3,3,3,4),(39.0089340982495,39.9028549193173,40.9004262923002,41.8979976652832,
42.8955690382661,43.893140411249,44.890711784232,45.2921194054291),
 .UNSPECIFIED.);
#3484=B_SPLINE_CURVE_WITH_KNOTS('',3,(#30046,#30047,#30048,#30049,#30050,
#30051,#30052,#30053,#30054,#30055,#30056,#30057,#30058,#30059,#30060,#30061,
#30062,#30063,#30064,#30065,#30066,#30067),.UNSPECIFIED.,.F.,.F.,(4,3,3,
3,3,3,3,4),(-41.5454951067698,-40.9004262923002,-39.9028549193173,-38.9052835463344,
-37.9077121733514,-36.9101408003685,-35.9125694273856,-35.2623097995902),
 .UNSPECIFIED.);
#3485=B_SPLINE_CURVE_WITH_KNOTS('',3,(#30072,#30073,#30074,#30075,#30076,
#30077,#30078,#30079,#30080,#30081,#30082,#30083,#30084,#30085,#30086,#30087,
#30088,#30089,#30090,#30091,#30092,#30093,#30094,#30095,#30096),
 .UNSPECIFIED.,.F.,.F.,(4,3,3,3,3,3,3,3,4),(32.7257487910699,32.9198553084368,
33.9174266814197,34.9149980544026,35.9125694273856,36.9101408003685,37.9077121733514,
38.9052835463344,39.0089340982495),.UNSPECIFIED.);
#3486=B_SPLINE_CURVE_WITH_KNOTS('',3,(#30097,#30098,#30099,#30100,#30101,
#30102,#30103,#30104,#30105,#30106,#30107,#30108,#30109,#30110,#30111,#30112,
#30113,#30114,#30115,#30116,#30117,#30118),.UNSPECIFIED.,.F.,.F.,(4,3,3,
3,3,3,3,4),(-35.2623097995902,-34.9149980544027,-33.9174266814197,-32.9198553084368,
-31.9222839354539,-30.9247125624709,-29.927141189488,-28.9791244924106),
 .UNSPECIFIED.);
#3487=B_SPLINE_CURVE_WITH_KNOTS('',3,(#30123,#30124,#30125,#30126,#30127,
#30128,#30129,#30130,#30131,#30132,#30133,#30134,#30135,#30136,#30137,#30138,
#30139,#30140,#30141,#30142,#30143,#30144),.UNSPECIFIED.,.F.,.F.,(4,3,3,
3,3,3,3,4),(26.4425634838903,26.9344270705392,27.9319984435221,28.929569816505,
29.927141189488,30.9247125624709,31.9222839354538,32.7257487910699),
 .UNSPECIFIED.);
#3488=B_SPLINE_CURVE_WITH_KNOTS('',3,(#30145,#30146,#30147,#30148,#30149,
#30150,#30151,#30152,#30153,#30154,#30155,#30156,#30157,#30158,#30159,#30160,
#30161,#30162,#30163,#30164,#30165,#30166,#30167,#30168,#30169),
 .UNSPECIFIED.,.F.,.F.,(4,3,3,3,3,3,3,3,4),(-28.9791244924106,-28.9295698165051,
-27.9319984435221,-26.9344270705392,-25.9368556975562,-24.9392843245733,
-23.9417129515904,-22.9441415786075,-22.695939185231),.UNSPECIFIED.);
#3489=B_SPLINE_CURVE_WITH_KNOTS('',3,(#30174,#30175,#30176,#30177,#30178,
#30179,#30180,#30181,#30182,#30183,#30184,#30185,#30186,#30187,#30188,#30189,
#30190,#30191,#30192,#30193,#30194,#30195),.UNSPECIFIED.,.F.,.F.,(4,3,3,
3,3,3,3,4),(20.1593781767107,20.9489988326416,21.9465702056245,22.9441415786074,
23.9417129515904,24.9392843245733,25.9368556975562,26.4425634838903),
 .UNSPECIFIED.);
#3490=B_SPLINE_CURVE_WITH_KNOTS('',3,(#30196,#30197,#30198,#30199,#30200,
#30201,#30202,#30203,#30204,#30205,#30206,#30207,#30208,#30209,#30210,#30211,
#30212,#30213,#30214,#30215,#30216,#30217),.UNSPECIFIED.,.F.,.F.,(4,3,3,
3,3,3,3,4),(-22.695939185231,-21.9465702056245,-20.9489988326416,-19.9514274596587,
-18.9538560866757,-17.9562847136928,-16.9587133407099,-16.4127538780514),
 .UNSPECIFIED.);
#3491=B_SPLINE_CURVE_WITH_KNOTS('',3,(#30222,#30223,#30224,#30225,#30226,
#30227,#30228,#30229,#30230,#30231,#30232,#30233,#30234,#30235,#30236,#30237,
#30238,#30239,#30240,#30241,#30242,#30243,#30244,#30245,#30246),
 .UNSPECIFIED.,.F.,.F.,(4,3,3,3,3,3,3,3,4),(13.8761928695311,13.9659992217611,
14.963570594744,15.9611419677269,16.9587133407099,17.9562847136928,18.9538560866757,
19.9514274596586,20.1593781767107),.UNSPECIFIED.);
#3492=B_SPLINE_CURVE_WITH_KNOTS('',3,(#30247,#30248,#30249,#30250,#30251,
#30252,#30253,#30254,#30255,#30256,#30257,#30258,#30259,#30260,#30261,#30262,
#30263,#30264,#30265,#30266,#30267,#30268),.UNSPECIFIED.,.F.,.F.,(4,3,3,
3,3,3,3,4),(-16.4127538780514,-15.9611419677269,-14.963570594744,-13.9659992217611,
-12.9684278487781,-11.9708564757952,-10.9732851028123,-10.1295685708718),
 .UNSPECIFIED.);
#3493=B_SPLINE_CURVE_WITH_KNOTS('',3,(#30274,#30275,#30276,#30277,#30278,
#30279,#30280,#30281,#30282,#30283,#30284,#30285,#30286),.UNSPECIFIED.,
 .F.,.F.,(4,3,3,3,4),(-3.84638326369223,-2.9927141189488,-1.99514274596587,
-0.997571372982933,0.),.UNSPECIFIED.);
#3494=B_SPLINE_CURVE_WITH_KNOTS('',3,(#30289,#30290,#30291,#30292,#30293,
#30294,#30295,#30296,#30297,#30298,#30299,#30300,#30301,#30302,#30303,#30304,
#30305,#30306,#30307),.UNSPECIFIED.,.F.,.F.,(4,3,3,3,3,3,4),(2.01461286527451,
2.9927141189488,3.99028549193173,4.98785686491466,5.98542823789759,6.98299961088052,
7.59300756235153),.UNSPECIFIED.);
#3495=B_SPLINE_CURVE_WITH_KNOTS('',3,(#30313,#30314,#30315,#30316,#30317,
#30318,#30319),.UNSPECIFIED.,.F.,.F.,(4,1,1,1,4),(91.106186954104,91.6672898428913,
92.6648612158742,93.6624325888572,94.6600039618401),.UNSPECIFIED.);
#3496=B_SPLINE_CURVE_WITH_KNOTS('',3,(#30322,#30323,#30324,#30325,#30326,
#30327,#30328,#30329),.UNSPECIFIED.,.F.,.F.,(4,1,1,1,1,4),(91.106186954104,
91.2111367324627,92.2087081054457,93.2062794784286,94.2038508514115,95.1819521050859),
 .UNSPECIFIED.);
#3497=B_SPLINE_CURVE_WITH_KNOTS('',3,(#30334,#30335,#30336,#30337,#30338,
#30339,#30340,#30341,#30342,#30343),.UNSPECIFIED.,.F.,.F.,(4,1,1,1,1,1,
1,4),(84.8230016469244,85.6818616049937,86.6794329779766,87.6770043509596,
88.6745757239425,89.6721470969254,90.6697184699084,91.106186954104),
 .UNSPECIFIED.);
#3498=B_SPLINE_CURVE_WITH_KNOTS('',3,(#30344,#30345,#30346,#30347,#30348,
#30349,#30350,#30351,#30352,#30353),.UNSPECIFIED.,.F.,.F.,(4,1,1,1,1,1,
1,4),(84.8230016469244,85.2257084945651,86.2232798675481,87.220851240531,
88.2184226135139,89.2159939864969,90.2135653594798,91.106186954104),
 .UNSPECIFIED.);
#3499=B_SPLINE_CURVE_WITH_KNOTS('',3,(#30358,#30359,#30360,#30361,#30362,
#30363,#30364,#30365,#30366,#30367,#30368),.UNSPECIFIED.,.F.,.F.,(4,1,1,
1,1,1,1,1,4),(78.5398163397448,78.6988619941132,79.6964333670961,80.694004740079,
81.691576113062,82.6891474860449,83.6867188590278,84.6842902320108,84.8230016469244),
 .UNSPECIFIED.);
#3500=B_SPLINE_CURVE_WITH_KNOTS('',3,(#30369,#30370,#30371,#30372,#30373,
#30374,#30375,#30376,#30377,#30378),.UNSPECIFIED.,.F.,.F.,(4,1,1,1,1,1,
1,4),(78.5398163397448,79.2402802566675,80.2378516296505,81.2354230026334,
82.2329943756163,83.2305657485993,84.2281371215822,84.8230016469244),
 .UNSPECIFIED.);
#3501=B_SPLINE_CURVE_WITH_KNOTS('',3,(#30383,#30384,#30385,#30386,#30387,
#30388,#30389,#30390,#30391,#30392),.UNSPECIFIED.,.F.,.F.,(4,1,1,1,1,1,
1,4),(72.2566310325652,72.7134337562156,73.7110051291985,74.7085765021814,
75.7061478751644,76.7037192481473,77.7012906211302,78.5398163397448),
 .UNSPECIFIED.);
#3502=B_SPLINE_CURVE_WITH_KNOTS('',3,(#30393,#30394,#30395,#30396,#30397,
#30398,#30399,#30400,#30401,#30402,#30403),.UNSPECIFIED.,.F.,.F.,(4,1,1,
1,1,1,1,1,4),(72.2566310325652,72.257280645787,73.25485201877,74.2524233917529,
75.2499947647358,76.2475661377187,77.2451375107017,78.2427088836846,78.5398163397448),
 .UNSPECIFIED.);
#3503=B_SPLINE_CURVE_WITH_KNOTS('',3,(#30408,#30409,#30410,#30411,#30412,
#30413,#30414,#30415,#30416,#30417),.UNSPECIFIED.,.F.,.F.,(4,1,1,1,1,1,
1,4),(65.9734457253856,66.728005518318,67.7255768913009,68.7231482642839,
69.7207196372668,70.7182910102497,71.7158623832326,72.2566310325652),
 .UNSPECIFIED.);
#3504=B_SPLINE_CURVE_WITH_KNOTS('',3,(#30418,#30419,#30420,#30421,#30422,
#30423,#30424,#30425,#30426,#30427),.UNSPECIFIED.,.F.,.F.,(4,1,1,1,1,1,
1,4),(65.9734457253856,66.2718524078894,67.2694237808724,68.2669951538553,
69.2645665268382,70.2621378998212,71.2597092728041,72.2566310325652),
 .UNSPECIFIED.);
#3505=B_SPLINE_CURVE_WITH_KNOTS('',3,(#30432,#30433,#30434,#30435,#30436,
#30437,#30438,#30439,#30440,#30441,#30442),.UNSPECIFIED.,.F.,.F.,(4,1,1,
1,1,1,1,1,4),(59.690260418206,59.7450059074374,60.7425772804204,61.7401486534033,
62.7377200263862,63.7352913993692,64.7328627723521,65.7304341453351,65.9734457253856),
 .UNSPECIFIED.);
#3506=B_SPLINE_CURVE_WITH_KNOTS('',3,(#30443,#30444,#30445,#30446,#30447,
#30448,#30449,#30450,#30451,#30452),.UNSPECIFIED.,.F.,.F.,(4,1,1,1,1,1,
1,4),(59.690260418206,60.2864241699918,61.2839955429748,62.2815669159577,
63.2791382889406,64.2767096619236,65.2742810349065,65.9734457253856),
 .UNSPECIFIED.);
#3507=B_SPLINE_CURVE_WITH_KNOTS('',3,(#30457,#30458,#30459,#30460,#30461,
#30462,#30463,#30464,#30465,#30466),.UNSPECIFIED.,.F.,.F.,(4,1,1,1,1,1,
1,4),(53.4070751110264,53.7595776695399,54.7571490425228,55.7547204155057,
56.7522917884886,57.7498631614716,58.7474345344545,59.690260418206),
 .UNSPECIFIED.);
#3508=B_SPLINE_CURVE_WITH_KNOTS('',3,(#30467,#30468,#30469,#30470,#30471,
#30472,#30473,#30474,#30475,#30476),.UNSPECIFIED.,.F.,.F.,(4,1,1,1,1,1,
1,4),(53.4070751110264,54.3009959320942,55.2985673050772,56.2961386780601,
57.293710051043,58.291281424026,59.2888527970089,59.690260418206),
 .UNSPECIFIED.);
#3509=B_SPLINE_CURVE_WITH_KNOTS('',3,(#30481,#30482,#30483,#30484,#30485,
#30486,#30487,#30488,#30489,#30490),.UNSPECIFIED.,.F.,.F.,(4,1,1,1,1,1,
1,4),(47.1238898038468,47.7741494316423,48.7717208046252,49.7692921776081,
50.7668635505911,51.764434923574,52.7620062965569,53.4070751110264),
 .UNSPECIFIED.);
#3510=B_SPLINE_CURVE_WITH_KNOTS('',3,(#30491,#30492,#30493,#30494,#30495,
#30496,#30497,#30498,#30499,#30500,#30501),.UNSPECIFIED.,.F.,.F.,(4,1,1,
1,1,1,1,1,4),(47.1238898038468,47.3179963212137,48.3155676941966,49.3131390671796,
50.3107104401625,51.3082818131454,52.3058531861284,53.3034245591113,53.4070751110264),
 .UNSPECIFIED.);
#3511=B_SPLINE_CURVE_WITH_KNOTS('',3,(#30506,#30507,#30508,#30509,#30510,
#30511,#30512,#30513,#30514,#30515),.UNSPECIFIED.,.F.,.F.,(4,1,1,1,1,1,
1,4),(40.8407044966672,41.7887211937447,42.7862925667276,43.7838639397105,
44.7814353126935,45.7790066856764,46.7765780586593,47.1238898038468),
 .UNSPECIFIED.);
#3512=B_SPLINE_CURVE_WITH_KNOTS('',3,(#30516,#30517,#30518,#30519,#30520,
#30521,#30522,#30523,#30524,#30525),.UNSPECIFIED.,.F.,.F.,(4,1,1,1,1,1,
1,4),(40.8407044966673,41.3325680833161,42.330139456299,43.327710829282,
44.3252822022649,45.3228535752478,46.3204249482308,47.1238898038468),
 .UNSPECIFIED.);
#3513=B_SPLINE_CURVE_WITH_KNOTS('',3,(#30530,#30531,#30532,#30533,#30534,
#30535,#30536,#30537,#30538,#30539,#30540),.UNSPECIFIED.,.F.,.F.,(4,1,1,
1,1,1,1,1,4),(34.5575191894876,34.8057215828641,35.8032929558471,36.80086432883,
37.7984357018129,38.7960070747959,39.7935784477788,40.7911498207617,40.8407044966672),
 .UNSPECIFIED.);
#3514=B_SPLINE_CURVE_WITH_KNOTS('',3,(#30541,#30542,#30543,#30544,#30545,
#30546,#30547,#30548,#30549,#30550),.UNSPECIFIED.,.F.,.F.,(4,1,1,1,1,1,
1,4),(34.5575191894876,35.3471398454185,36.3447112184014,37.3422825913844,
38.3398539643673,39.3374253373502,40.3349967103332,40.8407044966673),
 .UNSPECIFIED.);
#3515=B_SPLINE_CURVE_WITH_KNOTS('',3,(#30555,#30556,#30557,#30558,#30559,
#30560,#30561,#30562,#30563,#30564),.UNSPECIFIED.,.F.,.F.,(4,1,1,1,1,1,
1,4),(28.2743338823081,28.8202933449665,29.8178647179495,30.8154360909324,
31.8130074639153,32.8105788368983,33.8081502098812,34.5575191894876),
 .UNSPECIFIED.);
#3516=B_SPLINE_CURVE_WITH_KNOTS('',3,(#30565,#30566,#30567,#30568,#30569,
#30570,#30571,#30572,#30573,#30574,#30575),.UNSPECIFIED.,.F.,.F.,(4,1,1,
1,1,1,1,1,4),(28.2743338823081,28.364140234538,29.3617116075209,30.3592829805038,
31.3568543534868,32.3544257264697,33.3519970994526,34.3495684724356,34.5575191894876),
 .UNSPECIFIED.);
#3517=B_SPLINE_CURVE_WITH_KNOTS('',3,(#30580,#30581,#30582,#30583,#30584,
#30585,#30586,#30587,#30588,#30589),.UNSPECIFIED.,.F.,.F.,(4,1,1,1,1,1,
1,4),(21.9911485751285,22.8348651070689,23.8324364800519,24.8300078530348,
25.8275792260177,26.8251505990007,27.8227219719836,28.2743338823081),
 .UNSPECIFIED.);
#3518=B_SPLINE_CURVE_WITH_KNOTS('',3,(#30590,#30591,#30592,#30593,#30594,
#30595,#30596,#30597,#30598,#30599),.UNSPECIFIED.,.F.,.F.,(4,1,1,1,1,1,
1,4),(21.9911485751285,22.3787119966404,23.3762833696233,24.3738547426063,
25.3714261155892,26.3689974885721,27.3665688615551,28.2743338823081),
 .UNSPECIFIED.);
#3519=B_SPLINE_CURVE_WITH_KNOTS('',3,(#30605,#30606,#30607,#30608,#30609),
 .UNSPECIFIED.,.F.,.F.,(4,1,4),(14.3981410127769,15.3957123857599,15.7079632679489),
 .UNSPECIFIED.);
#3520=B_SPLINE_CURVE_WITH_KNOTS('',3,(#30612,#30613,#30614,#30615,#30616),
 .UNSPECIFIED.,.F.,.F.,(4,1,4),(13.8761928695311,14.8542941232055,15.7079632679489),
 .UNSPECIFIED.);
#3521=B_SPLINE_CURVE_WITH_KNOTS('',3,(#30622,#30623,#30624,#30625,#30626,
#30627,#30628,#30629,#30630,#30631,#30632,#30633,#30634,#30635,#30636,#30637,
#30638,#30639,#30640,#30641,#30642,#30643),.UNSPECIFIED.,.F.,.F.,(4,3,3,
3,3,3,3,4),(76.708045941327,76.8129957196858,77.8105670926687,78.8081384656517,
79.8057098386346,80.8032812116175,81.8008525846005,82.7984239575834),
 .UNSPECIFIED.);
#3522=B_SPLINE_CURVE_WITH_KNOTS('',3,(#30647,#30648,#30649,#30650,#30651,
#30652,#30653),.UNSPECIFIED.,.F.,.F.,(4,3,4),(-80.7838110923091,-79.8057098386346,
-79.2446069498473),.UNSPECIFIED.);
#3523=B_SPLINE_CURVE_WITH_KNOTS('',3,(#30657,#30658,#30659,#30660,#30661,
#30662,#30663,#30664,#30665,#30666,#30667,#30668,#30669,#30670,#30671,#30672,
#30673,#30674,#30675,#30676,#30677,#30678),.UNSPECIFIED.,.F.,.F.,(4,3,3,
3,3,3,3,4),(-79.2446069498473,-78.8081384656517,-77.8105670926688,-76.8129957196858,
-75.8154243467029,-74.81785297372,-73.820281600737,-72.9614216426677),
 .UNSPECIFIED.);
#3524=B_SPLINE_CURVE_WITH_KNOTS('',3,(#30683,#30684,#30685,#30686,#30687,
#30688,#30689,#30690,#30691,#30692,#30693,#30694,#30695,#30696,#30697,#30698,
#30699,#30700,#30701,#30702,#30703,#30704),.UNSPECIFIED.,.F.,.F.,(4,3,3,
3,3,3,3,4),(70.4248606341474,70.8275674817882,71.8251388547712,72.8227102277541,
73.820281600737,74.81785297372,75.8154243467029,76.708045941327),
 .UNSPECIFIED.);
#3525=B_SPLINE_CURVE_WITH_KNOTS('',3,(#30705,#30706,#30707,#30708,#30709,
#30710,#30711,#30712,#30713,#30714,#30715,#30716,#30717,#30718,#30719,#30720,
#30721,#30722,#30723,#30724,#30725,#30726,#30727,#30728,#30729),
 .UNSPECIFIED.,.F.,.F.,(4,3,3,3,3,3,3,3,4),(-72.9614216426677,-72.8227102277541,
-71.8251388547712,-70.8275674817882,-69.8299961088053,-68.8324247358224,
-67.8348533628394,-66.8372819898565,-66.6782363354882),.UNSPECIFIED.);
#3526=B_SPLINE_CURVE_WITH_KNOTS('',3,(#30734,#30735,#30736,#30737,#30738,
#30739,#30740,#30741,#30742,#30743,#30744,#30745,#30746,#30747,#30748,#30749,
#30750,#30751,#30752,#30753,#30754,#30755),.UNSPECIFIED.,.F.,.F.,(4,3,3,
3,3,3,3,4),(64.1416753269678,64.8421392438906,65.8397106168735,66.8372819898565,
67.8348533628394,68.8324247358223,69.8299961088053,70.4248606341474),
 .UNSPECIFIED.);
#3527=B_SPLINE_CURVE_WITH_KNOTS('',3,(#30756,#30757,#30758,#30759,#30760,
#30761,#30762,#30763,#30764,#30765,#30766,#30767,#30768,#30769,#30770,#30771,
#30772,#30773,#30774,#30775,#30776,#30777),.UNSPECIFIED.,.F.,.F.,(4,3,3,
3,3,3,3,4),(-66.6782363354882,-65.8397106168736,-64.8421392438906,-63.8445678709077,
-62.8469964979248,-61.8494251249418,-60.8518537519589,-60.3950510283086),
 .UNSPECIFIED.);
#3528=B_SPLINE_CURVE_WITH_KNOTS('',3,(#30782,#30783,#30784,#30785,#30786,
#30787,#30788,#30789,#30790,#30791,#30792,#30793,#30794,#30795,#30796,#30797,
#30798,#30799,#30800,#30801,#30802,#30803),.UNSPECIFIED.,.F.,.F.,(4,3,3,
3,3,3,3,4),(57.8584900197882,58.856711005993,59.854282378976,60.8518537519589,
61.8494251249418,62.8469964979248,63.8445678709077,64.1416753269678),
 .UNSPECIFIED.);
#3529=B_SPLINE_CURVE_WITH_KNOTS('',3,(#30804,#30805,#30806,#30807,#30808,
#30809,#30810,#30811,#30812,#30813,#30814,#30815,#30816,#30817,#30818,#30819,
#30820,#30821,#30822,#30823,#30824,#30825),.UNSPECIFIED.,.F.,.F.,(4,3,3,
3,3,3,3,4),(-60.3950510283086,-59.854282378976,-58.856711005993,-57.8591396330101,
-56.8615682600272,-55.8639968870442,-54.8664255140613,-54.111865721129),
 .UNSPECIFIED.);
#3530=B_SPLINE_CURVE_WITH_KNOTS('',3,(#30830,#30831,#30832,#30833,#30834,
#30835,#30836,#30837,#30838,#30839,#30840,#30841,#30842,#30843,#30844,#30845,
#30846,#30847,#30848,#30849,#30850,#30851),.UNSPECIFIED.,.F.,.F.,(4,3,3,
3,3,3,3,4),(51.5753047126087,51.8737113951125,52.8712827680954,53.8688541410784,
54.8664255140613,55.8639968870442,56.8615682600272,57.8584900197882),
 .UNSPECIFIED.);
#3531=B_SPLINE_CURVE_WITH_KNOTS('',3,(#30852,#30853,#30854,#30855,#30856,
#30857,#30858,#30859,#30860,#30861,#30862,#30863,#30864,#30865,#30866,#30867,
#30868,#30869,#30870,#30871,#30872,#30873,#30874,#30875,#30876),
 .UNSPECIFIED.,.F.,.F.,(4,3,3,3,3,3,3,3,4),(-54.111865721129,-53.8688541410784,
-52.8712827680954,-51.8737113951125,-50.8761400221296,-49.8785686491466,
-48.8809972761637,-47.8834259031808,-47.8286804139494),.UNSPECIFIED.);
#3532=B_SPLINE_CURVE_WITH_KNOTS('',3,(#30881,#30882,#30883,#30884,#30885,
#30886,#30887,#30888,#30889,#30890,#30891,#30892,#30893,#30894,#30895,#30896,
#30897,#30898,#30899,#30900,#30901,#30902),.UNSPECIFIED.,.F.,.F.,(4,3,3,
3,3,3,3,4),(45.2921194054291,45.8882831572149,46.8858545301978,47.8834259031808,
48.8809972761637,49.8785686491466,50.8761400221296,51.5753047126087),
 .UNSPECIFIED.);
#3533=B_SPLINE_CURVE_WITH_KNOTS('',3,(#30903,#30904,#30905,#30906,#30907,
#30908,#30909,#30910,#30911,#30912,#30913,#30914,#30915,#30916,#30917,#30918,
#30919,#30920,#30921,#30922,#30923,#30924),.UNSPECIFIED.,.F.,.F.,(4,3,3,
3,3,3,3,4),(-47.8286804139494,-46.8858545301978,-45.8882831572149,-44.890711784232,
-43.893140411249,-42.8955690382661,-41.8979976652832,-41.5454951067698),
 .UNSPECIFIED.);
#3534=B_SPLINE_CURVE_WITH_KNOTS('',3,(#30929,#30930,#30931,#30932,#30933,
#30934,#30935,#30936,#30937,#30938,#30939,#30940,#30941,#30942,#30943,#30944,
#30945,#30946,#30947,#30948,#30949,#30950),.UNSPECIFIED.,.F.,.F.,(4,3,3,
3,3,3,3,4),(39.0089340982495,39.9028549193173,40.9004262923002,41.8979976652832,
42.8955690382661,43.893140411249,44.890711784232,45.2921194054291),
 .UNSPECIFIED.);
#3535=B_SPLINE_CURVE_WITH_KNOTS('',3,(#30951,#30952,#30953,#30954,#30955,
#30956,#30957,#30958,#30959,#30960,#30961,#30962,#30963,#30964,#30965,#30966,
#30967,#30968,#30969,#30970,#30971,#30972),.UNSPECIFIED.,.F.,.F.,(4,3,3,
3,3,3,3,4),(-41.5454951067698,-40.9004262923002,-39.9028549193173,-38.9052835463344,
-37.9077121733514,-36.9101408003685,-35.9125694273856,-35.2623097995902),
 .UNSPECIFIED.);
#3536=B_SPLINE_CURVE_WITH_KNOTS('',3,(#30977,#30978,#30979,#30980,#30981,
#30982,#30983,#30984,#30985,#30986,#30987,#30988,#30989,#30990,#30991,#30992,
#30993,#30994,#30995,#30996,#30997,#30998,#30999,#31000,#31001),
 .UNSPECIFIED.,.F.,.F.,(4,3,3,3,3,3,3,3,4),(32.7257487910699,32.9198553084368,
33.9174266814197,34.9149980544026,35.9125694273856,36.9101408003685,37.9077121733514,
38.9052835463344,39.0089340982495),.UNSPECIFIED.);
#3537=B_SPLINE_CURVE_WITH_KNOTS('',3,(#31002,#31003,#31004,#31005,#31006,
#31007,#31008,#31009,#31010,#31011,#31012,#31013,#31014,#31015,#31016,#31017,
#31018,#31019,#31020,#31021,#31022,#31023),.UNSPECIFIED.,.F.,.F.,(4,3,3,
3,3,3,3,4),(-35.2623097995902,-34.9149980544027,-33.9174266814197,-32.9198553084368,
-31.9222839354538,-30.9247125624709,-29.927141189488,-28.9791244924106),
 .UNSPECIFIED.);
#3538=B_SPLINE_CURVE_WITH_KNOTS('',3,(#31028,#31029,#31030,#31031,#31032,
#31033,#31034,#31035,#31036,#31037,#31038,#31039,#31040,#31041,#31042,#31043,
#31044,#31045,#31046,#31047,#31048,#31049),.UNSPECIFIED.,.F.,.F.,(4,3,3,
3,3,3,3,4),(26.4425634838903,26.9344270705392,27.9319984435221,28.929569816505,
29.927141189488,30.9247125624709,31.9222839354538,32.7257487910699),
 .UNSPECIFIED.);
#3539=B_SPLINE_CURVE_WITH_KNOTS('',3,(#31050,#31051,#31052,#31053,#31054,
#31055,#31056,#31057,#31058,#31059,#31060,#31061,#31062,#31063,#31064,#31065,
#31066,#31067,#31068,#31069,#31070,#31071,#31072,#31073,#31074),
 .UNSPECIFIED.,.F.,.F.,(4,3,3,3,3,3,3,3,4),(-28.9791244924106,-28.9295698165051,
-27.9319984435221,-26.9344270705392,-25.9368556975562,-24.9392843245733,
-23.9417129515904,-22.9441415786074,-22.695939185231),.UNSPECIFIED.);
#3540=B_SPLINE_CURVE_WITH_KNOTS('',3,(#31079,#31080,#31081,#31082,#31083,
#31084,#31085,#31086,#31087,#31088,#31089,#31090,#31091,#31092,#31093,#31094,
#31095,#31096,#31097,#31098,#31099,#31100),.UNSPECIFIED.,.F.,.F.,(4,3,3,
3,3,3,3,4),(20.1593781767107,20.9489988326416,21.9465702056245,22.9441415786075,
23.9417129515904,24.9392843245733,25.9368556975563,26.4425634838903),
 .UNSPECIFIED.);
#3541=B_SPLINE_CURVE_WITH_KNOTS('',3,(#31101,#31102,#31103,#31104,#31105,
#31106,#31107,#31108,#31109,#31110,#31111,#31112,#31113,#31114,#31115,#31116,
#31117,#31118,#31119,#31120,#31121,#31122),.UNSPECIFIED.,.F.,.F.,(4,3,3,
3,3,3,3,4),(-22.695939185231,-21.9465702056245,-20.9489988326416,-19.9514274596586,
-18.9538560866757,-17.9562847136928,-16.9587133407099,-16.4127538780514),
 .UNSPECIFIED.);
#3542=B_SPLINE_CURVE_WITH_KNOTS('',3,(#31127,#31128,#31129,#31130,#31131,
#31132,#31133,#31134,#31135,#31136,#31137,#31138,#31139,#31140,#31141,#31142,
#31143,#31144,#31145,#31146,#31147,#31148,#31149,#31150,#31151),
 .UNSPECIFIED.,.F.,.F.,(4,3,3,3,3,3,3,3,4),(13.8761928695311,13.9659992217611,
14.963570594744,15.9611419677269,16.9587133407099,17.9562847136928,18.9538560866757,
19.9514274596586,20.1593781767107),.UNSPECIFIED.);
#3543=B_SPLINE_CURVE_WITH_KNOTS('',3,(#31152,#31153,#31154,#31155,#31156,
#31157,#31158,#31159,#31160,#31161,#31162,#31163,#31164,#31165,#31166,#31167,
#31168,#31169,#31170,#31171,#31172,#31173),.UNSPECIFIED.,.F.,.F.,(4,3,3,
3,3,3,3,4),(-16.4127538780514,-15.9611419677269,-14.963570594744,-13.9659992217611,
-12.9684278487781,-11.9708564757952,-10.9732851028123,-10.1295685708718),
 .UNSPECIFIED.);
#3544=B_SPLINE_CURVE_WITH_KNOTS('',3,(#31179,#31180,#31181,#31182,#31183,
#31184,#31185,#31186,#31187,#31188,#31189,#31190,#31191),.UNSPECIFIED.,
 .F.,.F.,(4,3,3,3,4),(-3.84638326369224,-2.9927141189488,-1.99514274596586,
-0.997571372982933,0.),.UNSPECIFIED.);
#3545=B_SPLINE_CURVE_WITH_KNOTS('',3,(#31194,#31195,#31196,#31197,#31198,
#31199,#31200,#31201,#31202,#31203,#31204,#31205,#31206,#31207,#31208,#31209,
#31210,#31211,#31212),.UNSPECIFIED.,.F.,.F.,(4,3,3,3,3,3,4),(2.01461286527433,
2.9927141189488,3.99028549193173,4.98785686491466,5.9854282378976,6.98299961088053,
7.59300756235153),.UNSPECIFIED.);
#3546=B_SPLINE_CURVE_WITH_KNOTS('',3,(#31218,#31219,#31220,#31221,#31222,
#31223,#31224),.UNSPECIFIED.,.F.,.F.,(4,1,1,1,4),(91.106186954104,91.6672898428913,
92.6648612158742,93.6624325888572,94.6600039618401),.UNSPECIFIED.);
#3547=B_SPLINE_CURVE_WITH_KNOTS('',3,(#31227,#31228,#31229,#31230,#31231,
#31232,#31233,#31234),.UNSPECIFIED.,.F.,.F.,(4,1,1,1,1,4),(91.106186954104,
91.2111367324627,92.2087081054457,93.2062794784286,94.2038508514115,95.1819521050859),
 .UNSPECIFIED.);
#3548=B_SPLINE_CURVE_WITH_KNOTS('',3,(#31239,#31240,#31241,#31242,#31243,
#31244,#31245,#31246,#31247,#31248),.UNSPECIFIED.,.F.,.F.,(4,1,1,1,1,1,
1,4),(84.8230016469244,85.6818616049937,86.6794329779766,87.6770043509596,
88.6745757239425,89.6721470969254,90.6697184699084,91.106186954104),
 .UNSPECIFIED.);
#3549=B_SPLINE_CURVE_WITH_KNOTS('',3,(#31249,#31250,#31251,#31252,#31253,
#31254,#31255,#31256,#31257,#31258),.UNSPECIFIED.,.F.,.F.,(4,1,1,1,1,1,
1,4),(84.8230016469244,85.2257084945651,86.2232798675481,87.220851240531,
88.2184226135139,89.2159939864969,90.2135653594798,91.106186954104),
 .UNSPECIFIED.);
#3550=B_SPLINE_CURVE_WITH_KNOTS('',3,(#31263,#31264,#31265,#31266,#31267,
#31268,#31269,#31270,#31271,#31272,#31273),.UNSPECIFIED.,.F.,.F.,(4,1,1,
1,1,1,1,1,4),(78.5398163397448,78.6988619941132,79.6964333670961,80.694004740079,
81.691576113062,82.6891474860449,83.6867188590278,84.6842902320108,84.8230016469244),
 .UNSPECIFIED.);
#3551=B_SPLINE_CURVE_WITH_KNOTS('',3,(#31274,#31275,#31276,#31277,#31278,
#31279,#31280,#31281,#31282,#31283),.UNSPECIFIED.,.F.,.F.,(4,1,1,1,1,1,
1,4),(78.5398163397448,79.2402802566675,80.2378516296505,81.2354230026334,
82.2329943756163,83.2305657485993,84.2281371215822,84.8230016469244),
 .UNSPECIFIED.);
#3552=B_SPLINE_CURVE_WITH_KNOTS('',3,(#31288,#31289,#31290,#31291,#31292,
#31293,#31294,#31295,#31296,#31297),.UNSPECIFIED.,.F.,.F.,(4,1,1,1,1,1,
1,4),(72.2566310325652,72.7134337562156,73.7110051291985,74.7085765021814,
75.7061478751644,76.7037192481473,77.7012906211302,78.5398163397448),
 .UNSPECIFIED.);
#3553=B_SPLINE_CURVE_WITH_KNOTS('',3,(#31298,#31299,#31300,#31301,#31302,
#31303,#31304,#31305,#31306,#31307,#31308),.UNSPECIFIED.,.F.,.F.,(4,1,1,
1,1,1,1,1,4),(72.2566310325652,72.257280645787,73.25485201877,74.2524233917529,
75.2499947647358,76.2475661377187,77.2451375107017,78.2427088836846,78.5398163397448),
 .UNSPECIFIED.);
#3554=B_SPLINE_CURVE_WITH_KNOTS('',3,(#31313,#31314,#31315,#31316,#31317,
#31318,#31319,#31320,#31321,#31322),.UNSPECIFIED.,.F.,.F.,(4,1,1,1,1,1,
1,4),(65.9734457253856,66.728005518318,67.7255768913009,68.7231482642838,
69.7207196372668,70.7182910102497,71.7158623832326,72.2566310325652),
 .UNSPECIFIED.);
#3555=B_SPLINE_CURVE_WITH_KNOTS('',3,(#31323,#31324,#31325,#31326,#31327,
#31328,#31329,#31330,#31331,#31332),.UNSPECIFIED.,.F.,.F.,(4,1,1,1,1,1,
1,4),(65.9734457253856,66.2718524078894,67.2694237808724,68.2669951538553,
69.2645665268382,70.2621378998212,71.2597092728041,72.2566310325652),
 .UNSPECIFIED.);
#3556=B_SPLINE_CURVE_WITH_KNOTS('',3,(#31337,#31338,#31339,#31340,#31341,
#31342,#31343,#31344,#31345,#31346,#31347),.UNSPECIFIED.,.F.,.F.,(4,1,1,
1,1,1,1,1,4),(59.690260418206,59.7450059074374,60.7425772804204,61.7401486534033,
62.7377200263862,63.7352913993692,64.7328627723521,65.730434145335,65.9734457253856),
 .UNSPECIFIED.);
#3557=B_SPLINE_CURVE_WITH_KNOTS('',3,(#31348,#31349,#31350,#31351,#31352,
#31353,#31354,#31355,#31356,#31357),.UNSPECIFIED.,.F.,.F.,(4,1,1,1,1,1,
1,4),(59.690260418206,60.2864241699918,61.2839955429748,62.2815669159577,
63.2791382889406,64.2767096619236,65.2742810349065,65.9734457253856),
 .UNSPECIFIED.);
#3558=B_SPLINE_CURVE_WITH_KNOTS('',3,(#31362,#31363,#31364,#31365,#31366,
#31367,#31368,#31369,#31370,#31371),.UNSPECIFIED.,.F.,.F.,(4,1,1,1,1,1,
1,4),(53.4070751110264,53.7595776695399,54.7571490425228,55.7547204155057,
56.7522917884886,57.7498631614716,58.7474345344545,59.690260418206),
 .UNSPECIFIED.);
#3559=B_SPLINE_CURVE_WITH_KNOTS('',3,(#31372,#31373,#31374,#31375,#31376,
#31377,#31378,#31379,#31380,#31381),.UNSPECIFIED.,.F.,.F.,(4,1,1,1,1,1,
1,4),(53.4070751110265,54.3009959320942,55.2985673050772,56.2961386780601,
57.293710051043,58.291281424026,59.2888527970089,59.690260418206),
 .UNSPECIFIED.);
#3560=B_SPLINE_CURVE_WITH_KNOTS('',3,(#31386,#31387,#31388,#31389,#31390,
#31391,#31392,#31393,#31394,#31395),.UNSPECIFIED.,.F.,.F.,(4,1,1,1,1,1,
1,4),(47.1238898038468,47.7741494316423,48.7717208046252,49.7692921776081,
50.7668635505911,51.764434923574,52.7620062965569,53.4070751110264),
 .UNSPECIFIED.);
#3561=B_SPLINE_CURVE_WITH_KNOTS('',3,(#31396,#31397,#31398,#31399,#31400,
#31401,#31402,#31403,#31404,#31405,#31406),.UNSPECIFIED.,.F.,.F.,(4,1,1,
1,1,1,1,1,4),(47.1238898038469,47.3179963212137,48.3155676941966,49.3131390671796,
50.3107104401625,51.3082818131454,52.3058531861284,53.3034245591113,53.4070751110265),
 .UNSPECIFIED.);
#3562=B_SPLINE_CURVE_WITH_KNOTS('',3,(#31411,#31412,#31413,#31414,#31415,
#31416,#31417,#31418,#31419,#31420),.UNSPECIFIED.,.F.,.F.,(4,1,1,1,1,1,
1,4),(40.8407044966673,41.7887211937447,42.7862925667276,43.7838639397105,
44.7814353126935,45.7790066856764,46.7765780586593,47.1238898038468),
 .UNSPECIFIED.);
#3563=B_SPLINE_CURVE_WITH_KNOTS('',3,(#31421,#31422,#31423,#31424,#31425,
#31426,#31427,#31428,#31429,#31430),.UNSPECIFIED.,.F.,.F.,(4,1,1,1,1,1,
1,4),(40.8407044966673,41.3325680833161,42.330139456299,43.327710829282,
44.3252822022649,45.3228535752478,46.3204249482308,47.1238898038469),
 .UNSPECIFIED.);
#3564=B_SPLINE_CURVE_WITH_KNOTS('',3,(#31435,#31436,#31437,#31438,#31439,
#31440,#31441,#31442,#31443,#31444,#31445),.UNSPECIFIED.,.F.,.F.,(4,1,1,
1,1,1,1,1,4),(34.5575191894876,34.8057215828641,35.8032929558471,36.80086432883,
37.7984357018129,38.7960070747959,39.7935784477788,40.7911498207617,40.8407044966673),
 .UNSPECIFIED.);
#3565=B_SPLINE_CURVE_WITH_KNOTS('',3,(#31446,#31447,#31448,#31449,#31450,
#31451,#31452,#31453,#31454,#31455),.UNSPECIFIED.,.F.,.F.,(4,1,1,1,1,1,
1,4),(34.5575191894877,35.3471398454185,36.3447112184014,37.3422825913844,
38.3398539643673,39.3374253373502,40.3349967103332,40.8407044966673),
 .UNSPECIFIED.);
#3566=B_SPLINE_CURVE_WITH_KNOTS('',3,(#31460,#31461,#31462,#31463,#31464,
#31465,#31466,#31467,#31468,#31469),.UNSPECIFIED.,.F.,.F.,(4,1,1,1,1,1,
1,4),(28.2743338823081,28.8202933449665,29.8178647179495,30.8154360909324,
31.8130074639153,32.8105788368983,33.8081502098812,34.5575191894876),
 .UNSPECIFIED.);
#3567=B_SPLINE_CURVE_WITH_KNOTS('',3,(#31470,#31471,#31472,#31473,#31474,
#31475,#31476,#31477,#31478,#31479,#31480),.UNSPECIFIED.,.F.,.F.,(4,1,1,
1,1,1,1,1,4),(28.2743338823081,28.364140234538,29.3617116075209,30.3592829805038,
31.3568543534868,32.3544257264697,33.3519970994526,34.3495684724356,34.5575191894877),
 .UNSPECIFIED.);
#3568=B_SPLINE_CURVE_WITH_KNOTS('',3,(#31485,#31486,#31487,#31488,#31489,
#31490,#31491,#31492,#31493,#31494),.UNSPECIFIED.,.F.,.F.,(4,1,1,1,1,1,
1,4),(21.9911485751285,22.8348651070689,23.8324364800519,24.8300078530348,
25.8275792260177,26.8251505990007,27.8227219719836,28.2743338823081),
 .UNSPECIFIED.);
#3569=B_SPLINE_CURVE_WITH_KNOTS('',3,(#31495,#31496,#31497,#31498,#31499,
#31500,#31501,#31502,#31503,#31504),.UNSPECIFIED.,.F.,.F.,(4,1,1,1,1,1,
1,4),(21.9911485751285,22.3787119966404,23.3762833696233,24.3738547426063,
25.3714261155892,26.3689974885721,27.3665688615551,28.2743338823081),
 .UNSPECIFIED.);
#3570=B_SPLINE_CURVE_WITH_KNOTS('',3,(#31510,#31511,#31512,#31513,#31514),
 .UNSPECIFIED.,.F.,.F.,(4,1,4),(14.3981410127769,15.3957123857599,15.7079632679489),
 .UNSPECIFIED.);
#3571=B_SPLINE_CURVE_WITH_KNOTS('',3,(#31517,#31518,#31519,#31520,#31521),
 .UNSPECIFIED.,.F.,.F.,(4,1,4),(13.8761928695311,14.8542941232055,15.7079632679489),
 .UNSPECIFIED.);
#3572=B_SPLINE_CURVE_WITH_KNOTS('',3,(#31527,#31528,#31529,#31530,#31531,
#31532,#31533,#31534,#31535,#31536,#31537,#31538,#31539,#31540,#31541,#31542,
#31543,#31544,#31545,#31546,#31547,#31548),.UNSPECIFIED.,.F.,.F.,(4,3,3,
3,3,3,3,4),(76.708045941327,76.8129957196858,77.8105670926687,78.8081384656517,
79.8057098386346,80.8032812116175,81.8008525846005,82.7984239575834),
 .UNSPECIFIED.);
#3573=B_SPLINE_CURVE_WITH_KNOTS('',3,(#31552,#31553,#31554,#31555,#31556,
#31557,#31558),.UNSPECIFIED.,.F.,.F.,(4,3,4),(-80.783811092309,-79.8057098386346,
-79.2446069498473),.UNSPECIFIED.);
#3574=B_SPLINE_CURVE_WITH_KNOTS('',3,(#31562,#31563,#31564,#31565,#31566,
#31567,#31568,#31569,#31570,#31571,#31572,#31573,#31574,#31575,#31576,#31577,
#31578,#31579,#31580,#31581,#31582,#31583),.UNSPECIFIED.,.F.,.F.,(4,3,3,
3,3,3,3,4),(-79.2446069498473,-78.8081384656517,-77.8105670926687,-76.8129957196858,
-75.8154243467029,-74.81785297372,-73.820281600737,-72.9614216426677),
 .UNSPECIFIED.);
#3575=B_SPLINE_CURVE_WITH_KNOTS('',3,(#31588,#31589,#31590,#31591,#31592,
#31593,#31594,#31595,#31596,#31597,#31598,#31599,#31600,#31601,#31602,#31603,
#31604,#31605,#31606,#31607,#31608,#31609),.UNSPECIFIED.,.F.,.F.,(4,3,3,
3,3,3,3,4),(70.4248606341474,70.8275674817882,71.8251388547712,72.8227102277541,
73.820281600737,74.81785297372,75.8154243467029,76.708045941327),
 .UNSPECIFIED.);
#3576=B_SPLINE_CURVE_WITH_KNOTS('',3,(#31610,#31611,#31612,#31613,#31614,
#31615,#31616,#31617,#31618,#31619,#31620,#31621,#31622,#31623,#31624,#31625,
#31626,#31627,#31628,#31629,#31630,#31631,#31632,#31633,#31634),
 .UNSPECIFIED.,.F.,.F.,(4,3,3,3,3,3,3,3,4),(-72.9614216426677,-72.8227102277541,
-71.8251388547712,-70.8275674817882,-69.8299961088053,-68.8324247358224,
-67.8348533628394,-66.8372819898565,-66.6782363354881),.UNSPECIFIED.);
#3577=B_SPLINE_CURVE_WITH_KNOTS('',3,(#31639,#31640,#31641,#31642,#31643,
#31644,#31645,#31646,#31647,#31648,#31649,#31650,#31651,#31652,#31653,#31654,
#31655,#31656,#31657,#31658,#31659,#31660),.UNSPECIFIED.,.F.,.F.,(4,3,3,
3,3,3,3,4),(64.1416753269678,64.8421392438906,65.8397106168735,66.8372819898565,
67.8348533628394,68.8324247358223,69.8299961088053,70.4248606341474),
 .UNSPECIFIED.);
#3578=B_SPLINE_CURVE_WITH_KNOTS('',3,(#31661,#31662,#31663,#31664,#31665,
#31666,#31667,#31668,#31669,#31670,#31671,#31672,#31673,#31674,#31675,#31676,
#31677,#31678,#31679,#31680,#31681,#31682),.UNSPECIFIED.,.F.,.F.,(4,3,3,
3,3,3,3,4),(-66.6782363354881,-65.8397106168736,-64.8421392438906,-63.8445678709077,
-62.8469964979248,-61.8494251249418,-60.8518537519589,-60.3950510283085),
 .UNSPECIFIED.);
#3579=B_SPLINE_CURVE_WITH_KNOTS('',3,(#31687,#31688,#31689,#31690,#31691,
#31692,#31693,#31694,#31695,#31696,#31697,#31698,#31699,#31700,#31701,#31702,
#31703,#31704,#31705,#31706,#31707,#31708),.UNSPECIFIED.,.F.,.F.,(4,3,3,
3,3,3,3,4),(57.8584900197882,58.856711005993,59.854282378976,60.8518537519589,
61.8494251249418,62.8469964979248,63.8445678709077,64.1416753269678),
 .UNSPECIFIED.);
#3580=B_SPLINE_CURVE_WITH_KNOTS('',3,(#31709,#31710,#31711,#31712,#31713,
#31714,#31715,#31716,#31717,#31718,#31719,#31720,#31721,#31722,#31723,#31724,
#31725,#31726,#31727,#31728,#31729,#31730),.UNSPECIFIED.,.F.,.F.,(4,3,3,
3,3,3,3,4),(-60.3950510283085,-59.854282378976,-58.856711005993,-57.8591396330101,
-56.8615682600271,-55.8639968870442,-54.8664255140613,-54.111865721129),
 .UNSPECIFIED.);
#3581=B_SPLINE_CURVE_WITH_KNOTS('',3,(#31735,#31736,#31737,#31738,#31739,
#31740,#31741,#31742,#31743,#31744,#31745,#31746,#31747,#31748,#31749,#31750,
#31751,#31752,#31753,#31754,#31755,#31756),.UNSPECIFIED.,.F.,.F.,(4,3,3,
3,3,3,3,4),(51.5753047126087,51.8737113951125,52.8712827680954,53.8688541410784,
54.8664255140613,55.8639968870442,56.8615682600272,57.8584900197882),
 .UNSPECIFIED.);
#3582=B_SPLINE_CURVE_WITH_KNOTS('',3,(#31757,#31758,#31759,#31760,#31761,
#31762,#31763,#31764,#31765,#31766,#31767,#31768,#31769,#31770,#31771,#31772,
#31773,#31774,#31775,#31776,#31777,#31778,#31779,#31780,#31781),
 .UNSPECIFIED.,.F.,.F.,(4,3,3,3,3,3,3,3,4),(-54.111865721129,-53.8688541410784,
-52.8712827680954,-51.8737113951125,-50.8761400221296,-49.8785686491466,
-48.8809972761637,-47.8834259031808,-47.8286804139494),.UNSPECIFIED.);
#3583=B_SPLINE_CURVE_WITH_KNOTS('',3,(#31786,#31787,#31788,#31789,#31790,
#31791,#31792,#31793,#31794,#31795,#31796,#31797,#31798,#31799,#31800,#31801,
#31802,#31803,#31804,#31805,#31806,#31807),.UNSPECIFIED.,.F.,.F.,(4,3,3,
3,3,3,3,4),(45.2921194054291,45.8882831572149,46.8858545301978,47.8834259031808,
48.8809972761637,49.8785686491466,50.8761400221296,51.5753047126087),
 .UNSPECIFIED.);
#3584=B_SPLINE_CURVE_WITH_KNOTS('',3,(#31808,#31809,#31810,#31811,#31812,
#31813,#31814,#31815,#31816,#31817,#31818,#31819,#31820,#31821,#31822,#31823,
#31824,#31825,#31826,#31827,#31828,#31829),.UNSPECIFIED.,.F.,.F.,(4,3,3,
3,3,3,3,4),(-47.8286804139494,-46.8858545301978,-45.8882831572149,-44.890711784232,
-43.893140411249,-42.8955690382661,-41.8979976652832,-41.5454951067698),
 .UNSPECIFIED.);
#3585=B_SPLINE_CURVE_WITH_KNOTS('',3,(#31834,#31835,#31836,#31837,#31838,
#31839,#31840,#31841,#31842,#31843,#31844,#31845,#31846,#31847,#31848,#31849,
#31850,#31851,#31852,#31853,#31854,#31855),.UNSPECIFIED.,.F.,.F.,(4,3,3,
3,3,3,3,4),(39.0089340982495,39.9028549193173,40.9004262923002,41.8979976652832,
42.8955690382661,43.893140411249,44.890711784232,45.2921194054291),
 .UNSPECIFIED.);
#3586=B_SPLINE_CURVE_WITH_KNOTS('',3,(#31856,#31857,#31858,#31859,#31860,
#31861,#31862,#31863,#31864,#31865,#31866,#31867,#31868,#31869,#31870,#31871,
#31872,#31873,#31874,#31875,#31876,#31877),.UNSPECIFIED.,.F.,.F.,(4,3,3,
3,3,3,3,4),(-41.5454951067698,-40.9004262923002,-39.9028549193173,-38.9052835463344,
-37.9077121733514,-36.9101408003685,-35.9125694273856,-35.2623097995902),
 .UNSPECIFIED.);
#3587=B_SPLINE_CURVE_WITH_KNOTS('',3,(#31882,#31883,#31884,#31885,#31886,
#31887,#31888,#31889,#31890,#31891,#31892,#31893,#31894,#31895,#31896,#31897,
#31898,#31899,#31900,#31901,#31902,#31903,#31904,#31905,#31906),
 .UNSPECIFIED.,.F.,.F.,(4,3,3,3,3,3,3,3,4),(32.7257487910699,32.9198553084368,
33.9174266814197,34.9149980544026,35.9125694273856,36.9101408003685,37.9077121733514,
38.9052835463344,39.0089340982495),.UNSPECIFIED.);
#3588=B_SPLINE_CURVE_WITH_KNOTS('',3,(#31907,#31908,#31909,#31910,#31911,
#31912,#31913,#31914,#31915,#31916,#31917,#31918,#31919,#31920,#31921,#31922,
#31923,#31924,#31925,#31926,#31927,#31928),.UNSPECIFIED.,.F.,.F.,(4,3,3,
3,3,3,3,4),(-35.2623097995902,-34.9149980544027,-33.9174266814197,-32.9198553084368,
-31.9222839354538,-30.9247125624709,-29.927141189488,-28.9791244924106),
 .UNSPECIFIED.);
#3589=B_SPLINE_CURVE_WITH_KNOTS('',3,(#31933,#31934,#31935,#31936,#31937,
#31938,#31939,#31940,#31941,#31942,#31943,#31944,#31945,#31946,#31947,#31948,
#31949,#31950,#31951,#31952,#31953,#31954),.UNSPECIFIED.,.F.,.F.,(4,3,3,
3,3,3,3,4),(26.4425634838903,26.9344270705392,27.9319984435221,28.929569816505,
29.927141189488,30.9247125624709,31.9222839354538,32.7257487910699),
 .UNSPECIFIED.);
#3590=B_SPLINE_CURVE_WITH_KNOTS('',3,(#31955,#31956,#31957,#31958,#31959,
#31960,#31961,#31962,#31963,#31964,#31965,#31966,#31967,#31968,#31969,#31970,
#31971,#31972,#31973,#31974,#31975,#31976,#31977,#31978,#31979),
 .UNSPECIFIED.,.F.,.F.,(4,3,3,3,3,3,3,3,4),(-28.9791244924106,-28.929569816505,
-27.9319984435221,-26.9344270705392,-25.9368556975562,-24.9392843245733,
-23.9417129515904,-22.9441415786075,-22.695939185231),.UNSPECIFIED.);
#3591=B_SPLINE_CURVE_WITH_KNOTS('',3,(#31984,#31985,#31986,#31987,#31988,
#31989,#31990,#31991,#31992,#31993,#31994,#31995,#31996,#31997,#31998,#31999,
#32000,#32001,#32002,#32003,#32004,#32005),.UNSPECIFIED.,.F.,.F.,(4,3,3,
3,3,3,3,4),(20.1593781767107,20.9489988326416,21.9465702056245,22.9441415786074,
23.9417129515904,24.9392843245733,25.9368556975562,26.4425634838903),
 .UNSPECIFIED.);
#3592=B_SPLINE_CURVE_WITH_KNOTS('',3,(#32006,#32007,#32008,#32009,#32010,
#32011,#32012,#32013,#32014,#32015,#32016,#32017,#32018,#32019,#32020,#32021,
#32022,#32023,#32024,#32025,#32026,#32027),.UNSPECIFIED.,.F.,.F.,(4,3,3,
3,3,3,3,4),(-22.695939185231,-21.9465702056245,-20.9489988326416,-19.9514274596587,
-18.9538560866757,-17.9562847136928,-16.9587133407099,-16.4127538780514),
 .UNSPECIFIED.);
#3593=B_SPLINE_CURVE_WITH_KNOTS('',3,(#32032,#32033,#32034,#32035,#32036,
#32037,#32038,#32039,#32040,#32041,#32042,#32043,#32044,#32045,#32046,#32047,
#32048,#32049,#32050,#32051,#32052,#32053,#32054,#32055,#32056),
 .UNSPECIFIED.,.F.,.F.,(4,3,3,3,3,3,3,3,4),(13.8761928695311,13.9659992217611,
14.963570594744,15.9611419677269,16.9587133407099,17.9562847136928,18.9538560866757,
19.9514274596586,20.1593781767107),.UNSPECIFIED.);
#3594=B_SPLINE_CURVE_WITH_KNOTS('',3,(#32057,#32058,#32059,#32060,#32061,
#32062,#32063,#32064,#32065,#32066,#32067,#32068,#32069,#32070,#32071,#32072,
#32073,#32074,#32075,#32076,#32077,#32078),.UNSPECIFIED.,.F.,.F.,(4,3,3,
3,3,3,3,4),(-16.4127538780514,-15.9611419677269,-14.963570594744,-13.9659992217611,
-12.9684278487781,-11.9708564757952,-10.9732851028123,-10.1295685708718),
 .UNSPECIFIED.);
#3595=B_SPLINE_CURVE_WITH_KNOTS('',3,(#32084,#32085,#32086,#32087,#32088,
#32089,#32090,#32091,#32092,#32093,#32094,#32095,#32096),.UNSPECIFIED.,
 .F.,.F.,(4,3,3,3,4),(-3.84638326369223,-2.9927141189488,-1.99514274596586,
-0.997571372982929,0.),.UNSPECIFIED.);
#3596=B_SPLINE_CURVE_WITH_KNOTS('',3,(#32099,#32100,#32101,#32102,#32103,
#32104,#32105,#32106,#32107,#32108,#32109,#32110,#32111,#32112,#32113,#32114,
#32115,#32116,#32117),.UNSPECIFIED.,.F.,.F.,(4,3,3,3,3,3,4),(2.01461286527443,
2.9927141189488,3.99028549193173,4.98785686491467,5.9854282378976,6.98299961088053,
7.59300756235153),.UNSPECIFIED.);
#3597=B_SPLINE_CURVE_WITH_KNOTS('',3,(#32123,#32124,#32125,#32126,#32127,
#32128,#32129),.UNSPECIFIED.,.F.,.F.,(4,1,1,1,4),(91.106186954104,91.6672898428913,
92.6648612158742,93.6624325888572,94.6600039618401),.UNSPECIFIED.);
#3598=B_SPLINE_CURVE_WITH_KNOTS('',3,(#32132,#32133,#32134,#32135,#32136,
#32137,#32138,#32139),.UNSPECIFIED.,.F.,.F.,(4,1,1,1,1,4),(91.106186954104,
91.2111367324627,92.2087081054457,93.2062794784286,94.2038508514115,95.1819521050859),
 .UNSPECIFIED.);
#3599=B_SPLINE_CURVE_WITH_KNOTS('',3,(#32144,#32145,#32146,#32147,#32148,
#32149,#32150,#32151,#32152,#32153),.UNSPECIFIED.,.F.,.F.,(4,1,1,1,1,1,
1,4),(84.8230016469244,85.6818616049937,86.6794329779766,87.6770043509596,
88.6745757239425,89.6721470969254,90.6697184699084,91.106186954104),
 .UNSPECIFIED.);
#3600=B_SPLINE_CURVE_WITH_KNOTS('',3,(#32154,#32155,#32156,#32157,#32158,
#32159,#32160,#32161,#32162,#32163),.UNSPECIFIED.,.F.,.F.,(4,1,1,1,1,1,
1,4),(84.8230016469244,85.2257084945651,86.2232798675481,87.220851240531,
88.2184226135139,89.2159939864969,90.2135653594798,91.106186954104),
 .UNSPECIFIED.);
#3601=B_SPLINE_CURVE_WITH_KNOTS('',3,(#32168,#32169,#32170,#32171,#32172,
#32173,#32174,#32175,#32176,#32177,#32178),.UNSPECIFIED.,.F.,.F.,(4,1,1,
1,1,1,1,1,4),(78.5398163397448,78.6988619941132,79.6964333670961,80.694004740079,
81.691576113062,82.6891474860449,83.6867188590278,84.6842902320108,84.8230016469244),
 .UNSPECIFIED.);
#3602=B_SPLINE_CURVE_WITH_KNOTS('',3,(#32179,#32180,#32181,#32182,#32183,
#32184,#32185,#32186,#32187,#32188),.UNSPECIFIED.,.F.,.F.,(4,1,1,1,1,1,
1,4),(78.5398163397448,79.2402802566675,80.2378516296505,81.2354230026334,
82.2329943756163,83.2305657485993,84.2281371215822,84.8230016469244),
 .UNSPECIFIED.);
#3603=B_SPLINE_CURVE_WITH_KNOTS('',3,(#32193,#32194,#32195,#32196,#32197,
#32198,#32199,#32200,#32201,#32202),.UNSPECIFIED.,.F.,.F.,(4,1,1,1,1,1,
1,4),(72.2566310325652,72.7134337562156,73.7110051291985,74.7085765021814,
75.7061478751644,76.7037192481473,77.7012906211302,78.5398163397448),
 .UNSPECIFIED.);
#3604=B_SPLINE_CURVE_WITH_KNOTS('',3,(#32203,#32204,#32205,#32206,#32207,
#32208,#32209,#32210,#32211,#32212,#32213),.UNSPECIFIED.,.F.,.F.,(4,1,1,
1,1,1,1,1,4),(72.2566310325652,72.257280645787,73.25485201877,74.2524233917529,
75.2499947647358,76.2475661377187,77.2451375107017,78.2427088836846,78.5398163397448),
 .UNSPECIFIED.);
#3605=B_SPLINE_CURVE_WITH_KNOTS('',3,(#32218,#32219,#32220,#32221,#32222,
#32223,#32224,#32225,#32226,#32227),.UNSPECIFIED.,.F.,.F.,(4,1,1,1,1,1,
1,4),(65.9734457253856,66.728005518318,67.7255768913009,68.7231482642838,
69.7207196372668,70.7182910102497,71.7158623832326,72.2566310325652),
 .UNSPECIFIED.);
#3606=B_SPLINE_CURVE_WITH_KNOTS('',3,(#32228,#32229,#32230,#32231,#32232,
#32233,#32234,#32235,#32236,#32237),.UNSPECIFIED.,.F.,.F.,(4,1,1,1,1,1,
1,4),(65.9734457253856,66.2718524078894,67.2694237808724,68.2669951538553,
69.2645665268382,70.2621378998212,71.2597092728041,72.2566310325652),
 .UNSPECIFIED.);
#3607=B_SPLINE_CURVE_WITH_KNOTS('',3,(#32242,#32243,#32244,#32245,#32246,
#32247,#32248,#32249,#32250,#32251,#32252),.UNSPECIFIED.,.F.,.F.,(4,1,1,
1,1,1,1,1,4),(59.690260418206,59.7450059074374,60.7425772804204,61.7401486534033,
62.7377200263862,63.7352913993692,64.7328627723521,65.730434145335,65.9734457253856),
 .UNSPECIFIED.);
#3608=B_SPLINE_CURVE_WITH_KNOTS('',3,(#32253,#32254,#32255,#32256,#32257,
#32258,#32259,#32260,#32261,#32262),.UNSPECIFIED.,.F.,.F.,(4,1,1,1,1,1,
1,4),(59.690260418206,60.2864241699918,61.2839955429748,62.2815669159577,
63.2791382889406,64.2767096619236,65.2742810349065,65.9734457253856),
 .UNSPECIFIED.);
#3609=B_SPLINE_CURVE_WITH_KNOTS('',3,(#32267,#32268,#32269,#32270,#32271,
#32272,#32273,#32274,#32275,#32276),.UNSPECIFIED.,.F.,.F.,(4,1,1,1,1,1,
1,4),(53.4070751110264,53.7595776695399,54.7571490425228,55.7547204155057,
56.7522917884886,57.7498631614716,58.7474345344545,59.690260418206),
 .UNSPECIFIED.);
#3610=B_SPLINE_CURVE_WITH_KNOTS('',3,(#32277,#32278,#32279,#32280,#32281,
#32282,#32283,#32284,#32285,#32286),.UNSPECIFIED.,.F.,.F.,(4,1,1,1,1,1,
1,4),(53.4070751110264,54.3009959320942,55.2985673050772,56.2961386780601,
57.293710051043,58.291281424026,59.2888527970089,59.690260418206),
 .UNSPECIFIED.);
#3611=B_SPLINE_CURVE_WITH_KNOTS('',3,(#32291,#32292,#32293,#32294,#32295,
#32296,#32297,#32298,#32299,#32300),.UNSPECIFIED.,.F.,.F.,(4,1,1,1,1,1,
1,4),(47.1238898038468,47.7741494316423,48.7717208046252,49.7692921776081,
50.7668635505911,51.764434923574,52.7620062965569,53.4070751110264),
 .UNSPECIFIED.);
#3612=B_SPLINE_CURVE_WITH_KNOTS('',3,(#32301,#32302,#32303,#32304,#32305,
#32306,#32307,#32308,#32309,#32310,#32311),.UNSPECIFIED.,.F.,.F.,(4,1,1,
1,1,1,1,1,4),(47.1238898038468,47.3179963212137,48.3155676941966,49.3131390671796,
50.3107104401625,51.3082818131454,52.3058531861284,53.3034245591113,53.4070751110264),
 .UNSPECIFIED.);
#3613=B_SPLINE_CURVE_WITH_KNOTS('',3,(#32316,#32317,#32318,#32319,#32320,
#32321,#32322,#32323,#32324,#32325),.UNSPECIFIED.,.F.,.F.,(4,1,1,1,1,1,
1,4),(40.8407044966673,41.7887211937447,42.7862925667276,43.7838639397105,
44.7814353126935,45.7790066856764,46.7765780586593,47.1238898038468),
 .UNSPECIFIED.);
#3614=B_SPLINE_CURVE_WITH_KNOTS('',3,(#32326,#32327,#32328,#32329,#32330,
#32331,#32332,#32333,#32334,#32335),.UNSPECIFIED.,.F.,.F.,(4,1,1,1,1,1,
1,4),(40.8407044966673,41.3325680833161,42.330139456299,43.327710829282,
44.3252822022649,45.3228535752478,46.3204249482308,47.1238898038468),
 .UNSPECIFIED.);
#3615=B_SPLINE_CURVE_WITH_KNOTS('',3,(#32340,#32341,#32342,#32343,#32344,
#32345,#32346,#32347,#32348,#32349,#32350),.UNSPECIFIED.,.F.,.F.,(4,1,1,
1,1,1,1,1,4),(34.5575191894876,34.8057215828641,35.8032929558471,36.80086432883,
37.7984357018129,38.7960070747959,39.7935784477788,40.7911498207617,40.8407044966673),
 .UNSPECIFIED.);
#3616=B_SPLINE_CURVE_WITH_KNOTS('',3,(#32351,#32352,#32353,#32354,#32355,
#32356,#32357,#32358,#32359,#32360),.UNSPECIFIED.,.F.,.F.,(4,1,1,1,1,1,
1,4),(34.5575191894876,35.3471398454185,36.3447112184014,37.3422825913844,
38.3398539643673,39.3374253373502,40.3349967103332,40.8407044966673),
 .UNSPECIFIED.);
#3617=B_SPLINE_CURVE_WITH_KNOTS('',3,(#32365,#32366,#32367,#32368,#32369,
#32370,#32371,#32372,#32373,#32374),.UNSPECIFIED.,.F.,.F.,(4,1,1,1,1,1,
1,4),(28.2743338823081,28.8202933449665,29.8178647179495,30.8154360909324,
31.8130074639153,32.8105788368983,33.8081502098812,34.5575191894876),
 .UNSPECIFIED.);
#3618=B_SPLINE_CURVE_WITH_KNOTS('',3,(#32375,#32376,#32377,#32378,#32379,
#32380,#32381,#32382,#32383,#32384,#32385),.UNSPECIFIED.,.F.,.F.,(4,1,1,
1,1,1,1,1,4),(28.2743338823081,28.364140234538,29.3617116075209,30.3592829805038,
31.3568543534868,32.3544257264697,33.3519970994526,34.3495684724356,34.5575191894876),
 .UNSPECIFIED.);
#3619=B_SPLINE_CURVE_WITH_KNOTS('',3,(#32390,#32391,#32392,#32393,#32394,
#32395,#32396,#32397,#32398,#32399),.UNSPECIFIED.,.F.,.F.,(4,1,1,1,1,1,
1,4),(21.9911485751285,22.8348651070689,23.8324364800519,24.8300078530348,
25.8275792260177,26.8251505990007,27.8227219719836,28.2743338823081),
 .UNSPECIFIED.);
#3620=B_SPLINE_CURVE_WITH_KNOTS('',3,(#32400,#32401,#32402,#32403,#32404,
#32405,#32406,#32407,#32408,#32409),.UNSPECIFIED.,.F.,.F.,(4,1,1,1,1,1,
1,4),(21.9911485751285,22.3787119966404,23.3762833696233,24.3738547426063,
25.3714261155892,26.3689974885721,27.3665688615551,28.2743338823081),
 .UNSPECIFIED.);
#3621=B_SPLINE_CURVE_WITH_KNOTS('',3,(#32415,#32416,#32417,#32418,#32419),
 .UNSPECIFIED.,.F.,.F.,(4,1,4),(14.3981410127769,15.3957123857599,15.7079632679489),
 .UNSPECIFIED.);
#3622=B_SPLINE_CURVE_WITH_KNOTS('',3,(#32422,#32423,#32424,#32425,#32426),
 .UNSPECIFIED.,.F.,.F.,(4,1,4),(13.8761928695311,14.8542941232055,15.7079632679489),
 .UNSPECIFIED.);
#3623=B_SPLINE_CURVE_WITH_KNOTS('',3,(#32432,#32433,#32434,#32435,#32436,
#32437,#32438,#32439,#32440,#32441,#32442,#32443,#32444,#32445,#32446,#32447,
#32448,#32449,#32450,#32451,#32452,#32453),.UNSPECIFIED.,.F.,.F.,(4,3,3,
3,3,3,3,4),(76.708045941327,76.8129957196858,77.8105670926687,78.8081384656517,
79.8057098386346,80.8032812116175,81.8008525846005,82.7984239575834),
 .UNSPECIFIED.);
#3624=B_SPLINE_CURVE_WITH_KNOTS('',3,(#32457,#32458,#32459,#32460,#32461,
#32462,#32463),.UNSPECIFIED.,.F.,.F.,(4,3,4),(-80.783811092309,-79.8057098386346,
-79.2446069498473),.UNSPECIFIED.);
#3625=B_SPLINE_CURVE_WITH_KNOTS('',3,(#32467,#32468,#32469,#32470,#32471,
#32472,#32473,#32474,#32475,#32476,#32477,#32478,#32479,#32480,#32481,#32482,
#32483,#32484,#32485,#32486,#32487,#32488),.UNSPECIFIED.,.F.,.F.,(4,3,3,
3,3,3,3,4),(-79.2446069498473,-78.8081384656517,-77.8105670926687,-76.8129957196858,
-75.8154243467029,-74.81785297372,-73.820281600737,-72.9614216426677),
 .UNSPECIFIED.);
#3626=B_SPLINE_CURVE_WITH_KNOTS('',3,(#32493,#32494,#32495,#32496,#32497,
#32498,#32499,#32500,#32501,#32502,#32503,#32504,#32505,#32506,#32507,#32508,
#32509,#32510,#32511,#32512,#32513,#32514),.UNSPECIFIED.,.F.,.F.,(4,3,3,
3,3,3,3,4),(70.4248606341474,70.8275674817882,71.8251388547712,72.8227102277541,
73.820281600737,74.81785297372,75.8154243467029,76.708045941327),
 .UNSPECIFIED.);
#3627=B_SPLINE_CURVE_WITH_KNOTS('',3,(#32515,#32516,#32517,#32518,#32519,
#32520,#32521,#32522,#32523,#32524,#32525,#32526,#32527,#32528,#32529,#32530,
#32531,#32532,#32533,#32534,#32535,#32536,#32537,#32538,#32539),
 .UNSPECIFIED.,.F.,.F.,(4,3,3,3,3,3,3,3,4),(-72.9614216426677,-72.8227102277541,
-71.8251388547712,-70.8275674817882,-69.8299961088053,-68.8324247358224,
-67.8348533628394,-66.8372819898565,-66.6782363354882),.UNSPECIFIED.);
#3628=B_SPLINE_CURVE_WITH_KNOTS('',3,(#32544,#32545,#32546,#32547,#32548,
#32549,#32550,#32551,#32552,#32553,#32554,#32555,#32556,#32557,#32558,#32559,
#32560,#32561,#32562,#32563,#32564,#32565),.UNSPECIFIED.,.F.,.F.,(4,3,3,
3,3,3,3,4),(64.1416753269678,64.8421392438906,65.8397106168736,66.8372819898565,
67.8348533628394,68.8324247358224,69.8299961088053,70.4248606341474),
 .UNSPECIFIED.);
#3629=B_SPLINE_CURVE_WITH_KNOTS('',3,(#32566,#32567,#32568,#32569,#32570,
#32571,#32572,#32573,#32574,#32575,#32576,#32577,#32578,#32579,#32580,#32581,
#32582,#32583,#32584,#32585,#32586,#32587),.UNSPECIFIED.,.F.,.F.,(4,3,3,
3,3,3,3,4),(-66.6782363354882,-65.8397106168736,-64.8421392438906,-63.8445678709077,
-62.8469964979248,-61.8494251249418,-60.8518537519589,-60.3950510283085),
 .UNSPECIFIED.);
#3630=B_SPLINE_CURVE_WITH_KNOTS('',3,(#32592,#32593,#32594,#32595,#32596,
#32597,#32598,#32599,#32600,#32601,#32602,#32603,#32604,#32605,#32606,#32607,
#32608,#32609,#32610,#32611,#32612,#32613),.UNSPECIFIED.,.F.,.F.,(4,3,3,
3,3,3,3,4),(57.8584900197882,58.856711005993,59.854282378976,60.8518537519589,
61.8494251249418,62.8469964979248,63.8445678709077,64.1416753269678),
 .UNSPECIFIED.);
#3631=B_SPLINE_CURVE_WITH_KNOTS('',3,(#32614,#32615,#32616,#32617,#32618,
#32619,#32620,#32621,#32622,#32623,#32624,#32625,#32626,#32627,#32628,#32629,
#32630,#32631,#32632,#32633,#32634,#32635),.UNSPECIFIED.,.F.,.F.,(4,3,3,
3,3,3,3,4),(-60.3950510283085,-59.854282378976,-58.856711005993,-57.8591396330101,
-56.8615682600272,-55.8639968870442,-54.8664255140613,-54.111865721129),
 .UNSPECIFIED.);
#3632=B_SPLINE_CURVE_WITH_KNOTS('',3,(#32640,#32641,#32642,#32643,#32644,
#32645,#32646,#32647,#32648,#32649,#32650,#32651,#32652,#32653,#32654,#32655,
#32656,#32657,#32658,#32659,#32660,#32661),.UNSPECIFIED.,.F.,.F.,(4,3,3,
3,3,3,3,4),(51.5753047126086,51.8737113951125,52.8712827680954,53.8688541410784,
54.8664255140613,55.8639968870442,56.8615682600272,57.8584900197882),
 .UNSPECIFIED.);
#3633=B_SPLINE_CURVE_WITH_KNOTS('',3,(#32662,#32663,#32664,#32665,#32666,
#32667,#32668,#32669,#32670,#32671,#32672,#32673,#32674,#32675,#32676,#32677,
#32678,#32679,#32680,#32681,#32682,#32683,#32684,#32685,#32686),
 .UNSPECIFIED.,.F.,.F.,(4,3,3,3,3,3,3,3,4),(-54.111865721129,-53.8688541410784,
-52.8712827680954,-51.8737113951125,-50.8761400221296,-49.8785686491466,
-48.8809972761637,-47.8834259031808,-47.8286804139494),.UNSPECIFIED.);
#3634=B_SPLINE_CURVE_WITH_KNOTS('',3,(#32691,#32692,#32693,#32694,#32695,
#32696,#32697,#32698,#32699,#32700,#32701,#32702,#32703,#32704,#32705,#32706,
#32707,#32708,#32709,#32710,#32711,#32712),.UNSPECIFIED.,.F.,.F.,(4,3,3,
3,3,3,3,4),(45.2921194054291,45.8882831572149,46.8858545301978,47.8834259031808,
48.8809972761637,49.8785686491466,50.8761400221296,51.5753047126086),
 .UNSPECIFIED.);
#3635=B_SPLINE_CURVE_WITH_KNOTS('',3,(#32713,#32714,#32715,#32716,#32717,
#32718,#32719,#32720,#32721,#32722,#32723,#32724,#32725,#32726,#32727,#32728,
#32729,#32730,#32731,#32732,#32733,#32734),.UNSPECIFIED.,.F.,.F.,(4,3,3,
3,3,3,3,4),(-47.8286804139494,-46.8858545301978,-45.8882831572149,-44.890711784232,
-43.893140411249,-42.8955690382661,-41.8979976652832,-41.5454951067698),
 .UNSPECIFIED.);
#3636=B_SPLINE_CURVE_WITH_KNOTS('',3,(#32739,#32740,#32741,#32742,#32743,
#32744,#32745,#32746,#32747,#32748,#32749,#32750,#32751,#32752,#32753,#32754,
#32755,#32756,#32757,#32758,#32759,#32760),.UNSPECIFIED.,.F.,.F.,(4,3,3,
3,3,3,3,4),(39.0089340982495,39.9028549193173,40.9004262923002,41.8979976652832,
42.8955690382661,43.893140411249,44.890711784232,45.2921194054291),
 .UNSPECIFIED.);
#3637=B_SPLINE_CURVE_WITH_KNOTS('',3,(#32761,#32762,#32763,#32764,#32765,
#32766,#32767,#32768,#32769,#32770,#32771,#32772,#32773,#32774,#32775,#32776,
#32777,#32778,#32779,#32780,#32781,#32782),.UNSPECIFIED.,.F.,.F.,(4,3,3,
3,3,3,3,4),(-41.5454951067698,-40.9004262923002,-39.9028549193173,-38.9052835463344,
-37.9077121733514,-36.9101408003685,-35.9125694273856,-35.2623097995902),
 .UNSPECIFIED.);
#3638=B_SPLINE_CURVE_WITH_KNOTS('',3,(#32787,#32788,#32789,#32790,#32791,
#32792,#32793,#32794,#32795,#32796,#32797,#32798,#32799,#32800,#32801,#32802,
#32803,#32804,#32805,#32806,#32807,#32808,#32809,#32810,#32811),
 .UNSPECIFIED.,.F.,.F.,(4,3,3,3,3,3,3,3,4),(32.7257487910699,32.9198553084368,
33.9174266814197,34.9149980544027,35.9125694273856,36.9101408003685,37.9077121733514,
38.9052835463344,39.0089340982495),.UNSPECIFIED.);
#3639=B_SPLINE_CURVE_WITH_KNOTS('',3,(#32812,#32813,#32814,#32815,#32816,
#32817,#32818,#32819,#32820,#32821,#32822,#32823,#32824,#32825,#32826,#32827,
#32828,#32829,#32830,#32831,#32832,#32833),.UNSPECIFIED.,.F.,.F.,(4,3,3,
3,3,3,3,4),(-35.2623097995902,-34.9149980544026,-33.9174266814197,-32.9198553084368,
-31.9222839354538,-30.9247125624709,-29.927141189488,-28.9791244924106),
 .UNSPECIFIED.);
#3640=B_SPLINE_CURVE_WITH_KNOTS('',3,(#32838,#32839,#32840,#32841,#32842,
#32843,#32844,#32845,#32846,#32847,#32848,#32849,#32850,#32851,#32852,#32853,
#32854,#32855,#32856,#32857,#32858,#32859),.UNSPECIFIED.,.F.,.F.,(4,3,3,
3,3,3,3,4),(26.4425634838903,26.9344270705392,27.9319984435221,28.9295698165051,
29.927141189488,30.9247125624709,31.9222839354539,32.7257487910699),
 .UNSPECIFIED.);
#3641=B_SPLINE_CURVE_WITH_KNOTS('',3,(#32860,#32861,#32862,#32863,#32864,
#32865,#32866,#32867,#32868,#32869,#32870,#32871,#32872,#32873,#32874,#32875,
#32876,#32877,#32878,#32879,#32880,#32881,#32882,#32883,#32884),
 .UNSPECIFIED.,.F.,.F.,(4,3,3,3,3,3,3,3,4),(-28.9791244924106,-28.9295698165051,
-27.9319984435221,-26.9344270705392,-25.9368556975562,-24.9392843245733,
-23.9417129515904,-22.9441415786074,-22.695939185231),.UNSPECIFIED.);
#3642=B_SPLINE_CURVE_WITH_KNOTS('',3,(#32889,#32890,#32891,#32892,#32893,
#32894,#32895,#32896,#32897,#32898,#32899,#32900,#32901,#32902,#32903,#32904,
#32905,#32906,#32907,#32908,#32909,#32910),.UNSPECIFIED.,.F.,.F.,(4,3,3,
3,3,3,3,4),(20.1593781767107,20.9489988326416,21.9465702056245,22.9441415786075,
23.9417129515904,24.9392843245733,25.9368556975563,26.4425634838903),
 .UNSPECIFIED.);
#3643=B_SPLINE_CURVE_WITH_KNOTS('',3,(#32911,#32912,#32913,#32914,#32915,
#32916,#32917,#32918,#32919,#32920,#32921,#32922,#32923,#32924,#32925,#32926,
#32927,#32928,#32929,#32930,#32931,#32932),.UNSPECIFIED.,.F.,.F.,(4,3,3,
3,3,3,3,4),(-22.695939185231,-21.9465702056245,-20.9489988326416,-19.9514274596587,
-18.9538560866757,-17.9562847136928,-16.9587133407099,-16.4127538780514),
 .UNSPECIFIED.);
#3644=B_SPLINE_CURVE_WITH_KNOTS('',3,(#32937,#32938,#32939,#32940,#32941,
#32942,#32943,#32944,#32945,#32946,#32947,#32948,#32949,#32950,#32951,#32952,
#32953,#32954,#32955,#32956,#32957,#32958,#32959,#32960,#32961),
 .UNSPECIFIED.,.F.,.F.,(4,3,3,3,3,3,3,3,4),(13.8761928695311,13.9659992217611,
14.963570594744,15.9611419677269,16.9587133407099,17.9562847136928,18.9538560866757,
19.9514274596587,20.1593781767107),.UNSPECIFIED.);
#3645=B_SPLINE_CURVE_WITH_KNOTS('',3,(#32962,#32963,#32964,#32965,#32966,
#32967,#32968,#32969,#32970,#32971,#32972,#32973,#32974,#32975,#32976,#32977,
#32978,#32979,#32980,#32981,#32982,#32983),.UNSPECIFIED.,.F.,.F.,(4,3,3,
3,3,3,3,4),(-16.4127538780514,-15.9611419677269,-14.963570594744,-13.9659992217611,
-12.9684278487781,-11.9708564757952,-10.9732851028123,-10.1295685708718),
 .UNSPECIFIED.);
#3646=B_SPLINE_CURVE_WITH_KNOTS('',3,(#32989,#32990,#32991,#32992,#32993,
#32994,#32995,#32996,#32997,#32998,#32999,#33000,#33001),.UNSPECIFIED.,
 .F.,.F.,(4,3,3,3,4),(-3.84638326369223,-2.9927141189488,-1.99514274596586,
-0.997571372982932,0.),.UNSPECIFIED.);
#3647=B_SPLINE_CURVE_WITH_KNOTS('',3,(#33004,#33005,#33006,#33007,#33008,
#33009,#33010,#33011,#33012,#33013,#33014,#33015,#33016,#33017,#33018,#33019,
#33020,#33021,#33022),.UNSPECIFIED.,.F.,.F.,(4,3,3,3,3,3,4),(2.01461286527439,
2.9927141189488,3.99028549193173,4.98785686491467,5.9854282378976,6.98299961088053,
7.59300756235152),.UNSPECIFIED.);
#3648=B_SPLINE_CURVE_WITH_KNOTS('',3,(#33028,#33029,#33030,#33031,#33032,
#33033,#33034),.UNSPECIFIED.,.F.,.F.,(4,1,1,1,4),(91.106186954104,91.6672898428913,
92.6648612158742,93.6624325888571,94.6600039618401),.UNSPECIFIED.);
#3649=B_SPLINE_CURVE_WITH_KNOTS('',3,(#33037,#33038,#33039,#33040,#33041,
#33042,#33043,#33044),.UNSPECIFIED.,.F.,.F.,(4,1,1,1,1,4),(91.106186954104,
91.2111367324627,92.2087081054457,93.2062794784286,94.2038508514115,95.1819521050859),
 .UNSPECIFIED.);
#3650=B_SPLINE_CURVE_WITH_KNOTS('',3,(#33049,#33050,#33051,#33052,#33053,
#33054,#33055,#33056,#33057,#33058),.UNSPECIFIED.,.F.,.F.,(4,1,1,1,1,1,
1,4),(84.8230016469244,85.6818616049937,86.6794329779766,87.6770043509595,
88.6745757239425,89.6721470969254,90.6697184699083,91.106186954104),
 .UNSPECIFIED.);
#3651=B_SPLINE_CURVE_WITH_KNOTS('',3,(#33059,#33060,#33061,#33062,#33063,
#33064,#33065,#33066,#33067,#33068),.UNSPECIFIED.,.F.,.F.,(4,1,1,1,1,1,
1,4),(84.8230016469244,85.2257084945651,86.2232798675481,87.220851240531,
88.2184226135139,89.2159939864969,90.2135653594798,91.106186954104),
 .UNSPECIFIED.);
#3652=B_SPLINE_CURVE_WITH_KNOTS('',3,(#33073,#33074,#33075,#33076,#33077,
#33078,#33079,#33080,#33081,#33082,#33083),.UNSPECIFIED.,.F.,.F.,(4,1,1,
1,1,1,1,1,4),(78.5398163397448,78.6988619941132,79.6964333670961,80.694004740079,
81.691576113062,82.6891474860449,83.6867188590278,84.6842902320108,84.8230016469244),
 .UNSPECIFIED.);
#3653=B_SPLINE_CURVE_WITH_KNOTS('',3,(#33084,#33085,#33086,#33087,#33088,
#33089,#33090,#33091,#33092,#33093),.UNSPECIFIED.,.F.,.F.,(4,1,1,1,1,1,
1,4),(78.5398163397448,79.2402802566675,80.2378516296505,81.2354230026334,
82.2329943756163,83.2305657485993,84.2281371215822,84.8230016469244),
 .UNSPECIFIED.);
#3654=B_SPLINE_CURVE_WITH_KNOTS('',3,(#33098,#33099,#33100,#33101,#33102,
#33103,#33104,#33105,#33106,#33107),.UNSPECIFIED.,.F.,.F.,(4,1,1,1,1,1,
1,4),(72.2566310325652,72.7134337562156,73.7110051291985,74.7085765021814,
75.7061478751644,76.7037192481473,77.7012906211302,78.5398163397448),
 .UNSPECIFIED.);
#3655=B_SPLINE_CURVE_WITH_KNOTS('',3,(#33108,#33109,#33110,#33111,#33112,
#33113,#33114,#33115,#33116,#33117,#33118),.UNSPECIFIED.,.F.,.F.,(4,1,1,
1,1,1,1,1,4),(72.2566310325652,72.257280645787,73.25485201877,74.2524233917529,
75.2499947647358,76.2475661377187,77.2451375107017,78.2427088836846,78.5398163397448),
 .UNSPECIFIED.);
#3656=B_SPLINE_CURVE_WITH_KNOTS('',3,(#33123,#33124,#33125,#33126,#33127,
#33128,#33129,#33130,#33131,#33132),.UNSPECIFIED.,.F.,.F.,(4,1,1,1,1,1,
1,4),(65.9734457253856,66.728005518318,67.7255768913009,68.7231482642838,
69.7207196372668,70.7182910102497,71.7158623832326,72.2566310325652),
 .UNSPECIFIED.);
#3657=B_SPLINE_CURVE_WITH_KNOTS('',3,(#33133,#33134,#33135,#33136,#33137,
#33138,#33139,#33140,#33141,#33142),.UNSPECIFIED.,.F.,.F.,(4,1,1,1,1,1,
1,4),(65.9734457253856,66.2718524078894,67.2694237808723,68.2669951538553,
69.2645665268382,70.2621378998211,71.2597092728041,72.2566310325652),
 .UNSPECIFIED.);
#3658=B_SPLINE_CURVE_WITH_KNOTS('',3,(#33147,#33148,#33149,#33150,#33151,
#33152,#33153,#33154,#33155,#33156,#33157),.UNSPECIFIED.,.F.,.F.,(4,1,1,
1,1,1,1,1,4),(59.690260418206,59.7450059074374,60.7425772804204,61.7401486534033,
62.7377200263862,63.7352913993692,64.7328627723521,65.730434145335,65.9734457253856),
 .UNSPECIFIED.);
#3659=B_SPLINE_CURVE_WITH_KNOTS('',3,(#33158,#33159,#33160,#33161,#33162,
#33163,#33164,#33165,#33166,#33167),.UNSPECIFIED.,.F.,.F.,(4,1,1,1,1,1,
1,4),(59.690260418206,60.2864241699918,61.2839955429748,62.2815669159577,
63.2791382889406,64.2767096619235,65.2742810349065,65.9734457253856),
 .UNSPECIFIED.);
#3660=B_SPLINE_CURVE_WITH_KNOTS('',3,(#33172,#33173,#33174,#33175,#33176,
#33177,#33178,#33179,#33180,#33181),.UNSPECIFIED.,.F.,.F.,(4,1,1,1,1,1,
1,4),(53.4070751110265,53.7595776695398,54.7571490425228,55.7547204155057,
56.7522917884886,57.7498631614716,58.7474345344545,59.690260418206),
 .UNSPECIFIED.);
#3661=B_SPLINE_CURVE_WITH_KNOTS('',3,(#33182,#33183,#33184,#33185,#33186,
#33187,#33188,#33189,#33190,#33191),.UNSPECIFIED.,.F.,.F.,(4,1,1,1,1,1,
1,4),(53.4070751110264,54.3009959320942,55.2985673050772,56.2961386780601,
57.293710051043,58.291281424026,59.2888527970089,59.690260418206),
 .UNSPECIFIED.);
#3662=B_SPLINE_CURVE_WITH_KNOTS('',3,(#33196,#33197,#33198,#33199,#33200,
#33201,#33202,#33203,#33204,#33205),.UNSPECIFIED.,.F.,.F.,(4,1,1,1,1,1,
1,4),(47.1238898038469,47.7741494316422,48.7717208046252,49.7692921776081,
50.766863550591,51.764434923574,52.7620062965569,53.4070751110265),
 .UNSPECIFIED.);
#3663=B_SPLINE_CURVE_WITH_KNOTS('',3,(#33206,#33207,#33208,#33209,#33210,
#33211,#33212,#33213,#33214,#33215,#33216),.UNSPECIFIED.,.F.,.F.,(4,1,1,
1,1,1,1,1,4),(47.1238898038468,47.3179963212137,48.3155676941966,49.3131390671796,
50.3107104401625,51.3082818131454,52.3058531861284,53.3034245591113,53.4070751110264),
 .UNSPECIFIED.);
#3664=B_SPLINE_CURVE_WITH_KNOTS('',3,(#33221,#33222,#33223,#33224,#33225,
#33226,#33227,#33228,#33229,#33230),.UNSPECIFIED.,.F.,.F.,(4,1,1,1,1,1,
1,4),(40.8407044966673,41.7887211937446,42.7862925667276,43.7838639397105,
44.7814353126934,45.7790066856764,46.7765780586593,47.1238898038469),
 .UNSPECIFIED.);
#3665=B_SPLINE_CURVE_WITH_KNOTS('',3,(#33231,#33232,#33233,#33234,#33235,
#33236,#33237,#33238,#33239,#33240),.UNSPECIFIED.,.F.,.F.,(4,1,1,1,1,1,
1,4),(40.8407044966673,41.3325680833161,42.330139456299,43.327710829282,
44.3252822022649,45.3228535752478,46.3204249482308,47.1238898038468),
 .UNSPECIFIED.);
#3666=B_SPLINE_CURVE_WITH_KNOTS('',3,(#33245,#33246,#33247,#33248,#33249,
#33250,#33251,#33252,#33253,#33254,#33255),.UNSPECIFIED.,.F.,.F.,(4,1,1,
1,1,1,1,1,4),(34.5575191894877,34.8057215828641,35.803292955847,36.80086432883,
37.7984357018129,38.7960070747959,39.7935784477788,40.7911498207617,40.8407044966673),
 .UNSPECIFIED.);
#3667=B_SPLINE_CURVE_WITH_KNOTS('',3,(#33256,#33257,#33258,#33259,#33260,
#33261,#33262,#33263,#33264,#33265),.UNSPECIFIED.,.F.,.F.,(4,1,1,1,1,1,
1,4),(34.5575191894876,35.3471398454185,36.3447112184014,37.3422825913844,
38.3398539643673,39.3374253373502,40.3349967103332,40.8407044966673),
 .UNSPECIFIED.);
#3668=B_SPLINE_CURVE_WITH_KNOTS('',3,(#33270,#33271,#33272,#33273,#33274,
#33275,#33276,#33277,#33278,#33279),.UNSPECIFIED.,.F.,.F.,(4,1,1,1,1,1,
1,4),(28.2743338823081,28.8202933449665,29.8178647179495,30.8154360909324,
31.8130074639153,32.8105788368983,33.8081502098812,34.5575191894877),
 .UNSPECIFIED.);
#3669=B_SPLINE_CURVE_WITH_KNOTS('',3,(#33280,#33281,#33282,#33283,#33284,
#33285,#33286,#33287,#33288,#33289,#33290),.UNSPECIFIED.,.F.,.F.,(4,1,1,
1,1,1,1,1,4),(28.2743338823081,28.364140234538,29.3617116075209,30.3592829805038,
31.3568543534868,32.3544257264697,33.3519970994526,34.3495684724356,34.5575191894876),
 .UNSPECIFIED.);
#3670=B_SPLINE_CURVE_WITH_KNOTS('',3,(#33295,#33296,#33297,#33298,#33299,
#33300,#33301,#33302,#33303,#33304),.UNSPECIFIED.,.F.,.F.,(4,1,1,1,1,1,
1,4),(21.9911485751285,22.8348651070689,23.8324364800519,24.8300078530348,
25.8275792260177,26.8251505990007,27.8227219719836,28.2743338823081),
 .UNSPECIFIED.);
#3671=B_SPLINE_CURVE_WITH_KNOTS('',3,(#33305,#33306,#33307,#33308,#33309,
#33310,#33311,#33312,#33313,#33314),.UNSPECIFIED.,.F.,.F.,(4,1,1,1,1,1,
1,4),(21.9911485751285,22.3787119966404,23.3762833696233,24.3738547426062,
25.3714261155892,26.3689974885721,27.366568861555,28.2743338823081),
 .UNSPECIFIED.);
#3672=B_SPLINE_CURVE_WITH_KNOTS('',3,(#33320,#33321,#33322,#33323,#33324),
 .UNSPECIFIED.,.F.,.F.,(4,1,4),(14.3981410127769,15.3957123857599,15.7079632679489),
 .UNSPECIFIED.);
#3673=B_SPLINE_CURVE_WITH_KNOTS('',3,(#33327,#33328,#33329,#33330,#33331),
 .UNSPECIFIED.,.F.,.F.,(4,1,4),(13.8761928695311,14.8542941232055,15.7079632679489),
 .UNSPECIFIED.);
#3674=B_SPLINE_CURVE_WITH_KNOTS('',3,(#33337,#33338,#33339,#33340,#33341,
#33342,#33343,#33344,#33345,#33346,#33347,#33348,#33349,#33350,#33351,#33352,
#33353,#33354,#33355,#33356,#33357,#33358),.UNSPECIFIED.,.F.,.F.,(4,3,3,
3,3,3,3,4),(76.708045941327,76.8129957196858,77.8105670926687,78.8081384656517,
79.8057098386346,80.8032812116175,81.8008525846005,82.7984239575834),
 .UNSPECIFIED.);
#3675=B_SPLINE_CURVE_WITH_KNOTS('',3,(#33362,#33363,#33364,#33365,#33366,
#33367,#33368),.UNSPECIFIED.,.F.,.F.,(4,3,4),(-80.783811092309,-79.8057098386346,
-79.2446069498473),.UNSPECIFIED.);
#3676=B_SPLINE_CURVE_WITH_KNOTS('',3,(#33372,#33373,#33374,#33375,#33376,
#33377,#33378,#33379,#33380,#33381,#33382,#33383,#33384,#33385,#33386,#33387,
#33388,#33389,#33390,#33391,#33392,#33393),.UNSPECIFIED.,.F.,.F.,(4,3,3,
3,3,3,3,4),(-79.2446069498473,-78.8081384656517,-77.8105670926688,-76.8129957196858,
-75.8154243467029,-74.81785297372,-73.820281600737,-72.9614216426677),
 .UNSPECIFIED.);
#3677=B_SPLINE_CURVE_WITH_KNOTS('',3,(#33398,#33399,#33400,#33401,#33402,
#33403,#33404,#33405,#33406,#33407,#33408,#33409,#33410,#33411,#33412,#33413,
#33414,#33415,#33416,#33417,#33418,#33419),.UNSPECIFIED.,.F.,.F.,(4,3,3,
3,3,3,3,4),(70.4248606341474,70.8275674817882,71.8251388547711,72.8227102277541,
73.820281600737,74.8178529737199,75.8154243467029,76.708045941327),
 .UNSPECIFIED.);
#3678=B_SPLINE_CURVE_WITH_KNOTS('',3,(#33420,#33421,#33422,#33423,#33424,
#33425,#33426,#33427,#33428,#33429,#33430,#33431,#33432,#33433,#33434,#33435,
#33436,#33437,#33438,#33439,#33440,#33441,#33442,#33443,#33444),
 .UNSPECIFIED.,.F.,.F.,(4,3,3,3,3,3,3,3,4),(-72.9614216426677,-72.8227102277541,
-71.8251388547712,-70.8275674817882,-69.8299961088053,-68.8324247358224,
-67.8348533628394,-66.8372819898565,-66.6782363354882),.UNSPECIFIED.);
#3679=B_SPLINE_CURVE_WITH_KNOTS('',3,(#33449,#33450,#33451,#33452,#33453,
#33454,#33455,#33456,#33457,#33458,#33459,#33460,#33461,#33462,#33463,#33464,
#33465,#33466,#33467,#33468,#33469,#33470),.UNSPECIFIED.,.F.,.F.,(4,3,3,
3,3,3,3,4),(64.1416753269678,64.8421392438906,65.8397106168736,66.8372819898565,
67.8348533628394,68.8324247358223,69.8299961088053,70.4248606341474),
 .UNSPECIFIED.);
#3680=B_SPLINE_CURVE_WITH_KNOTS('',3,(#33471,#33472,#33473,#33474,#33475,
#33476,#33477,#33478,#33479,#33480,#33481,#33482,#33483,#33484,#33485,#33486,
#33487,#33488,#33489,#33490,#33491,#33492),.UNSPECIFIED.,.F.,.F.,(4,3,3,
3,3,3,3,4),(-66.6782363354882,-65.8397106168736,-64.8421392438906,-63.8445678709077,
-62.8469964979248,-61.8494251249418,-60.8518537519589,-60.3950510283085),
 .UNSPECIFIED.);
#3681=B_SPLINE_CURVE_WITH_KNOTS('',3,(#33497,#33498,#33499,#33500,#33501,
#33502,#33503,#33504,#33505,#33506,#33507,#33508,#33509,#33510,#33511,#33512,
#33513,#33514,#33515,#33516,#33517,#33518),.UNSPECIFIED.,.F.,.F.,(4,3,3,
3,3,3,3,4),(57.8584900197882,58.856711005993,59.854282378976,60.8518537519589,
61.8494251249418,62.8469964979247,63.8445678709077,64.1416753269678),
 .UNSPECIFIED.);
#3682=B_SPLINE_CURVE_WITH_KNOTS('',3,(#33519,#33520,#33521,#33522,#33523,
#33524,#33525,#33526,#33527,#33528,#33529,#33530,#33531,#33532,#33533,#33534,
#33535,#33536,#33537,#33538,#33539,#33540),.UNSPECIFIED.,.F.,.F.,(4,3,3,
3,3,3,3,4),(-60.3950510283085,-59.854282378976,-58.856711005993,-57.8591396330101,
-56.8615682600272,-55.8639968870442,-54.8664255140613,-54.111865721129),
 .UNSPECIFIED.);
#3683=B_SPLINE_CURVE_WITH_KNOTS('',3,(#33545,#33546,#33547,#33548,#33549,
#33550,#33551,#33552,#33553,#33554,#33555,#33556,#33557,#33558,#33559,#33560,
#33561,#33562,#33563,#33564,#33565,#33566),.UNSPECIFIED.,.F.,.F.,(4,3,3,
3,3,3,3,4),(51.5753047126087,51.8737113951125,52.8712827680954,53.8688541410784,
54.8664255140613,55.8639968870442,56.8615682600272,57.8584900197882),
 .UNSPECIFIED.);
#3684=B_SPLINE_CURVE_WITH_KNOTS('',3,(#33567,#33568,#33569,#33570,#33571,
#33572,#33573,#33574,#33575,#33576,#33577,#33578,#33579,#33580,#33581,#33582,
#33583,#33584,#33585,#33586,#33587,#33588,#33589,#33590,#33591),
 .UNSPECIFIED.,.F.,.F.,(4,3,3,3,3,3,3,3,4),(-54.111865721129,-53.8688541410784,
-52.8712827680954,-51.8737113951125,-50.8761400221296,-49.8785686491466,
-48.8809972761637,-47.8834259031808,-47.8286804139494),.UNSPECIFIED.);
#3685=B_SPLINE_CURVE_WITH_KNOTS('',3,(#33596,#33597,#33598,#33599,#33600,
#33601,#33602,#33603,#33604,#33605,#33606,#33607,#33608,#33609,#33610,#33611,
#33612,#33613,#33614,#33615,#33616,#33617),.UNSPECIFIED.,.F.,.F.,(4,3,3,
3,3,3,3,4),(45.2921194054291,45.8882831572149,46.8858545301978,47.8834259031808,
48.8809972761637,49.8785686491466,50.8761400221295,51.5753047126087),
 .UNSPECIFIED.);
#3686=B_SPLINE_CURVE_WITH_KNOTS('',3,(#33618,#33619,#33620,#33621,#33622,
#33623,#33624,#33625,#33626,#33627,#33628,#33629,#33630,#33631,#33632,#33633,
#33634,#33635,#33636,#33637,#33638,#33639),.UNSPECIFIED.,.F.,.F.,(4,3,3,
3,3,3,3,4),(-47.8286804139494,-46.8858545301978,-45.8882831572149,-44.890711784232,
-43.893140411249,-42.8955690382661,-41.8979976652832,-41.5454951067698),
 .UNSPECIFIED.);
#3687=B_SPLINE_CURVE_WITH_KNOTS('',3,(#33644,#33645,#33646,#33647,#33648,
#33649,#33650,#33651,#33652,#33653,#33654,#33655,#33656,#33657,#33658,#33659,
#33660,#33661,#33662,#33663,#33664,#33665),.UNSPECIFIED.,.F.,.F.,(4,3,3,
3,3,3,3,4),(39.0089340982495,39.9028549193173,40.9004262923002,41.8979976652832,
42.8955690382661,43.893140411249,44.890711784232,45.2921194054291),
 .UNSPECIFIED.);
#3688=B_SPLINE_CURVE_WITH_KNOTS('',3,(#33666,#33667,#33668,#33669,#33670,
#33671,#33672,#33673,#33674,#33675,#33676,#33677,#33678,#33679,#33680,#33681,
#33682,#33683,#33684,#33685,#33686,#33687),.UNSPECIFIED.,.F.,.F.,(4,3,3,
3,3,3,3,4),(-41.5454951067698,-40.9004262923002,-39.9028549193173,-38.9052835463344,
-37.9077121733514,-36.9101408003685,-35.9125694273856,-35.2623097995902),
 .UNSPECIFIED.);
#3689=B_SPLINE_CURVE_WITH_KNOTS('',3,(#33692,#33693,#33694,#33695,#33696,
#33697,#33698,#33699,#33700,#33701,#33702,#33703,#33704,#33705,#33706,#33707,
#33708,#33709,#33710,#33711,#33712,#33713,#33714,#33715,#33716),
 .UNSPECIFIED.,.F.,.F.,(4,3,3,3,3,3,3,3,4),(32.7257487910699,32.9198553084368,
33.9174266814197,34.9149980544026,35.9125694273856,36.9101408003685,37.9077121733514,
38.9052835463344,39.0089340982495),.UNSPECIFIED.);
#3690=B_SPLINE_CURVE_WITH_KNOTS('',3,(#33717,#33718,#33719,#33720,#33721,
#33722,#33723,#33724,#33725,#33726,#33727,#33728,#33729,#33730,#33731,#33732,
#33733,#33734,#33735,#33736,#33737,#33738),.UNSPECIFIED.,.F.,.F.,(4,3,3,
3,3,3,3,4),(-35.2623097995902,-34.9149980544027,-33.9174266814197,-32.9198553084368,
-31.9222839354538,-30.9247125624709,-29.927141189488,-28.9791244924106),
 .UNSPECIFIED.);
#3691=B_SPLINE_CURVE_WITH_KNOTS('',3,(#33743,#33744,#33745,#33746,#33747,
#33748,#33749,#33750,#33751,#33752,#33753,#33754,#33755,#33756,#33757,#33758,
#33759,#33760,#33761,#33762,#33763,#33764),.UNSPECIFIED.,.F.,.F.,(4,3,3,
3,3,3,3,4),(26.4425634838903,26.9344270705392,27.9319984435221,28.929569816505,
29.927141189488,30.9247125624709,31.9222839354538,32.7257487910699),
 .UNSPECIFIED.);
#3692=B_SPLINE_CURVE_WITH_KNOTS('',3,(#33765,#33766,#33767,#33768,#33769,
#33770,#33771,#33772,#33773,#33774,#33775,#33776,#33777,#33778,#33779,#33780,
#33781,#33782,#33783,#33784,#33785,#33786,#33787,#33788,#33789),
 .UNSPECIFIED.,.F.,.F.,(4,3,3,3,3,3,3,3,4),(-28.9791244924106,-28.929569816505,
-27.9319984435221,-26.9344270705392,-25.9368556975563,-24.9392843245733,
-23.9417129515904,-22.9441415786075,-22.695939185231),.UNSPECIFIED.);
#3693=B_SPLINE_CURVE_WITH_KNOTS('',3,(#33794,#33795,#33796,#33797,#33798,
#33799,#33800,#33801,#33802,#33803,#33804,#33805,#33806,#33807,#33808,#33809,
#33810,#33811,#33812,#33813,#33814,#33815),.UNSPECIFIED.,.F.,.F.,(4,3,3,
3,3,3,3,4),(20.1593781767107,20.9489988326416,21.9465702056245,22.9441415786075,
23.9417129515904,24.9392843245733,25.9368556975563,26.4425634838903),
 .UNSPECIFIED.);
#3694=B_SPLINE_CURVE_WITH_KNOTS('',3,(#33816,#33817,#33818,#33819,#33820,
#33821,#33822,#33823,#33824,#33825,#33826,#33827,#33828,#33829,#33830,#33831,
#33832,#33833,#33834,#33835,#33836,#33837),.UNSPECIFIED.,.F.,.F.,(4,3,3,
3,3,3,3,4),(-22.695939185231,-21.9465702056245,-20.9489988326416,-19.9514274596587,
-18.9538560866757,-17.9562847136928,-16.9587133407099,-16.4127538780514),
 .UNSPECIFIED.);
#3695=B_SPLINE_CURVE_WITH_KNOTS('',3,(#33842,#33843,#33844,#33845,#33846,
#33847,#33848,#33849,#33850,#33851,#33852,#33853,#33854,#33855,#33856,#33857,
#33858,#33859,#33860,#33861,#33862,#33863,#33864,#33865,#33866),
 .UNSPECIFIED.,.F.,.F.,(4,3,3,3,3,3,3,3,4),(13.8761928695311,13.9659992217611,
14.963570594744,15.9611419677269,16.9587133407099,17.9562847136928,18.9538560866757,
19.9514274596586,20.1593781767107),.UNSPECIFIED.);
#3696=B_SPLINE_CURVE_WITH_KNOTS('',3,(#33867,#33868,#33869,#33870,#33871,
#33872,#33873,#33874,#33875,#33876,#33877,#33878,#33879,#33880,#33881,#33882,
#33883,#33884,#33885,#33886,#33887,#33888),.UNSPECIFIED.,.F.,.F.,(4,3,3,
3,3,3,3,4),(-16.4127538780514,-15.9611419677269,-14.963570594744,-13.9659992217611,
-12.9684278487781,-11.9708564757952,-10.9732851028123,-10.1295685708718),
 .UNSPECIFIED.);
#3697=B_SPLINE_CURVE_WITH_KNOTS('',3,(#33894,#33895,#33896,#33897,#33898,
#33899,#33900,#33901,#33902,#33903,#33904,#33905,#33906),.UNSPECIFIED.,
 .F.,.F.,(4,3,3,3,4),(-3.84638326369224,-2.9927141189488,-1.99514274596586,
-0.997571372982931,0.),.UNSPECIFIED.);
#3698=B_SPLINE_CURVE_WITH_KNOTS('',3,(#33909,#33910,#33911,#33912,#33913,
#33914,#33915,#33916,#33917,#33918,#33919,#33920,#33921,#33922,#33923,#33924,
#33925,#33926,#33927),.UNSPECIFIED.,.F.,.F.,(4,3,3,3,3,3,4),(2.01461286527446,
2.99271411894879,3.99028549193172,4.98785686491466,5.98542823789759,6.98299961088052,
7.59300756235153),.UNSPECIFIED.);
#3699=B_SPLINE_CURVE_WITH_KNOTS('',3,(#33933,#33934,#33935,#33936,#33937,
#33938,#33939),.UNSPECIFIED.,.F.,.F.,(4,1,1,1,4),(91.106186954104,91.6672898428913,
92.6648612158742,93.6624325888571,94.6600039618401),.UNSPECIFIED.);
#3700=B_SPLINE_CURVE_WITH_KNOTS('',3,(#33942,#33943,#33944,#33945,#33946,
#33947,#33948,#33949),.UNSPECIFIED.,.F.,.F.,(4,1,1,1,1,4),(91.106186954104,
91.2111367324627,92.2087081054457,93.2062794784286,94.2038508514115,95.1819521050859),
 .UNSPECIFIED.);
#3701=B_SPLINE_CURVE_WITH_KNOTS('',3,(#33954,#33955,#33956,#33957,#33958,
#33959,#33960,#33961,#33962,#33963),.UNSPECIFIED.,.F.,.F.,(4,1,1,1,1,1,
1,4),(84.8230016469244,85.6818616049937,86.6794329779766,87.6770043509595,
88.6745757239425,89.6721470969254,90.6697184699083,91.106186954104),
 .UNSPECIFIED.);
#3702=B_SPLINE_CURVE_WITH_KNOTS('',3,(#33964,#33965,#33966,#33967,#33968,
#33969,#33970,#33971,#33972,#33973),.UNSPECIFIED.,.F.,.F.,(4,1,1,1,1,1,
1,4),(84.8230016469244,85.2257084945651,86.2232798675481,87.220851240531,
88.2184226135139,89.2159939864968,90.2135653594798,91.106186954104),
 .UNSPECIFIED.);
#3703=B_SPLINE_CURVE_WITH_KNOTS('',3,(#33978,#33979,#33980,#33981,#33982,
#33983,#33984,#33985,#33986,#33987,#33988),.UNSPECIFIED.,.F.,.F.,(4,1,1,
1,1,1,1,1,4),(78.5398163397448,78.6988619941132,79.6964333670961,80.694004740079,
81.691576113062,82.6891474860449,83.6867188590278,84.6842902320108,84.8230016469244),
 .UNSPECIFIED.);
#3704=B_SPLINE_CURVE_WITH_KNOTS('',3,(#33989,#33990,#33991,#33992,#33993,
#33994,#33995,#33996,#33997,#33998),.UNSPECIFIED.,.F.,.F.,(4,1,1,1,1,1,
1,4),(78.5398163397448,79.2402802566675,80.2378516296505,81.2354230026334,
82.2329943756163,83.2305657485992,84.2281371215822,84.8230016469244),
 .UNSPECIFIED.);
#3705=B_SPLINE_CURVE_WITH_KNOTS('',3,(#34003,#34004,#34005,#34006,#34007,
#34008,#34009,#34010,#34011,#34012),.UNSPECIFIED.,.F.,.F.,(4,1,1,1,1,1,
1,4),(72.2566310325652,72.7134337562156,73.7110051291985,74.7085765021814,
75.7061478751643,76.7037192481473,77.7012906211302,78.5398163397448),
 .UNSPECIFIED.);
#3706=B_SPLINE_CURVE_WITH_KNOTS('',3,(#34013,#34014,#34015,#34016,#34017,
#34018,#34019,#34020,#34021,#34022,#34023),.UNSPECIFIED.,.F.,.F.,(4,1,1,
1,1,1,1,1,4),(72.2566310325652,72.257280645787,73.2548520187699,74.2524233917529,
75.2499947647358,76.2475661377187,77.2451375107017,78.2427088836846,78.5398163397448),
 .UNSPECIFIED.);
#3707=B_SPLINE_CURVE_WITH_KNOTS('',3,(#34028,#34029,#34030,#34031,#34032,
#34033,#34034,#34035,#34036,#34037),.UNSPECIFIED.,.F.,.F.,(4,1,1,1,1,1,
1,4),(65.9734457253856,66.728005518318,67.7255768913009,68.7231482642838,
69.7207196372668,70.7182910102497,71.7158623832326,72.2566310325652),
 .UNSPECIFIED.);
#3708=B_SPLINE_CURVE_WITH_KNOTS('',3,(#34038,#34039,#34040,#34041,#34042,
#34043,#34044,#34045,#34046,#34047),.UNSPECIFIED.,.F.,.F.,(4,1,1,1,1,1,
1,4),(65.9734457253856,66.2718524078894,67.2694237808723,68.2669951538553,
69.2645665268382,70.2621378998211,71.2597092728041,72.2566310325652),
 .UNSPECIFIED.);
#3709=B_SPLINE_CURVE_WITH_KNOTS('',3,(#34052,#34053,#34054,#34055,#34056,
#34057,#34058,#34059,#34060,#34061,#34062),.UNSPECIFIED.,.F.,.F.,(4,1,1,
1,1,1,1,1,4),(59.690260418206,59.7450059074374,60.7425772804204,61.7401486534033,
62.7377200263862,63.7352913993692,64.7328627723521,65.730434145335,65.9734457253856),
 .UNSPECIFIED.);
#3710=B_SPLINE_CURVE_WITH_KNOTS('',3,(#34063,#34064,#34065,#34066,#34067,
#34068,#34069,#34070,#34071,#34072),.UNSPECIFIED.,.F.,.F.,(4,1,1,1,1,1,
1,4),(59.690260418206,60.2864241699918,61.2839955429747,62.2815669159577,
63.2791382889406,64.2767096619235,65.2742810349065,65.9734457253856),
 .UNSPECIFIED.);
#3711=B_SPLINE_CURVE_WITH_KNOTS('',3,(#34077,#34078,#34079,#34080,#34081,
#34082,#34083,#34084,#34085,#34086),.UNSPECIFIED.,.F.,.F.,(4,1,1,1,1,1,
1,4),(53.4070751110265,53.7595776695398,54.7571490425228,55.7547204155057,
56.7522917884886,57.7498631614716,58.7474345344545,59.690260418206),
 .UNSPECIFIED.);
#3712=B_SPLINE_CURVE_WITH_KNOTS('',3,(#34087,#34088,#34089,#34090,#34091,
#34092,#34093,#34094,#34095,#34096),.UNSPECIFIED.,.F.,.F.,(4,1,1,1,1,1,
1,4),(53.4070751110264,54.3009959320942,55.2985673050771,56.2961386780601,
57.293710051043,58.2912814240259,59.2888527970089,59.690260418206),
 .UNSPECIFIED.);
#3713=B_SPLINE_CURVE_WITH_KNOTS('',3,(#34101,#34102,#34103,#34104,#34105,
#34106,#34107,#34108,#34109,#34110),.UNSPECIFIED.,.F.,.F.,(4,1,1,1,1,1,
1,4),(47.1238898038469,47.7741494316422,48.7717208046252,49.7692921776081,
50.766863550591,51.764434923574,52.7620062965569,53.4070751110265),
 .UNSPECIFIED.);
#3714=B_SPLINE_CURVE_WITH_KNOTS('',3,(#34111,#34112,#34113,#34114,#34115,
#34116,#34117,#34118,#34119,#34120,#34121),.UNSPECIFIED.,.F.,.F.,(4,1,1,
1,1,1,1,1,4),(47.1238898038468,47.3179963212137,48.3155676941966,49.3131390671795,
50.3107104401625,51.3082818131454,52.3058531861283,53.3034245591113,53.4070751110264),
 .UNSPECIFIED.);
#3715=B_SPLINE_CURVE_WITH_KNOTS('',3,(#34126,#34127,#34128,#34129,#34130,
#34131,#34132,#34133,#34134,#34135),.UNSPECIFIED.,.F.,.F.,(4,1,1,1,1,1,
1,4),(40.8407044966673,41.7887211937446,42.7862925667276,43.7838639397105,
44.7814353126934,45.7790066856764,46.7765780586593,47.1238898038469),
 .UNSPECIFIED.);
#3716=B_SPLINE_CURVE_WITH_KNOTS('',3,(#34136,#34137,#34138,#34139,#34140,
#34141,#34142,#34143,#34144,#34145),.UNSPECIFIED.,.F.,.F.,(4,1,1,1,1,1,
1,4),(40.8407044966673,41.3325680833161,42.330139456299,43.327710829282,
44.3252822022649,45.3228535752478,46.3204249482308,47.1238898038468),
 .UNSPECIFIED.);
#3717=B_SPLINE_CURVE_WITH_KNOTS('',3,(#34150,#34151,#34152,#34153,#34154,
#34155,#34156,#34157,#34158,#34159,#34160),.UNSPECIFIED.,.F.,.F.,(4,1,1,
1,1,1,1,1,4),(34.5575191894877,34.8057215828641,35.803292955847,36.80086432883,
37.7984357018129,38.7960070747958,39.7935784477788,40.7911498207617,40.8407044966673),
 .UNSPECIFIED.);
#3718=B_SPLINE_CURVE_WITH_KNOTS('',3,(#34161,#34162,#34163,#34164,#34165,
#34166,#34167,#34168,#34169,#34170),.UNSPECIFIED.,.F.,.F.,(4,1,1,1,1,1,
1,4),(34.5575191894876,35.3471398454185,36.3447112184014,37.3422825913844,
38.3398539643673,39.3374253373502,40.3349967103332,40.8407044966673),
 .UNSPECIFIED.);
#3719=B_SPLINE_CURVE_WITH_KNOTS('',3,(#34175,#34176,#34177,#34178,#34179,
#34180,#34181,#34182,#34183,#34184),.UNSPECIFIED.,.F.,.F.,(4,1,1,1,1,1,
1,4),(28.2743338823081,28.8202933449665,29.8178647179495,30.8154360909324,
31.8130074639153,32.8105788368983,33.8081502098812,34.5575191894877),
 .UNSPECIFIED.);
#3720=B_SPLINE_CURVE_WITH_KNOTS('',3,(#34185,#34186,#34187,#34188,#34189,
#34190,#34191,#34192,#34193,#34194,#34195),.UNSPECIFIED.,.F.,.F.,(4,1,1,
1,1,1,1,1,4),(28.2743338823081,28.364140234538,29.3617116075209,30.3592829805038,
31.3568543534868,32.3544257264697,33.3519970994526,34.3495684724356,34.5575191894876),
 .UNSPECIFIED.);
#3721=B_SPLINE_CURVE_WITH_KNOTS('',3,(#34200,#34201,#34202,#34203,#34204,
#34205,#34206,#34207,#34208,#34209),.UNSPECIFIED.,.F.,.F.,(4,1,1,1,1,1,
1,4),(21.9911485751285,22.8348651070689,23.8324364800519,24.8300078530348,
25.8275792260177,26.8251505990007,27.8227219719836,28.2743338823081),
 .UNSPECIFIED.);
#3722=B_SPLINE_CURVE_WITH_KNOTS('',3,(#34210,#34211,#34212,#34213,#34214,
#34215,#34216,#34217,#34218,#34219),.UNSPECIFIED.,.F.,.F.,(4,1,1,1,1,1,
1,4),(21.9911485751285,22.3787119966404,23.3762833696233,24.3738547426062,
25.3714261155892,26.3689974885721,27.366568861555,28.2743338823081),
 .UNSPECIFIED.);
#3723=B_SPLINE_CURVE_WITH_KNOTS('',3,(#34225,#34226,#34227,#34228,#34229),
 .UNSPECIFIED.,.F.,.F.,(4,1,4),(14.3981410127769,15.3957123857598,15.7079632679489),
 .UNSPECIFIED.);
#3724=B_SPLINE_CURVE_WITH_KNOTS('',3,(#34232,#34233,#34234,#34235,#34236),
 .UNSPECIFIED.,.F.,.F.,(4,1,4),(13.8761928695311,14.8542941232055,15.7079632679489),
 .UNSPECIFIED.);
#3725=B_SPLINE_CURVE_WITH_KNOTS('',3,(#34242,#34243,#34244,#34245),
 .UNSPECIFIED.,.F.,.F.,(4,4),(51.5750455984138,52.2824273504651),
 .UNSPECIFIED.);
#3726=B_SPLINE_CURVE_WITH_KNOTS('',3,(#34248,#34249,#34250,#34251,#34252,
#34253,#34254,#34255,#34256,#34257),.UNSPECIFIED.,.F.,.F.,(4,3,3,4),(-50.2654824574366,
-49.3356538821136,-48.3533960593298,-47.8312715558982),.UNSPECIFIED.);
#3727=B_SPLINE_CURVE_WITH_KNOTS('',3,(#34262,#34263,#34264,#34265,#34266,
#34267,#34268,#34269,#34270,#34271,#34272,#34273,#34274,#34275,#34276,#34277,
#34278,#34279,#34280,#34281,#34282,#34283,#34284,#34285,#34286),
 .UNSPECIFIED.,.F.,.F.,(4,3,3,3,3,3,3,3,4),(45.2918602912342,45.3820193336359,
46.3677919074686,47.3535644813014,48.3393370551341,49.3251096289668,50.3108822027996,
51.2966547766323,51.5750455984138),.UNSPECIFIED.);
#3728=B_SPLINE_CURVE_WITH_KNOTS('',3,(#34287,#34288,#34289,#34290,#34291,
#34292,#34293,#34294,#34295,#34296,#34297,#34298,#34299,#34300,#34301,#34302,
#34303,#34304,#34305,#34306,#34307,#34308),.UNSPECIFIED.,.F.,.F.,(4,3,3,
3,3,3,3,4),(-47.8312715558982,-47.371138236546,-46.3888804137622,-45.4066225909784,
-44.4243647681946,-43.4421069454108,-42.459849122627,-41.5480862487186),
 .UNSPECIFIED.);
#3729=B_SPLINE_CURVE_WITH_KNOTS('',3,(#34313,#34314,#34315,#34316,#34317,
#34318,#34319,#34320,#34321,#34322,#34323,#34324,#34325,#34326,#34327,#34328,
#34329,#34330,#34331,#34332,#34333,#34334),.UNSPECIFIED.,.F.,.F.,(4,3,3,
3,3,3,3,4),(39.0086749840547,39.4673838906394,40.4531564644721,41.4389290383049,
42.4247016121376,43.4104741859704,44.3962467598031,45.2918602912342),
 .UNSPECIFIED.);
#3730=B_SPLINE_CURVE_WITH_KNOTS('',3,(#34335,#34336,#34337,#34338,#34339,
#34340,#34341,#34342,#34343,#34344,#34345,#34346,#34347,#34348,#34349,#34350,
#34351,#34352,#34353,#34354,#34355,#34356,#34357,#34358,#34359),
 .UNSPECIFIED.,.F.,.F.,(4,3,3,3,3,3,3,3,4),(-41.5480862487186,-41.4775912998432,
-40.4953334770593,-39.5130756542755,-38.5308178314917,-37.5485600087079,
-36.5663021859241,-35.5840443631403,-35.264900941539),.UNSPECIFIED.);
#3731=B_SPLINE_CURVE_WITH_KNOTS('',3,(#34364,#34365,#34366,#34367,#34368,
#34369,#34370,#34371,#34372,#34373,#34374,#34375,#34376,#34377,#34378,#34379,
#34380,#34381,#34382,#34383,#34384,#34385),.UNSPECIFIED.,.F.,.F.,(4,3,3,
3,3,3,3,4),(32.7254896768751,33.5527484476429,34.5385210214757,35.5242935953084,
36.5100661691412,37.4958387429739,38.4816113168067,39.0086749840547),
 .UNSPECIFIED.);
#3732=B_SPLINE_CURVE_WITH_KNOTS('',3,(#34386,#34387,#34388,#34389,#34390,
#34391,#34392,#34393,#34394,#34395,#34396,#34397,#34398,#34399,#34400,#34401,
#34402,#34403,#34404,#34405,#34406,#34407),.UNSPECIFIED.,.F.,.F.,(4,3,3,
3,3,3,3,4),(-35.264900941539,-34.6017865403565,-33.6195287175727,-32.6372708947889,
-31.6550130720051,-30.6727552492213,-29.6904974264375,-28.9817156343594),
 .UNSPECIFIED.);
#3733=B_SPLINE_CURVE_WITH_KNOTS('',3,(#34412,#34413,#34414,#34415,#34416,
#34417,#34418,#34419,#34420,#34421,#34422,#34423,#34424,#34425,#34426,#34427,
#34428,#34429,#34430,#34431,#34432,#34433,#34434,#34435,#34436),
 .UNSPECIFIED.,.F.,.F.,(4,3,3,3,3,3,3,3,4),(26.4423043696954,26.6523404308137,
27.6381130046465,28.6238855784792,29.609658152312,30.5954307261447,31.5812032999775,
32.5669758738102,32.7254896768751),.UNSPECIFIED.);
#3734=B_SPLINE_CURVE_WITH_KNOTS('',3,(#34437,#34438,#34439,#34440,#34441,
#34442,#34443,#34444,#34445,#34446,#34447,#34448,#34449,#34450,#34451,#34452,
#34453,#34454,#34455,#34456,#34457,#34458,#34459,#34460,#34461),
 .UNSPECIFIED.,.F.,.F.,(4,3,3,3,3,3,3,3,4),(-28.9817156343594,-28.7082396036537,
-27.7259817808699,-26.7437239580861,-25.7614661353022,-24.7792083125184,
-23.7969504897346,-22.8146926669508,-22.6985303271799),.UNSPECIFIED.);
#3735=B_SPLINE_CURVE_WITH_KNOTS('',3,(#34466,#34467,#34468,#34469,#34470,
#34471,#34472,#34473,#34474,#34475,#34476,#34477,#34478,#34479,#34480,#34481,
#34482,#34483,#34484,#34485,#34486,#34487),.UNSPECIFIED.,.F.,.F.,(4,3,3,
3,3,3,3,4),(20.1591190625158,20.7377049878173,21.72347756165,22.7092501354828,
23.6950227093155,24.6807952831482,25.666567856981,26.4423043696954),
 .UNSPECIFIED.);
#3736=B_SPLINE_CURVE_WITH_KNOTS('',3,(#34488,#34489,#34490,#34491,#34492,
#34493,#34494,#34495,#34496,#34497,#34498,#34499,#34500,#34501,#34502,#34503,
#34504,#34505,#34506,#34507,#34508,#34509),.UNSPECIFIED.,.F.,.F.,(4,3,3,
3,3,3,3,4),(-22.6985303271799,-21.832434844167,-20.8501770213832,-19.8679191985994,
-18.8856613758156,-17.9034035530318,-16.921145730248,-16.4153450200003),
 .UNSPECIFIED.);
#3737=B_SPLINE_CURVE_WITH_KNOTS('',3,(#34514,#34515,#34516,#34517,#34518,
#34519,#34520,#34521,#34522,#34523,#34524,#34525,#34526,#34527,#34528,#34529,
#34530,#34531,#34532,#34533,#34534,#34535),.UNSPECIFIED.,.F.,.F.,(4,3,3,
3,3,3,3,4),(13.8759337553363,14.8230695448208,15.8088421186535,16.7946146924863,
17.780387266319,18.7661598401518,19.7519324139845,20.1591190625158),
 .UNSPECIFIED.);
#3738=B_SPLINE_CURVE_WITH_KNOTS('',3,(#34536,#34537,#34538,#34539,#34540,
#34541,#34542,#34543,#34544,#34545,#34546,#34547,#34548,#34549,#34550,#34551,
#34552,#34553,#34554,#34555,#34556,#34557),.UNSPECIFIED.,.F.,.F.,(4,3,3,
3,3,3,3,4),(-16.4153450200003,-15.9388879074642,-14.9566300846804,-13.9743722618966,
-12.9921144391128,-12.009856616329,-11.0275987935451,-10.1321597128207),
 .UNSPECIFIED.);
#3739=B_SPLINE_CURVE_WITH_KNOTS('',3,(#34563,#34564,#34565,#34566,#34567,
#34568,#34569,#34570,#34571,#34572,#34573,#34574,#34575),.UNSPECIFIED.,
 .F.,.F.,(4,3,3,3,4),(-3.84897440564113,-3.1695362112747,-2.18727838849089,
-1.20502056570709,-0.222762742923284),.UNSPECIFIED.);
#3740=B_SPLINE_CURVE_WITH_KNOTS('',3,(#34577,#34578,#34579,#34580,#34581,
#34582,#34583,#34584,#34585,#34586,#34587,#34588),.UNSPECIFIED.,.F.,.F.,
(4,2,2,2,2,4),(0.202168863441191,0.284518942728512,0.37935858673359,0.474198230738669,
0.569037874743748,0.642071595472288),.UNSPECIFIED.);
#3741=B_SPLINE_CURVE_WITH_KNOTS('',3,(#34589,#34590,#34591,#34592,#34593,
#34594,#34595,#34596,#34597,#34598,#34599,#34600,#34601,#34602,#34603,#34604,
#34605,#34606,#34607),.UNSPECIFIED.,.F.,.F.,(4,3,3,3,3,3,4),(2.14497997264822,
2.99379865882787,3.97957123266061,4.96534380649336,5.9511163803261,6.93688895415885,
7.5927484481567),.UNSPECIFIED.);
#3742=B_SPLINE_CURVE_WITH_KNOTS('',3,(#34613,#34614,#34615,#34616,#34617,
#34618,#34619,#34620),.UNSPECIFIED.,.F.,.F.,(4,1,1,1,1,4),(59.6902604182061,
60.2123849216376,61.1946427444214,62.1769005672052,63.159158389989,64.1414162127728),
 .UNSPECIFIED.);
#3743=B_SPLINE_CURVE_WITH_KNOTS('',3,(#34623,#34624,#34625,#34626,#34627,
#34628,#34629,#34630,#34631),.UNSPECIFIED.,.F.,.F.,(4,1,1,1,1,1,4),(59.6902604182061,
59.7804194606077,60.7661920344404,61.7519646082732,62.7377371821059,63.7235097559386,
64.6638825844084),.UNSPECIFIED.);
#3744=B_SPLINE_CURVE_WITH_KNOTS('',3,(#34636,#34637,#34638,#34639,#34640,
#34641,#34642,#34643,#34644,#34645),.UNSPECIFIED.,.F.,.F.,(4,1,1,1,1,1,
1,4),(53.4070751110265,54.3188379849348,55.3010958077186,56.2833536305024,
57.2656114532862,58.24786927607,59.2301270988538,59.6902604182061),
 .UNSPECIFIED.);
#3745=B_SPLINE_CURVE_WITH_KNOTS('',3,(#34646,#34647,#34648,#34649,#34650,
#34651,#34652,#34653,#34654,#34655),.UNSPECIFIED.,.F.,.F.,(4,1,1,1,1,1,
1,4),(53.4070751110265,53.8657840176112,54.8515565914439,55.8373291652767,
56.8231017391094,57.8088743129422,58.7946468867749,59.6902604182061),
 .UNSPECIFIED.);
#3746=B_SPLINE_CURVE_WITH_KNOTS('',3,(#34660,#34661,#34662,#34663,#34664,
#34665,#34666,#34667,#34668,#34669,#34670),.UNSPECIFIED.,.F.,.F.,(4,1,1,
1,1,1,1,1,4),(47.1238898038469,47.4430332254481,48.4252910482319,49.4075488710157,
50.3898066937995,51.3720645165834,52.3543223393672,53.336580162151,53.4070751110265),
 .UNSPECIFIED.);
#3747=B_SPLINE_CURVE_WITH_KNOTS('',3,(#34671,#34672,#34673,#34674,#34675,
#34676,#34677,#34678,#34679,#34680),.UNSPECIFIED.,.F.,.F.,(4,1,1,1,1,1,
1,4),(47.1238898038469,47.9511485746147,48.9369211484475,49.9226937222802,
50.908466296113,51.8942388699457,52.8800114437785,53.4070751110265),
 .UNSPECIFIED.);
#3748=B_SPLINE_CURVE_WITH_KNOTS('',3,(#34685,#34686,#34687,#34688,#34689,
#34690,#34691,#34692,#34693,#34694),.UNSPECIFIED.,.F.,.F.,(4,1,1,1,1,1,
1,4),(40.8407044966673,41.5494862887453,42.5317441115291,43.5140019343129,
44.4962597570967,45.4785175798805,46.4607754026643,47.1238898038469),
 .UNSPECIFIED.);
#3749=B_SPLINE_CURVE_WITH_KNOTS('',3,(#34695,#34696,#34697,#34698,#34699,
#34700,#34701,#34702,#34703,#34704,#34705),.UNSPECIFIED.,.F.,.F.,(4,1,1,
1,1,1,1,1,4),(40.8407044966673,41.0507405577855,42.0365131316183,43.022285705451,
44.0080582792838,44.9938308531165,45.9796034269492,46.965376000782,47.1238898038469),
 .UNSPECIFIED.);
#3750=B_SPLINE_CURVE_WITH_KNOTS('',3,(#34710,#34711,#34712,#34713,#34714,
#34715,#34716,#34717,#34718,#34719,#34720),.UNSPECIFIED.,.F.,.F.,(4,1,1,
1,1,1,1,1,4),(34.5575191894877,34.6736815292587,35.6559393520425,36.6381971748263,
37.6204549976101,38.6027128203939,39.5849706431777,40.5672284659615,40.8407044966673),
 .UNSPECIFIED.);
#3751=B_SPLINE_CURVE_WITH_KNOTS('',3,(#34721,#34722,#34723,#34724,#34725,
#34726,#34727,#34728,#34729,#34730),.UNSPECIFIED.,.F.,.F.,(4,1,1,1,1,1,
1,4),(34.5575191894877,35.1361051147891,36.1218776886218,37.1076502624545,
38.0934228362873,39.07919541012,40.0649679839528,40.8407044966673),
 .UNSPECIFIED.);
#3752=B_SPLINE_CURVE_WITH_KNOTS('',3,(#34735,#34736,#34737,#34738,#34739,
#34740,#34741,#34742,#34743,#34744),.UNSPECIFIED.,.F.,.F.,(4,1,1,1,1,1,
1,4),(28.2743338823081,28.7801345925558,29.7623924153396,30.7446502381234,
31.7269080609072,32.709165883691,33.6914237064748,34.5575191894877),
 .UNSPECIFIED.);
#3753=B_SPLINE_CURVE_WITH_KNOTS('',3,(#34745,#34746,#34747,#34748,#34749,
#34750,#34751,#34752,#34753,#34754),.UNSPECIFIED.,.F.,.F.,(4,1,1,1,1,1,
1,4),(28.2743338823081,29.2214696717926,30.2072422456253,31.1930148194581,
32.1787873932908,33.1645599671236,34.1503325409563,34.5575191894877),
 .UNSPECIFIED.);
#3754=B_SPLINE_CURVE_WITH_KNOTS('',3,(#34759,#34760,#34761,#34762,#34763,
#34764,#34765,#34766,#34767,#34768),.UNSPECIFIED.,.F.,.F.,(4,1,1,1,1,1,
1,4),(21.9911485751285,22.886587655853,23.8688454786368,24.8511033014206,
25.8333611242044,26.8156189469882,27.797876769772,28.2743338823081),
 .UNSPECIFIED.);
#3755=B_SPLINE_CURVE_WITH_KNOTS('',3,(#34769,#34770,#34771,#34772,#34773,
#34774,#34775,#34776,#34777,#34778,#34779),.UNSPECIFIED.,.F.,.F.,(4,1,1,
1,1,1,1,1,4),(21.9911485751285,22.3210616549634,23.3068342287961,24.2926068026289,
25.2783793764616,26.2641519502944,27.2499245241271,28.2356970979599,28.2743338823081),
 .UNSPECIFIED.);
#3756=B_SPLINE_CURVE_WITH_KNOTS('',3,(#34785,#34786,#34787,#34788,#34789),
 .UNSPECIFIED.,.F.,.F.,(4,1,4),(14.4348810643014,15.4206536381342,15.7079632679489),
 .UNSPECIFIED.);
#3757=B_SPLINE_CURVE_WITH_KNOTS('',3,(#34791,#34792,#34793,#34794),
 .UNSPECIFIED.,.F.,.F.,(4,4),(1.38948745034524,1.47775448763834),
 .UNSPECIFIED.);
#3758=B_SPLINE_CURVE_WITH_KNOTS('',3,(#34796,#34797,#34798,#34799),
 .UNSPECIFIED.,.F.,.F.,(4,4),(1.3186667718152,1.38948745034524),
 .UNSPECIFIED.);
#3759=B_SPLINE_CURVE_WITH_KNOTS('',3,(#34800,#34801,#34802,#34803,#34804,
#34805),.UNSPECIFIED.,.F.,.F.,(4,1,1,4),(13.8994448374521,14.0462672507987,
15.0285250735825,15.7079632679489),.UNSPECIFIED.);
#3760=B_SPLINE_CURVE_WITH_KNOTS('',3,(#34811,#34812,#34813,#34814),
 .UNSPECIFIED.,.F.,.F.,(4,4),(51.5750455984139,52.282427350465),
 .UNSPECIFIED.);
#3761=B_SPLINE_CURVE_WITH_KNOTS('',3,(#34817,#34818,#34819,#34820,#34821,
#34822,#34823,#34824,#34825,#34826),.UNSPECIFIED.,.F.,.F.,(4,3,3,4),(-50.2654824574365,
-49.3356538821136,-48.3533960593298,-47.8312715558982),.UNSPECIFIED.);
#3762=B_SPLINE_CURVE_WITH_KNOTS('',3,(#34831,#34832,#34833,#34834,#34835,
#34836,#34837,#34838,#34839,#34840,#34841,#34842,#34843,#34844,#34845,#34846,
#34847,#34848,#34849,#34850,#34851,#34852,#34853,#34854,#34855),
 .UNSPECIFIED.,.F.,.F.,(4,3,3,3,3,3,3,3,4),(45.2918602912343,45.3820193336358,
46.3677919074686,47.3535644813013,48.3393370551341,49.3251096289668,50.3108822027995,
51.2966547766323,51.5750455984139),.UNSPECIFIED.);
#3763=B_SPLINE_CURVE_WITH_KNOTS('',3,(#34856,#34857,#34858,#34859,#34860,
#34861,#34862,#34863,#34864,#34865,#34866,#34867,#34868,#34869,#34870,#34871,
#34872,#34873,#34874,#34875,#34876,#34877),.UNSPECIFIED.,.F.,.F.,(4,3,3,
3,3,3,3,4),(-47.8312715558982,-47.371138236546,-46.3888804137622,-45.4066225909784,
-44.4243647681946,-43.4421069454107,-42.459849122627,-41.5480862487186),
 .UNSPECIFIED.);
#3764=B_SPLINE_CURVE_WITH_KNOTS('',3,(#34882,#34883,#34884,#34885,#34886,
#34887,#34888,#34889,#34890,#34891,#34892,#34893,#34894,#34895,#34896,#34897,
#34898,#34899,#34900,#34901,#34902,#34903),.UNSPECIFIED.,.F.,.F.,(4,3,3,
3,3,3,3,4),(39.0086749840547,39.4673838906393,40.4531564644721,41.4389290383048,
42.4247016121376,43.4104741859703,44.3962467598031,45.2918602912343),
 .UNSPECIFIED.);
#3765=B_SPLINE_CURVE_WITH_KNOTS('',3,(#34904,#34905,#34906,#34907,#34908,
#34909,#34910,#34911,#34912,#34913,#34914,#34915,#34916,#34917,#34918,#34919,
#34920,#34921,#34922,#34923,#34924,#34925,#34926,#34927,#34928),
 .UNSPECIFIED.,.F.,.F.,(4,3,3,3,3,3,3,3,4),(-41.5480862487186,-41.4775912998431,
-40.4953334770593,-39.5130756542755,-38.5308178314917,-37.5485600087079,
-36.5663021859241,-35.5840443631403,-35.264900941539),.UNSPECIFIED.);
#3766=B_SPLINE_CURVE_WITH_KNOTS('',3,(#34933,#34934,#34935,#34936,#34937,
#34938,#34939,#34940,#34941,#34942,#34943,#34944,#34945,#34946,#34947,#34948,
#34949,#34950,#34951,#34952,#34953,#34954),.UNSPECIFIED.,.F.,.F.,(4,3,3,
3,3,3,3,4),(32.7254896768751,33.5527484476429,34.5385210214756,35.5242935953084,
36.5100661691411,37.4958387429738,38.4816113168066,39.0086749840547),
 .UNSPECIFIED.);
#3767=B_SPLINE_CURVE_WITH_KNOTS('',3,(#34955,#34956,#34957,#34958,#34959,
#34960,#34961,#34962,#34963,#34964,#34965,#34966,#34967,#34968,#34969,#34970,
#34971,#34972,#34973,#34974,#34975,#34976),.UNSPECIFIED.,.F.,.F.,(4,3,3,
3,3,3,3,4),(-35.264900941539,-34.6017865403565,-33.6195287175727,-32.6372708947889,
-31.6550130720051,-30.6727552492213,-29.6904974264375,-28.9817156343594),
 .UNSPECIFIED.);
#3768=B_SPLINE_CURVE_WITH_KNOTS('',3,(#34981,#34982,#34983,#34984,#34985,
#34986,#34987,#34988,#34989,#34990,#34991,#34992,#34993,#34994,#34995,#34996,
#34997,#34998,#34999,#35000,#35001,#35002,#35003,#35004,#35005),
 .UNSPECIFIED.,.F.,.F.,(4,3,3,3,3,3,3,3,4),(26.4423043696955,26.6523404308136,
27.6381130046464,28.6238855784791,29.6096581523119,30.5954307261446,31.5812032999774,
32.5669758738101,32.7254896768751),.UNSPECIFIED.);
#3769=B_SPLINE_CURVE_WITH_KNOTS('',3,(#35006,#35007,#35008,#35009,#35010,
#35011,#35012,#35013,#35014,#35015,#35016,#35017,#35018,#35019,#35020,#35021,
#35022,#35023,#35024,#35025,#35026,#35027,#35028,#35029,#35030),
 .UNSPECIFIED.,.F.,.F.,(4,3,3,3,3,3,3,3,4),(-28.9817156343594,-28.7082396036537,
-27.7259817808699,-26.7437239580861,-25.7614661353022,-24.7792083125184,
-23.7969504897346,-22.8146926669508,-22.6985303271799),.UNSPECIFIED.);
#3770=B_SPLINE_CURVE_WITH_KNOTS('',3,(#35035,#35036,#35037,#35038,#35039,
#35040,#35041,#35042,#35043,#35044,#35045,#35046,#35047,#35048,#35049,#35050,
#35051,#35052,#35053,#35054,#35055,#35056),.UNSPECIFIED.,.F.,.F.,(4,3,3,
3,3,3,3,4),(20.1591190625159,20.7377049878172,21.7234775616499,22.7092501354827,
23.6950227093154,24.6807952831481,25.6665678569809,26.4423043696955),
 .UNSPECIFIED.);
#3771=B_SPLINE_CURVE_WITH_KNOTS('',3,(#35057,#35058,#35059,#35060,#35061,
#35062,#35063,#35064,#35065,#35066,#35067,#35068,#35069,#35070,#35071,#35072,
#35073,#35074,#35075,#35076,#35077,#35078),.UNSPECIFIED.,.F.,.F.,(4,3,3,
3,3,3,3,4),(-22.6985303271799,-21.832434844167,-20.8501770213832,-19.8679191985994,
-18.8856613758156,-17.9034035530318,-16.921145730248,-16.4153450200003),
 .UNSPECIFIED.);
#3772=B_SPLINE_CURVE_WITH_KNOTS('',3,(#35083,#35084,#35085,#35086,#35087,
#35088,#35089,#35090,#35091,#35092,#35093,#35094,#35095,#35096,#35097,#35098,
#35099,#35100,#35101,#35102,#35103,#35104),.UNSPECIFIED.,.F.,.F.,(4,3,3,
3,3,3,3,4),(13.8759337553364,14.8230695448207,15.8088421186534,16.7946146924862,
17.7803872663189,18.7661598401517,19.7519324139844,20.1591190625159),
 .UNSPECIFIED.);
#3773=B_SPLINE_CURVE_WITH_KNOTS('',3,(#35105,#35106,#35107,#35108,#35109,
#35110,#35111,#35112,#35113,#35114,#35115,#35116,#35117,#35118,#35119,#35120,
#35121,#35122,#35123,#35124,#35125,#35126),.UNSPECIFIED.,.F.,.F.,(4,3,3,
3,3,3,3,4),(-16.4153450200003,-15.9388879074642,-14.9566300846804,-13.9743722618966,
-12.9921144391128,-12.009856616329,-11.0275987935452,-10.1321597128207),
 .UNSPECIFIED.);
#3774=B_SPLINE_CURVE_WITH_KNOTS('',3,(#35132,#35133,#35134,#35135,#35136,
#35137,#35138,#35139,#35140,#35141,#35142,#35143,#35144),.UNSPECIFIED.,
 .F.,.F.,(4,3,3,3,4),(-3.84897440564107,-3.16953621127471,-2.1872783884909,
-1.20502056570709,-0.222762742923288),.UNSPECIFIED.);
#3775=B_SPLINE_CURVE_WITH_KNOTS('',3,(#35146,#35147,#35148,#35149,#35150,
#35151,#35152,#35153,#35154,#35155,#35156,#35157),.UNSPECIFIED.,.F.,.F.,
(4,2,2,2,2,4),(0.202168863441159,0.284518942728512,0.379358586733591,0.474198230738669,
0.569037874743748,0.642071595472281),.UNSPECIFIED.);
#3776=B_SPLINE_CURVE_WITH_KNOTS('',3,(#35158,#35159,#35160,#35161,#35162,
#35163,#35164,#35165,#35166,#35167,#35168,#35169,#35170,#35171,#35172,#35173,
#35174,#35175,#35176),.UNSPECIFIED.,.F.,.F.,(4,3,3,3,3,3,4),(2.14497997264816,
2.99379865882773,3.97957123266047,4.96534380649322,5.95111638032597,6.93688895415871,
7.59274844815675),.UNSPECIFIED.);
#3777=B_SPLINE_CURVE_WITH_KNOTS('',3,(#35182,#35183,#35184,#35185),
 .UNSPECIFIED.,.F.,.F.,(4,4),(51.5750455984139,52.2824273504652),
 .UNSPECIFIED.);
#3778=B_SPLINE_CURVE_WITH_KNOTS('',3,(#35188,#35189,#35190,#35191,#35192,
#35193,#35194,#35195,#35196,#35197),.UNSPECIFIED.,.F.,.F.,(4,3,3,4),(-50.2654824574367,
-49.3356538821138,-48.35339605933,-47.8312715558982),.UNSPECIFIED.);
#3779=B_SPLINE_CURVE_WITH_KNOTS('',3,(#35202,#35203,#35204,#35205,#35206,
#35207,#35208,#35209,#35210,#35211,#35212,#35213,#35214,#35215,#35216,#35217,
#35218,#35219,#35220,#35221,#35222,#35223,#35224,#35225,#35226),
 .UNSPECIFIED.,.F.,.F.,(4,3,3,3,3,3,3,3,4),(45.2918602912343,45.382019333636,
46.3677919074688,47.3535644813015,48.3393370551343,49.325109628967,50.3108822027997,
51.2966547766325,51.5750455984139),.UNSPECIFIED.);
#3780=B_SPLINE_CURVE_WITH_KNOTS('',3,(#35227,#35228,#35229,#35230,#35231,
#35232,#35233,#35234,#35235,#35236,#35237,#35238,#35239,#35240,#35241,#35242,
#35243,#35244,#35245,#35246,#35247,#35248),.UNSPECIFIED.,.F.,.F.,(4,3,3,
3,3,3,3,4),(-47.8312715558982,-47.3711382365462,-46.3888804137624,-45.4066225909786,
-44.4243647681948,-43.442106945411,-42.4598491226272,-41.5480862487186),
 .UNSPECIFIED.);
#3781=B_SPLINE_CURVE_WITH_KNOTS('',3,(#35253,#35254,#35255,#35256,#35257,
#35258,#35259,#35260,#35261,#35262,#35263,#35264,#35265,#35266,#35267,#35268,
#35269,#35270,#35271,#35272,#35273,#35274),.UNSPECIFIED.,.F.,.F.,(4,3,3,
3,3,3,3,4),(39.0086749840547,39.4673838906396,40.4531564644723,41.438929038305,
42.4247016121378,43.4104741859705,44.3962467598033,45.2918602912343),
 .UNSPECIFIED.);
#3782=B_SPLINE_CURVE_WITH_KNOTS('',3,(#35275,#35276,#35277,#35278,#35279,
#35280,#35281,#35282,#35283,#35284,#35285,#35286,#35287,#35288,#35289,#35290,
#35291,#35292,#35293,#35294,#35295,#35296,#35297,#35298,#35299),
 .UNSPECIFIED.,.F.,.F.,(4,3,3,3,3,3,3,3,4),(-41.5480862487186,-41.4775912998434,
-40.4953334770596,-39.5130756542758,-38.5308178314919,-37.5485600087081,
-36.5663021859243,-35.5840443631405,-35.264900941539),.UNSPECIFIED.);
#3783=B_SPLINE_CURVE_WITH_KNOTS('',3,(#35304,#35305,#35306,#35307,#35308,
#35309,#35310,#35311,#35312,#35313,#35314,#35315,#35316,#35317,#35318,#35319,
#35320,#35321,#35322,#35323,#35324,#35325),.UNSPECIFIED.,.F.,.F.,(4,3,3,
3,3,3,3,4),(32.7254896768751,33.5527484476431,34.5385210214758,35.5242935953086,
36.5100661691413,37.4958387429741,38.4816113168068,39.0086749840547),
 .UNSPECIFIED.);
#3784=B_SPLINE_CURVE_WITH_KNOTS('',3,(#35326,#35327,#35328,#35329,#35330,
#35331,#35332,#35333,#35334,#35335,#35336,#35337,#35338,#35339,#35340,#35341,
#35342,#35343,#35344,#35345,#35346,#35347),.UNSPECIFIED.,.F.,.F.,(4,3,3,
3,3,3,3,4),(-35.264900941539,-34.6017865403567,-33.6195287175729,-32.6372708947891,
-31.6550130720053,-30.6727552492215,-29.6904974264377,-28.9817156343594),
 .UNSPECIFIED.);
#3785=B_SPLINE_CURVE_WITH_KNOTS('',3,(#35352,#35353,#35354,#35355,#35356,
#35357,#35358,#35359,#35360,#35361,#35362,#35363,#35364,#35365,#35366,#35367,
#35368,#35369,#35370,#35371,#35372,#35373,#35374,#35375,#35376),
 .UNSPECIFIED.,.F.,.F.,(4,3,3,3,3,3,3,3,4),(26.4423043696955,26.6523404308139,
27.6381130046466,28.6238855784794,29.6096581523121,30.5954307261449,31.5812032999776,
32.5669758738103,32.7254896768751),.UNSPECIFIED.);
#3786=B_SPLINE_CURVE_WITH_KNOTS('',3,(#35377,#35378,#35379,#35380,#35381,
#35382,#35383,#35384,#35385,#35386,#35387,#35388,#35389,#35390,#35391,#35392,
#35393,#35394,#35395,#35396,#35397,#35398,#35399,#35400,#35401),
 .UNSPECIFIED.,.F.,.F.,(4,3,3,3,3,3,3,3,4),(-28.9817156343594,-28.7082396036539,
-27.7259817808701,-26.7437239580863,-25.7614661353025,-24.7792083125187,
-23.7969504897349,-22.8146926669511,-22.6985303271798),.UNSPECIFIED.);
#3787=B_SPLINE_CURVE_WITH_KNOTS('',3,(#35406,#35407,#35408,#35409,#35410,
#35411,#35412,#35413,#35414,#35415,#35416,#35417,#35418,#35419,#35420,#35421,
#35422,#35423,#35424,#35425,#35426,#35427),.UNSPECIFIED.,.F.,.F.,(4,3,3,
3,3,3,3,4),(20.1591190625159,20.7377049878174,21.7234775616502,22.7092501354829,
23.6950227093156,24.6807952831484,25.6665678569811,26.4423043696955),
 .UNSPECIFIED.);
#3788=B_SPLINE_CURVE_WITH_KNOTS('',3,(#35428,#35429,#35430,#35431,#35432,
#35433,#35434,#35435,#35436,#35437,#35438,#35439,#35440,#35441,#35442,#35443,
#35444,#35445,#35446,#35447,#35448,#35449),.UNSPECIFIED.,.F.,.F.,(4,3,3,
3,3,3,3,4),(-22.6985303271798,-21.8324348441672,-20.8501770213834,-19.8679191985996,
-18.8856613758158,-17.903403553032,-16.9211457302482,-16.4153450200003),
 .UNSPECIFIED.);
#3789=B_SPLINE_CURVE_WITH_KNOTS('',3,(#35454,#35455,#35456,#35457,#35458,
#35459,#35460,#35461,#35462,#35463,#35464,#35465,#35466,#35467,#35468,#35469,
#35470,#35471,#35472,#35473,#35474,#35475),.UNSPECIFIED.,.F.,.F.,(4,3,3,
3,3,3,3,4),(13.8759337553364,14.8230695448209,15.8088421186537,16.7946146924864,
17.7803872663192,18.7661598401519,19.7519324139847,20.1591190625159),
 .UNSPECIFIED.);
#3790=B_SPLINE_CURVE_WITH_KNOTS('',3,(#35476,#35477,#35478,#35479,#35480,
#35481,#35482,#35483,#35484,#35485,#35486,#35487,#35488,#35489,#35490,#35491,
#35492,#35493,#35494,#35495,#35496,#35497),.UNSPECIFIED.,.F.,.F.,(4,3,3,
3,3,3,3,4),(-16.4153450200003,-15.9388879074644,-14.9566300846806,-13.9743722618968,
-12.992114439113,-12.0098566163292,-11.0275987935454,-10.1321597128207),
 .UNSPECIFIED.);
#3791=B_SPLINE_CURVE_WITH_KNOTS('',3,(#35503,#35504,#35505,#35506,#35507,
#35508,#35509,#35510,#35511,#35512,#35513,#35514,#35515),.UNSPECIFIED.,
 .F.,.F.,(4,3,3,3,4),(-3.84897440564108,-3.16953621127493,-2.18727838849113,
-1.20502056570732,-0.222762742923517),.UNSPECIFIED.);
#3792=B_SPLINE_CURVE_WITH_KNOTS('',3,(#35517,#35518,#35519,#35520,#35521,
#35522,#35523,#35524,#35525,#35526,#35527,#35528),.UNSPECIFIED.,.F.,.F.,
(4,2,2,2,2,4),(0.202168863441204,0.284518942728512,0.379358586733591,0.474198230738669,
0.569037874743748,0.64207159547233),.UNSPECIFIED.);
#3793=B_SPLINE_CURVE_WITH_KNOTS('',3,(#35529,#35530,#35531,#35532,#35533,
#35534,#35535,#35536,#35537,#35538,#35539,#35540,#35541,#35542,#35543,#35544,
#35545,#35546,#35547),.UNSPECIFIED.,.F.,.F.,(4,3,3,3,3,3,4),(2.14497997264827,
2.99379865882801,3.97957123266076,4.9653438064935,5.95111638032624,6.93688895415899,
7.59274844815675),.UNSPECIFIED.);
#3794=B_SPLINE_CURVE_WITH_KNOTS('',3,(#35553,#35554,#35555,#35556),
 .UNSPECIFIED.,.F.,.F.,(4,4),(51.5750455984139,52.2824273504652),
 .UNSPECIFIED.);
#3795=B_SPLINE_CURVE_WITH_KNOTS('',3,(#35559,#35560,#35561,#35562,#35563,
#35564,#35565,#35566,#35567,#35568),.UNSPECIFIED.,.F.,.F.,(4,3,3,4),(-50.2654824574367,
-49.3356538821137,-48.3533960593299,-47.8312715558983),.UNSPECIFIED.);
#3796=B_SPLINE_CURVE_WITH_KNOTS('',3,(#35573,#35574,#35575,#35576,#35577,
#35578,#35579,#35580,#35581,#35582,#35583,#35584,#35585,#35586,#35587,#35588,
#35589,#35590,#35591,#35592,#35593,#35594,#35595,#35596,#35597),
 .UNSPECIFIED.,.F.,.F.,(4,3,3,3,3,3,3,3,4),(45.2918602912343,45.382019333636,
46.3677919074687,47.3535644813014,48.3393370551342,49.3251096289669,50.3108822027997,
51.2966547766324,51.5750455984139),.UNSPECIFIED.);
#3797=B_SPLINE_CURVE_WITH_KNOTS('',3,(#35598,#35599,#35600,#35601,#35602,
#35603,#35604,#35605,#35606,#35607,#35608,#35609,#35610,#35611,#35612,#35613,
#35614,#35615,#35616,#35617,#35618,#35619),.UNSPECIFIED.,.F.,.F.,(4,3,3,
3,3,3,3,4),(-47.8312715558983,-47.3711382365461,-46.3888804137623,-45.4066225909785,
-44.4243647681947,-43.4421069454109,-42.4598491226271,-41.5480862487187),
 .UNSPECIFIED.);
#3798=B_SPLINE_CURVE_WITH_KNOTS('',3,(#35624,#35625,#35626,#35627,#35628,
#35629,#35630,#35631,#35632,#35633,#35634,#35635,#35636,#35637,#35638,#35639,
#35640,#35641,#35642,#35643,#35644,#35645),.UNSPECIFIED.,.F.,.F.,(4,3,3,
3,3,3,3,4),(39.0086749840547,39.4673838906395,40.4531564644722,41.438929038305,
42.4247016121377,43.4104741859705,44.3962467598032,45.2918602912343),
 .UNSPECIFIED.);
#3799=B_SPLINE_CURVE_WITH_KNOTS('',3,(#35646,#35647,#35648,#35649,#35650,
#35651,#35652,#35653,#35654,#35655,#35656,#35657,#35658,#35659,#35660,#35661,
#35662,#35663,#35664,#35665,#35666,#35667,#35668,#35669,#35670),
 .UNSPECIFIED.,.F.,.F.,(4,3,3,3,3,3,3,3,4),(-41.5480862487187,-41.4775912998433,
-40.4953334770595,-39.5130756542757,-38.5308178314919,-37.5485600087081,
-36.5663021859243,-35.5840443631405,-35.2649009415391),.UNSPECIFIED.);
#3800=B_SPLINE_CURVE_WITH_KNOTS('',3,(#35675,#35676,#35677,#35678,#35679,
#35680,#35681,#35682,#35683,#35684,#35685,#35686,#35687,#35688,#35689,#35690,
#35691,#35692,#35693,#35694,#35695,#35696),.UNSPECIFIED.,.F.,.F.,(4,3,3,
3,3,3,3,4),(32.7254896768751,33.552748447643,34.5385210214758,35.5242935953085,
36.5100661691413,37.495838742974,38.4816113168067,39.0086749840547),
 .UNSPECIFIED.);
#3801=B_SPLINE_CURVE_WITH_KNOTS('',3,(#35697,#35698,#35699,#35700,#35701,
#35702,#35703,#35704,#35705,#35706,#35707,#35708,#35709,#35710,#35711,#35712,
#35713,#35714,#35715,#35716,#35717,#35718),.UNSPECIFIED.,.F.,.F.,(4,3,3,
3,3,3,3,4),(-35.2649009415391,-34.6017865403566,-33.6195287175728,-32.637270894789,
-31.6550130720052,-30.6727552492214,-29.6904974264376,-28.9817156343595),
 .UNSPECIFIED.);
#3802=B_SPLINE_CURVE_WITH_KNOTS('',3,(#35723,#35724,#35725,#35726,#35727,
#35728,#35729,#35730,#35731,#35732,#35733,#35734,#35735,#35736,#35737,#35738,
#35739,#35740,#35741,#35742,#35743,#35744,#35745,#35746,#35747),
 .UNSPECIFIED.,.F.,.F.,(4,3,3,3,3,3,3,3,4),(26.4423043696955,26.6523404308138,
27.6381130046466,28.6238855784793,29.609658152312,30.5954307261448,31.5812032999775,
32.5669758738103,32.7254896768751),.UNSPECIFIED.);
#3803=B_SPLINE_CURVE_WITH_KNOTS('',3,(#35748,#35749,#35750,#35751,#35752,
#35753,#35754,#35755,#35756,#35757,#35758,#35759,#35760,#35761,#35762,#35763,
#35764,#35765,#35766,#35767,#35768,#35769,#35770,#35771,#35772),
 .UNSPECIFIED.,.F.,.F.,(4,3,3,3,3,3,3,3,4),(-28.9817156343595,-28.7082396036538,
-27.72598178087,-26.7437239580862,-25.7614661353024,-24.7792083125186,-23.7969504897348,
-22.814692666951,-22.6985303271799),.UNSPECIFIED.);
#3804=B_SPLINE_CURVE_WITH_KNOTS('',3,(#35777,#35778,#35779,#35780,#35781,
#35782,#35783,#35784,#35785,#35786,#35787,#35788,#35789,#35790,#35791,#35792,
#35793,#35794,#35795,#35796,#35797,#35798),.UNSPECIFIED.,.F.,.F.,(4,3,3,
3,3,3,3,4),(20.159119062516,20.7377049878173,21.7234775616501,22.7092501354828,
23.6950227093156,24.6807952831483,25.6665678569811,26.4423043696955),
 .UNSPECIFIED.);
#3805=B_SPLINE_CURVE_WITH_KNOTS('',3,(#35799,#35800,#35801,#35802,#35803,
#35804,#35805,#35806,#35807,#35808,#35809,#35810,#35811,#35812,#35813,#35814,
#35815,#35816,#35817,#35818,#35819,#35820),.UNSPECIFIED.,.F.,.F.,(4,3,3,
3,3,3,3,4),(-22.6985303271799,-21.8324348441671,-20.8501770213833,-19.8679191985995,
-18.8856613758157,-17.9034035530319,-16.9211457302481,-16.4153450200003),
 .UNSPECIFIED.);
#3806=B_SPLINE_CURVE_WITH_KNOTS('',3,(#35825,#35826,#35827,#35828,#35829,
#35830,#35831,#35832,#35833,#35834,#35835,#35836,#35837,#35838,#35839,#35840,
#35841,#35842,#35843,#35844,#35845,#35846),.UNSPECIFIED.,.F.,.F.,(4,3,3,
3,3,3,3,4),(13.8759337553364,14.8230695448209,15.8088421186536,16.7946146924864,
17.7803872663191,18.7661598401519,19.7519324139846,20.159119062516),
 .UNSPECIFIED.);
#3807=B_SPLINE_CURVE_WITH_KNOTS('',3,(#35847,#35848,#35849,#35850,#35851,
#35852,#35853,#35854,#35855,#35856,#35857,#35858,#35859,#35860,#35861,#35862,
#35863,#35864,#35865,#35866,#35867,#35868),.UNSPECIFIED.,.F.,.F.,(4,3,3,
3,3,3,3,4),(-16.4153450200003,-15.9388879074643,-14.9566300846805,-13.9743722618967,
-12.9921144391129,-12.0098566163291,-11.0275987935453,-10.1321597128208),
 .UNSPECIFIED.);
#3808=B_SPLINE_CURVE_WITH_KNOTS('',3,(#35874,#35875,#35876,#35877,#35878,
#35879,#35880,#35881,#35882,#35883,#35884,#35885,#35886),.UNSPECIFIED.,
 .F.,.F.,(4,3,3,3,4),(-3.84897440564119,-3.16953621127481,-2.187278388491,
-1.2050205657072,-0.22276274292349),.UNSPECIFIED.);
#3809=B_SPLINE_CURVE_WITH_KNOTS('',3,(#35888,#35889,#35890,#35891,#35892,
#35893,#35894,#35895,#35896,#35897,#35898,#35899),.UNSPECIFIED.,.F.,.F.,
(4,2,2,2,2,4),(0.202168863441194,0.284518942728512,0.379358586733591,0.474198230738669,
0.569037874743748,0.642071595472304),.UNSPECIFIED.);
#3810=B_SPLINE_CURVE_WITH_KNOTS('',3,(#35900,#35901,#35902,#35903,#35904,
#35905,#35906,#35907,#35908,#35909,#35910,#35911,#35912,#35913,#35914,#35915,
#35916,#35917,#35918),.UNSPECIFIED.,.F.,.F.,(4,3,3,3,3,3,4),(2.14497997264832,
2.99379865882794,3.97957123266068,4.96534380649343,5.95111638032618,6.93688895415892,
7.59274844815675),.UNSPECIFIED.);
#3811=B_SPLINE_CURVE_WITH_KNOTS('',3,(#35924,#35925,#35926,#35927,#35928,
#35929,#35930,#35931),.UNSPECIFIED.,.F.,.F.,(4,1,1,1,1,4),(59.690260418206,
60.2123849216376,61.1946427444214,62.1769005672052,63.159158389989,64.1414162127728),
 .UNSPECIFIED.);
#3812=B_SPLINE_CURVE_WITH_KNOTS('',3,(#35934,#35935,#35936,#35937,#35938,
#35939,#35940,#35941,#35942),.UNSPECIFIED.,.F.,.F.,(4,1,1,1,1,1,4),(59.6902604182061,
59.7804194606076,60.7661920344403,61.751964608273,62.7377371821058,63.7235097559385,
64.6638825844083),.UNSPECIFIED.);
#3813=B_SPLINE_CURVE_WITH_KNOTS('',3,(#35947,#35948,#35949,#35950,#35951,
#35952,#35953,#35954,#35955,#35956),.UNSPECIFIED.,.F.,.F.,(4,1,1,1,1,1,
1,4),(53.4070751110265,54.3188379849348,55.3010958077186,56.2833536305024,
57.2656114532862,58.24786927607,59.2301270988538,59.690260418206),
 .UNSPECIFIED.);
#3814=B_SPLINE_CURVE_WITH_KNOTS('',3,(#35957,#35958,#35959,#35960,#35961,
#35962,#35963,#35964,#35965,#35966),.UNSPECIFIED.,.F.,.F.,(4,1,1,1,1,1,
1,4),(53.4070751110265,53.8657840176111,54.8515565914438,55.8373291652766,
56.8231017391093,57.8088743129421,58.7946468867748,59.6902604182061),
 .UNSPECIFIED.);
#3815=B_SPLINE_CURVE_WITH_KNOTS('',3,(#35971,#35972,#35973,#35974,#35975,
#35976,#35977,#35978,#35979,#35980,#35981),.UNSPECIFIED.,.F.,.F.,(4,1,1,
1,1,1,1,1,4),(47.1238898038469,47.4430332254481,48.4252910482319,49.4075488710157,
50.3898066937996,51.3720645165834,52.3543223393672,53.336580162151,53.4070751110265),
 .UNSPECIFIED.);
#3816=B_SPLINE_CURVE_WITH_KNOTS('',3,(#35982,#35983,#35984,#35985,#35986,
#35987,#35988,#35989,#35990,#35991),.UNSPECIFIED.,.F.,.F.,(4,1,1,1,1,1,
1,4),(47.1238898038469,47.9511485746146,48.9369211484474,49.9226937222801,
50.9084662961128,51.8942388699456,52.8800114437783,53.4070751110265),
 .UNSPECIFIED.);
#3817=B_SPLINE_CURVE_WITH_KNOTS('',3,(#35996,#35997,#35998,#35999,#36000,
#36001,#36002,#36003,#36004,#36005),.UNSPECIFIED.,.F.,.F.,(4,1,1,1,1,1,
1,4),(40.8407044966673,41.5494862887453,42.5317441115291,43.5140019343129,
44.4962597570967,45.4785175798805,46.4607754026643,47.1238898038469),
 .UNSPECIFIED.);
#3818=B_SPLINE_CURVE_WITH_KNOTS('',3,(#36006,#36007,#36008,#36009,#36010,
#36011,#36012,#36013,#36014,#36015,#36016),.UNSPECIFIED.,.F.,.F.,(4,1,1,
1,1,1,1,1,4),(40.8407044966673,41.0507405577854,42.0365131316181,43.0222857054509,
44.0080582792836,44.9938308531164,45.9796034269491,46.9653760007819,47.1238898038469),
 .UNSPECIFIED.);
#3819=B_SPLINE_CURVE_WITH_KNOTS('',3,(#36021,#36022,#36023,#36024,#36025,
#36026,#36027,#36028,#36029,#36030,#36031),.UNSPECIFIED.,.F.,.F.,(4,1,1,
1,1,1,1,1,4),(34.5575191894877,34.6736815292587,35.6559393520425,36.6381971748263,
37.6204549976101,38.6027128203939,39.5849706431777,40.5672284659615,40.8407044966673),
 .UNSPECIFIED.);
#3820=B_SPLINE_CURVE_WITH_KNOTS('',3,(#36032,#36033,#36034,#36035,#36036,
#36037,#36038,#36039,#36040,#36041),.UNSPECIFIED.,.F.,.F.,(4,1,1,1,1,1,
1,4),(34.5575191894877,35.1361051147889,36.1218776886216,37.1076502624544,
38.0934228362871,39.0791954101199,40.0649679839526,40.8407044966673),
 .UNSPECIFIED.);
#3821=B_SPLINE_CURVE_WITH_KNOTS('',3,(#36046,#36047,#36048,#36049,#36050,
#36051,#36052,#36053,#36054,#36055),.UNSPECIFIED.,.F.,.F.,(4,1,1,1,1,1,
1,4),(28.2743338823081,28.7801345925558,29.7623924153396,30.7446502381234,
31.7269080609072,32.709165883691,33.6914237064749,34.5575191894877),
 .UNSPECIFIED.);
#3822=B_SPLINE_CURVE_WITH_KNOTS('',3,(#36056,#36057,#36058,#36059,#36060,
#36061,#36062,#36063,#36064,#36065),.UNSPECIFIED.,.F.,.F.,(4,1,1,1,1,1,
1,4),(28.2743338823082,29.2214696717924,30.2072422456252,31.1930148194579,
32.1787873932907,33.1645599671234,34.1503325409562,34.5575191894877),
 .UNSPECIFIED.);
#3823=B_SPLINE_CURVE_WITH_KNOTS('',3,(#36070,#36071,#36072,#36073,#36074,
#36075,#36076,#36077,#36078,#36079),.UNSPECIFIED.,.F.,.F.,(4,1,1,1,1,1,
1,4),(21.9911485751285,22.886587655853,23.8688454786368,24.8511033014206,
25.8333611242044,26.8156189469882,27.797876769772,28.2743338823081),
 .UNSPECIFIED.);
#3824=B_SPLINE_CURVE_WITH_KNOTS('',3,(#36080,#36081,#36082,#36083,#36084,
#36085,#36086,#36087,#36088,#36089,#36090),.UNSPECIFIED.,.F.,.F.,(4,1,1,
1,1,1,1,1,4),(21.9911485751285,22.3210616549632,23.3068342287959,24.2926068026287,
25.2783793764614,26.2641519502942,27.2499245241269,28.2356970979597,28.2743338823082),
 .UNSPECIFIED.);
#3825=B_SPLINE_CURVE_WITH_KNOTS('',3,(#36096,#36097,#36098,#36099,#36100),
 .UNSPECIFIED.,.F.,.F.,(4,1,4),(14.4348810643012,15.420653638134,15.7079632679489),
 .UNSPECIFIED.);
#3826=B_SPLINE_CURVE_WITH_KNOTS('',3,(#36102,#36103,#36104,#36105),
 .UNSPECIFIED.,.F.,.F.,(4,4),(1.38948745034524,1.47775448763829),
 .UNSPECIFIED.);
#3827=B_SPLINE_CURVE_WITH_KNOTS('',3,(#36107,#36108,#36109,#36110),
 .UNSPECIFIED.,.F.,.F.,(4,4),(1.31866677181519,1.38948745034524),
 .UNSPECIFIED.);
#3828=B_SPLINE_CURVE_WITH_KNOTS('',3,(#36111,#36112,#36113,#36114,#36115,
#36116),.UNSPECIFIED.,.F.,.F.,(4,1,1,4),(13.8994448374521,14.0462672507987,
15.0285250735825,15.7079632679489),.UNSPECIFIED.);
#3829=B_SPLINE_CURVE_WITH_KNOTS('',3,(#36122,#36123,#36124,#36125,#36126,
#36127,#36128,#36129),.UNSPECIFIED.,.F.,.F.,(4,1,1,1,1,4),(59.690260418206,
60.2123849216378,61.1946427444216,62.1769005672054,63.1591583899892,64.1414162127731),
 .UNSPECIFIED.);
#3830=B_SPLINE_CURVE_WITH_KNOTS('',3,(#36132,#36133,#36134,#36135,#36136,
#36137,#36138,#36139,#36140),.UNSPECIFIED.,.F.,.F.,(4,1,1,1,1,1,4),(59.6902604182061,
59.7804194606078,60.7661920344405,61.7519646082732,62.737737182106,63.7235097559387,
64.6638825844085),.UNSPECIFIED.);
#3831=B_SPLINE_CURVE_WITH_KNOTS('',3,(#36145,#36146,#36147,#36148,#36149,
#36150,#36151,#36152,#36153,#36154),.UNSPECIFIED.,.F.,.F.,(4,1,1,1,1,1,
1,4),(53.4070751110265,54.318837984935,55.3010958077188,56.2833536305026,
57.2656114532864,58.2478692760702,59.230127098854,59.690260418206),
 .UNSPECIFIED.);
#3832=B_SPLINE_CURVE_WITH_KNOTS('',3,(#36155,#36156,#36157,#36158,#36159,
#36160,#36161,#36162,#36163,#36164),.UNSPECIFIED.,.F.,.F.,(4,1,1,1,1,1,
1,4),(53.4070751110265,53.8657840176113,54.851556591444,55.8373291652768,
56.8231017391095,57.8088743129423,58.794646886775,59.6902604182061),
 .UNSPECIFIED.);
#3833=B_SPLINE_CURVE_WITH_KNOTS('',3,(#36169,#36170,#36171,#36172,#36173,
#36174,#36175,#36176,#36177,#36178,#36179),.UNSPECIFIED.,.F.,.F.,(4,1,1,
1,1,1,1,1,4),(47.1238898038469,47.4430332254484,48.4252910482322,49.407548871016,
50.3898066937998,51.3720645165836,52.3543223393674,53.3365801621512,53.4070751110265),
 .UNSPECIFIED.);
#3834=B_SPLINE_CURVE_WITH_KNOTS('',3,(#36180,#36181,#36182,#36183,#36184,
#36185,#36186,#36187,#36188,#36189),.UNSPECIFIED.,.F.,.F.,(4,1,1,1,1,1,
1,4),(47.1238898038469,47.9511485746148,48.9369211484476,49.9226937222803,
50.908466296113,51.8942388699458,52.8800114437785,53.4070751110265),
 .UNSPECIFIED.);
#3835=B_SPLINE_CURVE_WITH_KNOTS('',3,(#36194,#36195,#36196,#36197,#36198,
#36199,#36200,#36201,#36202,#36203),.UNSPECIFIED.,.F.,.F.,(4,1,1,1,1,1,
1,4),(40.8407044966673,41.5494862887455,42.5317441115293,43.5140019343131,
44.4962597570969,45.4785175798807,46.4607754026645,47.1238898038469),
 .UNSPECIFIED.);
#3836=B_SPLINE_CURVE_WITH_KNOTS('',3,(#36204,#36205,#36206,#36207,#36208,
#36209,#36210,#36211,#36212,#36213,#36214),.UNSPECIFIED.,.F.,.F.,(4,1,1,
1,1,1,1,1,4),(40.8407044966673,41.0507405577856,42.0365131316183,43.0222857054511,
44.0080582792838,44.9938308531166,45.9796034269493,46.9653760007821,47.1238898038469),
 .UNSPECIFIED.);
#3837=B_SPLINE_CURVE_WITH_KNOTS('',3,(#36219,#36220,#36221,#36222,#36223,
#36224,#36225,#36226,#36227,#36228,#36229),.UNSPECIFIED.,.F.,.F.,(4,1,1,
1,1,1,1,1,4),(34.5575191894877,34.6736815292589,35.6559393520427,36.6381971748265,
37.6204549976103,38.6027128203941,39.5849706431779,40.5672284659617,40.8407044966673),
 .UNSPECIFIED.);
#3838=B_SPLINE_CURVE_WITH_KNOTS('',3,(#36230,#36231,#36232,#36233,#36234,
#36235,#36236,#36237,#36238,#36239),.UNSPECIFIED.,.F.,.F.,(4,1,1,1,1,1,
1,4),(34.5575191894877,35.1361051147891,36.1218776886219,37.1076502624546,
38.0934228362874,39.0791954101201,40.0649679839529,40.8407044966673),
 .UNSPECIFIED.);
#3839=B_SPLINE_CURVE_WITH_KNOTS('',3,(#36244,#36245,#36246,#36247,#36248,
#36249,#36250,#36251,#36252,#36253),.UNSPECIFIED.,.F.,.F.,(4,1,1,1,1,1,
1,4),(28.2743338823081,28.780134592556,29.7623924153398,30.7446502381237,
31.7269080609075,32.7091658836913,33.6914237064751,34.5575191894877),
 .UNSPECIFIED.);
#3840=B_SPLINE_CURVE_WITH_KNOTS('',3,(#36254,#36255,#36256,#36257,#36258,
#36259,#36260,#36261,#36262,#36263),.UNSPECIFIED.,.F.,.F.,(4,1,1,1,1,1,
1,4),(28.2743338823081,29.2214696717927,30.2072422456254,31.1930148194582,
32.1787873932909,33.1645599671237,34.1503325409564,34.5575191894877),
 .UNSPECIFIED.);
#3841=B_SPLINE_CURVE_WITH_KNOTS('',3,(#36268,#36269,#36270,#36271,#36272,
#36273,#36274,#36275,#36276,#36277),.UNSPECIFIED.,.F.,.F.,(4,1,1,1,1,1,
1,4),(21.9911485751285,22.8865876558532,23.868845478637,24.8511033014208,
25.8333611242046,26.8156189469884,27.7978767697722,28.2743338823081),
 .UNSPECIFIED.);
#3842=B_SPLINE_CURVE_WITH_KNOTS('',3,(#36278,#36279,#36280,#36281,#36282,
#36283,#36284,#36285,#36286,#36287,#36288),.UNSPECIFIED.,.F.,.F.,(4,1,1,
1,1,1,1,1,4),(21.9911485751285,22.3210616549635,23.3068342287962,24.292606802629,
25.2783793764617,26.2641519502944,27.2499245241272,28.2356970979599,28.2743338823081),
 .UNSPECIFIED.);
#3843=B_SPLINE_CURVE_WITH_KNOTS('',3,(#36294,#36295,#36296,#36297,#36298),
 .UNSPECIFIED.,.F.,.F.,(4,1,4),(14.4348810643015,15.4206536381343,15.7079632679489),
 .UNSPECIFIED.);
#3844=B_SPLINE_CURVE_WITH_KNOTS('',3,(#36300,#36301,#36302,#36303),
 .UNSPECIFIED.,.F.,.F.,(4,4),(1.38948745034523,1.47775448763837),
 .UNSPECIFIED.);
#3845=B_SPLINE_CURVE_WITH_KNOTS('',3,(#36305,#36306,#36307,#36308),
 .UNSPECIFIED.,.F.,.F.,(4,4),(1.31866677181523,1.38948745034523),
 .UNSPECIFIED.);
#3846=B_SPLINE_CURVE_WITH_KNOTS('',3,(#36309,#36310,#36311,#36312,#36313,
#36314),.UNSPECIFIED.,.F.,.F.,(4,1,1,4),(13.8994448374522,14.046267250799,
15.0285250735828,15.7079632679489),.UNSPECIFIED.);
#3847=B_SPLINE_CURVE_WITH_KNOTS('',3,(#36320,#36321,#36322,#36323,#36324,
#36325,#36326,#36327),.UNSPECIFIED.,.F.,.F.,(4,1,1,1,1,4),(59.690260418206,
60.2123849216377,61.1946427444215,62.1769005672053,63.1591583899891,64.1414162127729),
 .UNSPECIFIED.);
#3848=B_SPLINE_CURVE_WITH_KNOTS('',3,(#36330,#36331,#36332,#36333,#36334,
#36335,#36336,#36337,#36338),.UNSPECIFIED.,.F.,.F.,(4,1,1,1,1,1,4),(59.690260418206,
59.7804194606077,60.7661920344404,61.7519646082732,62.7377371821059,63.7235097559387,
64.6638825844084),.UNSPECIFIED.);
#3849=B_SPLINE_CURVE_WITH_KNOTS('',3,(#36343,#36344,#36345,#36346,#36347,
#36348,#36349,#36350,#36351,#36352),.UNSPECIFIED.,.F.,.F.,(4,1,1,1,1,1,
1,4),(53.4070751110265,54.3188379849348,55.3010958077186,56.2833536305025,
57.2656114532863,58.2478692760701,59.2301270988539,59.690260418206),
 .UNSPECIFIED.);
#3850=B_SPLINE_CURVE_WITH_KNOTS('',3,(#36353,#36354,#36355,#36356,#36357,
#36358,#36359,#36360,#36361,#36362),.UNSPECIFIED.,.F.,.F.,(4,1,1,1,1,1,
1,4),(53.4070751110265,53.8657840176112,54.851556591444,55.8373291652767,
56.8231017391094,57.8088743129422,58.7946468867749,59.690260418206),
 .UNSPECIFIED.);
#3851=B_SPLINE_CURVE_WITH_KNOTS('',3,(#36367,#36368,#36369,#36370,#36371,
#36372,#36373,#36374,#36375,#36376,#36377),.UNSPECIFIED.,.F.,.F.,(4,1,1,
1,1,1,1,1,4),(47.1238898038469,47.4430332254482,48.425291048232,49.4075488710158,
50.3898066937996,51.3720645165834,52.3543223393672,53.336580162151,53.4070751110265),
 .UNSPECIFIED.);
#3852=B_SPLINE_CURVE_WITH_KNOTS('',3,(#36378,#36379,#36380,#36381,#36382,
#36383,#36384,#36385,#36386,#36387),.UNSPECIFIED.,.F.,.F.,(4,1,1,1,1,1,
1,4),(47.1238898038469,47.9511485746147,48.9369211484475,49.9226937222802,
50.908466296113,51.8942388699457,52.8800114437785,53.4070751110265),
 .UNSPECIFIED.);
#3853=B_SPLINE_CURVE_WITH_KNOTS('',3,(#36392,#36393,#36394,#36395,#36396,
#36397,#36398,#36399,#36400,#36401),.UNSPECIFIED.,.F.,.F.,(4,1,1,1,1,1,
1,4),(40.8407044966673,41.5494862887453,42.5317441115292,43.514001934313,
44.4962597570968,45.4785175798806,46.4607754026644,47.1238898038469),
 .UNSPECIFIED.);
#3854=B_SPLINE_CURVE_WITH_KNOTS('',3,(#36402,#36403,#36404,#36405,#36406,
#36407,#36408,#36409,#36410,#36411,#36412),.UNSPECIFIED.,.F.,.F.,(4,1,1,
1,1,1,1,1,4),(40.8407044966673,41.0507405577855,42.0365131316183,43.022285705451,
44.0080582792838,44.9938308531165,45.9796034269493,46.965376000782,47.1238898038469),
 .UNSPECIFIED.);
#3855=B_SPLINE_CURVE_WITH_KNOTS('',3,(#36417,#36418,#36419,#36420,#36421,
#36422,#36423,#36424,#36425,#36426,#36427),.UNSPECIFIED.,.F.,.F.,(4,1,1,
1,1,1,1,1,4),(34.5575191894877,34.6736815292587,35.6559393520425,36.6381971748263,
37.6204549976101,38.6027128203939,39.5849706431777,40.5672284659615,40.8407044966673),
 .UNSPECIFIED.);
#3856=B_SPLINE_CURVE_WITH_KNOTS('',3,(#36428,#36429,#36430,#36431,#36432,
#36433,#36434,#36435,#36436,#36437),.UNSPECIFIED.,.F.,.F.,(4,1,1,1,1,1,
1,4),(34.5575191894877,35.1361051147891,36.1218776886218,37.1076502624546,
38.0934228362873,39.07919541012,40.0649679839528,40.8407044966673),
 .UNSPECIFIED.);
#3857=B_SPLINE_CURVE_WITH_KNOTS('',3,(#36442,#36443,#36444,#36445,#36446,
#36447,#36448,#36449,#36450,#36451),.UNSPECIFIED.,.F.,.F.,(4,1,1,1,1,1,
1,4),(28.2743338823081,28.7801345925559,29.7623924153397,30.7446502381235,
31.7269080609073,32.7091658836911,33.6914237064749,34.5575191894877),
 .UNSPECIFIED.);
#3858=B_SPLINE_CURVE_WITH_KNOTS('',3,(#36452,#36453,#36454,#36455,#36456,
#36457,#36458,#36459,#36460,#36461),.UNSPECIFIED.,.F.,.F.,(4,1,1,1,1,1,
1,4),(28.2743338823081,29.2214696717926,30.2072422456253,31.1930148194581,
32.1787873932908,33.1645599671236,34.1503325409563,34.5575191894877),
 .UNSPECIFIED.);
#3859=B_SPLINE_CURVE_WITH_KNOTS('',3,(#36466,#36467,#36468,#36469,#36470,
#36471,#36472,#36473,#36474,#36475),.UNSPECIFIED.,.F.,.F.,(4,1,1,1,1,1,
1,4),(21.9911485751285,22.886587655853,23.8688454786368,24.8511033014206,
25.8333611242044,26.8156189469882,27.797876769772,28.2743338823081),
 .UNSPECIFIED.);
#3860=B_SPLINE_CURVE_WITH_KNOTS('',3,(#36476,#36477,#36478,#36479,#36480,
#36481,#36482,#36483,#36484,#36485,#36486),.UNSPECIFIED.,.F.,.F.,(4,1,1,
1,1,1,1,1,4),(21.9911485751285,22.3210616549634,23.3068342287961,24.2926068026289,
25.2783793764616,26.2641519502944,27.2499245241271,28.2356970979599,28.2743338823081),
 .UNSPECIFIED.);
#3861=B_SPLINE_CURVE_WITH_KNOTS('',3,(#36492,#36493,#36494,#36495,#36496),
 .UNSPECIFIED.,.F.,.F.,(4,1,4),(14.4348810643014,15.4206536381342,15.7079632679489),
 .UNSPECIFIED.);
#3862=B_SPLINE_CURVE_WITH_KNOTS('',3,(#36498,#36499,#36500,#36501),
 .UNSPECIFIED.,.F.,.F.,(4,4),(1.38948745034523,1.47775448763834),
 .UNSPECIFIED.);
#3863=B_SPLINE_CURVE_WITH_KNOTS('',3,(#36503,#36504,#36505,#36506),
 .UNSPECIFIED.,.F.,.F.,(4,4),(1.31866677181519,1.38948745034523),
 .UNSPECIFIED.);
#3864=B_SPLINE_CURVE_WITH_KNOTS('',3,(#36507,#36508,#36509,#36510,#36511,
#36512),.UNSPECIFIED.,.F.,.F.,(4,1,1,4),(13.8994448374521,14.0462672507987,
15.0285250735825,15.7079632679489),.UNSPECIFIED.);
#3865=B_SPLINE_CURVE_WITH_KNOTS('',3,(#36737,#36738,#36739,#36740,#36741,
#36742,#36743,#36744,#36745,#36746,#36747,#36748),.UNSPECIFIED.,.F.,.F.,
(4,2,2,2,2,4),(0.,0.0939720040697306,0.191040004611618,0.294727654301763,
0.396757250727393,0.506753893125291),.UNSPECIFIED.);
#3866=B_SPLINE_CURVE_WITH_KNOTS('',3,(#36749,#36750,#36751,#36752,#36753,
#36754,#36755,#36756,#36757,#36758,#36759,#36760,#36761,#36762,#36763,#36764,
#36765,#36766,#36767,#36768,#36769,#36770,#36771,#36772,#36773),
 .UNSPECIFIED.,.F.,.F.,(4,3,3,3,3,3,3,3,4),(-10.1321597128208,-10.0453409707615,
-9.06308314797765,-8.08082532519384,-7.09856750241004,-6.11630967962623,
-5.13405185684243,-4.15179403405862,-3.84897440564119),.UNSPECIFIED.);
#3867=B_SPLINE_CURVE_WITH_KNOTS('',3,(#36774,#36775,#36776,#36777,#36778,
#36779,#36780,#36781,#36782,#36783,#36784,#36785,#36786,#36787,#36788,#36789,
#36790,#36791,#36792,#36793,#36794,#36795,#36796,#36797,#36798,#36799,#36800,
#36801,#36802,#36803,#36804,#36805,#36806,#36807,#36808,#36809,#36810,#36811,
#36812,#36813,#36814,#36815,#36816,#36817,#36818,#36819,#36820,#36821,#36822,
#36823,#36824,#36825,#36826,#36827,#36828,#36829,#36830,#36831,#36832,#36833,
#36834,#36835,#36836,#36837,#36838,#36839,#36840,#36841,#36842,#36843,#36844,
#36845,#36846,#36847,#36848,#36849,#36850,#36851,#36852,#36853,#36854,#36855,
#36856,#36857,#36858,#36859,#36860,#36861,#36862,#36863,#36864,#36865,#36866,
#36867),.UNSPECIFIED.,.F.,.F.,(4,3,3,3,3,3,3,3,3,3,3,3,3,3,3,3,3,3,3,3,
3,3,3,3,3,3,3,3,3,3,3,4),(-0.566847306048089,-0.536661395473507,-0.506059016755951,
-0.497326650809489,-0.490463963747992,-0.460323979286527,-0.437444973964932,
-0.425645739517285,-0.420672568156472,-0.391255347604605,-0.362370453937528,
-0.334033562322262,-0.319848155920138,-0.313024468520039,-0.308668713479008,
-0.280666905255211,-0.277291936713766,-0.248847901203608,-0.219408150886093,
-0.20505599758711,-0.200814316443281,-0.172984028418683,-0.14523356468346,
-0.11796097413067,-0.104882089697273,-0.100481501514816,-0.0962956903621217,
-0.0696281223924694,-0.0434020873669322,-0.0179348500541518,-0.0133298986634882,
0.),.UNSPECIFIED.);
#3868=B_SPLINE_CURVE_WITH_KNOTS('',3,(#36868,#36869,#36870,#36871,#36872,
#36873,#36874,#36875,#36876,#36877,#36878),.UNSPECIFIED.,.F.,.F.,(4,1,1,
1,1,1,1,1,4),(15.7079632679489,16.0107828963664,16.9930407191502,17.975298541934,
18.9575563647178,19.9398141875016,20.9220720102854,21.9043298330692,21.9911485751285),
 .UNSPECIFIED.);
#3869=B_SPLINE_CURVE_WITH_KNOTS('',3,(#36880,#36881,#36882,#36883,#36884,
#36885,#36886,#36887,#36888,#36889),.UNSPECIFIED.,.F.,.F.,(4,1,1,1,1,1,
1,4),(15.7079632679489,16.4064262119669,17.3921987857997,18.3779713596324,
19.3637439334652,20.3495165072979,21.3352890811306,21.9911485751285),
 .UNSPECIFIED.);
#3870=B_SPLINE_CURVE_WITH_KNOTS('',3,(#37114,#37115,#37116,#37117,#37118,
#37119,#37120,#37121,#37122,#37123,#37124,#37125,#37126,#37127),
 .UNSPECIFIED.,.F.,.F.,(4,2,2,2,2,2,4),(0.,0.122341475621437,0.233773139394309,
0.328065713266122,0.418619986828863,0.511091556851628,0.605234881207264),
 .UNSPECIFIED.);
#3871=B_SPLINE_CURVE_WITH_KNOTS('',3,(#37128,#37129,#37130,#37131,#37132,
#37133,#37134,#37135,#37136,#37137,#37138,#37139,#37140,#37141,#37142,#37143,
#37144,#37145,#37146,#37147,#37148,#37149,#37150,#37151,#37152,#37153,#37154,
#37155,#37156,#37157,#37158,#37159,#37160,#37161,#37162,#37163,#37164,#37165,
#37166,#37167,#37168,#37169,#37170,#37171,#37172,#37173,#37174,#37175,#37176,
#37177,#37178,#37179,#37180,#37181,#37182,#37183,#37184,#37185,#37186,#37187,
#37188,#37189,#37190,#37191,#37192,#37193,#37194,#37195,#37196,#37197,#37198,
#37199,#37200,#37201,#37202,#37203,#37204,#37205,#37206,#37207,#37208,#37209,
#37210,#37211,#37212,#37213,#37214,#37215,#37216,#37217,#37218,#37219,#37220,
#37221),.UNSPECIFIED.,.F.,.F.,(4,3,3,3,3,3,3,3,3,3,3,3,3,3,3,3,3,3,3,3,
3,3,3,3,3,3,3,3,3,3,3,4),(-0.569248610399481,-0.543568168745277,-0.517260903357168,
-0.510376876051222,-0.504799164129705,-0.477737437228182,-0.456135094562755,
-0.449160314492888,-0.442513472342989,-0.414784053155389,-0.386626551258596,
-0.358686347322027,-0.345244434467712,-0.34080557042231,-0.33631776891126,
-0.30739232536096,-0.30491869590477,-0.277130714479983,-0.248706827603265,
-0.233107805251665,-0.228466848903046,-0.199477467537415,-0.169916466664947,
-0.14012139652544,-0.124355841110362,-0.118742223062163,-0.114429203491767,
-0.083895606230837,-0.0533233406469446,-0.0233305921302133,-0.0139969532048209,
0.),.UNSPECIFIED.);
#3872=B_SPLINE_CURVE_WITH_KNOTS('',3,(#37222,#37223,#37224,#37225,#37226,
#37227,#37228,#37229,#37230,#37231,#37232,#37233,#37234,#37235,#37236,#37237,
#37238,#37239,#37240,#37241,#37242,#37243,#37244,#37245,#37246),
 .UNSPECIFIED.,.F.,.F.,(4,3,3,3,3,3,3,3,4),(7.59274844815675,7.92266152799166,
8.90843410182441,9.89420667565716,10.8799792494899,11.8657518233226,12.8515243971554,
13.8372969709881,13.8759337553364),.UNSPECIFIED.);
#3873=B_SPLINE_CURVE_WITH_KNOTS('',3,(#37471,#37472,#37473,#37474,#37475,
#37476,#37477,#37478,#37479,#37480,#37481,#37482),.UNSPECIFIED.,.F.,.F.,
(4,2,2,2,2,4),(0.,0.0939720040697043,0.191040004611567,0.294727654301641,
0.396757250727202,0.506753893125061),.UNSPECIFIED.);
#3874=B_SPLINE_CURVE_WITH_KNOTS('',3,(#37483,#37484,#37485,#37486,#37487,
#37488,#37489,#37490,#37491,#37492,#37493,#37494,#37495,#37496,#37497,#37498,
#37499,#37500,#37501,#37502,#37503,#37504,#37505,#37506,#37507),
 .UNSPECIFIED.,.F.,.F.,(4,3,3,3,3,3,3,3,4),(-10.1321597128207,-10.0453409707616,
-9.06308314797777,-8.08082532519396,-7.09856750241015,-6.11630967962635,
-5.13405185684255,-4.15179403405874,-3.84897440564108),.UNSPECIFIED.);
#3875=B_SPLINE_CURVE_WITH_KNOTS('',3,(#37508,#37509,#37510,#37511,#37512,
#37513,#37514,#37515,#37516,#37517,#37518,#37519,#37520,#37521,#37522,#37523,
#37524,#37525,#37526,#37527,#37528,#37529,#37530,#37531,#37532,#37533,#37534,
#37535,#37536,#37537,#37538,#37539,#37540,#37541,#37542,#37543,#37544,#37545,
#37546,#37547,#37548,#37549,#37550,#37551,#37552,#37553,#37554,#37555,#37556,
#37557,#37558,#37559,#37560,#37561,#37562,#37563,#37564,#37565,#37566,#37567,
#37568,#37569,#37570,#37571,#37572,#37573,#37574,#37575,#37576,#37577,#37578,
#37579,#37580,#37581,#37582,#37583,#37584,#37585,#37586,#37587,#37588,#37589,
#37590,#37591,#37592,#37593,#37594,#37595,#37596,#37597,#37598,#37599,#37600,
#37601),.UNSPECIFIED.,.F.,.F.,(4,3,3,3,3,3,3,3,3,3,3,3,3,3,3,3,3,3,3,3,
3,3,3,3,3,3,3,3,3,3,3,4),(-0.566847306048109,-0.536661395468383,-0.506059016754568,
-0.497326650805892,-0.490463963797695,-0.460323979336568,-0.437444974008718,
-0.425645739590181,-0.420672568143048,-0.391255347593568,-0.362370453926602,
-0.334033562313392,-0.319848155913487,-0.313024468510124,-0.308668713420628,
-0.280666905198208,-0.277291936713773,-0.248847901202399,-0.219408150885036,
-0.205055997585609,-0.200814316430888,-0.172984028406577,-0.145233564671321,
-0.117960974121696,-0.104882089689421,-0.100481501534044,-0.0962956903887221,
-0.0696281224182907,-0.04340208739252,-0.0179348500828051,-0.0133298986634936,
0.),.UNSPECIFIED.);
#3876=B_SPLINE_CURVE_WITH_KNOTS('',3,(#37602,#37603,#37604,#37605,#37606,
#37607,#37608,#37609,#37610,#37611,#37612),.UNSPECIFIED.,.F.,.F.,(4,1,1,
1,1,1,1,1,4),(15.7079632679489,16.0107828963666,16.9930407191504,17.9752985419342,
18.957556364718,19.9398141875018,20.9220720102856,21.9043298330694,21.9911485751285),
 .UNSPECIFIED.);
#3877=B_SPLINE_CURVE_WITH_KNOTS('',3,(#37614,#37615,#37616,#37617,#37618,
#37619,#37620,#37621,#37622,#37623),.UNSPECIFIED.,.F.,.F.,(4,1,1,1,1,1,
1,4),(15.7079632679489,16.406426211967,17.3921987857997,18.3779713596325,
19.3637439334652,20.349516507298,21.3352890811307,21.9911485751285),
 .UNSPECIFIED.);
#3878=B_SPLINE_CURVE_WITH_KNOTS('',3,(#37848,#37849,#37850,#37851,#37852,
#37853,#37854,#37855,#37856,#37857,#37858,#37859,#37860,#37861),
 .UNSPECIFIED.,.F.,.F.,(4,2,2,2,2,2,4),(0.,0.12234147562142,0.233773139394286,
0.328065713266116,0.418619986828843,0.511091556851594,0.605234881207211),
 .UNSPECIFIED.);
#3879=B_SPLINE_CURVE_WITH_KNOTS('',3,(#37862,#37863,#37864,#37865,#37866,
#37867,#37868,#37869,#37870,#37871,#37872,#37873,#37874,#37875,#37876,#37877,
#37878,#37879,#37880,#37881,#37882,#37883,#37884,#37885,#37886,#37887,#37888,
#37889,#37890,#37891,#37892,#37893,#37894,#37895,#37896,#37897,#37898,#37899,
#37900,#37901,#37902,#37903,#37904,#37905,#37906,#37907,#37908,#37909,#37910,
#37911,#37912,#37913,#37914,#37915,#37916,#37917,#37918,#37919,#37920,#37921,
#37922,#37923,#37924,#37925,#37926,#37927,#37928,#37929,#37930,#37931,#37932,
#37933,#37934,#37935,#37936,#37937,#37938,#37939,#37940,#37941,#37942,#37943,
#37944,#37945,#37946,#37947,#37948,#37949,#37950,#37951,#37952,#37953,#37954,
#37955),.UNSPECIFIED.,.F.,.F.,(4,3,3,3,3,3,3,3,3,3,3,3,3,3,3,3,3,3,3,3,
3,3,3,3,3,3,3,3,3,3,3,4),(-0.569248610399453,-0.543568168745332,-0.517260903359189,
-0.510376876055068,-0.504799164150761,-0.477737437250597,-0.456135094582367,
-0.44916031457044,-0.442513472333628,-0.414784053145682,-0.386626551248794,
-0.358686347310781,-0.345244434459274,-0.340805570317779,-0.336317768890034,
-0.307392325339199,-0.304918695904753,-0.277130714478965,-0.248706827603545,
-0.233107805253122,-0.228466848911822,-0.199477467538772,-0.169916466667501,
-0.140121396526104,-0.124355841110945,-0.118742223070016,-0.114429203500742,
-0.0838956062406663,-0.0533233406584259,-0.023330592138883,-0.013996953204826,
0.),.UNSPECIFIED.);
#3880=B_SPLINE_CURVE_WITH_KNOTS('',3,(#37956,#37957,#37958,#37959,#37960,
#37961,#37962,#37963,#37964,#37965,#37966,#37967,#37968,#37969,#37970,#37971,
#37972,#37973,#37974,#37975,#37976,#37977,#37978,#37979,#37980),
 .UNSPECIFIED.,.F.,.F.,(4,3,3,3,3,3,3,3,4),(7.59274844815675,7.92266152799173,
8.90843410182448,9.89420667565722,10.87997924949,11.8657518233227,12.8515243971555,
13.8372969709882,13.8759337553364),.UNSPECIFIED.);
#3881=B_SPLINE_CURVE_WITH_KNOTS('',3,(#38205,#38206,#38207,#38208,#38209,
#38210,#38211,#38212,#38213,#38214,#38215,#38216),.UNSPECIFIED.,.F.,.F.,
(4,2,2,2,2,4),(0.,0.09397200406971,0.191040004611562,0.294727654301647,
0.396757250727143,0.506753893124957),.UNSPECIFIED.);
#3882=B_SPLINE_CURVE_WITH_KNOTS('',3,(#38217,#38218,#38219,#38220,#38221,
#38222,#38223,#38224,#38225,#38226,#38227,#38228,#38229,#38230,#38231,#38232,
#38233,#38234,#38235,#38236,#38237,#38238,#38239,#38240,#38241),
 .UNSPECIFIED.,.F.,.F.,(4,3,3,3,3,3,3,3,4),(-10.1321597128207,-10.0453409707614,
-9.06308314797754,-8.08082532519374,-7.09856750240993,-6.11630967962613,
-5.13405185684232,-4.15179403405851,-3.84897440564107),.UNSPECIFIED.);
#3883=B_SPLINE_CURVE_WITH_KNOTS('',3,(#38242,#38243,#38244,#38245,#38246,
#38247,#38248,#38249,#38250,#38251,#38252,#38253,#38254,#38255,#38256,#38257,
#38258,#38259,#38260,#38261,#38262,#38263,#38264,#38265,#38266,#38267,#38268,
#38269,#38270,#38271,#38272,#38273,#38274,#38275,#38276,#38277,#38278,#38279,
#38280,#38281,#38282,#38283,#38284,#38285,#38286,#38287,#38288,#38289,#38290,
#38291,#38292,#38293,#38294,#38295,#38296,#38297,#38298,#38299,#38300,#38301,
#38302,#38303,#38304,#38305,#38306,#38307,#38308,#38309,#38310,#38311,#38312,
#38313,#38314,#38315,#38316,#38317,#38318,#38319,#38320,#38321,#38322,#38323,
#38324,#38325,#38326,#38327,#38328,#38329,#38330,#38331,#38332,#38333,#38334,
#38335),.UNSPECIFIED.,.F.,.F.,(4,3,3,3,3,3,3,3,3,3,3,3,3,3,3,3,3,3,3,3,
3,3,3,3,3,3,3,3,3,3,3,4),(-0.566847306048032,-0.536661395466917,-0.506059016751992,
-0.497326650803245,-0.490463963758655,-0.460323979298246,-0.437444973975183,
-0.425645739534236,-0.420672568143549,-0.391255347592175,-0.362370453925434,
-0.33403356230877,-0.319848155910013,-0.313024468504981,-0.308668713474399,
-0.280666905255003,-0.277291936713742,-0.248847901201056,-0.219408150883858,
-0.205055997583148,-0.20081431637463,-0.172984028349664,-0.145233564613907,
-0.117960974064228,-0.104882089639133,-0.100481501504229,-0.0962956903645289,
-0.0696281223931707,-0.0434020873672608,-0.0179348500541578,-0.0133298986634736,
0.),.UNSPECIFIED.);
#3884=B_SPLINE_CURVE_WITH_KNOTS('',3,(#38336,#38337,#38338,#38339,#38340,
#38341,#38342,#38343,#38344,#38345,#38346),.UNSPECIFIED.,.F.,.F.,(4,1,1,
1,1,1,1,1,4),(15.7079632679489,16.0107828963663,16.9930407191502,17.975298541934,
18.9575563647178,19.9398141875016,20.9220720102854,21.9043298330692,21.9911485751285),
 .UNSPECIFIED.);
#3885=B_SPLINE_CURVE_WITH_KNOTS('',3,(#38348,#38349,#38350,#38351,#38352,
#38353,#38354,#38355,#38356,#38357),.UNSPECIFIED.,.F.,.F.,(4,1,1,1,1,1,
1,4),(15.7079632679489,16.4064262119667,17.3921987857995,18.3779713596322,
19.363743933465,20.3495165072977,21.3352890811305,21.9911485751285),
 .UNSPECIFIED.);
#3886=B_SPLINE_CURVE_WITH_KNOTS('',3,(#38582,#38583,#38584,#38585,#38586,
#38587,#38588,#38589,#38590,#38591,#38592,#38593,#38594,#38595),
 .UNSPECIFIED.,.F.,.F.,(4,2,2,2,2,2,4),(0.,0.122341475621424,0.233773139394306,
0.328065713266132,0.41861998682885,0.511091556851618,0.605234881207287),
 .UNSPECIFIED.);
#3887=B_SPLINE_CURVE_WITH_KNOTS('',3,(#38596,#38597,#38598,#38599,#38600,
#38601,#38602,#38603,#38604,#38605,#38606,#38607,#38608,#38609,#38610,#38611,
#38612,#38613,#38614,#38615,#38616,#38617,#38618,#38619,#38620,#38621,#38622,
#38623,#38624,#38625,#38626,#38627,#38628,#38629,#38630,#38631,#38632,#38633,
#38634,#38635,#38636,#38637,#38638,#38639,#38640,#38641,#38642,#38643,#38644,
#38645,#38646,#38647,#38648,#38649,#38650,#38651,#38652,#38653,#38654,#38655,
#38656,#38657,#38658,#38659,#38660,#38661,#38662,#38663,#38664,#38665,#38666,
#38667,#38668,#38669,#38670,#38671,#38672,#38673,#38674,#38675,#38676,#38677,
#38678,#38679,#38680,#38681,#38682,#38683,#38684,#38685,#38686,#38687,#38688,
#38689),.UNSPECIFIED.,.F.,.F.,(4,3,3,3,3,3,3,3,3,3,3,3,3,3,3,3,3,3,3,3,
3,3,3,3,3,3,3,3,3,3,3,4),(-0.569248610399429,-0.543568168745069,-0.517260903354712,
-0.510376876043647,-0.504799164152385,-0.477737437252708,-0.456135094584214,
-0.449160314584278,-0.44251347235757,-0.414784053166835,-0.386626551270024,
-0.358686347331947,-0.345244434475149,-0.340805570470318,-0.336317768921927,
-0.307392325367316,-0.304918695904754,-0.277130714480542,-0.248706827608405,
-0.233107805261332,-0.2284668489227,-0.199477467554332,-0.169916466682518,
-0.140121396541974,-0.12435584112483,-0.118742223078146,-0.114429203510237,
-0.0838956062485887,-0.0533233406698207,-0.0233305921507268,-0.0139969532048219,
0.),.UNSPECIFIED.);
#3888=B_SPLINE_CURVE_WITH_KNOTS('',3,(#38690,#38691,#38692,#38693,#38694,
#38695,#38696,#38697,#38698,#38699,#38700,#38701,#38702,#38703,#38704,#38705,
#38706,#38707,#38708,#38709,#38710,#38711,#38712,#38713,#38714),
 .UNSPECIFIED.,.F.,.F.,(4,3,3,3,3,3,3,3,4),(7.59274844815675,7.92266152799146,
8.90843410182421,9.89420667565695,10.8799792494897,11.8657518233224,12.8515243971552,
13.8372969709879,13.8759337553364),.UNSPECIFIED.);
#3889=B_SPLINE_CURVE_WITH_KNOTS('',3,(#38945,#38946,#38947,#38948,#38949,
#38950,#38951,#38952,#38953,#38954,#38955,#38956),.UNSPECIFIED.,.F.,.F.,
(4,2,2,2,2,4),(0.,0.0939720040697054,0.191040004611548,0.294727654301647,
0.396757250727165,0.50675389312503),.UNSPECIFIED.);
#3890=B_SPLINE_CURVE_WITH_KNOTS('',3,(#38957,#38958,#38959,#38960,#38961,
#38962,#38963,#38964,#38965,#38966,#38967,#38968,#38969,#38970,#38971,#38972,
#38973,#38974,#38975,#38976,#38977,#38978,#38979,#38980,#38981),
 .UNSPECIFIED.,.F.,.F.,(4,3,3,3,3,3,3,3,4),(-10.1321597128207,-10.0453409707613,
-9.06308314797754,-8.08082532519373,-7.09856750240993,-6.11630967962612,
-5.13405185684231,-4.15179403405851,-3.84897440564113),.UNSPECIFIED.);
#3891=B_SPLINE_CURVE_WITH_KNOTS('',3,(#38982,#38983,#38984,#38985,#38986,
#38987,#38988,#38989,#38990,#38991,#38992,#38993,#38994,#38995,#38996,#38997,
#38998,#38999,#39000,#39001,#39002,#39003,#39004,#39005,#39006,#39007,#39008,
#39009,#39010,#39011,#39012,#39013,#39014,#39015,#39016,#39017,#39018,#39019,
#39020,#39021,#39022,#39023,#39024,#39025,#39026,#39027,#39028,#39029,#39030,
#39031,#39032,#39033,#39034,#39035,#39036,#39037,#39038,#39039,#39040,#39041,
#39042,#39043,#39044,#39045,#39046,#39047,#39048,#39049,#39050,#39051,#39052,
#39053,#39054,#39055,#39056,#39057,#39058,#39059,#39060,#39061,#39062,#39063,
#39064,#39065,#39066,#39067,#39068,#39069,#39070,#39071,#39072,#39073,#39074,
#39075),.UNSPECIFIED.,.F.,.F.,(4,3,3,3,3,3,3,3,3,3,3,3,3,3,3,3,3,3,3,3,
3,3,3,3,3,3,3,3,3,3,3,4),(-0.566847306048062,-0.53666139547184,-0.506059016754063,
-0.49732665080814,-0.490463963821467,-0.460323979361128,-0.437444974030206,
-0.425645739625527,-0.42067256805228,-0.391255347501007,-0.362370453835405,
-0.334033562222944,-0.319848155845646,-0.313024468412086,-0.30866871342461,
-0.280666905204325,-0.277291936713753,-0.248847901203833,-0.21940815088629,
-0.205055997588386,-0.200814316362458,-0.17298402833657,-0.145233564602108,
-0.117960974053518,-0.104882089629765,-0.100481501481134,-0.0962956902597121,
-0.0696281222892088,-0.043402087264509,-0.0179348499542768,-0.0133298986634882,
0.),.UNSPECIFIED.);
#3892=B_SPLINE_CURVE_WITH_KNOTS('',3,(#39076,#39077,#39078,#39079,#39080,
#39081,#39082,#39083,#39084,#39085,#39086),.UNSPECIFIED.,.F.,.F.,(4,1,1,
1,1,1,1,1,4),(15.7079632679489,16.0107828963663,16.9930407191501,17.9752985419339,
18.9575563647177,19.9398141875016,20.9220720102854,21.9043298330692,21.9911485751285),
 .UNSPECIFIED.);
#3893=B_SPLINE_CURVE_WITH_KNOTS('',3,(#39088,#39089,#39090,#39091,#39092,
#39093,#39094,#39095,#39096,#39097),.UNSPECIFIED.,.F.,.F.,(4,1,1,1,1,1,
1,4),(15.7079632679489,16.4064262119669,17.3921987857997,18.3779713596324,
19.3637439334652,20.3495165072979,21.3352890811306,21.9911485751285),
 .UNSPECIFIED.);
#3894=B_SPLINE_CURVE_WITH_KNOTS('',3,(#39322,#39323,#39324,#39325,#39326,
#39327,#39328,#39329,#39330,#39331,#39332,#39333,#39334,#39335),
 .UNSPECIFIED.,.F.,.F.,(4,2,2,2,2,2,4),(0.,0.122341475621436,0.233773139394342,
0.328065713266181,0.418619986828953,0.511091556851744,0.605234881207393),
 .UNSPECIFIED.);
#3895=B_SPLINE_CURVE_WITH_KNOTS('',3,(#39336,#39337,#39338,#39339,#39340,
#39341,#39342,#39343,#39344,#39345,#39346,#39347,#39348,#39349,#39350,#39351,
#39352,#39353,#39354,#39355,#39356,#39357,#39358,#39359,#39360,#39361,#39362,
#39363,#39364,#39365,#39366,#39367,#39368,#39369,#39370,#39371,#39372,#39373,
#39374,#39375,#39376,#39377,#39378,#39379,#39380,#39381,#39382,#39383,#39384,
#39385,#39386,#39387,#39388,#39389,#39390,#39391,#39392,#39393,#39394,#39395,
#39396,#39397,#39398,#39399,#39400,#39401,#39402,#39403,#39404,#39405,#39406,
#39407,#39408,#39409,#39410,#39411,#39412,#39413,#39414,#39415,#39416,#39417,
#39418,#39419,#39420,#39421,#39422,#39423,#39424,#39425,#39426,#39427,#39428,
#39429),.UNSPECIFIED.,.F.,.F.,(4,3,3,3,3,3,3,3,3,3,3,3,3,3,3,3,3,3,3,3,
3,3,3,3,3,3,3,3,3,3,3,4),(-0.56924861039948,-0.543568168743065,-0.517260903356135,
-0.51037687605013,-0.504799164228155,-0.477737437329509,-0.456135094651419,
-0.449160314870292,-0.442513472316536,-0.414784053132704,-0.386626551235781,
-0.358686347299406,-0.345244434450751,-0.340805570359703,-0.336317768898936,
-0.307392325353166,-0.304918695904789,-0.277130714479285,-0.248706827607001,
-0.233107805259422,-0.228466848824526,-0.199477467452263,-0.169916466577901,
-0.140121396437131,-0.124355841033094,-0.118742223014663,-0.114429203367402,
-0.0838956061053275,-0.0533233405264678,-0.02333059201217,-0.0139969532048341,
0.),.UNSPECIFIED.);
#3896=B_SPLINE_CURVE_WITH_KNOTS('',3,(#39430,#39431,#39432,#39433,#39434,
#39435,#39436,#39437,#39438,#39439,#39440,#39441,#39442,#39443,#39444,#39445,
#39446,#39447,#39448,#39449,#39450,#39451,#39452,#39453,#39454),
 .UNSPECIFIED.,.F.,.F.,(4,3,3,3,3,3,3,3,4),(7.5927484481567,7.92266152799159,
8.90843410182433,9.89420667565708,10.8799792494898,11.8657518233226,12.8515243971553,
13.8372969709881,13.8759337553363),.UNSPECIFIED.);
#3897=B_SPLINE_CURVE_WITH_KNOTS('',3,(#39458,#39459,#39460,#39461,#39462,
#39463,#39464,#39465,#39466,#39467,#39468,#39469,#39470,#39471,#39472,#39473,
#39474,#39475,#39476,#39477,#39478,#39479,#39480,#39481,#39482,#39483,#39484,
#39485,#39486,#39487,#39488,#39489,#39490,#39491,#39492,#39493,#39494,#39495,
#39496,#39497,#39498,#39499,#39500,#39501,#39502,#39503,#39504,#39505,#39506,
#39507,#39508,#39509,#39510,#39511,#39512,#39513,#39514,#39515,#39516,#39517,
#39518,#39519,#39520,#39521,#39522,#39523,#39524,#39525,#39526,#39527,#39528,
#39529,#39530,#39531,#39532,#39533,#39534,#39535,#39536,#39537,#39538,#39539,
#39540,#39541,#39542,#39543,#39544,#39545),.UNSPECIFIED.,.F.,.F.,(4,3,3,
3,3,3,3,3,3,3,3,3,3,3,3,3,3,3,3,3,3,3,3,3,3,3,3,3,3,4),(-0.378621596831439,
-0.359797351563908,-0.34785658095904,-0.339691168491925,-0.33536812849937,
-0.31549598337044,-0.301162672408894,-0.29722662849187,-0.293222646083178,
-0.272820189148395,-0.252122545583708,-0.239299283107299,-0.228793967352159,
-0.22450143777299,-0.203196862142534,-0.200829495678071,-0.180342172305092,
-0.158301477242566,-0.154267258991073,-0.150798053974315,-0.129414619358608,
-0.107580334749735,-0.0856137297500737,-0.0801849312914882,-0.075938243267924,
-0.0533906056048975,-0.0308184408529723,-0.00876003301059033,-0.00401661180488397,
0.),.UNSPECIFIED.);
#3898=B_SPLINE_CURVE_WITH_KNOTS('',3,(#39546,#39547,#39548,#39549,#39550,
#39551,#39552,#39553,#39554,#39555,#39556,#39557,#39558,#39559,#39560,#39561,
#39562,#39563,#39564,#39565,#39566,#39567,#39568,#39569,#39570,#39571,#39572,
#39573,#39574,#39575,#39576,#39577,#39578,#39579,#39580,#39581,#39582,#39583,
#39584,#39585,#39586,#39587,#39588,#39589,#39590,#39591,#39592,#39593,#39594,
#39595,#39596,#39597,#39598,#39599,#39600,#39601,#39602,#39603,#39604,#39605,
#39606,#39607,#39608,#39609,#39610,#39611,#39612,#39613,#39614,#39615,#39616,
#39617,#39618,#39619,#39620,#39621,#39622,#39623,#39624,#39625,#39626,#39627,
#39628,#39629,#39630),.UNSPECIFIED.,.F.,.F.,(4,3,3,3,3,3,3,3,3,3,3,3,3,
3,3,3,3,3,3,3,3,3,3,3,3,3,3,3,4),(-0.376940817211618,-0.354634182890013,
-0.332911763637628,-0.328063423851266,-0.305814805697609,-0.290194808594274,
-0.284256159181052,-0.27860087990661,-0.256917704097231,-0.23570018939777,
-0.214948003756356,-0.208204616608779,-0.204400619135709,-0.183824594219919,
-0.180854828870929,-0.159872080701967,-0.140296871743027,-0.135976593191014,
-0.1325994058261,-0.112140134041277,-0.0917753374355066,-0.0718467835548272,
-0.0676478648747052,-0.0636677276964501,-0.0441097307614711,-0.0249236995043246,
-0.00636086853661492,-0.00327040903044951,0.),.UNSPECIFIED.);
#3899=B_SPLINE_CURVE_WITH_KNOTS('',3,(#39632,#39633,#39634,#39635,#39636,
#39637,#39638,#39639,#39640,#39641,#39642),.UNSPECIFIED.,.F.,.F.,(4,1,1,
1,1,1,1,1,4),(15.7079632679489,15.8518654961884,16.8494368691713,17.8470082421543,
18.8445796151372,19.8421509881201,20.8397223611031,21.837293734086,21.9911485751285),
 .UNSPECIFIED.);
#3900=B_SPLINE_CURVE_WITH_KNOTS('',3,(#39643,#39644,#39645,#39646,#39647,
#39648,#39649,#39650,#39651,#39652),.UNSPECIFIED.,.F.,.F.,(4,1,1,1,1,1,
1,4),(15.7079632679489,16.3932837587428,17.3908551317257,18.3884265047086,
19.3859978776916,20.3835692506745,21.3811406236574,21.9911485751285),
 .UNSPECIFIED.);
#3901=B_SPLINE_CURVE_WITH_KNOTS('',3,(#39997,#39998,#39999,#40000,#40001,
#40002,#40003,#40004,#40005,#40006,#40007,#40008,#40009,#40010,#40011,#40012,
#40013,#40014,#40015,#40016,#40017,#40018,#40019,#40020,#40021,#40022,#40023,
#40024,#40025,#40026,#40027,#40028,#40029,#40030,#40031,#40032,#40033,#40034,
#40035,#40036,#40037,#40038,#40039,#40040,#40041,#40042,#40043,#40044,#40045,
#40046,#40047,#40048,#40049,#40050,#40051,#40052,#40053,#40054,#40055,#40056,
#40057,#40058,#40059,#40060,#40061,#40062,#40063,#40064,#40065,#40066,#40067,
#40068,#40069,#40070,#40071,#40072,#40073,#40074,#40075,#40076,#40077,#40078),
 .UNSPECIFIED.,.F.,.F.,(4,3,3,3,3,3,3,3,3,3,3,3,3,3,3,3,3,3,3,3,3,3,3,3,
3,3,3,4),(0.,0.0185976526102971,0.038423603067765,0.0557713097180495,0.0644755844468549,
0.068451628882596,0.0885059681202624,0.108915976702059,0.125988296594055,
0.133854408336341,0.137287722938539,0.15836259811627,0.177205256270041,
0.197733028930863,0.205653066409013,0.20912748618408,0.230133047566578,
0.251625243351313,0.268069199559052,0.278304581266316,0.284046628828574,
0.306315638091715,0.322971918689363,0.328167813305499,0.333183176091069,
0.355704559012681,0.372940760482309,0.376940817211655),.UNSPECIFIED.);
#3902=B_SPLINE_CURVE_WITH_KNOTS('',3,(#40079,#40080,#40081,#40082,#40083,
#40084,#40085,#40086,#40087,#40088,#40089,#40090,#40091,#40092,#40093,#40094,
#40095,#40096,#40097,#40098,#40099,#40100,#40101,#40102,#40103),
 .UNSPECIFIED.,.F.,.F.,(4,3,3,3,3,3,3,3,4),(-10.1295685708718,-9.97571372982932,
-8.97814235684639,-7.98057098386346,-6.98299961088053,-5.9854282378976,
-4.98785686491466,-3.99028549193173,-3.84638326369224),.UNSPECIFIED.);
#3903=B_SPLINE_CURVE_WITH_KNOTS('',3,(#40448,#40449,#40450,#40451,#40452,
#40453,#40454,#40455,#40456,#40457,#40458,#40459,#40460,#40461,#40462,#40463,
#40464,#40465,#40466,#40467,#40468,#40469),.UNSPECIFIED.,.F.,.F.,(4,3,3,
3,3,3,3,4),(7.59300756235153,7.98057098386346,8.97814235684639,9.97571372982932,
10.9732851028123,11.9708564757952,12.9684278487781,13.8761928695311),
 .UNSPECIFIED.);
#3904=B_SPLINE_CURVE_WITH_KNOTS('',3,(#40470,#40471,#40472,#40473,#40474,
#40475,#40476,#40477,#40478,#40479,#40480,#40481,#40482,#40483,#40484,#40485,
#40486,#40487,#40488,#40489,#40490,#40491,#40492,#40493,#40494,#40495,#40496,
#40497,#40498,#40499,#40500,#40501,#40502,#40503,#40504,#40505,#40506,#40507,
#40508,#40509,#40510,#40511,#40512,#40513,#40514,#40515,#40516,#40517,#40518,
#40519,#40520,#40521,#40522,#40523,#40524,#40525,#40526,#40527,#40528,#40529,
#40530,#40531,#40532,#40533,#40534,#40535,#40536,#40537,#40538,#40539,#40540,
#40541,#40542,#40543,#40544,#40545,#40546,#40547,#40548,#40549,#40550,#40551,
#40552,#40553,#40554),.UNSPECIFIED.,.F.,.F.,(4,3,3,3,3,3,3,3,3,3,3,3,3,
3,3,3,3,3,3,3,3,3,3,3,3,3,3,3,4),(0.,0.0219662478558776,0.0445437519028764,
0.0636212321933215,0.07209685366591,0.0767538544095747,0.0810484322391913,
0.102995052369132,0.124771335602438,0.142869400258438,0.150423566581854,
0.153920154512486,0.157567047704503,0.178337711801077,0.197163594226437,
0.219435545910495,0.224339035444425,0.229398553889566,0.250063614193726,
0.270724500169195,0.285678958575898,0.296896594122732,0.30062412117991,
0.320396425756097,0.334309228897919,0.338775005408962,0.357799813892921,
0.375339207698899,0.378621596831459),.UNSPECIFIED.);
#3905=B_SPLINE_CURVE_WITH_KNOTS('',3,(#40557,#40558,#40559,#40560,#40561,
#40562,#40563,#40564,#40565,#40566,#40567,#40568,#40569,#40570,#40571,#40572,
#40573,#40574,#40575,#40576,#40577,#40578,#40579,#40580,#40581,#40582,#40583,
#40584,#40585,#40586,#40587,#40588,#40589,#40590,#40591,#40592,#40593,#40594,
#40595,#40596,#40597,#40598,#40599,#40600,#40601,#40602,#40603,#40604,#40605,
#40606,#40607,#40608,#40609,#40610,#40611,#40612,#40613,#40614,#40615,#40616,
#40617,#40618,#40619,#40620,#40621,#40622,#40623,#40624,#40625,#40626,#40627,
#40628,#40629,#40630,#40631,#40632,#40633,#40634,#40635,#40636,#40637,#40638,
#40639,#40640,#40641,#40642,#40643,#40644),.UNSPECIFIED.,.F.,.F.,(4,3,3,
3,3,3,3,3,3,3,3,3,3,3,3,3,3,3,3,3,3,3,3,3,3,3,3,3,3,4),(-0.378621596831376,
-0.359797363526263,-0.347856611388035,-0.339691444400771,-0.335368277656519,
-0.315496143991729,-0.301162812952519,-0.297226950788673,-0.293222691569,
-0.272820243253334,-0.252122598473177,-0.239299322774394,-0.228794025865611,
-0.22450145691891,-0.203196880773058,-0.200829495678047,-0.180342164145179,
-0.158301470102644,-0.154267209525513,-0.150798043946759,-0.129414602665861,
-0.107580315103531,-0.0856137100538687,-0.0801848970193141,-0.0759382309635091,
-0.0533905919171353,-0.0308184274161136,-0.00876001820599945,-0.00401661180489279,
0.),.UNSPECIFIED.);
#3906=B_SPLINE_CURVE_WITH_KNOTS('',3,(#40645,#40646,#40647,#40648,#40649,
#40650,#40651,#40652,#40653,#40654,#40655,#40656,#40657,#40658,#40659,#40660,
#40661,#40662,#40663,#40664,#40665,#40666,#40667,#40668,#40669,#40670,#40671,
#40672,#40673,#40674,#40675,#40676,#40677,#40678,#40679,#40680,#40681,#40682,
#40683,#40684,#40685,#40686,#40687,#40688,#40689,#40690,#40691,#40692,#40693,
#40694,#40695,#40696,#40697,#40698,#40699,#40700,#40701,#40702,#40703,#40704,
#40705,#40706,#40707,#40708,#40709,#40710,#40711,#40712,#40713,#40714,#40715,
#40716,#40717,#40718,#40719,#40720,#40721,#40722,#40723,#40724,#40725,#40726,
#40727,#40728,#40729),.UNSPECIFIED.,.F.,.F.,(4,3,3,3,3,3,3,3,3,3,3,3,3,
3,3,3,3,3,3,3,3,3,3,3,3,3,3,3,4),(-0.376940817211658,-0.354634181776293,
-0.332911762663124,-0.32806342264117,-0.305814804501951,-0.290194807548075,
-0.28425615687011,-0.278600880008221,-0.256917704384274,-0.235700190161406,
-0.214948004827601,-0.20820461591444,-0.204400619278192,-0.183824594824418,
-0.180854828870941,-0.159872080703541,-0.140296871744405,-0.135976593972186,
-0.132599406442617,-0.112140134586177,-0.0917753381175245,-0.0718467848499371,
-0.0676478684587749,-0.063667728849533,-0.0441097322463572,-0.0249237017162217,
-0.00636087194527781,-0.00327040903045192,0.),.UNSPECIFIED.);
#3907=B_SPLINE_CURVE_WITH_KNOTS('',3,(#40731,#40732,#40733,#40734,#40735,
#40736,#40737,#40738,#40739,#40740,#40741),.UNSPECIFIED.,.F.,.F.,(4,1,1,
1,1,1,1,1,4),(15.7079632679489,15.8518654961884,16.8494368691713,17.8470082421543,
18.8445796151372,19.8421509881201,20.8397223611031,21.837293734086,21.9911485751285),
 .UNSPECIFIED.);
#3908=B_SPLINE_CURVE_WITH_KNOTS('',3,(#40742,#40743,#40744,#40745,#40746,
#40747,#40748,#40749,#40750,#40751),.UNSPECIFIED.,.F.,.F.,(4,1,1,1,1,1,
1,4),(15.7079632679489,16.3932837587428,17.3908551317257,18.3884265047086,
19.3859978776916,20.3835692506745,21.3811406236574,21.9911485751285),
 .UNSPECIFIED.);
#3909=B_SPLINE_CURVE_WITH_KNOTS('',3,(#41096,#41097,#41098,#41099,#41100,
#41101,#41102,#41103,#41104,#41105,#41106,#41107,#41108,#41109,#41110,#41111,
#41112,#41113,#41114,#41115,#41116,#41117,#41118,#41119,#41120,#41121,#41122,
#41123,#41124,#41125,#41126,#41127,#41128,#41129,#41130,#41131,#41132,#41133,
#41134,#41135,#41136,#41137,#41138,#41139,#41140,#41141,#41142,#41143,#41144,
#41145,#41146,#41147,#41148,#41149,#41150,#41151,#41152,#41153,#41154,#41155,
#41156,#41157,#41158,#41159,#41160,#41161,#41162,#41163,#41164,#41165,#41166,
#41167,#41168,#41169,#41170,#41171,#41172,#41173,#41174,#41175,#41176,#41177),
 .UNSPECIFIED.,.F.,.F.,(4,3,3,3,3,3,3,3,3,3,3,3,3,3,3,3,3,3,3,3,3,3,3,3,
3,3,3,4),(0.,0.0185976544397309,0.0384236046685196,0.0557713111187097,0.0644755868718208,
0.0684516295212589,0.088505970063774,0.10891597920695,0.125988298472723,
0.133854411295539,0.137287724515988,0.158362599521173,0.17720525627004,
0.197733028011595,0.205653065916169,0.209127485831402,0.230133046133618,
0.251625241350057,0.26806920002886,0.278304582355908,0.284046628542303,
0.306315637737753,0.322971918423894,0.328167812754554,0.333183175813273,
0.35570455874239,0.372940760482319,0.376940817211663),.UNSPECIFIED.);
#3910=B_SPLINE_CURVE_WITH_KNOTS('',3,(#41178,#41179,#41180,#41181,#41182,
#41183,#41184,#41185,#41186,#41187,#41188,#41189,#41190,#41191,#41192,#41193,
#41194,#41195,#41196,#41197,#41198,#41199,#41200,#41201,#41202),
 .UNSPECIFIED.,.F.,.F.,(4,3,3,3,3,3,3,3,4),(-10.1295685708718,-9.97571372982932,
-8.97814235684639,-7.98057098386346,-6.98299961088053,-5.98542823789759,
-4.98785686491466,-3.99028549193173,-3.84638326369223),.UNSPECIFIED.);
#3911=B_SPLINE_CURVE_WITH_KNOTS('',3,(#41547,#41548,#41549,#41550,#41551,
#41552,#41553,#41554,#41555,#41556,#41557,#41558,#41559,#41560,#41561,#41562,
#41563,#41564,#41565,#41566,#41567,#41568),.UNSPECIFIED.,.F.,.F.,(4,3,3,
3,3,3,3,4),(7.59300756235152,7.98057098386347,8.97814235684639,9.97571372982933,
10.9732851028123,11.9708564757952,12.9684278487781,13.8761928695311),
 .UNSPECIFIED.);
#3912=B_SPLINE_CURVE_WITH_KNOTS('',3,(#41569,#41570,#41571,#41572,#41573,
#41574,#41575,#41576,#41577,#41578,#41579,#41580,#41581,#41582,#41583,#41584,
#41585,#41586,#41587,#41588,#41589,#41590,#41591,#41592,#41593,#41594,#41595,
#41596,#41597,#41598,#41599,#41600,#41601,#41602,#41603,#41604,#41605,#41606,
#41607,#41608,#41609,#41610,#41611,#41612,#41613,#41614,#41615,#41616,#41617,
#41618,#41619,#41620,#41621,#41622,#41623,#41624,#41625,#41626,#41627,#41628,
#41629,#41630,#41631,#41632,#41633,#41634,#41635,#41636,#41637,#41638,#41639,
#41640,#41641,#41642,#41643,#41644,#41645,#41646,#41647,#41648,#41649,#41650,
#41651,#41652,#41653),.UNSPECIFIED.,.F.,.F.,(4,3,3,3,3,3,3,3,3,3,3,3,3,
3,3,3,3,3,3,3,3,3,3,3,3,3,3,3,4),(0.,0.0219662374681043,0.0445437405167695,
0.0636212222304769,0.0720968506878746,0.076753848109775,0.0810484305510295,
0.102995050890004,0.12477133726383,0.14286940150448,0.150423566044572,0.153920151202922,
0.157567046659697,0.178337713883236,0.197163594226428,0.219435545910486,
0.224339036280714,0.229398553932371,0.250063613828033,0.270724500179063,
0.28567896807331,0.296896610194788,0.300624125785386,0.320396434080511,
0.334309242700404,0.338775018539486,0.357799832913783,0.375339207698892,
0.378621596831452),.UNSPECIFIED.);
#3913=B_SPLINE_CURVE_WITH_KNOTS('',3,(#41656,#41657,#41658,#41659,#41660,
#41661,#41662,#41663,#41664,#41665,#41666,#41667,#41668,#41669,#41670,#41671,
#41672,#41673,#41674,#41675,#41676,#41677,#41678,#41679,#41680,#41681,#41682,
#41683,#41684,#41685,#41686,#41687,#41688,#41689,#41690,#41691,#41692,#41693,
#41694,#41695,#41696,#41697,#41698,#41699,#41700,#41701,#41702,#41703,#41704,
#41705,#41706,#41707,#41708,#41709,#41710,#41711,#41712,#41713,#41714,#41715,
#41716,#41717,#41718,#41719,#41720,#41721,#41722,#41723,#41724,#41725,#41726,
#41727,#41728,#41729,#41730,#41731,#41732,#41733,#41734,#41735,#41736,#41737,
#41738,#41739,#41740,#41741,#41742,#41743),.UNSPECIFIED.,.F.,.F.,(4,3,3,
3,3,3,3,3,3,3,3,3,3,3,3,3,3,3,3,3,3,3,3,3,3,3,3,3,3,4),(-0.378621596831417,
-0.359796324497287,-0.347853968212287,-0.339667381014858,-0.335354793046504,
-0.315481654145321,-0.301150134336916,-0.297197750169864,-0.293218427785562,
-0.272815226606713,-0.25211769236358,-0.239295643192204,-0.228788599050033,
-0.224499673213218,-0.203195145604267,-0.200829495678076,-0.180342878343926,
-0.158302095026546,-0.154271536503135,-0.150798918827255,-0.129416060220185,
-0.107582030156302,-0.085615429447784,-0.0801878898688665,-0.0759393010019052,
-0.0533917820942347,-0.0308195963821799,-0.00876131063080365,-0.00401661180488985,
0.),.UNSPECIFIED.);
#3914=B_SPLINE_CURVE_WITH_KNOTS('',3,(#41744,#41745,#41746,#41747,#41748,
#41749,#41750,#41751,#41752,#41753,#41754,#41755,#41756,#41757,#41758,#41759,
#41760,#41761,#41762,#41763,#41764,#41765,#41766,#41767,#41768,#41769,#41770,
#41771,#41772,#41773,#41774,#41775,#41776,#41777,#41778,#41779,#41780,#41781,
#41782,#41783,#41784,#41785,#41786,#41787,#41788,#41789,#41790,#41791,#41792,
#41793,#41794,#41795,#41796,#41797,#41798,#41799,#41800,#41801,#41802,#41803,
#41804,#41805,#41806,#41807,#41808,#41809,#41810,#41811,#41812,#41813,#41814,
#41815,#41816,#41817,#41818,#41819,#41820,#41821,#41822,#41823,#41824,#41825,
#41826,#41827,#41828),.UNSPECIFIED.,.F.,.F.,(4,3,3,3,3,3,3,3,3,3,3,3,3,
3,3,3,3,3,3,3,3,3,3,3,3,3,3,3,4),(-0.376940817211595,-0.354633525341539,
-0.332911188282713,-0.328062756081701,-0.305814149652336,-0.29019423455466,
-0.284254884688389,-0.278600964735507,-0.256917900776687,-0.235700669545305,
-0.214948669523327,-0.208204193208427,-0.204400682428168,-0.183824932405233,
-0.180854828870931,-0.15987208389359,-0.140296874535698,-0.135977073921547,
-0.132599774501717,-0.112140461891992,-0.0917757502446185,-0.0718475645954736,
-0.0676500217282804,-0.0636684046323996,-0.044110611854005,-0.0249250199568782,
-0.0063629054909037,-0.00327040903044969,0.),.UNSPECIFIED.);
#3915=B_SPLINE_CURVE_WITH_KNOTS('',3,(#41830,#41831,#41832,#41833,#41834,
#41835,#41836,#41837,#41838,#41839,#41840),.UNSPECIFIED.,.F.,.F.,(4,1,1,
1,1,1,1,1,4),(15.7079632679489,15.8518654961884,16.8494368691713,17.8470082421543,
18.8445796151372,19.8421509881201,20.8397223611031,21.837293734086,21.9911485751285),
 .UNSPECIFIED.);
#3916=B_SPLINE_CURVE_WITH_KNOTS('',3,(#41841,#41842,#41843,#41844,#41845,
#41846,#41847,#41848,#41849,#41850),.UNSPECIFIED.,.F.,.F.,(4,1,1,1,1,1,
1,4),(15.7079632679489,16.3932837587428,17.3908551317257,18.3884265047087,
19.3859978776916,20.3835692506745,21.3811406236575,21.9911485751285),
 .UNSPECIFIED.);
#3917=B_SPLINE_CURVE_WITH_KNOTS('',3,(#42195,#42196,#42197,#42198,#42199,
#42200,#42201,#42202,#42203,#42204,#42205,#42206,#42207,#42208,#42209,#42210,
#42211,#42212,#42213,#42214,#42215,#42216,#42217,#42218,#42219,#42220,#42221,
#42222,#42223,#42224,#42225,#42226,#42227,#42228,#42229,#42230,#42231,#42232,
#42233,#42234,#42235,#42236,#42237,#42238,#42239,#42240,#42241,#42242,#42243,
#42244,#42245,#42246,#42247,#42248,#42249,#42250,#42251,#42252,#42253,#42254,
#42255,#42256,#42257,#42258,#42259,#42260,#42261,#42262,#42263,#42264,#42265,
#42266,#42267,#42268,#42269,#42270,#42271,#42272,#42273,#42274,#42275,#42276),
 .UNSPECIFIED.,.F.,.F.,(4,3,3,3,3,3,3,3,3,3,3,3,3,3,3,3,3,3,3,3,3,3,3,3,
3,3,3,4),(0.,0.0185987341991705,0.0384245494580317,0.0557721378095353,0.0644770178564968,
0.0684520053950054,0.0885071145915648,0.108917452402041,0.125989403369046,
0.133856151023374,0.137288655787116,0.158363425172233,0.17720525627006,
0.197732482353245,0.205652770441454,0.209127273143543,0.230132191377097,
0.251624049744365,0.268069475041104,0.27830521821788,0.284046462285339,
0.306315432124743,0.322971764214144,0.328167478822272,0.333183009449727,
0.355704395480073,0.372940760482347,0.376940817211692),.UNSPECIFIED.);
#3918=B_SPLINE_CURVE_WITH_KNOTS('',3,(#42277,#42278,#42279,#42280,#42281,
#42282,#42283,#42284,#42285,#42286,#42287,#42288,#42289,#42290,#42291,#42292,
#42293,#42294,#42295,#42296,#42297,#42298,#42299,#42300,#42301),
 .UNSPECIFIED.,.F.,.F.,(4,3,3,3,3,3,3,3,4),(-10.1295685708718,-9.97571372982932,
-8.97814235684639,-7.98057098386346,-6.98299961088053,-5.98542823789759,
-4.98785686491466,-3.99028549193173,-3.84638326369223),.UNSPECIFIED.);
#3919=B_SPLINE_CURVE_WITH_KNOTS('',3,(#42646,#42647,#42648,#42649,#42650,
#42651,#42652,#42653,#42654,#42655,#42656,#42657,#42658,#42659,#42660,#42661,
#42662,#42663,#42664,#42665,#42666,#42667),.UNSPECIFIED.,.F.,.F.,(4,3,3,
3,3,3,3,4),(7.59300756235153,7.98057098386347,8.9781423568464,9.97571372982933,
10.9732851028123,11.9708564757952,12.9684278487781,13.8761928695311),
 .UNSPECIFIED.);
#3920=B_SPLINE_CURVE_WITH_KNOTS('',3,(#42668,#42669,#42670,#42671,#42672,
#42673,#42674,#42675,#42676,#42677,#42678,#42679,#42680,#42681,#42682,#42683,
#42684,#42685,#42686,#42687,#42688,#42689,#42690,#42691,#42692,#42693,#42694,
#42695,#42696,#42697,#42698,#42699,#42700,#42701,#42702,#42703,#42704,#42705,
#42706,#42707,#42708,#42709,#42710,#42711,#42712,#42713,#42714,#42715,#42716,
#42717,#42718,#42719,#42720,#42721,#42722,#42723,#42724,#42725,#42726,#42727,
#42728,#42729,#42730,#42731,#42732,#42733,#42734,#42735,#42736,#42737,#42738,
#42739,#42740,#42741,#42742,#42743,#42744,#42745,#42746,#42747,#42748,#42749,
#42750,#42751,#42752),.UNSPECIFIED.,.F.,.F.,(4,3,3,3,3,3,3,3,3,3,3,3,3,
3,3,3,3,3,3,3,3,3,3,3,3,3,3,3,4),(0.,0.0219671392711931,0.0445447270616514,
0.0636220854572485,0.0720971088191602,0.0767543937612894,0.0810485771086071,
0.102995177264468,0.124771188719879,0.142869290096516,0.150423609225613,
0.15392042550993,0.157567134754784,0.178337528535704,0.197163594226428,
0.219435545910483,0.224338960691668,0.229398550509701,0.250063644964382,
0.27072449500928,0.285678123754087,0.296895177895067,0.300623717144677,
0.320395694438786,0.334308019634333,0.338773858976101,0.35779815161244,
0.375339207698864,0.378621596831424),.UNSPECIFIED.);
#3921=B_SPLINE_CURVE_WITH_KNOTS('',3,(#42755,#42756,#42757,#42758,#42759,
#42760,#42761,#42762,#42763,#42764,#42765,#42766,#42767,#42768,#42769,#42770,
#42771,#42772,#42773,#42774,#42775,#42776,#42777,#42778,#42779,#42780,#42781,
#42782,#42783,#42784,#42785,#42786,#42787,#42788,#42789,#42790,#42791,#42792,
#42793,#42794,#42795,#42796,#42797,#42798,#42799,#42800,#42801,#42802,#42803,
#42804,#42805,#42806,#42807,#42808,#42809,#42810,#42811,#42812,#42813,#42814,
#42815,#42816,#42817,#42818,#42819,#42820,#42821,#42822,#42823,#42824,#42825,
#42826,#42827,#42828,#42829,#42830,#42831,#42832,#42833,#42834,#42835,#42836,
#42837,#42838,#42839,#42840,#42841,#42842),.UNSPECIFIED.,.F.,.F.,(4,3,3,
3,3,3,3,3,3,3,3,3,3,3,3,3,3,3,3,3,3,3,3,3,3,3,3,3,3,4),(-0.378621596831428,
-0.359797351570199,-0.347856580972857,-0.339691168602623,-0.335368128537906,
-0.315495983408754,-0.301162672442419,-0.297226628519414,-0.293222646087005,
-0.272820189154467,-0.25212254559016,-0.239299283112138,-0.228793967359004,
-0.224501437751794,-0.203196862127902,-0.200829495678073,-0.180342172303858,
-0.158301477241488,-0.154267258837984,-0.150798053944791,-0.129414619327559,
-0.107580334717304,-0.0856137297167705,-0.0801849312391385,-0.07593824324878,
-0.0533906055818233,-0.0308184408320373,-0.00876003298857159,-0.00401661180489581,
0.),.UNSPECIFIED.);
#3922=B_SPLINE_CURVE_WITH_KNOTS('',3,(#42843,#42844,#42845,#42846,#42847,
#42848,#42849,#42850,#42851,#42852,#42853,#42854,#42855,#42856,#42857,#42858,
#42859,#42860,#42861,#42862,#42863,#42864,#42865,#42866,#42867,#42868,#42869,
#42870,#42871,#42872,#42873,#42874,#42875,#42876,#42877,#42878,#42879,#42880,
#42881,#42882,#42883,#42884,#42885,#42886,#42887,#42888,#42889,#42890,#42891,
#42892,#42893,#42894,#42895,#42896,#42897,#42898,#42899,#42900,#42901,#42902,
#42903,#42904,#42905,#42906,#42907,#42908,#42909,#42910,#42911,#42912,#42913,
#42914,#42915,#42916,#42917,#42918,#42919,#42920,#42921,#42922,#42923,#42924,
#42925,#42926,#42927),.UNSPECIFIED.,.F.,.F.,(4,3,3,3,3,3,3,3,3,3,3,3,3,
3,3,3,3,3,3,3,3,3,3,3,3,3,3,3,4),(-0.376940817211567,-0.354634182893048,
-0.332911763640281,-0.328063423788498,-0.30581480563381,-0.290194808538448,
-0.284256159068131,-0.2786008798737,-0.256917704060186,-0.235700189361117,
-0.214948003718043,-0.208204616625186,-0.204400619173506,-0.183824594259318,
-0.180854828870914,-0.15987208070365,-0.1402968717445,-0.135976593196673,
-0.132599405819727,-0.112140134034935,-0.091775337431271,-0.0718467835475,
-0.0676478648567277,-0.0636677277271933,-0.0441097307912725,-0.0249236995322422,
-0.00636086856298682,-0.0032704090304496,0.),.UNSPECIFIED.);
#3923=B_SPLINE_CURVE_WITH_KNOTS('',3,(#42929,#42930,#42931,#42932,#42933,
#42934,#42935,#42936,#42937,#42938,#42939),.UNSPECIFIED.,.F.,.F.,(4,1,1,
1,1,1,1,1,4),(15.7079632679489,15.8518654961884,16.8494368691713,17.8470082421543,
18.8445796151372,19.8421509881201,20.8397223611031,21.837293734086,21.9911485751285),
 .UNSPECIFIED.);
#3924=B_SPLINE_CURVE_WITH_KNOTS('',3,(#42940,#42941,#42942,#42943,#42944,
#42945,#42946,#42947,#42948,#42949),.UNSPECIFIED.,.F.,.F.,(4,1,1,1,1,1,
1,4),(15.7079632679489,16.3932837587428,17.3908551317257,18.3884265047087,
19.3859978776916,20.3835692506745,21.3811406236575,21.9911485751285),
 .UNSPECIFIED.);
#3925=B_SPLINE_CURVE_WITH_KNOTS('',3,(#43294,#43295,#43296,#43297,#43298,
#43299,#43300,#43301,#43302,#43303,#43304,#43305,#43306,#43307,#43308,#43309,
#43310,#43311,#43312,#43313,#43314,#43315,#43316,#43317,#43318,#43319,#43320,
#43321,#43322,#43323,#43324,#43325,#43326,#43327,#43328,#43329,#43330,#43331,
#43332,#43333,#43334,#43335,#43336,#43337,#43338,#43339,#43340,#43341,#43342,
#43343,#43344,#43345,#43346,#43347,#43348,#43349,#43350,#43351,#43352,#43353,
#43354,#43355,#43356,#43357,#43358,#43359,#43360,#43361,#43362,#43363,#43364,
#43365,#43366,#43367,#43368,#43369,#43370,#43371,#43372,#43373,#43374,#43375),
 .UNSPECIFIED.,.F.,.F.,(4,3,3,3,3,3,3,3,3,3,3,3,3,3,3,3,3,3,3,3,3,3,3,3,
3,3,3,4),(0.,0.0185976526101627,0.038423603067645,0.055771309717942,0.0644755844464768,
0.0684516288828876,0.0885059681204507,0.108915976701888,0.125988296593921,
0.133854408336107,0.137287722941701,0.158362598119627,0.177205256270021,
0.197733028930412,0.205653066408773,0.209127486181638,0.230133047564113,
0.251625243348866,0.268069199560575,0.278304581270923,0.284046628826471,
0.306315638089425,0.322971918687632,0.32816781331511,0.333183176093119,
0.355704559014731,0.372940760482252,0.376940817211595),.UNSPECIFIED.);
#3926=B_SPLINE_CURVE_WITH_KNOTS('',3,(#43376,#43377,#43378,#43379,#43380,
#43381,#43382,#43383,#43384,#43385,#43386,#43387,#43388,#43389,#43390,#43391,
#43392,#43393,#43394,#43395,#43396,#43397,#43398,#43399,#43400),
 .UNSPECIFIED.,.F.,.F.,(4,3,3,3,3,3,3,3,4),(-10.1295685708718,-9.97571372982933,
-8.9781423568464,-7.98057098386346,-6.98299961088053,-5.9854282378976,-4.98785686491467,
-3.99028549193173,-3.84638326369224),.UNSPECIFIED.);
#3927=B_SPLINE_CURVE_WITH_KNOTS('',3,(#43745,#43746,#43747,#43748,#43749,
#43750,#43751,#43752,#43753,#43754,#43755,#43756,#43757,#43758,#43759,#43760,
#43761,#43762,#43763,#43764,#43765,#43766),.UNSPECIFIED.,.F.,.F.,(4,3,3,
3,3,3,3,4),(7.59300756235153,7.98057098386347,8.9781423568464,9.97571372982933,
10.9732851028123,11.9708564757952,12.9684278487781,13.8761928695311),
 .UNSPECIFIED.);
#3928=B_SPLINE_CURVE_WITH_KNOTS('',3,(#43767,#43768,#43769,#43770,#43771,
#43772,#43773,#43774,#43775,#43776,#43777,#43778,#43779,#43780,#43781,#43782,
#43783,#43784,#43785,#43786,#43787,#43788,#43789,#43790,#43791,#43792,#43793,
#43794,#43795,#43796,#43797,#43798,#43799,#43800,#43801,#43802,#43803,#43804,
#43805,#43806,#43807,#43808,#43809,#43810,#43811,#43812,#43813,#43814,#43815,
#43816,#43817,#43818,#43819,#43820,#43821,#43822,#43823,#43824,#43825,#43826,
#43827,#43828,#43829,#43830,#43831,#43832,#43833,#43834,#43835,#43836,#43837,
#43838,#43839,#43840,#43841,#43842,#43843,#43844,#43845,#43846,#43847,#43848,
#43849,#43850,#43851),.UNSPECIFIED.,.F.,.F.,(4,3,3,3,3,3,3,3,3,3,3,3,3,
3,3,3,3,3,3,3,3,3,3,3,3,3,3,3,4),(0.,0.021966247856033,0.0445437519030381,
0.063621232193463,0.0720968536658468,0.0767538544094051,0.0810484322397289,
0.102995052369737,0.124771335603005,0.142869400258863,0.150423566582265,
0.153920154508921,0.157567047703951,0.178337711800534,0.197163594226437,
0.219435545910494,0.224339035444409,0.229398553891155,0.250063614195313,
0.270724500170669,0.285678958579524,0.296896594129061,0.300624121181404,
0.320396425757778,0.334309228900126,0.338775005400257,0.357799813884156,
0.37533920769889,0.378621596831449),.UNSPECIFIED.);
#3929=B_SPLINE_CURVE_WITH_KNOTS('',3,(#43854,#43855,#43856,#43857,#43858,
#43859,#43860,#43861,#43862,#43863,#43864,#43865,#43866,#43867,#43868,#43869,
#43870,#43871,#43872,#43873,#43874,#43875,#43876,#43877,#43878,#43879,#43880,
#43881,#43882,#43883,#43884,#43885,#43886,#43887,#43888,#43889,#43890,#43891,
#43892,#43893,#43894,#43895,#43896,#43897,#43898,#43899,#43900,#43901,#43902,
#43903,#43904,#43905,#43906,#43907,#43908,#43909,#43910,#43911,#43912,#43913,
#43914,#43915,#43916,#43917,#43918,#43919,#43920,#43921,#43922,#43923,#43924,
#43925,#43926,#43927,#43928,#43929,#43930,#43931,#43932,#43933,#43934,#43935,
#43936,#43937,#43938,#43939,#43940,#43941),.UNSPECIFIED.,.F.,.F.,(4,3,3,
3,3,3,3,3,3,3,3,3,3,3,3,3,3,3,3,3,3,3,3,3,3,3,3,3,3,4),(-0.378621596831424,
-0.359797363524264,-0.34785661137902,-0.339691444332018,-0.335368277601998,
-0.315496143936723,-0.301162812904392,-0.297226950674736,-0.293222691552817,
-0.272820243231133,-0.252122598450948,-0.23929932275773,-0.228794025841657,
-0.224501456899104,-0.203196880753619,-0.200829495678077,-0.180342164145496,
-0.158301470102921,-0.154267209386573,-0.150798043919975,-0.129414602637409,
-0.107580315073585,-0.085613710021042,-0.0801848969680599,-0.075938230951137,
-0.0533905919055191,-0.0308184274067072,-0.00876001819588422,-0.00401661180489569,
0.),.UNSPECIFIED.);
#3930=B_SPLINE_CURVE_WITH_KNOTS('',3,(#43942,#43943,#43944,#43945,#43946,
#43947,#43948,#43949,#43950,#43951,#43952,#43953,#43954,#43955,#43956,#43957,
#43958,#43959,#43960,#43961,#43962,#43963,#43964,#43965,#43966,#43967,#43968,
#43969,#43970,#43971,#43972,#43973,#43974,#43975,#43976,#43977,#43978,#43979,
#43980,#43981,#43982,#43983,#43984,#43985,#43986,#43987,#43988,#43989,#43990,
#43991,#43992,#43993,#43994,#43995,#43996,#43997,#43998,#43999,#44000,#44001,
#44002,#44003,#44004,#44005,#44006,#44007,#44008,#44009,#44010,#44011,#44012,
#44013,#44014,#44015,#44016,#44017,#44018,#44019,#44020,#44021,#44022,#44023,
#44024,#44025,#44026),.UNSPECIFIED.,.F.,.F.,(4,3,3,3,3,3,3,3,3,3,3,3,3,
3,3,3,3,3,3,3,3,3,3,3,3,3,3,3,4),(-0.376940817211591,-0.354634181778186,
-0.332911762664777,-0.328063422667595,-0.305814804529428,-0.290194807572113,
-0.284256156918697,-0.278600880016598,-0.256917704389392,-0.235700190166293,
-0.214948004837694,-0.208204615907423,-0.204400619237651,-0.183824594781149,
-0.180854828870913,-0.15987208070781,-0.14029687174814,-0.135976593989551,
-0.13259940641991,-0.112140134563278,-0.0917753380936809,-0.0718467848234281,
-0.0676478683961129,-0.0636677288398687,-0.0441097322383243,-0.0249237017087955,
-0.0063608719337389,-0.00327040903045198,0.),.UNSPECIFIED.);
#3931=B_SPLINE_CURVE_WITH_KNOTS('',3,(#44028,#44029,#44030,#44031,#44032,
#44033,#44034,#44035,#44036,#44037,#44038),.UNSPECIFIED.,.F.,.F.,(4,1,1,
1,1,1,1,1,4),(15.7079632679489,15.8518654961884,16.8494368691713,17.8470082421543,
18.8445796151372,19.8421509881201,20.8397223611031,21.837293734086,21.9911485751285),
 .UNSPECIFIED.);
#3932=B_SPLINE_CURVE_WITH_KNOTS('',3,(#44039,#44040,#44041,#44042,#44043,
#44044,#44045,#44046,#44047,#44048),.UNSPECIFIED.,.F.,.F.,(4,1,1,1,1,1,
1,4),(15.7079632679489,16.3932837587428,17.3908551317257,18.3884265047087,
19.3859978776916,20.3835692506745,21.3811406236575,21.9911485751285),
 .UNSPECIFIED.);
#3933=B_SPLINE_CURVE_WITH_KNOTS('',3,(#44393,#44394,#44395,#44396,#44397,
#44398,#44399,#44400,#44401,#44402,#44403,#44404,#44405,#44406,#44407,#44408,
#44409,#44410,#44411,#44412,#44413,#44414,#44415,#44416,#44417,#44418,#44419,
#44420,#44421,#44422,#44423,#44424,#44425,#44426,#44427,#44428,#44429,#44430,
#44431,#44432,#44433,#44434,#44435,#44436,#44437,#44438,#44439,#44440,#44441,
#44442,#44443,#44444,#44445,#44446,#44447,#44448,#44449,#44450,#44451,#44452,
#44453,#44454,#44455,#44456,#44457,#44458,#44459,#44460,#44461,#44462,#44463,
#44464,#44465,#44466,#44467,#44468,#44469,#44470,#44471,#44472,#44473,#44474),
 .UNSPECIFIED.,.F.,.F.,(4,3,3,3,3,3,3,3,3,3,3,3,3,3,3,3,3,3,3,3,3,3,3,3,
3,3,3,4),(0.,0.0185976544398407,0.0384236046686153,0.0557713111187932,0.0644755868719157,
0.0684516295230809,0.0885059700661988,0.108915979209154,0.125988298474375,
0.133854411297929,0.137287724526441,0.158362599531486,0.177205256270038,
0.197733028011421,0.205653065916,0.20912748582868,0.230133046130665,0.251625241346934,
0.268069200030553,0.278304582359924,0.28404662854489,0.306315637741208,
0.322971918426484,0.328167812746273,0.333183175811798,0.355704558740549,
0.372940760482311,0.376940817211655),.UNSPECIFIED.);
#3934=B_SPLINE_CURVE_WITH_KNOTS('',3,(#44475,#44476,#44477,#44478,#44479,
#44480,#44481,#44482,#44483,#44484,#44485,#44486,#44487,#44488,#44489,#44490,
#44491,#44492,#44493,#44494,#44495,#44496,#44497,#44498,#44499),
 .UNSPECIFIED.,.F.,.F.,(4,3,3,3,3,3,3,3,4),(-10.1295685708718,-9.97571372982933,
-8.9781423568464,-7.98057098386346,-6.98299961088053,-5.9854282378976,-4.98785686491467,
-3.99028549193173,-3.84638326369223),.UNSPECIFIED.);
#3935=B_SPLINE_CURVE_WITH_KNOTS('',3,(#44844,#44845,#44846,#44847,#44848,
#44849,#44850,#44851,#44852,#44853,#44854,#44855,#44856,#44857,#44858,#44859,
#44860,#44861,#44862,#44863,#44864,#44865),.UNSPECIFIED.,.F.,.F.,(4,3,3,
3,3,3,3,4),(7.59300756235153,7.98057098386346,8.97814235684639,9.97571372982932,
10.9732851028123,11.9708564757952,12.9684278487781,13.8761928695311),
 .UNSPECIFIED.);
#3936=B_SPLINE_CURVE_WITH_KNOTS('',3,(#44866,#44867,#44868,#44869,#44870,
#44871,#44872,#44873,#44874,#44875,#44876,#44877,#44878,#44879,#44880,#44881,
#44882,#44883,#44884,#44885,#44886,#44887,#44888,#44889,#44890,#44891,#44892,
#44893,#44894,#44895,#44896,#44897,#44898,#44899,#44900,#44901,#44902,#44903,
#44904,#44905,#44906,#44907,#44908,#44909,#44910,#44911,#44912,#44913,#44914,
#44915,#44916,#44917,#44918,#44919,#44920,#44921,#44922,#44923,#44924,#44925,
#44926,#44927,#44928,#44929,#44930,#44931,#44932,#44933,#44934,#44935,#44936,
#44937,#44938,#44939,#44940,#44941,#44942,#44943,#44944,#44945,#44946,#44947,
#44948,#44949,#44950),.UNSPECIFIED.,.F.,.F.,(4,3,3,3,3,3,3,3,3,3,3,3,3,
3,3,3,3,3,3,3,3,3,3,3,3,3,3,3,4),(0.,0.0219662374680391,0.0445437405167158,
0.0636212222304308,0.0720968506878779,0.0767538481096382,0.081048430551138,
0.102995050890364,0.124771337264665,0.142869401505108,0.150423566045082,
0.153920151218966,0.157567046662202,0.178337713885749,0.197163594226436,
0.219435545910489,0.224339036280642,0.229398553932292,0.250063613827866,
0.270724500178625,0.285678968070037,0.296896610190914,0.30062412578472,
0.320396434080142,0.334309242699549,0.338775018538281,0.357799832912367,
0.375339207698863,0.378621596831421),.UNSPECIFIED.);
#3937=B_SPLINE_CURVE_WITH_KNOTS('',3,(#44958,#44959,#44960,#44961,#44962,
#44963,#44964,#44965,#44966,#44967,#44968,#44969,#44970,#44971,#44972,#44973,
#44974,#44975,#44976,#44977,#44978,#44979,#44980,#44981,#44982,#44983,#44984,
#44985,#44986,#44987,#44988,#44989,#44990,#44991,#44992,#44993,#44994,#44995,
#44996,#44997,#44998,#44999,#45000,#45001,#45002,#45003,#45004,#45005,#45006,
#45007,#45008,#45009,#45010,#45011,#45012,#45013,#45014,#45015,#45016,#45017,
#45018,#45019,#45020,#45021,#45022,#45023,#45024,#45025,#45026,#45027,#45028,
#45029,#45030,#45031,#45032,#45033,#45034,#45035,#45036,#45037,#45038,#45039,
#45040,#45041,#45042,#45043,#45044,#45045),.UNSPECIFIED.,.F.,.F.,(4,3,3,
3,3,3,3,3,3,3,3,3,3,3,3,3,3,3,3,3,3,3,3,3,3,3,3,3,3,4),(-0.378621596831482,
-0.359797939671017,-0.347858077335423,-0.339704706610793,-0.33537529913106,
-0.315503714728244,-0.301169437346976,-0.297242106085975,-0.293224790533046,
-0.27282275550358,-0.252125053752483,-0.239301164233888,-0.22879674266649,
-0.224502344128615,-0.203197744285114,-0.200829495678103,-0.180341772881595,
-0.158301127747009,-0.154264834760236,-0.150797561842571,-0.12941380077193,
-0.107579371162969,-0.0856127635779262,-0.0801832505987719,-0.0759376400558302,
-0.0533899343754914,-0.0308177819508918,-0.008759308379451,-0.00401661180490152,
0.),.UNSPECIFIED.);
#3938=B_SPLINE_CURVE_WITH_KNOTS('',3,(#45046,#45047,#45048,#45049,#45050,
#45051,#45052,#45053,#45054,#45055,#45056,#45057,#45058,#45059,#45060,#45061,
#45062,#45063,#45064,#45065,#45066,#45067,#45068,#45069,#45070,#45071,#45072,
#45073,#45074,#45075,#45076,#45077,#45078,#45079,#45080,#45081,#45082,#45083,
#45084,#45085,#45086,#45087,#45088,#45089,#45090,#45091,#45092,#45093,#45094,
#45095,#45096,#45097,#45098,#45099,#45100,#45101,#45102,#45103,#45104,#45105,
#45106,#45107,#45108,#45109,#45110,#45111,#45112,#45113,#45114,#45115,#45116,
#45117,#45118,#45119,#45120,#45121,#45122,#45123,#45124,#45125,#45126,#45127,
#45128,#45129,#45130),.UNSPECIFIED.,.F.,.F.,(4,3,3,3,3,3,3,3,3,3,3,3,3,
3,3,3,3,3,3,3,3,3,3,3,3,3,3,3,4),(-0.376940817211645,-0.354634583492538,
-0.332912114164838,-0.328063830062097,-0.305815206809885,-0.290195159567516,
-0.284256938553548,-0.278600828101315,-0.25691758637424,-0.23569990131557,
-0.214947604399832,-0.208204874074823,-0.204400580937649,-0.183824390832658,
-0.180854828870938,-0.159872079452346,-0.14029687064961,-0.135976312797154,
-0.132599190254655,-0.112139944657484,-0.0917751008216024,-0.0718463313280328,
-0.067646608948578,-0.0636673307706993,-0.044109215855187,-0.0249229264978586,
-0.00635967183413765,-0.0032704090304543,0.),.UNSPECIFIED.);
#3939=B_SPLINE_CURVE_WITH_KNOTS('',3,(#45132,#45133,#45134,#45135,#45136,
#45137,#45138,#45139,#45140,#45141,#45142),.UNSPECIFIED.,.F.,.F.,(4,1,1,
1,1,1,1,1,4),(15.7079632679489,15.8518654961883,16.8494368691713,17.8470082421542,
18.8445796151371,19.8421509881201,20.839722361103,21.8372937340859,21.9911485751285),
 .UNSPECIFIED.);
#3940=B_SPLINE_CURVE_WITH_KNOTS('',3,(#45143,#45144,#45145,#45146,#45147,
#45148,#45149,#45150,#45151,#45152),.UNSPECIFIED.,.F.,.F.,(4,1,1,1,1,1,
1,4),(15.7079632679489,16.3932837587427,17.3908551317257,18.3884265047086,
19.3859978776915,20.3835692506745,21.3811406236574,21.9911485751285),
 .UNSPECIFIED.);
#3941=B_SPLINE_CURVE_WITH_KNOTS('',3,(#45497,#45498,#45499,#45500,#45501,
#45502,#45503,#45504,#45505,#45506,#45507,#45508,#45509,#45510,#45511,#45512,
#45513,#45514,#45515,#45516,#45517,#45518,#45519,#45520,#45521,#45522,#45523,
#45524,#45525,#45526,#45527,#45528,#45529,#45530,#45531,#45532,#45533,#45534,
#45535,#45536,#45537,#45538,#45539,#45540,#45541,#45542,#45543,#45544,#45545,
#45546,#45547,#45548,#45549,#45550,#45551,#45552,#45553,#45554,#45555,#45556,
#45557,#45558,#45559,#45560,#45561,#45562,#45563,#45564,#45565,#45566,#45567,
#45568,#45569,#45570,#45571,#45572,#45573,#45574,#45575,#45576,#45577,#45578),
 .UNSPECIFIED.,.F.,.F.,(4,3,3,3,3,3,3,3,3,3,3,3,3,3,3,3,3,3,3,3,3,3,3,3,
3,3,3,4),(0.,0.0185969955131322,0.0384230281077451,0.0557708066280314,0.0644747133135174,
0.0684514005852745,0.0885052705827287,0.108915076403666,0.125987621370258,
0.133853344527305,0.137287156143503,0.158362091944416,0.177205256270036,
0.19773335754956,0.205653241463164,0.20912761153043,0.230133559208142,0.251625958497864,
0.268069030050869,0.27830418763456,0.284046730395759,0.306315763835364,
0.322972012997098,0.328168014027546,0.333183276135758,0.355704655810399,
0.372940760482301,0.376940817211646),.UNSPECIFIED.);
#3942=B_SPLINE_CURVE_WITH_KNOTS('',3,(#45579,#45580,#45581,#45582,#45583,
#45584,#45585,#45586,#45587,#45588,#45589,#45590,#45591,#45592,#45593,#45594,
#45595,#45596,#45597,#45598,#45599,#45600,#45601,#45602,#45603),
 .UNSPECIFIED.,.F.,.F.,(4,3,3,3,3,3,3,3,4),(-10.1295685708719,-9.97571372982932,
-8.97814235684639,-7.98057098386345,-6.98299961088052,-5.98542823789759,
-4.98785686491465,-3.99028549193172,-3.8463832636923),.UNSPECIFIED.);
#3943=B_SPLINE_CURVE_WITH_KNOTS('',3,(#45948,#45949,#45950,#45951,#45952,
#45953,#45954,#45955,#45956,#45957,#45958,#45959,#45960,#45961,#45962,#45963,
#45964,#45965,#45966,#45967,#45968,#45969),.UNSPECIFIED.,.F.,.F.,(4,3,3,
3,3,3,3,4),(7.59300756235157,7.98057098386346,8.97814235684639,9.97571372982932,
10.9732851028123,11.9708564757952,12.9684278487781,13.8761928695311),
 .UNSPECIFIED.);
#3944=B_SPLINE_CURVE_WITH_KNOTS('',3,(#45970,#45971,#45972,#45973,#45974,
#45975,#45976,#45977,#45978,#45979,#45980,#45981,#45982,#45983,#45984,#45985,
#45986,#45987,#45988,#45989,#45990,#45991,#45992,#45993,#45994,#45995,#45996,
#45997,#45998,#45999,#46000,#46001,#46002,#46003,#46004,#46005,#46006,#46007,
#46008,#46009,#46010,#46011,#46012,#46013,#46014,#46015,#46016,#46017,#46018,
#46019,#46020,#46021,#46022,#46023,#46024,#46025,#46026,#46027,#46028,#46029,
#46030,#46031,#46032,#46033,#46034,#46035,#46036,#46037,#46038,#46039,#46040,
#46041,#46042,#46043,#46044,#46045,#46046,#46047,#46048,#46049,#46050,#46051,
#46052,#46053,#46054),.UNSPECIFIED.,.F.,.F.,(4,3,3,3,3,3,3,3,3,3,3,3,3,
3,3,3,3,3,3,3,3,3,3,3,3,3,3,3,4),(0.,0.0219657370419595,0.0445431913692733,
0.0636207417264163,0.072096707092799,0.0767535441972317,0.0810483489290845,
0.102994978685481,0.124771415616641,0.142869460269085,0.150423538874486,
0.153919987844215,0.157566995524998,0.178337812740353,0.197163594226417,
0.219435545910471,0.224339075599447,0.229398555825431,0.250063595737514,
0.270724499006124,0.285679418592838,0.296897371656218,0.300624344614772,
0.320396829483506,0.334309899382154,0.338775644838224,0.357800739663862,
0.37533920769885,0.37862159683141),.UNSPECIFIED.);
#3945=B_SPLINE_CURVE_WITH_KNOTS('',3,(#46057,#46058,#46059,#46060,#46061,
#46062,#46063,#46064,#46065,#46066,#46067,#46068,#46069,#46070,#46071,#46072,
#46073,#46074,#46075,#46076,#46077,#46078,#46079,#46080,#46081,#46082,#46083,
#46084,#46085,#46086,#46087,#46088,#46089,#46090,#46091,#46092,#46093,#46094,
#46095,#46096,#46097,#46098,#46099,#46100,#46101,#46102,#46103,#46104,#46105,
#46106,#46107,#46108,#46109,#46110,#46111,#46112,#46113,#46114,#46115,#46116,
#46117,#46118,#46119,#46120,#46121,#46122,#46123,#46124,#46125,#46126,#46127,
#46128,#46129,#46130,#46131,#46132,#46133,#46134,#46135,#46136,#46137,#46138,
#46139,#46140,#46141,#46142,#46143,#46144),.UNSPECIFIED.,.F.,.F.,(4,3,3,
3,3,3,3,3,3,3,3,3,3,3,3,3,3,3,3,3,3,3,3,3,3,3,3,3,3,4),(-0.378621596831388,
-0.359797936891699,-0.347858070259707,-0.339704642744632,-0.335375265981626,
-0.315503678944408,-0.301169406036115,-0.297242034708142,-0.293224780830876,
-0.272822743809878,-0.252125042326135,-0.239301155664117,-0.228796730020428,
-0.224502340033354,-0.203197740293726,-0.200829495678066,-0.180341774760636,
-0.158301129391169,-0.15426484634161,-0.150797564195065,-0.129413804659794,
-0.107579375734867,-0.0856127681572894,-0.0801832585579418,-0.075937642934926,
-0.0533899375766034,-0.030817785094969,-0.00875931182590463,-0.0040166118048955,
0.),.UNSPECIFIED.);
#3946=B_SPLINE_CURVE_WITH_KNOTS('',3,(#46145,#46146,#46147,#46148,#46149,
#46150,#46151,#46152,#46153,#46154,#46155,#46156,#46157,#46158,#46159,#46160,
#46161,#46162,#46163,#46164,#46165,#46166,#46167,#46168,#46169,#46170,#46171,
#46172,#46173,#46174,#46175,#46176,#46177,#46178,#46179,#46180,#46181,#46182,
#46183,#46184,#46185,#46186,#46187,#46188,#46189,#46190,#46191,#46192,#46193,
#46194,#46195,#46196,#46197,#46198,#46199,#46200,#46201,#46202,#46203,#46204,
#46205,#46206,#46207,#46208,#46209,#46210,#46211,#46212,#46213,#46214,#46215,
#46216,#46217,#46218,#46219,#46220,#46221,#46222,#46223,#46224,#46225,#46226,
#46227,#46228,#46229),.UNSPECIFIED.,.F.,.F.,(4,3,3,3,3,3,3,3,3,3,3,3,3,
3,3,3,3,3,3,3,3,3,3,3,3,3,3,3,4),(-0.376940817211649,-0.354634582184037,
-0.332912113019899,-0.328063828659571,-0.305815205420689,-0.29019515835197,
-0.284256935866937,-0.27860082826073,-0.256917586745712,-0.235699902239903,
-0.214947605686915,-0.208204873234999,-0.2044005811046,-0.183824391534274,
-0.180854828870936,-0.159872079459671,-0.140296870656019,-0.135976313715434,
-0.132599191025858,-0.112139945341909,-0.0917751016524139,-0.0718463328503837,
-0.0676466131531402,-0.063667332080833,-0.0441092175415555,-0.0249229290113584,
-0.00635967571411871,-0.003270409030452,0.),.UNSPECIFIED.);
#3947=B_SPLINE_CURVE_WITH_KNOTS('',3,(#46231,#46232,#46233,#46234,#46235,
#46236,#46237,#46238,#46239,#46240,#46241),.UNSPECIFIED.,.F.,.F.,(4,1,1,
1,1,1,1,1,4),(15.7079632679489,15.8518654961883,16.8494368691713,17.8470082421542,
18.8445796151371,19.8421509881201,20.839722361103,21.8372937340859,21.9911485751285),
 .UNSPECIFIED.);
#3948=B_SPLINE_CURVE_WITH_KNOTS('',3,(#46242,#46243,#46244,#46245,#46246,
#46247,#46248,#46249,#46250,#46251),.UNSPECIFIED.,.F.,.F.,(4,1,1,1,1,1,
1,4),(15.7079632679489,16.3932837587427,17.3908551317257,18.3884265047086,
19.3859978776915,20.3835692506745,21.3811406236574,21.9911485751285),
 .UNSPECIFIED.);
#3949=B_SPLINE_CURVE_WITH_KNOTS('',3,(#46596,#46597,#46598,#46599,#46600,
#46601,#46602,#46603,#46604,#46605,#46606,#46607,#46608,#46609,#46610,#46611,
#46612,#46613,#46614,#46615,#46616,#46617,#46618,#46619,#46620,#46621,#46622,
#46623,#46624,#46625,#46626,#46627,#46628,#46629,#46630,#46631,#46632,#46633,
#46634,#46635,#46636,#46637,#46638,#46639,#46640,#46641,#46642,#46643,#46644,
#46645,#46646,#46647,#46648,#46649,#46650,#46651,#46652,#46653,#46654,#46655,
#46656,#46657,#46658,#46659,#46660,#46661,#46662,#46663,#46664,#46665,#46666,
#46667,#46668,#46669,#46670,#46671,#46672,#46673,#46674,#46675,#46676,#46677),
 .UNSPECIFIED.,.F.,.F.,(4,3,3,3,3,3,3,3,3,3,3,3,3,3,3,3,3,3,3,3,3,3,3,3,
3,3,3,4),(0.,0.0185969976548629,0.0384230299817592,0.0557708082677935,0.0644747161532653,
0.0684514013184625,0.0885052728468933,0.108915079332587,0.125987623566949,
0.133853347989331,0.137287157984682,0.158362093592479,0.177205256270033,
0.197733356483111,0.205653240898836,0.209127611126219,0.230133557550482,
0.251625956178859,0.26806903060611,0.278304188926851,0.28404673006319,0.30631576342394,
0.322972012688533,0.328168013360337,0.33318327580766,0.35570465549395,0.372940760482311,
0.376940817211655),.UNSPECIFIED.);
#3950=B_SPLINE_CURVE_WITH_KNOTS('',3,(#46678,#46679,#46680,#46681,#46682,
#46683,#46684,#46685,#46686,#46687,#46688,#46689,#46690,#46691,#46692,#46693,
#46694,#46695,#46696,#46697,#46698,#46699,#46700,#46701,#46702),
 .UNSPECIFIED.,.F.,.F.,(4,3,3,3,3,3,3,3,4),(-10.1295685708719,-9.97571372982933,
-8.97814235684639,-7.98057098386346,-6.98299961088053,-5.9854282378976,
-4.98785686491466,-3.99028549193173,-3.8463832636923),.UNSPECIFIED.);
#3951=B_SPLINE_CURVE_WITH_KNOTS('',3,(#47047,#47048,#47049,#47050,#47051,
#47052,#47053,#47054,#47055,#47056,#47057,#47058,#47059,#47060,#47061,#47062,
#47063,#47064,#47065,#47066,#47067,#47068),.UNSPECIFIED.,.F.,.F.,(4,3,3,
3,3,3,3,4),(7.59300756235157,7.98057098386346,8.97814235684639,9.97571372982933,
10.9732851028123,11.9708564757952,12.9684278487781,13.8761928695312),
 .UNSPECIFIED.);
#3952=B_SPLINE_CURVE_WITH_KNOTS('',3,(#47069,#47070,#47071,#47072,#47073,
#47074,#47075,#47076,#47077,#47078,#47079,#47080,#47081,#47082,#47083,#47084,
#47085,#47086,#47087,#47088,#47089,#47090,#47091,#47092,#47093,#47094,#47095,
#47096,#47097,#47098,#47099,#47100,#47101,#47102,#47103,#47104,#47105,#47106,
#47107,#47108,#47109,#47110,#47111,#47112,#47113,#47114,#47115,#47116,#47117,
#47118,#47119,#47120,#47121,#47122,#47123,#47124,#47125,#47126,#47127,#47128,
#47129,#47130,#47131,#47132,#47133,#47134,#47135,#47136,#47137,#47138,#47139,
#47140,#47141,#47142,#47143,#47144,#47145,#47146,#47147,#47148,#47149,#47150,
#47151,#47152,#47153),.UNSPECIFIED.,.F.,.F.,(4,3,3,3,3,3,3,3,3,3,3,3,3,
3,3,3,3,3,3,3,3,3,3,3,3,3,3,3,4),(0.,0.021965739453955,0.0445431940190658,
0.0636207440449849,0.0720967077854655,0.0767535456635768,0.0810483493206851,
0.102994979034739,0.124771415243574,0.142869459989285,0.150423539009583,
0.1539199886521,0.157566995775498,0.178337812271127,0.197163594226419,0.219435545910471,
0.2243390754146,0.229398555820982,0.250063595830876,0.270724499023616,0.285679416466335,
0.296897368065093,0.300624343578509,0.320396827608135,0.334309896261688,
0.338775641864317,0.357800735353592,0.37533920769884,0.378621596831401),
 .UNSPECIFIED.);
#3953=B_SPLINE_CURVE_WITH_KNOTS('',3,(#47156,#47157,#47158,#47159,#47160,
#47161,#47162,#47163,#47164,#47165,#47166,#47167,#47168,#47169,#47170,#47171,
#47172,#47173,#47174,#47175,#47176,#47177,#47178,#47179,#47180,#47181,#47182,
#47183,#47184,#47185,#47186,#47187,#47188,#47189,#47190,#47191,#47192,#47193,
#47194,#47195,#47196,#47197,#47198,#47199,#47200,#47201,#47202,#47203,#47204,
#47205,#47206,#47207,#47208,#47209,#47210,#47211,#47212,#47213,#47214,#47215,
#47216,#47217,#47218,#47219,#47220,#47221,#47222,#47223,#47224,#47225,#47226,
#47227,#47228,#47229,#47230,#47231,#47232,#47233,#47234,#47235,#47236,#47237,
#47238,#47239,#47240,#47241,#47242,#47243),.UNSPECIFIED.,.F.,.F.,(4,3,3,
3,3,3,3,3,3,3,3,3,3,3,3,3,3,3,3,3,3,3,3,3,3,3,3,3,3,4),(-0.378621596831452,
-0.359796964371007,-0.347855595893935,-0.3396822224573,-0.335363223682036,
-0.315490706099021,-0.301158054796405,-0.297216022503385,-0.293221129613966,
-0.272818393289542,-0.252120789784161,-0.239297966257643,-0.22879202499115,
-0.224500801126252,-0.203196242755057,-0.200829495678088,-0.18034243723251,
-0.158301709054058,-0.154268865136119,-0.150798379245078,-0.129415160921567,
-0.10758097209064,-0.0856143687498464,-0.0801860432915195,-0.0759386414271447,
-0.0533910485483734,-0.0308188758174934,-0.00876051290910059,-0.0040166118048957,
0.),.UNSPECIFIED.);
#3954=B_SPLINE_CURVE_WITH_KNOTS('',3,(#47244,#47245,#47246,#47247,#47248,
#47249,#47250,#47251,#47252,#47253,#47254,#47255,#47256,#47257,#47258,#47259,
#47260,#47261,#47262,#47263,#47264,#47265,#47266,#47267,#47268,#47269,#47270,
#47271,#47272,#47273,#47274,#47275,#47276,#47277,#47278,#47279,#47280,#47281,
#47282,#47283,#47284,#47285,#47286,#47287,#47288,#47289,#47290,#47291,#47292,
#47293,#47294,#47295,#47296,#47297,#47298,#47299,#47300,#47301,#47302,#47303,
#47304,#47305,#47306,#47307,#47308,#47309,#47310,#47311,#47312,#47313,#47314,
#47315,#47316,#47317,#47318,#47319,#47320,#47321,#47322,#47323,#47324,#47325,
#47326,#47327,#47328),.UNSPECIFIED.,.F.,.F.,(4,3,3,3,3,3,3,3,3,3,3,3,3,
3,3,3,3,3,3,3,3,3,3,3,3,3,3,3,4),(-0.376940817211631,-0.35463396460261,
-0.332911572636152,-0.328063202289398,-0.305814587568867,-0.290194617731627,
-0.28425573539935,-0.278600908076312,-0.2569177688984,-0.235700347785391,
-0.214948223363317,-0.208204476166349,-0.20440064004034,-0.183824705876023,
-0.180854828870946,-0.159872081610939,-0.140296872538378,-0.13597675000539,
-0.132599526202686,-0.112140240570565,-0.0917754711453113,-0.0718470375330435,
-0.0676485678532571,-0.0636679489962621,-0.0441100183864258,-0.0249241308188154,
-0.0063615348116712,-0.00327040903045197,0.),.UNSPECIFIED.);
#3955=B_SPLINE_CURVE_WITH_KNOTS('',3,(#47330,#47331,#47332,#47333,#47334,
#47335,#47336,#47337,#47338,#47339,#47340),.UNSPECIFIED.,.F.,.F.,(4,1,1,
1,1,1,1,1,4),(15.7079632679489,15.8518654961884,16.8494368691713,17.8470082421542,
18.8445796151372,19.8421509881201,20.839722361103,21.837293734086,21.9911485751285),
 .UNSPECIFIED.);
#3956=B_SPLINE_CURVE_WITH_KNOTS('',3,(#47341,#47342,#47343,#47344,#47345,
#47346,#47347,#47348,#47349,#47350),.UNSPECIFIED.,.F.,.F.,(4,1,1,1,1,1,
1,4),(15.7079632679489,16.3932837587428,17.3908551317257,18.3884265047086,
19.3859978776916,20.3835692506745,21.3811406236574,21.9911485751285),
 .UNSPECIFIED.);
#3957=B_SPLINE_CURVE_WITH_KNOTS('',3,(#47695,#47696,#47697,#47698,#47699,
#47700,#47701,#47702,#47703,#47704,#47705,#47706,#47707,#47708,#47709,#47710,
#47711,#47712,#47713,#47714,#47715,#47716,#47717,#47718,#47719,#47720,#47721,
#47722,#47723,#47724,#47725,#47726,#47727,#47728,#47729,#47730,#47731,#47732,
#47733,#47734,#47735,#47736,#47737,#47738,#47739,#47740,#47741,#47742,#47743,
#47744,#47745,#47746,#47747,#47748,#47749,#47750,#47751,#47752,#47753,#47754,
#47755,#47756,#47757,#47758,#47759,#47760,#47761,#47762,#47763,#47764,#47765,
#47766,#47767,#47768,#47769,#47770,#47771,#47772,#47773,#47774,#47775,#47776),
 .UNSPECIFIED.,.F.,.F.,(4,3,3,3,3,3,3,3,3,3,3,3,3,3,3,3,3,3,3,3,3,3,3,3,
3,3,3,4),(0.,0.0185980112514911,0.038423916878807,0.0557715843027085,0.0644760598123438,
0.0684517536303943,0.0885063485075443,0.10891646687441,0.125988664223312,
0.133854987331634,0.137288032273647,0.158362873189272,0.177205256270019,
0.197732848455495,0.20565296933075,0.209127416437683,0.230132765546023,
0.251624849770108,0.268069291425062,0.278304794066786,0.28404657349794,
0.306315569631616,0.322971867344282,0.328167702944214,0.333183121096512,
0.35570450535538,0.372940760482276,0.37694081721162),.UNSPECIFIED.);
#3958=B_SPLINE_CURVE_WITH_KNOTS('',3,(#47777,#47778,#47779,#47780,#47781,
#47782,#47783,#47784,#47785,#47786,#47787,#47788,#47789,#47790,#47791,#47792,
#47793,#47794,#47795,#47796,#47797,#47798,#47799,#47800,#47801),
 .UNSPECIFIED.,.F.,.F.,(4,3,3,3,3,3,3,3,4),(-10.1295685708719,-9.97571372982933,
-8.97814235684639,-7.98057098386346,-6.98299961088053,-5.9854282378976,
-4.98785686491466,-3.99028549193173,-3.84638326369226),.UNSPECIFIED.);
#3959=B_SPLINE_CURVE_WITH_KNOTS('',3,(#48146,#48147,#48148,#48149,#48150,
#48151,#48152,#48153,#48154,#48155,#48156,#48157,#48158,#48159,#48160,#48161,
#48162,#48163,#48164,#48165,#48166,#48167),.UNSPECIFIED.,.F.,.F.,(4,3,3,
3,3,3,3,4),(7.59300756235153,7.98057098386346,8.97814235684639,9.97571372982933,
10.9732851028123,11.9708564757952,12.9684278487781,13.8761928695311),
 .UNSPECIFIED.);
#3960=B_SPLINE_CURVE_WITH_KNOTS('',3,(#48168,#48169,#48170,#48171,#48172,
#48173,#48174,#48175,#48176,#48177,#48178,#48179,#48180,#48181,#48182,#48183,
#48184,#48185,#48186,#48187,#48188,#48189,#48190,#48191,#48192,#48193,#48194,
#48195,#48196,#48197,#48198,#48199,#48200,#48201,#48202,#48203,#48204,#48205,
#48206,#48207,#48208,#48209,#48210,#48211,#48212,#48213,#48214,#48215,#48216,
#48217,#48218,#48219,#48220,#48221,#48222,#48223,#48224,#48225,#48226,#48227,
#48228,#48229,#48230,#48231,#48232,#48233,#48234,#48235,#48236,#48237,#48238,
#48239,#48240,#48241,#48242,#48243,#48244,#48245,#48246,#48247,#48248,#48249,
#48250,#48251,#48252),.UNSPECIFIED.,.F.,.F.,(4,3,3,3,3,3,3,3,3,3,3,3,3,
3,3,3,3,3,3,3,3,3,3,3,3,3,3,3,4),(0.,0.0219665840178867,0.0445441200922607,
0.0636215543590298,0.0720969499798807,0.0767540580968768,0.0810484869492208,
0.102995100015702,0.124771281281709,0.142869359517885,0.150423583504265,
0.153920259627952,0.157567081121822,0.178337643732188,0.197163594226413,
0.21943554591047,0.224339007945502,0.229398552615548,0.250063626007469,
0.270724499289659,0.285678648504219,0.296896068874714,0.300623970906574,
0.320396153948268,0.334308778690984,0.338774577578954,0.357799193940268,
0.375339207698864,0.378621596831425),.UNSPECIFIED.);
#3961=B_SPLINE_CURVE_WITH_KNOTS('',3,(#48255,#48256,#48257,#48258,#48259,
#48260,#48261,#48262,#48263,#48264,#48265,#48266,#48267,#48268,#48269,#48270,
#48271,#48272,#48273,#48274,#48275,#48276,#48277,#48278,#48279,#48280,#48281,
#48282,#48283,#48284,#48285,#48286,#48287,#48288,#48289,#48290,#48291,#48292,
#48293,#48294,#48295,#48296,#48297,#48298,#48299,#48300,#48301,#48302,#48303,
#48304,#48305,#48306,#48307,#48308,#48309,#48310,#48311,#48312,#48313,#48314,
#48315,#48316,#48317,#48318,#48319,#48320,#48321,#48322,#48323,#48324,#48325,
#48326,#48327,#48328,#48329,#48330,#48331,#48332,#48333,#48334,#48335,#48336,
#48337,#48338,#48339,#48340,#48341,#48342),.UNSPECIFIED.,.F.,.F.,(4,3,3,
3,3,3,3,3,3,3,3,3,3,3,3,3,3,3,3,3,3,3,3,3,3,3,3,3,3,4),(-0.378621596831355,
-0.359797939668059,-0.347858077317233,-0.339704706466932,-0.335375299042539,
-0.315503714637518,-0.301169437267586,-0.297242105936665,-0.293224790512653,
-0.272822755477615,-0.252125053726975,-0.239301164214745,-0.228796742638415,
-0.224502344135147,-0.203197744287783,-0.200829495678057,-0.180341772881768,
-0.158301127747159,-0.154264834896697,-0.150797561869219,-0.129413800799564,
-0.107579371191749,-0.0856127636019974,-0.080183250637186,-0.0759376400731541,
-0.0533899343934191,-0.0308177819684862,-0.00875930839909695,-0.00401661180489583,
0.),.UNSPECIFIED.);
#3962=B_SPLINE_CURVE_WITH_KNOTS('',3,(#48343,#48344,#48345,#48346,#48347,
#48348,#48349,#48350,#48351,#48352,#48353,#48354,#48355,#48356,#48357,#48358,
#48359,#48360,#48361,#48362,#48363,#48364,#48365,#48366,#48367,#48368,#48369,
#48370,#48371,#48372,#48373,#48374,#48375,#48376,#48377,#48378,#48379,#48380,
#48381,#48382,#48383,#48384,#48385,#48386,#48387,#48388,#48389,#48390,#48391,
#48392,#48393,#48394,#48395,#48396,#48397,#48398,#48399,#48400,#48401,#48402,
#48403,#48404,#48405,#48406,#48407,#48408,#48409,#48410,#48411,#48412,#48413,
#48414,#48415,#48416,#48417,#48418,#48419,#48420,#48421,#48422,#48423,#48424,
#48425,#48426,#48427),.UNSPECIFIED.,.F.,.F.,(4,3,3,3,3,3,3,3,3,3,3,3,3,
3,3,3,3,3,3,3,3,3,3,3,3,3,3,3,4),(-0.376940817211684,-0.35463458349161,
-0.332912114164028,-0.328063829993201,-0.305815206742055,-0.290195159508168,
-0.284256938433436,-0.278600828085135,-0.256917586360118,-0.23569990130069,
-0.214947604386309,-0.208204874079122,-0.204400580976051,-0.183824390870239,
-0.180854828870958,-0.159872079452921,-0.140296870650113,-0.135976312799136,
-0.132599190292493,-0.112139944695331,-0.091775100858925,-0.0718463313651108,
-0.0676466090368204,-0.0636673307830578,-0.0441092158685665,-0.0249229265103377,
-0.00635967184351045,-0.00327040903045443,0.),.UNSPECIFIED.);
#3963=B_SPLINE_CURVE_WITH_KNOTS('',3,(#48429,#48430,#48431,#48432,#48433,
#48434,#48435,#48436,#48437,#48438,#48439),.UNSPECIFIED.,.F.,.F.,(4,1,1,
1,1,1,1,1,4),(15.7079632679489,15.8518654961883,16.8494368691713,17.8470082421542,
18.8445796151371,19.8421509881201,20.839722361103,21.8372937340859,21.9911485751285),
 .UNSPECIFIED.);
#3964=B_SPLINE_CURVE_WITH_KNOTS('',3,(#48440,#48441,#48442,#48443,#48444,
#48445,#48446,#48447,#48448,#48449),.UNSPECIFIED.,.F.,.F.,(4,1,1,1,1,1,
1,4),(15.7079632679489,16.3932837587427,17.3908551317257,18.3884265047086,
19.3859978776915,20.3835692506745,21.3811406236574,21.9911485751285),
 .UNSPECIFIED.);
#3965=B_SPLINE_CURVE_WITH_KNOTS('',3,(#48794,#48795,#48796,#48797,#48798,
#48799,#48800,#48801,#48802,#48803,#48804,#48805,#48806,#48807,#48808,#48809,
#48810,#48811,#48812,#48813,#48814,#48815,#48816,#48817,#48818,#48819,#48820,
#48821,#48822,#48823,#48824,#48825,#48826,#48827,#48828,#48829,#48830,#48831,
#48832,#48833,#48834,#48835,#48836,#48837,#48838,#48839,#48840,#48841,#48842,
#48843,#48844,#48845,#48846,#48847,#48848,#48849,#48850,#48851,#48852,#48853,
#48854,#48855,#48856,#48857,#48858,#48859,#48860,#48861,#48862,#48863,#48864,
#48865,#48866,#48867,#48868,#48869,#48870,#48871,#48872,#48873,#48874,#48875),
 .UNSPECIFIED.,.F.,.F.,(4,3,3,3,3,3,3,3,3,3,3,3,3,3,3,3,3,3,3,3,3,3,3,3,
3,3,3,4),(0.,0.018596995512751,0.0384230281074114,0.0557708066277392,0.0644747133130811,
0.0684514005740294,0.088505270571274,0.108915076392686,0.125987621362023,
0.133853344514643,0.137287156136604,0.158362091937476,0.177205256270034,
0.197733357549519,0.205653241463143,0.209127611534079,0.230133559211876,
0.251625958501743,0.268069030048616,0.278304187628649,0.284046730391058,
0.306315763830865,0.322972012993724,0.328168014023333,0.33318327613479,
0.355704655809054,0.3729407604823,0.376940817211644),.UNSPECIFIED.);
#3966=B_SPLINE_CURVE_WITH_KNOTS('',3,(#48876,#48877,#48878,#48879,#48880,
#48881,#48882,#48883,#48884,#48885,#48886,#48887,#48888,#48889,#48890,#48891,
#48892,#48893,#48894,#48895,#48896,#48897,#48898,#48899,#48900),
 .UNSPECIFIED.,.F.,.F.,(4,3,3,3,3,3,3,3,4),(-10.1295685708719,-9.97571372982932,
-8.97814235684639,-7.98057098386345,-6.98299961088052,-5.98542823789759,
-4.98785686491466,-3.99028549193172,-3.8463832636923),.UNSPECIFIED.);
#3967=B_SPLINE_CURVE_WITH_KNOTS('',3,(#49245,#49246,#49247,#49248,#49249,
#49250,#49251,#49252,#49253,#49254,#49255,#49256,#49257,#49258,#49259,#49260,
#49261,#49262,#49263,#49264,#49265,#49266),.UNSPECIFIED.,.F.,.F.,(4,3,3,
3,3,3,3,4),(7.59300756235157,7.98057098386346,8.97814235684639,9.97571372982933,
10.9732851028123,11.9708564757952,12.9684278487781,13.8761928695312),
 .UNSPECIFIED.);
#3968=B_SPLINE_CURVE_WITH_KNOTS('',3,(#49267,#49268,#49269,#49270,#49271,
#49272,#49273,#49274,#49275,#49276,#49277,#49278,#49279,#49280,#49281,#49282,
#49283,#49284,#49285,#49286,#49287,#49288,#49289,#49290,#49291,#49292,#49293,
#49294,#49295,#49296,#49297,#49298,#49299,#49300,#49301,#49302,#49303,#49304,
#49305,#49306,#49307,#49308,#49309,#49310,#49311,#49312,#49313,#49314,#49315,
#49316,#49317,#49318,#49319,#49320,#49321,#49322,#49323,#49324,#49325,#49326,
#49327,#49328,#49329,#49330,#49331,#49332,#49333,#49334,#49335,#49336,#49337,
#49338,#49339,#49340,#49341,#49342,#49343,#49344,#49345,#49346,#49347,#49348,
#49349,#49350,#49351),.UNSPECIFIED.,.F.,.F.,(4,3,3,3,3,3,3,3,3,3,3,3,3,
3,3,3,3,3,3,3,3,3,3,3,3,3,3,3,4),(0.,0.0219657370421621,0.0445431913694635,
0.0636207417265848,0.0720967070927941,0.0767535441972933,0.0810483489287806,
0.10299497868505,0.124771415616059,0.142869460268653,0.15042353887417,0.15391998785172,
0.157566995526094,0.17833781274149,0.197163594226434,0.219435545910493,
0.224339075599542,0.229398555827627,0.250063595739872,0.270724499008654,
0.285679418600401,0.296897371668684,0.300624344617424,0.320396829485849,
0.334309899384856,0.338775644842177,0.357800739667655,0.375339207698901,
0.378621596831463),.UNSPECIFIED.);
#3969=B_SPLINE_CURVE_WITH_KNOTS('',3,(#49354,#49355,#49356,#49357,#49358,
#49359,#49360,#49361,#49362,#49363,#49364,#49365,#49366,#49367,#49368,#49369,
#49370,#49371,#49372,#49373,#49374,#49375,#49376,#49377,#49378,#49379,#49380,
#49381,#49382,#49383,#49384,#49385,#49386,#49387,#49388,#49389,#49390,#49391,
#49392,#49393,#49394,#49395,#49396,#49397,#49398,#49399,#49400,#49401,#49402,
#49403,#49404,#49405,#49406,#49407,#49408,#49409,#49410,#49411,#49412,#49413,
#49414,#49415,#49416,#49417,#49418,#49419,#49420,#49421,#49422,#49423,#49424,
#49425,#49426,#49427,#49428,#49429,#49430,#49431,#49432,#49433,#49434,#49435,
#49436,#49437,#49438,#49439,#49440,#49441),.UNSPECIFIED.,.F.,.F.,(4,3,3,
3,3,3,3,3,3,3,3,3,3,3,3,3,3,3,3,3,3,3,3,3,3,3,3,3,3,4),(-0.378621596831419,
-0.359797936894149,-0.347858070276125,-0.339704642905692,-0.335375266132442,
-0.315503679098809,-0.301169406171218,-0.297242034943752,-0.293224780862376,
-0.272822743843532,-0.252125042359958,-0.239301155689489,-0.228796730058329,
-0.224502340016174,-0.203197740281884,-0.200829495678081,-0.180341774760402,
-0.158301129390964,-0.154264846295692,-0.150797564186461,-0.129413804651141,
-0.107579375726104,-0.085612768153713,-0.0801832585527506,-0.0759376429114784,
-0.0533899375499779,-0.0308177850670804,-0.0087593118006187,-0.0040166118048958,
0.),.UNSPECIFIED.);
#3970=B_SPLINE_CURVE_WITH_KNOTS('',3,(#49442,#49443,#49444,#49445,#49446,
#49447,#49448,#49449,#49450,#49451,#49452,#49453,#49454,#49455,#49456,#49457,
#49458,#49459,#49460,#49461,#49462,#49463,#49464,#49465,#49466,#49467,#49468,
#49469,#49470,#49471,#49472,#49473,#49474,#49475,#49476,#49477,#49478,#49479,
#49480,#49481,#49482,#49483,#49484,#49485,#49486,#49487,#49488,#49489,#49490,
#49491,#49492,#49493,#49494,#49495,#49496,#49497,#49498,#49499,#49500,#49501,
#49502,#49503,#49504,#49505,#49506,#49507,#49508,#49509,#49510,#49511,#49512,
#49513,#49514,#49515,#49516,#49517,#49518,#49519,#49520,#49521,#49522,#49523,
#49524,#49525,#49526),.UNSPECIFIED.,.F.,.F.,(4,3,3,3,3,3,3,3,3,3,3,3,3,
3,3,3,3,3,3,3,3,3,3,3,3,3,3,3,4),(-0.376940817211647,-0.354634582187994,
-0.332912113023362,-0.328063828673689,-0.305815205437262,-0.290195158366472,
-0.284256935896806,-0.2786008282367,-0.256917586723634,-0.235699902217931,
-0.214947605661536,-0.208204873247512,-0.204400581023048,-0.183824391454496,
-0.180854828870938,-0.159872079456263,-0.140296870653037,-0.135976313701251,
-0.132599190986633,-0.112139945302261,-0.0917751016125585,-0.0718463328109456,
-0.0676466130607016,-0.0636673320630382,-0.0441092175240187,-0.0249229289937617,
-0.00635967569699575,-0.00327040903045435,0.),.UNSPECIFIED.);
#3971=B_SPLINE_CURVE_WITH_KNOTS('',3,(#49528,#49529,#49530,#49531,#49532,
#49533,#49534,#49535,#49536,#49537,#49538),.UNSPECIFIED.,.F.,.F.,(4,1,1,
1,1,1,1,1,4),(15.7079632679489,15.8518654961883,16.8494368691713,17.8470082421542,
18.8445796151371,19.8421509881201,20.839722361103,21.8372937340859,21.9911485751285),
 .UNSPECIFIED.);
#3972=B_SPLINE_CURVE_WITH_KNOTS('',3,(#49539,#49540,#49541,#49542,#49543,
#49544,#49545,#49546,#49547,#49548),.UNSPECIFIED.,.F.,.F.,(4,1,1,1,1,1,
1,4),(15.7079632679489,16.3932837587427,17.3908551317257,18.3884265047086,
19.3859978776915,20.3835692506745,21.3811406236574,21.9911485751285),
 .UNSPECIFIED.);
#3973=B_SPLINE_CURVE_WITH_KNOTS('',3,(#49893,#49894,#49895,#49896,#49897,
#49898,#49899,#49900,#49901,#49902,#49903,#49904,#49905,#49906,#49907,#49908,
#49909,#49910,#49911,#49912,#49913,#49914,#49915,#49916,#49917,#49918,#49919,
#49920,#49921,#49922,#49923,#49924,#49925,#49926,#49927,#49928,#49929,#49930,
#49931,#49932,#49933,#49934,#49935,#49936,#49937,#49938,#49939,#49940,#49941,
#49942,#49943,#49944,#49945,#49946,#49947,#49948,#49949,#49950,#49951,#49952,
#49953,#49954,#49955,#49956,#49957,#49958,#49959,#49960,#49961,#49962,#49963,
#49964,#49965,#49966,#49967,#49968,#49969,#49970,#49971,#49972,#49973,#49974),
 .UNSPECIFIED.,.F.,.F.,(4,3,3,3,3,3,3,3,3,3,3,3,3,3,3,3,3,3,3,3,3,3,3,3,
3,3,3,4),(0.,0.0185969976546447,0.0384230299815686,0.0557708082676271,0.0644747161530116,
0.0684514013219826,0.0885052728499997,0.108915079335808,0.125987623569365,
0.133853347992972,0.13728715798927,0.158362093597067,0.177205256270036,
0.197733356483041,0.205653240898805,0.209127611124312,0.23013355754844,
0.251625956176866,0.268069030607125,0.278304188929636,0.284046730059679,
0.306315763420324,0.322972012685815,0.328168013379916,0.333183275811836,
0.355704655498454,0.372940760482288,0.376940817211632),.UNSPECIFIED.);
#3974=B_SPLINE_CURVE_WITH_KNOTS('',3,(#49975,#49976,#49977,#49978,#49979,
#49980,#49981,#49982,#49983,#49984,#49985,#49986,#49987,#49988,#49989,#49990,
#49991,#49992,#49993,#49994,#49995,#49996,#49997,#49998,#49999),
 .UNSPECIFIED.,.F.,.F.,(4,3,3,3,3,3,3,3,4),(-10.1295685708719,-9.97571372982932,
-8.97814235684639,-7.98057098386346,-6.98299961088053,-5.9854282378976,
-4.98785686491466,-3.99028549193173,-3.8463832636923),.UNSPECIFIED.);
#3975=B_SPLINE_CURVE_WITH_KNOTS('',3,(#50344,#50345,#50346,#50347,#50348,
#50349,#50350,#50351,#50352,#50353,#50354,#50355,#50356,#50357,#50358,#50359,
#50360,#50361,#50362,#50363,#50364,#50365),.UNSPECIFIED.,.F.,.F.,(4,3,3,
3,3,3,3,4),(7.59300756235161,7.98057098386346,8.97814235684639,9.97571372982932,
10.9732851028123,11.9708564757952,12.9684278487781,13.8761928695312),
 .UNSPECIFIED.);
#3976=B_SPLINE_CURVE_WITH_KNOTS('',3,(#50366,#50367,#50368,#50369,#50370,
#50371,#50372,#50373,#50374,#50375,#50376,#50377,#50378,#50379,#50380,#50381,
#50382,#50383,#50384,#50385,#50386,#50387,#50388,#50389,#50390,#50391,#50392,
#50393,#50394,#50395,#50396,#50397,#50398,#50399,#50400,#50401,#50402,#50403,
#50404,#50405,#50406,#50407,#50408,#50409,#50410,#50411,#50412,#50413,#50414,
#50415,#50416,#50417,#50418,#50419,#50420,#50421,#50422,#50423,#50424,#50425,
#50426,#50427,#50428,#50429,#50430,#50431,#50432,#50433,#50434,#50435,#50436,
#50437,#50438,#50439,#50440,#50441,#50442,#50443,#50444,#50445,#50446,#50447,
#50448,#50449,#50450),.UNSPECIFIED.,.F.,.F.,(4,3,3,3,3,3,3,3,3,3,3,3,3,
3,3,3,3,3,3,3,3,3,3,3,3,3,3,3,4),(0.,0.0219657394536776,0.0445431940187976,
0.0636207440447494,0.0720967077855105,0.0767535456638122,0.0810483493275398,
0.102994979041479,0.124771415249923,0.142869459994045,0.150423539013126,
0.153919988666253,0.15756699577772,0.178337812273338,0.197163594226412,
0.219435545910467,0.224339075414555,0.229398555814321,0.250063595824097,
0.270724499016863,0.285679416448513,0.296897368037468,0.300624343572328,
0.320396827601905,0.334309896252106,0.338775641841365,0.357800735330979,
0.375339207698853,0.378621596831413),.UNSPECIFIED.);
#3977=B_SPLINE_CURVE_WITH_KNOTS('',3,(#50458,#50459,#50460,#50461,#50462,
#50463,#50464,#50465,#50466,#50467,#50468,#50469,#50470,#50471,#50472,#50473,
#50474,#50475,#50476,#50477,#50478,#50479,#50480,#50481,#50482,#50483,#50484,
#50485,#50486,#50487,#50488,#50489,#50490,#50491,#50492,#50493,#50494,#50495,
#50496,#50497,#50498,#50499,#50500,#50501,#50502,#50503,#50504,#50505,#50506,
#50507,#50508,#50509,#50510,#50511,#50512,#50513,#50514,#50515,#50516,#50517,
#50518,#50519,#50520,#50521,#50522,#50523,#50524,#50525,#50526,#50527,#50528,
#50529,#50530,#50531,#50532,#50533,#50534,#50535,#50536,#50537,#50538,#50539,
#50540,#50541,#50542,#50543,#50544,#50545),.UNSPECIFIED.,.F.,.F.,(4,3,3,
3,3,3,3,3,3,3,3,3,3,3,3,3,3,3,3,3,3,3,3,3,3,3,3,3,3,4),(-0.378621596831417,
-0.359796324497933,-0.347853968215386,-0.339667381051392,-0.33535479313986,
-0.315481654241569,-0.301150134421133,-0.297197750394092,-0.293218427819012,
-0.272815226641669,-0.252117692398167,-0.239295643218144,-0.228788599088732,
-0.224499673218097,-0.203195145608534,-0.200829495678077,-0.18034287834285,
-0.158302095025605,-0.154271536511048,-0.150798918828779,-0.129416060221611,
-0.107582030158341,-0.0856154294482134,-0.0801878898697612,-0.0759393010155595,
-0.0533917821073025,-0.0308195963955261,-0.00876131064632734,-0.00401661180488987,
0.),.UNSPECIFIED.);
#3978=B_SPLINE_CURVE_WITH_KNOTS('',3,(#50546,#50547,#50548,#50549,#50550,
#50551,#50552,#50553,#50554,#50555,#50556,#50557,#50558,#50559,#50560,#50561,
#50562,#50563,#50564,#50565,#50566,#50567,#50568,#50569,#50570,#50571,#50572,
#50573,#50574,#50575,#50576,#50577,#50578,#50579,#50580,#50581,#50582,#50583,
#50584,#50585,#50586,#50587,#50588,#50589,#50590,#50591,#50592,#50593,#50594,
#50595,#50596,#50597,#50598,#50599,#50600,#50601,#50602,#50603,#50604,#50605,
#50606,#50607,#50608,#50609,#50610,#50611,#50612,#50613,#50614,#50615,#50616,
#50617,#50618,#50619,#50620,#50621,#50622,#50623,#50624,#50625,#50626,#50627,
#50628,#50629,#50630),.UNSPECIFIED.,.F.,.F.,(4,3,3,3,3,3,3,3,3,3,3,3,3,
3,3,3,3,3,3,3,3,3,3,3,3,3,3,3,4),(-0.376940817211599,-0.354633525341571,
-0.332911188282741,-0.328062756116004,-0.305814149686869,-0.290194234584877,
-0.284254884750481,-0.278600964800113,-0.256917900841735,-0.235700669608916,
-0.214948669584839,-0.208204193177863,-0.204400682430755,-0.18382493241094,
-0.180854828870933,-0.159872083890278,-0.1402968745328,-0.135977073907336,
-0.132599774507536,-0.112140461897276,-0.0917757502511294,-0.0718475646021411,
-0.0676500217440913,-0.0636684046549802,-0.044110611876292,-0.0249250199794228,
-0.00636290551127469,-0.00327040903045178,0.),.UNSPECIFIED.);
#3979=B_SPLINE_CURVE_WITH_KNOTS('',3,(#50632,#50633,#50634,#50635,#50636,
#50637,#50638,#50639,#50640,#50641,#50642),.UNSPECIFIED.,.F.,.F.,(4,1,1,
1,1,1,1,1,4),(15.7079632679489,15.8518654961884,16.8494368691713,17.8470082421543,
18.8445796151372,19.8421509881201,20.8397223611031,21.837293734086,21.9911485751285),
 .UNSPECIFIED.);
#3980=B_SPLINE_CURVE_WITH_KNOTS('',3,(#50643,#50644,#50645,#50646,#50647,
#50648,#50649,#50650,#50651,#50652),.UNSPECIFIED.,.F.,.F.,(4,1,1,1,1,1,
1,4),(15.7079632679489,16.3932837587428,17.3908551317257,18.3884265047087,
19.3859978776916,20.3835692506745,21.3811406236575,21.9911485751285),
 .UNSPECIFIED.);
#3981=B_SPLINE_CURVE_WITH_KNOTS('',3,(#50997,#50998,#50999,#51000,#51001,
#51002,#51003,#51004,#51005,#51006,#51007,#51008,#51009,#51010,#51011,#51012,
#51013,#51014,#51015,#51016,#51017,#51018,#51019,#51020,#51021,#51022,#51023,
#51024,#51025,#51026,#51027,#51028,#51029,#51030,#51031,#51032,#51033,#51034,
#51035,#51036,#51037,#51038,#51039,#51040,#51041,#51042,#51043,#51044,#51045,
#51046,#51047,#51048,#51049,#51050,#51051,#51052,#51053,#51054,#51055,#51056,
#51057,#51058,#51059,#51060,#51061,#51062,#51063,#51064,#51065,#51066,#51067,
#51068,#51069,#51070,#51071,#51072,#51073,#51074,#51075,#51076,#51077,#51078),
 .UNSPECIFIED.,.F.,.F.,(4,3,3,3,3,3,3,3,3,3,3,3,3,3,3,3,3,3,3,3,3,3,3,3,
3,3,3,4),(0.,0.0185987341995647,0.0384245494583765,0.0557721378098369,0.0644770178569765,
0.068452005390303,0.0885071145869722,0.108917452397134,0.125989403365366,
0.133856151017707,0.137288655783233,0.15836342516836,0.177205256270059,
0.197732482353179,0.20565277044136,0.209127273146685,0.230132191380251,
0.251624049747522,0.268069475039372,0.27830521821265,0.284046462288397,
0.306315432127717,0.322971764216374,0.328167478835643,0.333183009452404,
0.355704395482805,0.372940760482345,0.37694081721169),.UNSPECIFIED.);
#3982=B_SPLINE_CURVE_WITH_KNOTS('',3,(#51079,#51080,#51081,#51082,#51083,
#51084,#51085,#51086,#51087,#51088,#51089,#51090,#51091,#51092,#51093,#51094,
#51095,#51096,#51097,#51098,#51099,#51100,#51101,#51102,#51103),
 .UNSPECIFIED.,.F.,.F.,(4,3,3,3,3,3,3,3,4),(-10.1295685708718,-9.97571372982932,
-8.97814235684639,-7.98057098386346,-6.98299961088053,-5.98542823789759,
-4.98785686491466,-3.99028549193173,-3.84638326369223),.UNSPECIFIED.);
#3983=B_SPLINE_CURVE_WITH_KNOTS('',3,(#51448,#51449,#51450,#51451,#51452,
#51453,#51454,#51455,#51456,#51457,#51458,#51459,#51460,#51461,#51462,#51463,
#51464,#51465,#51466,#51467,#51468,#51469),.UNSPECIFIED.,.F.,.F.,(4,3,3,
3,3,3,3,4),(7.59300756235153,7.98057098386347,8.9781423568464,9.97571372982933,
10.9732851028123,11.9708564757952,12.9684278487781,13.8761928695311),
 .UNSPECIFIED.);
#3984=B_SPLINE_CURVE_WITH_KNOTS('',3,(#51470,#51471,#51472,#51473,#51474,
#51475,#51476,#51477,#51478,#51479,#51480,#51481,#51482,#51483,#51484,#51485,
#51486,#51487,#51488,#51489,#51490,#51491,#51492,#51493,#51494,#51495,#51496,
#51497,#51498,#51499,#51500,#51501,#51502,#51503,#51504,#51505,#51506,#51507,
#51508,#51509,#51510,#51511,#51512,#51513,#51514,#51515,#51516,#51517,#51518,
#51519,#51520,#51521,#51522,#51523,#51524,#51525,#51526,#51527,#51528,#51529,
#51530,#51531,#51532,#51533,#51534,#51535,#51536,#51537,#51538,#51539,#51540,
#51541,#51542,#51543,#51544,#51545,#51546,#51547,#51548,#51549,#51550,#51551,
#51552,#51553,#51554),.UNSPECIFIED.,.F.,.F.,(4,3,3,3,3,3,3,3,3,3,3,3,3,
3,3,3,3,3,3,3,3,3,3,3,3,3,3,3,4),(0.,0.0219671392710627,0.0445447270614996,
0.0636220854571156,0.0720971088190858,0.0767543937611971,0.0810485771087931,
0.102995177264397,0.12477118871929,0.142869290096075,0.150423609225186,
0.153920425498144,0.15756713475292,0.178337528533867,0.197163594226427,
0.219435545910481,0.224338960691702,0.229398550502591,0.250063644957184,
0.270724495002125,0.2856781237343,0.296895177864656,0.300623717137974,0.32039569443208,
0.334308019624689,0.338773858972783,0.357798151609198,0.37533920769886,
0.37862159683142),.UNSPECIFIED.);
#3985=B_SPLINE_CURVE_WITH_KNOTS('',3,(#51558,#51559,#51560,#51561,#51562,
#51563,#51564,#51565,#51566,#51567,#51568,#51569,#51570,#51571,#51572,#51573,
#51574,#51575,#51576,#51577,#51578,#51579,#51580,#51581,#51582,#51583,#51584,
#51585,#51586,#51587,#51588,#51589,#51590,#51591,#51592,#51593,#51594,#51595,
#51596,#51597,#51598,#51599,#51600,#51601,#51602,#51603,#51604,#51605,#51606,
#51607,#51608,#51609,#51610,#51611,#51612,#51613,#51614,#51615,#51616,#51617,
#51618,#51619,#51620,#51621,#51622,#51623,#51624,#51625,#51626,#51627,#51628,
#51629,#51630,#51631,#51632,#51633,#51634,#51635,#51636,#51637,#51638,#51639,
#51640,#51641,#51642,#51643,#51644,#51645),.UNSPECIFIED.,.F.,.F.,(4,3,3,
3,3,3,3,3,3,3,3,3,3,3,3,3,3,3,3,3,3,3,3,3,3,3,3,3,3,4),(-0.378621596831453,
-0.359796964367516,-0.34785559588844,-0.339682222403536,-0.335363223677477,
-0.31549070609328,-0.301158054791382,-0.297216022364776,-0.29322112959255,
-0.272818393264414,-0.252120789758935,-0.239297966238724,-0.228792024964215,
-0.224500801096337,-0.203196242733446,-0.200829495678093,-0.180342437231382,
-0.158301709053072,-0.15426886502637,-0.150798379224116,-0.129415160899972,
-0.10758097206945,-0.0856143687245085,-0.080186043251393,-0.0759386413924393,
-0.053391048511125,-0.0308188757754254,-0.00876051286996735,-0.00401661180489571,
0.),.UNSPECIFIED.);
#3986=B_SPLINE_CURVE_WITH_KNOTS('',3,(#51646,#51647,#51648,#51649,#51650,
#51651,#51652,#51653,#51654,#51655,#51656,#51657,#51658,#51659,#51660,#51661,
#51662,#51663,#51664,#51665,#51666,#51667,#51668,#51669,#51670,#51671,#51672,
#51673,#51674,#51675,#51676,#51677,#51678,#51679,#51680,#51681,#51682,#51683,
#51684,#51685,#51686,#51687,#51688,#51689,#51690,#51691,#51692,#51693,#51694,
#51695,#51696,#51697,#51698,#51699,#51700,#51701,#51702,#51703,#51704,#51705,
#51706,#51707,#51708,#51709,#51710,#51711,#51712,#51713,#51714,#51715,#51716,
#51717,#51718,#51719,#51720,#51721,#51722,#51723,#51724,#51725,#51726,#51727,
#51728,#51729,#51730),.UNSPECIFIED.,.F.,.F.,(4,3,3,3,3,3,3,3,3,3,3,3,3,
3,3,3,3,3,3,3,3,3,3,3,3,3,3,3,4),(-0.376940817211633,-0.354633964602481,
-0.332911572636038,-0.328063202247457,-0.305814587526729,-0.290194617694755,
-0.284255735322417,-0.278600908077479,-0.256917768897898,-0.235700347784253,
-0.214948223366311,-0.208204476162521,-0.204400640110824,-0.183824705944621,
-0.180854828870941,-0.159872081610359,-0.140296872537871,-0.13597675000398,
-0.132599526175717,-0.112140240543943,-0.0917754711192709,-0.0718470375036391,
-0.0676485677836509,-0.0636679489822672,-0.0441100183726961,-0.0249241308057409,
-0.00636153480048415,-0.00327040903045198,0.),.UNSPECIFIED.);
#3987=B_SPLINE_CURVE_WITH_KNOTS('',3,(#51732,#51733,#51734,#51735,#51736,
#51737,#51738,#51739,#51740,#51741,#51742),.UNSPECIFIED.,.F.,.F.,(4,1,1,
1,1,1,1,1,4),(15.7079632679489,15.8518654961884,16.8494368691713,17.8470082421542,
18.8445796151372,19.8421509881201,20.839722361103,21.837293734086,21.9911485751285),
 .UNSPECIFIED.);
#3988=B_SPLINE_CURVE_WITH_KNOTS('',3,(#51743,#51744,#51745,#51746,#51747,
#51748,#51749,#51750,#51751,#51752),.UNSPECIFIED.,.F.,.F.,(4,1,1,1,1,1,
1,4),(15.7079632679489,16.3932837587428,17.3908551317257,18.3884265047086,
19.3859978776916,20.3835692506745,21.3811406236574,21.9911485751285),
 .UNSPECIFIED.);
#3989=B_SPLINE_CURVE_WITH_KNOTS('',3,(#52097,#52098,#52099,#52100,#52101,
#52102,#52103,#52104,#52105,#52106,#52107,#52108,#52109,#52110,#52111,#52112,
#52113,#52114,#52115,#52116,#52117,#52118,#52119,#52120,#52121,#52122,#52123,
#52124,#52125,#52126,#52127,#52128,#52129,#52130,#52131,#52132,#52133,#52134,
#52135,#52136,#52137,#52138,#52139,#52140,#52141,#52142,#52143,#52144,#52145,
#52146,#52147,#52148,#52149,#52150,#52151,#52152,#52153,#52154,#52155,#52156,
#52157,#52158,#52159,#52160,#52161,#52162,#52163,#52164,#52165,#52166,#52167,
#52168,#52169,#52170,#52171,#52172,#52173,#52174,#52175,#52176,#52177,#52178),
 .UNSPECIFIED.,.F.,.F.,(4,3,3,3,3,3,3,3,3,3,3,3,3,3,3,3,3,3,3,3,3,3,3,3,
3,3,3,4),(0.,0.0185980112512777,0.0384239168786204,0.0557715843025452,0.0644760598120422,
0.0684517536273742,0.0885063485050852,0.108916466871302,0.125988664220981,
0.133854987328047,0.137288032277356,0.158362873192896,0.177205256270019,
0.197732848455459,0.205652969330799,0.209127416443499,0.230132765552162,
0.251624849776322,0.268069291421993,0.278304794057273,0.284046573502879,
0.306315569636911,0.322971867348254,0.328167702950825,0.333183121098172,
0.355704505357051,0.372940760482282,0.376940817211626),.UNSPECIFIED.);
#3990=B_SPLINE_CURVE_WITH_KNOTS('',3,(#52179,#52180,#52181,#52182,#52183,
#52184,#52185,#52186,#52187,#52188,#52189,#52190,#52191,#52192,#52193,#52194,
#52195,#52196,#52197,#52198,#52199,#52200,#52201,#52202,#52203),
 .UNSPECIFIED.,.F.,.F.,(4,3,3,3,3,3,3,3,4),(-10.1295685708719,-9.97571372982933,
-8.97814235684639,-7.98057098386346,-6.98299961088053,-5.9854282378976,
-4.98785686491466,-3.99028549193173,-3.84638326369226),.UNSPECIFIED.);
#3991=B_SPLINE_CURVE_WITH_KNOTS('',3,(#52548,#52549,#52550,#52551,#52552,
#52553,#52554,#52555,#52556,#52557,#52558,#52559,#52560,#52561,#52562,#52563,
#52564,#52565,#52566,#52567,#52568,#52569),.UNSPECIFIED.,.F.,.F.,(4,3,3,
3,3,3,3,4),(7.59300756235153,7.98057098386346,8.97814235684639,9.97571372982933,
10.9732851028123,11.9708564757952,12.9684278487781,13.8761928695311),
 .UNSPECIFIED.);
#3992=B_SPLINE_CURVE_WITH_KNOTS('',3,(#52570,#52571,#52572,#52573,#52574,
#52575,#52576,#52577,#52578,#52579,#52580,#52581,#52582,#52583,#52584,#52585,
#52586,#52587,#52588,#52589,#52590,#52591,#52592,#52593,#52594,#52595,#52596,
#52597,#52598,#52599,#52600,#52601,#52602,#52603,#52604,#52605,#52606,#52607,
#52608,#52609,#52610,#52611,#52612,#52613,#52614,#52615,#52616,#52617,#52618,
#52619,#52620,#52621,#52622,#52623,#52624,#52625,#52626,#52627,#52628,#52629,
#52630,#52631,#52632,#52633,#52634,#52635,#52636,#52637,#52638,#52639,#52640,
#52641,#52642,#52643,#52644,#52645,#52646,#52647,#52648,#52649,#52650,#52651,
#52652,#52653,#52654),.UNSPECIFIED.,.F.,.F.,(4,3,3,3,3,3,3,3,3,3,3,3,3,
3,3,3,3,3,3,3,3,3,3,3,3,3,3,3,4),(0.,0.0219665840177821,0.0445441200922931,
0.0636215543590582,0.0720969499799132,0.0767540580968699,0.0810484869491109,
0.102995100015314,0.12477128128117,0.142869359517481,0.150423583503905,
0.153920259630152,0.157567081122177,0.178337643732528,0.197163594226414,
0.219435545910471,0.224339007945445,0.229398552617908,0.250063626009798,
0.270724499291964,0.285678648510981,0.296896068885296,0.300623970908951,
0.320396153950705,0.334308778694922,0.338774577569346,0.357799193930767,
0.375339207698866,0.378621596831428),.UNSPECIFIED.);
#4630=LINE('',#23380,#5534);
#4631=LINE('',#23415,#5535);
#4632=LINE('',#23442,#5536);
#4633=LINE('',#23493,#5537);
#4634=LINE('',#23541,#5538);
#4635=LINE('',#23589,#5539);
#4636=LINE('',#23640,#5540);
#4637=LINE('',#23688,#5541);
#4638=LINE('',#23736,#5542);
#4639=LINE('',#23787,#5543);
#4640=LINE('',#23838,#5544);
#4641=LINE('',#23886,#5545);
#4642=LINE('',#23937,#5546);
#4643=LINE('',#23976,#5547);
#4644=LINE('',#23998,#5548);
#4645=LINE('',#24022,#5549);
#4646=LINE('',#24047,#5550);
#4647=LINE('',#24072,#5551);
#4648=LINE('',#24096,#5552);
#4649=LINE('',#24121,#5553);
#4650=LINE('',#24145,#5554);
#4651=LINE('',#24170,#5555);
#4652=LINE('',#24194,#5556);
#4653=LINE('',#24219,#5557);
#4654=LINE('',#24244,#5558);
#4655=LINE('',#24268,#5559);
#4656=LINE('',#24285,#5560);
#4657=LINE('',#24320,#5561);
#4658=LINE('',#24347,#5562);
#4659=LINE('',#24398,#5563);
#4660=LINE('',#24446,#5564);
#4661=LINE('',#24494,#5565);
#4662=LINE('',#24545,#5566);
#4663=LINE('',#24593,#5567);
#4664=LINE('',#24641,#5568);
#4665=LINE('',#24692,#5569);
#4666=LINE('',#24743,#5570);
#4667=LINE('',#24791,#5571);
#4668=LINE('',#24842,#5572);
#4669=LINE('',#24881,#5573);
#4670=LINE('',#24903,#5574);
#4671=LINE('',#24927,#5575);
#4672=LINE('',#24952,#5576);
#4673=LINE('',#24977,#5577);
#4674=LINE('',#25001,#5578);
#4675=LINE('',#25026,#5579);
#4676=LINE('',#25050,#5580);
#4677=LINE('',#25075,#5581);
#4678=LINE('',#25099,#5582);
#4679=LINE('',#25124,#5583);
#4680=LINE('',#25149,#5584);
#4681=LINE('',#25173,#5585);
#4682=LINE('',#25190,#5586);
#4683=LINE('',#25225,#5587);
#4684=LINE('',#25252,#5588);
#4685=LINE('',#25303,#5589);
#4686=LINE('',#25351,#5590);
#4687=LINE('',#25399,#5591);
#4688=LINE('',#25450,#5592);
#4689=LINE('',#25498,#5593);
#4690=LINE('',#25546,#5594);
#4691=LINE('',#25597,#5595);
#4692=LINE('',#25648,#5596);
#4693=LINE('',#25696,#5597);
#4694=LINE('',#25747,#5598);
#4695=LINE('',#25786,#5599);
#4696=LINE('',#25808,#5600);
#4697=LINE('',#25832,#5601);
#4698=LINE('',#25857,#5602);
#4699=LINE('',#25882,#5603);
#4700=LINE('',#25906,#5604);
#4701=LINE('',#25931,#5605);
#4702=LINE('',#25955,#5606);
#4703=LINE('',#25980,#5607);
#4704=LINE('',#26004,#5608);
#4705=LINE('',#26029,#5609);
#4706=LINE('',#26054,#5610);
#4707=LINE('',#26078,#5611);
#4708=LINE('',#26095,#5612);
#4709=LINE('',#26130,#5613);
#4710=LINE('',#26157,#5614);
#4711=LINE('',#26208,#5615);
#4712=LINE('',#26256,#5616);
#4713=LINE('',#26304,#5617);
#4714=LINE('',#26355,#5618);
#4715=LINE('',#26403,#5619);
#4716=LINE('',#26451,#5620);
#4717=LINE('',#26502,#5621);
#4718=LINE('',#26553,#5622);
#4719=LINE('',#26601,#5623);
#4720=LINE('',#26652,#5624);
#4721=LINE('',#26691,#5625);
#4722=LINE('',#26713,#5626);
#4723=LINE('',#26737,#5627);
#4724=LINE('',#26762,#5628);
#4725=LINE('',#26787,#5629);
#4726=LINE('',#26811,#5630);
#4727=LINE('',#26836,#5631);
#4728=LINE('',#26860,#5632);
#4729=LINE('',#26885,#5633);
#4730=LINE('',#26909,#5634);
#4731=LINE('',#26934,#5635);
#4732=LINE('',#26959,#5636);
#4733=LINE('',#26983,#5637);
#4734=LINE('',#27000,#5638);
#4735=LINE('',#27035,#5639);
#4736=LINE('',#27062,#5640);
#4737=LINE('',#27113,#5641);
#4738=LINE('',#27161,#5642);
#4739=LINE('',#27209,#5643);
#4740=LINE('',#27260,#5644);
#4741=LINE('',#27308,#5645);
#4742=LINE('',#27356,#5646);
#4743=LINE('',#27407,#5647);
#4744=LINE('',#27458,#5648);
#4745=LINE('',#27506,#5649);
#4746=LINE('',#27557,#5650);
#4747=LINE('',#27596,#5651);
#4748=LINE('',#27618,#5652);
#4749=LINE('',#27642,#5653);
#4750=LINE('',#27667,#5654);
#4751=LINE('',#27692,#5655);
#4752=LINE('',#27716,#5656);
#4753=LINE('',#27741,#5657);
#4754=LINE('',#27765,#5658);
#4755=LINE('',#27790,#5659);
#4756=LINE('',#27814,#5660);
#4757=LINE('',#27839,#5661);
#4758=LINE('',#27864,#5662);
#4759=LINE('',#27888,#5663);
#4760=LINE('',#27905,#5664);
#4761=LINE('',#27940,#5665);
#4762=LINE('',#27967,#5666);
#4763=LINE('',#28018,#5667);
#4764=LINE('',#28066,#5668);
#4765=LINE('',#28114,#5669);
#4766=LINE('',#28165,#5670);
#4767=LINE('',#28213,#5671);
#4768=LINE('',#28261,#5672);
#4769=LINE('',#28312,#5673);
#4770=LINE('',#28363,#5674);
#4771=LINE('',#28411,#5675);
#4772=LINE('',#28462,#5676);
#4773=LINE('',#28501,#5677);
#4774=LINE('',#28523,#5678);
#4775=LINE('',#28547,#5679);
#4776=LINE('',#28572,#5680);
#4777=LINE('',#28597,#5681);
#4778=LINE('',#28621,#5682);
#4779=LINE('',#28646,#5683);
#4780=LINE('',#28670,#5684);
#4781=LINE('',#28695,#5685);
#4782=LINE('',#28719,#5686);
#4783=LINE('',#28744,#5687);
#4784=LINE('',#28769,#5688);
#4785=LINE('',#28793,#5689);
#4786=LINE('',#28810,#5690);
#4787=LINE('',#28845,#5691);
#4788=LINE('',#28872,#5692);
#4789=LINE('',#28923,#5693);
#4790=LINE('',#28971,#5694);
#4791=LINE('',#29019,#5695);
#4792=LINE('',#29070,#5696);
#4793=LINE('',#29118,#5697);
#4794=LINE('',#29166,#5698);
#4795=LINE('',#29217,#5699);
#4796=LINE('',#29268,#5700);
#4797=LINE('',#29316,#5701);
#4798=LINE('',#29367,#5702);
#4799=LINE('',#29406,#5703);
#4800=LINE('',#29428,#5704);
#4801=LINE('',#29452,#5705);
#4802=LINE('',#29477,#5706);
#4803=LINE('',#29502,#5707);
#4804=LINE('',#29526,#5708);
#4805=LINE('',#29551,#5709);
#4806=LINE('',#29575,#5710);
#4807=LINE('',#29600,#5711);
#4808=LINE('',#29624,#5712);
#4809=LINE('',#29649,#5713);
#4810=LINE('',#29674,#5714);
#4811=LINE('',#29698,#5715);
#4812=LINE('',#29715,#5716);
#4813=LINE('',#29750,#5717);
#4814=LINE('',#29777,#5718);
#4815=LINE('',#29828,#5719);
#4816=LINE('',#29876,#5720);
#4817=LINE('',#29924,#5721);
#4818=LINE('',#29975,#5722);
#4819=LINE('',#30023,#5723);
#4820=LINE('',#30071,#5724);
#4821=LINE('',#30122,#5725);
#4822=LINE('',#30173,#5726);
#4823=LINE('',#30221,#5727);
#4824=LINE('',#30272,#5728);
#4825=LINE('',#30311,#5729);
#4826=LINE('',#30333,#5730);
#4827=LINE('',#30357,#5731);
#4828=LINE('',#30382,#5732);
#4829=LINE('',#30407,#5733);
#4830=LINE('',#30431,#5734);
#4831=LINE('',#30456,#5735);
#4832=LINE('',#30480,#5736);
#4833=LINE('',#30505,#5737);
#4834=LINE('',#30529,#5738);
#4835=LINE('',#30554,#5739);
#4836=LINE('',#30579,#5740);
#4837=LINE('',#30603,#5741);
#4838=LINE('',#30620,#5742);
#4839=LINE('',#30655,#5743);
#4840=LINE('',#30682,#5744);
#4841=LINE('',#30733,#5745);
#4842=LINE('',#30781,#5746);
#4843=LINE('',#30829,#5747);
#4844=LINE('',#30880,#5748);
#4845=LINE('',#30928,#5749);
#4846=LINE('',#30976,#5750);
#4847=LINE('',#31027,#5751);
#4848=LINE('',#31078,#5752);
#4849=LINE('',#31126,#5753);
#4850=LINE('',#31177,#5754);
#4851=LINE('',#31216,#5755);
#4852=LINE('',#31238,#5756);
#4853=LINE('',#31262,#5757);
#4854=LINE('',#31287,#5758);
#4855=LINE('',#31312,#5759);
#4856=LINE('',#31336,#5760);
#4857=LINE('',#31361,#5761);
#4858=LINE('',#31385,#5762);
#4859=LINE('',#31410,#5763);
#4860=LINE('',#31434,#5764);
#4861=LINE('',#31459,#5765);
#4862=LINE('',#31484,#5766);
#4863=LINE('',#31508,#5767);
#4864=LINE('',#31525,#5768);
#4865=LINE('',#31560,#5769);
#4866=LINE('',#31587,#5770);
#4867=LINE('',#31638,#5771);
#4868=LINE('',#31686,#5772);
#4869=LINE('',#31734,#5773);
#4870=LINE('',#31785,#5774);
#4871=LINE('',#31833,#5775);
#4872=LINE('',#31881,#5776);
#4873=LINE('',#31932,#5777);
#4874=LINE('',#31983,#5778);
#4875=LINE('',#32031,#5779);
#4876=LINE('',#32082,#5780);
#4877=LINE('',#32121,#5781);
#4878=LINE('',#32143,#5782);
#4879=LINE('',#32167,#5783);
#4880=LINE('',#32192,#5784);
#4881=LINE('',#32217,#5785);
#4882=LINE('',#32241,#5786);
#4883=LINE('',#32266,#5787);
#4884=LINE('',#32290,#5788);
#4885=LINE('',#32315,#5789);
#4886=LINE('',#32339,#5790);
#4887=LINE('',#32364,#5791);
#4888=LINE('',#32389,#5792);
#4889=LINE('',#32413,#5793);
#4890=LINE('',#32430,#5794);
#4891=LINE('',#32465,#5795);
#4892=LINE('',#32492,#5796);
#4893=LINE('',#32543,#5797);
#4894=LINE('',#32591,#5798);
#4895=LINE('',#32639,#5799);
#4896=LINE('',#32690,#5800);
#4897=LINE('',#32738,#5801);
#4898=LINE('',#32786,#5802);
#4899=LINE('',#32837,#5803);
#4900=LINE('',#32888,#5804);
#4901=LINE('',#32936,#5805);
#4902=LINE('',#32987,#5806);
#4903=LINE('',#33026,#5807);
#4904=LINE('',#33048,#5808);
#4905=LINE('',#33072,#5809);
#4906=LINE('',#33097,#5810);
#4907=LINE('',#33122,#5811);
#4908=LINE('',#33146,#5812);
#4909=LINE('',#33171,#5813);
#4910=LINE('',#33195,#5814);
#4911=LINE('',#33220,#5815);
#4912=LINE('',#33244,#5816);
#4913=LINE('',#33269,#5817);
#4914=LINE('',#33294,#5818);
#4915=LINE('',#33318,#5819);
#4916=LINE('',#33335,#5820);
#4917=LINE('',#33370,#5821);
#4918=LINE('',#33397,#5822);
#4919=LINE('',#33448,#5823);
#4920=LINE('',#33496,#5824);
#4921=LINE('',#33544,#5825);
#4922=LINE('',#33595,#5826);
#4923=LINE('',#33643,#5827);
#4924=LINE('',#33691,#5828);
#4925=LINE('',#33742,#5829);
#4926=LINE('',#33793,#5830);
#4927=LINE('',#33841,#5831);
#4928=LINE('',#33892,#5832);
#4929=LINE('',#33931,#5833);
#4930=LINE('',#33953,#5834);
#4931=LINE('',#33977,#5835);
#4932=LINE('',#34002,#5836);
#4933=LINE('',#34027,#5837);
#4934=LINE('',#34051,#5838);
#4935=LINE('',#34076,#5839);
#4936=LINE('',#34100,#5840);
#4937=LINE('',#34125,#5841);
#4938=LINE('',#34149,#5842);
#4939=LINE('',#34174,#5843);
#4940=LINE('',#34199,#5844);
#4941=LINE('',#34223,#5845);
#4942=LINE('',#34240,#5846);
#4943=LINE('',#34261,#5847);
#4944=LINE('',#34312,#5848);
#4945=LINE('',#34363,#5849);
#4946=LINE('',#34411,#5850);
#4947=LINE('',#34465,#5851);
#4948=LINE('',#34513,#5852);
#4949=LINE('',#34561,#5853);
#4950=LINE('',#34611,#5854);
#4951=LINE('',#34635,#5855);
#4952=LINE('',#34659,#5856);
#4953=LINE('',#34684,#5857);
#4954=LINE('',#34709,#5858);
#4955=LINE('',#34734,#5859);
#4956=LINE('',#34758,#5860);
#4957=LINE('',#34783,#5861);
#4958=LINE('',#34809,#5862);
#4959=LINE('',#34830,#5863);
#4960=LINE('',#34881,#5864);
#4961=LINE('',#34932,#5865);
#4962=LINE('',#34980,#5866);
#4963=LINE('',#35034,#5867);
#4964=LINE('',#35082,#5868);
#4965=LINE('',#35130,#5869);
#4966=LINE('',#35180,#5870);
#4967=LINE('',#35201,#5871);
#4968=LINE('',#35252,#5872);
#4969=LINE('',#35303,#5873);
#4970=LINE('',#35351,#5874);
#4971=LINE('',#35405,#5875);
#4972=LINE('',#35453,#5876);
#4973=LINE('',#35501,#5877);
#4974=LINE('',#35551,#5878);
#4975=LINE('',#35572,#5879);
#4976=LINE('',#35623,#5880);
#4977=LINE('',#35674,#5881);
#4978=LINE('',#35722,#5882);
#4979=LINE('',#35776,#5883);
#4980=LINE('',#35824,#5884);
#4981=LINE('',#35872,#5885);
#4982=LINE('',#35922,#5886);
#4983=LINE('',#35946,#5887);
#4984=LINE('',#35970,#5888);
#4985=LINE('',#35995,#5889);
#4986=LINE('',#36020,#5890);
#4987=LINE('',#36045,#5891);
#4988=LINE('',#36069,#5892);
#4989=LINE('',#36094,#5893);
#4990=LINE('',#36120,#5894);
#4991=LINE('',#36144,#5895);
#4992=LINE('',#36168,#5896);
#4993=LINE('',#36193,#5897);
#4994=LINE('',#36218,#5898);
#4995=LINE('',#36243,#5899);
#4996=LINE('',#36267,#5900);
#4997=LINE('',#36292,#5901);
#4998=LINE('',#36318,#5902);
#4999=LINE('',#36342,#5903);
#5000=LINE('',#36366,#5904);
#5001=LINE('',#36391,#5905);
#5002=LINE('',#36416,#5906);
#5003=LINE('',#36441,#5907);
#5004=LINE('',#36465,#5908);
#5005=LINE('',#36490,#5909);
#5006=LINE('',#52661,#5910);
#5007=LINE('',#52667,#5911);
#5534=VECTOR('',#19805,2.);
#5535=VECTOR('',#19808,2.);
#5536=VECTOR('',#19813,2.);
#5537=VECTOR('',#19816,2.);
#5538=VECTOR('',#19819,2.);
#5539=VECTOR('',#19822,2.);
#5540=VECTOR('',#19825,2.);
#5541=VECTOR('',#19828,2.);
#5542=VECTOR('',#19831,2.);
#5543=VECTOR('',#19834,2.);
#5544=VECTOR('',#19837,2.);
#5545=VECTOR('',#19840,2.);
#5546=VECTOR('',#19843,2.);
#5547=VECTOR('',#19848,2.05475);
#5548=VECTOR('',#19853,2.05475);
#5549=VECTOR('',#19856,2.05475);
#5550=VECTOR('',#19859,2.05475);
#5551=VECTOR('',#19862,2.05475);
#5552=VECTOR('',#19865,2.05475);
#5553=VECTOR('',#19868,2.05475);
#5554=VECTOR('',#19871,2.05475);
#5555=VECTOR('',#19874,2.05475);
#5556=VECTOR('',#19877,2.05475);
#5557=VECTOR('',#19880,2.05475);
#5558=VECTOR('',#19883,2.05475);
#5559=VECTOR('',#19886,2.05475);
#5560=VECTOR('',#19891,2.);
#5561=VECTOR('',#19894,2.);
#5562=VECTOR('',#19899,2.);
#5563=VECTOR('',#19902,2.);
#5564=VECTOR('',#19905,2.);
#5565=VECTOR('',#19908,2.);
#5566=VECTOR('',#19911,2.);
#5567=VECTOR('',#19914,2.);
#5568=VECTOR('',#19917,2.);
#5569=VECTOR('',#19920,2.);
#5570=VECTOR('',#19923,2.);
#5571=VECTOR('',#19926,2.);
#5572=VECTOR('',#19929,2.);
#5573=VECTOR('',#19934,2.05475);
#5574=VECTOR('',#19939,2.05475);
#5575=VECTOR('',#19942,2.05475);
#5576=VECTOR('',#19945,2.05475);
#5577=VECTOR('',#19948,2.05475);
#5578=VECTOR('',#19951,2.05475);
#5579=VECTOR('',#19954,2.05475);
#5580=VECTOR('',#19957,2.05475);
#5581=VECTOR('',#19960,2.05475);
#5582=VECTOR('',#19963,2.05475);
#5583=VECTOR('',#19966,2.05475);
#5584=VECTOR('',#19969,2.05475);
#5585=VECTOR('',#19972,2.05475);
#5586=VECTOR('',#19977,2.);
#5587=VECTOR('',#19980,2.);
#5588=VECTOR('',#19985,2.);
#5589=VECTOR('',#19988,2.);
#5590=VECTOR('',#19991,2.);
#5591=VECTOR('',#19994,2.);
#5592=VECTOR('',#19997,2.);
#5593=VECTOR('',#20000,2.);
#5594=VECTOR('',#20003,2.);
#5595=VECTOR('',#20006,2.);
#5596=VECTOR('',#20009,2.);
#5597=VECTOR('',#20012,2.);
#5598=VECTOR('',#20015,2.);
#5599=VECTOR('',#20020,2.05475);
#5600=VECTOR('',#20025,2.05475);
#5601=VECTOR('',#20028,2.05475);
#5602=VECTOR('',#20031,2.05475);
#5603=VECTOR('',#20034,2.05475);
#5604=VECTOR('',#20037,2.05475);
#5605=VECTOR('',#20040,2.05475);
#5606=VECTOR('',#20043,2.05475);
#5607=VECTOR('',#20046,2.05475);
#5608=VECTOR('',#20049,2.05475);
#5609=VECTOR('',#20052,2.05475);
#5610=VECTOR('',#20055,2.05475);
#5611=VECTOR('',#20058,2.05475);
#5612=VECTOR('',#20063,2.);
#5613=VECTOR('',#20066,2.);
#5614=VECTOR('',#20071,2.);
#5615=VECTOR('',#20074,2.);
#5616=VECTOR('',#20077,2.);
#5617=VECTOR('',#20080,2.);
#5618=VECTOR('',#20083,2.);
#5619=VECTOR('',#20086,2.);
#5620=VECTOR('',#20089,2.);
#5621=VECTOR('',#20092,2.);
#5622=VECTOR('',#20095,2.);
#5623=VECTOR('',#20098,2.);
#5624=VECTOR('',#20101,2.);
#5625=VECTOR('',#20106,2.05474999999998);
#5626=VECTOR('',#20111,2.05474999999998);
#5627=VECTOR('',#20114,2.05474999999998);
#5628=VECTOR('',#20117,2.05474999999998);
#5629=VECTOR('',#20120,2.05474999999998);
#5630=VECTOR('',#20123,2.05474999999998);
#5631=VECTOR('',#20126,2.05474999999998);
#5632=VECTOR('',#20129,2.05474999999998);
#5633=VECTOR('',#20132,2.05474999999998);
#5634=VECTOR('',#20135,2.05474999999998);
#5635=VECTOR('',#20138,2.05474999999998);
#5636=VECTOR('',#20141,2.05474999999998);
#5637=VECTOR('',#20144,2.05474999999998);
#5638=VECTOR('',#20149,2.);
#5639=VECTOR('',#20152,2.);
#5640=VECTOR('',#20157,2.);
#5641=VECTOR('',#20160,2.);
#5642=VECTOR('',#20163,2.);
#5643=VECTOR('',#20166,2.);
#5644=VECTOR('',#20169,2.);
#5645=VECTOR('',#20172,2.);
#5646=VECTOR('',#20175,2.);
#5647=VECTOR('',#20178,2.);
#5648=VECTOR('',#20181,2.);
#5649=VECTOR('',#20184,2.);
#5650=VECTOR('',#20187,2.);
#5651=VECTOR('',#20192,2.05475);
#5652=VECTOR('',#20197,2.05475);
#5653=VECTOR('',#20200,2.05475);
#5654=VECTOR('',#20203,2.05475);
#5655=VECTOR('',#20206,2.05475);
#5656=VECTOR('',#20209,2.05475);
#5657=VECTOR('',#20212,2.05475);
#5658=VECTOR('',#20215,2.05475);
#5659=VECTOR('',#20218,2.05475);
#5660=VECTOR('',#20221,2.05475);
#5661=VECTOR('',#20224,2.05475);
#5662=VECTOR('',#20227,2.05475);
#5663=VECTOR('',#20230,2.05475);
#5664=VECTOR('',#20235,2.);
#5665=VECTOR('',#20238,2.);
#5666=VECTOR('',#20243,2.);
#5667=VECTOR('',#20246,2.);
#5668=VECTOR('',#20249,2.);
#5669=VECTOR('',#20252,2.);
#5670=VECTOR('',#20255,2.);
#5671=VECTOR('',#20258,2.);
#5672=VECTOR('',#20261,2.);
#5673=VECTOR('',#20264,2.);
#5674=VECTOR('',#20267,2.);
#5675=VECTOR('',#20270,2.);
#5676=VECTOR('',#20273,2.);
#5677=VECTOR('',#20278,2.05474999999998);
#5678=VECTOR('',#20283,2.05474999999998);
#5679=VECTOR('',#20286,2.05474999999998);
#5680=VECTOR('',#20289,2.05474999999998);
#5681=VECTOR('',#20292,2.05474999999998);
#5682=VECTOR('',#20295,2.05474999999998);
#5683=VECTOR('',#20298,2.05474999999998);
#5684=VECTOR('',#20301,2.05474999999998);
#5685=VECTOR('',#20304,2.05474999999998);
#5686=VECTOR('',#20307,2.05474999999998);
#5687=VECTOR('',#20310,2.05474999999998);
#5688=VECTOR('',#20313,2.05474999999998);
#5689=VECTOR('',#20316,2.05474999999998);
#5690=VECTOR('',#20321,2.);
#5691=VECTOR('',#20324,2.);
#5692=VECTOR('',#20329,2.);
#5693=VECTOR('',#20332,2.);
#5694=VECTOR('',#20335,2.);
#5695=VECTOR('',#20338,2.);
#5696=VECTOR('',#20341,2.);
#5697=VECTOR('',#20344,2.);
#5698=VECTOR('',#20347,2.);
#5699=VECTOR('',#20350,2.);
#5700=VECTOR('',#20353,2.);
#5701=VECTOR('',#20356,2.);
#5702=VECTOR('',#20359,2.);
#5703=VECTOR('',#20364,2.05474999999998);
#5704=VECTOR('',#20369,2.05474999999998);
#5705=VECTOR('',#20372,2.05474999999998);
#5706=VECTOR('',#20375,2.05474999999998);
#5707=VECTOR('',#20378,2.05474999999998);
#5708=VECTOR('',#20381,2.05474999999998);
#5709=VECTOR('',#20384,2.05474999999998);
#5710=VECTOR('',#20387,2.05474999999998);
#5711=VECTOR('',#20390,2.05474999999998);
#5712=VECTOR('',#20393,2.05474999999998);
#5713=VECTOR('',#20396,2.05474999999998);
#5714=VECTOR('',#20399,2.05474999999998);
#5715=VECTOR('',#20402,2.05474999999998);
#5716=VECTOR('',#20407,2.);
#5717=VECTOR('',#20410,2.);
#5718=VECTOR('',#20415,2.);
#5719=VECTOR('',#20418,2.);
#5720=VECTOR('',#20421,2.);
#5721=VECTOR('',#20424,2.);
#5722=VECTOR('',#20427,2.);
#5723=VECTOR('',#20430,2.);
#5724=VECTOR('',#20433,2.);
#5725=VECTOR('',#20436,2.);
#5726=VECTOR('',#20439,2.);
#5727=VECTOR('',#20442,2.);
#5728=VECTOR('',#20445,2.);
#5729=VECTOR('',#20450,2.05475000000002);
#5730=VECTOR('',#20455,2.05475000000002);
#5731=VECTOR('',#20458,2.05475000000002);
#5732=VECTOR('',#20461,2.05475000000002);
#5733=VECTOR('',#20464,2.05475000000002);
#5734=VECTOR('',#20467,2.05475000000002);
#5735=VECTOR('',#20470,2.05475000000002);
#5736=VECTOR('',#20473,2.05475000000002);
#5737=VECTOR('',#20476,2.05475000000002);
#5738=VECTOR('',#20479,2.05475000000002);
#5739=VECTOR('',#20482,2.05475000000002);
#5740=VECTOR('',#20485,2.05475000000002);
#5741=VECTOR('',#20488,2.05475000000002);
#5742=VECTOR('',#20493,2.);
#5743=VECTOR('',#20496,2.);
#5744=VECTOR('',#20501,2.);
#5745=VECTOR('',#20504,2.);
#5746=VECTOR('',#20507,2.);
#5747=VECTOR('',#20510,2.);
#5748=VECTOR('',#20513,2.);
#5749=VECTOR('',#20516,2.);
#5750=VECTOR('',#20519,2.);
#5751=VECTOR('',#20522,2.);
#5752=VECTOR('',#20525,2.);
#5753=VECTOR('',#20528,2.);
#5754=VECTOR('',#20531,2.);
#5755=VECTOR('',#20536,2.05474999999998);
#5756=VECTOR('',#20541,2.05474999999998);
#5757=VECTOR('',#20544,2.05474999999998);
#5758=VECTOR('',#20547,2.05474999999998);
#5759=VECTOR('',#20550,2.05474999999998);
#5760=VECTOR('',#20553,2.05474999999998);
#5761=VECTOR('',#20556,2.05474999999998);
#5762=VECTOR('',#20559,2.05474999999998);
#5763=VECTOR('',#20562,2.05474999999998);
#5764=VECTOR('',#20565,2.05474999999998);
#5765=VECTOR('',#20568,2.05474999999998);
#5766=VECTOR('',#20571,2.05474999999998);
#5767=VECTOR('',#20574,2.05474999999998);
#5768=VECTOR('',#20579,2.);
#5769=VECTOR('',#20582,2.);
#5770=VECTOR('',#20587,2.);
#5771=VECTOR('',#20590,2.);
#5772=VECTOR('',#20593,2.);
#5773=VECTOR('',#20596,2.);
#5774=VECTOR('',#20599,2.);
#5775=VECTOR('',#20602,2.);
#5776=VECTOR('',#20605,2.);
#5777=VECTOR('',#20608,2.);
#5778=VECTOR('',#20611,2.);
#5779=VECTOR('',#20614,2.);
#5780=VECTOR('',#20617,2.);
#5781=VECTOR('',#20622,2.05475);
#5782=VECTOR('',#20627,2.05475);
#5783=VECTOR('',#20630,2.05475);
#5784=VECTOR('',#20633,2.05475);
#5785=VECTOR('',#20636,2.05475);
#5786=VECTOR('',#20639,2.05475);
#5787=VECTOR('',#20642,2.05475);
#5788=VECTOR('',#20645,2.05475);
#5789=VECTOR('',#20648,2.05475);
#5790=VECTOR('',#20651,2.05475);
#5791=VECTOR('',#20654,2.05475);
#5792=VECTOR('',#20657,2.05475);
#5793=VECTOR('',#20660,2.05475);
#5794=VECTOR('',#20665,2.);
#5795=VECTOR('',#20668,2.);
#5796=VECTOR('',#20673,2.);
#5797=VECTOR('',#20676,2.);
#5798=VECTOR('',#20679,2.);
#5799=VECTOR('',#20682,2.);
#5800=VECTOR('',#20685,2.);
#5801=VECTOR('',#20688,2.);
#5802=VECTOR('',#20691,2.);
#5803=VECTOR('',#20694,2.);
#5804=VECTOR('',#20697,2.);
#5805=VECTOR('',#20700,2.);
#5806=VECTOR('',#20703,2.);
#5807=VECTOR('',#20708,2.05474999999999);
#5808=VECTOR('',#20713,2.05474999999999);
#5809=VECTOR('',#20716,2.05474999999999);
#5810=VECTOR('',#20719,2.05474999999999);
#5811=VECTOR('',#20722,2.05474999999999);
#5812=VECTOR('',#20725,2.05474999999999);
#5813=VECTOR('',#20728,2.05474999999999);
#5814=VECTOR('',#20731,2.05474999999999);
#5815=VECTOR('',#20734,2.05474999999999);
#5816=VECTOR('',#20737,2.05474999999999);
#5817=VECTOR('',#20740,2.05474999999999);
#5818=VECTOR('',#20743,2.05474999999999);
#5819=VECTOR('',#20746,2.05474999999999);
#5820=VECTOR('',#20751,2.);
#5821=VECTOR('',#20754,2.);
#5822=VECTOR('',#20759,2.);
#5823=VECTOR('',#20762,2.);
#5824=VECTOR('',#20765,2.);
#5825=VECTOR('',#20768,2.);
#5826=VECTOR('',#20771,2.);
#5827=VECTOR('',#20774,2.);
#5828=VECTOR('',#20777,2.);
#5829=VECTOR('',#20780,2.);
#5830=VECTOR('',#20783,2.);
#5831=VECTOR('',#20786,2.);
#5832=VECTOR('',#20789,2.);
#5833=VECTOR('',#20794,2.05475);
#5834=VECTOR('',#20799,2.05475);
#5835=VECTOR('',#20802,2.05475);
#5836=VECTOR('',#20805,2.05475);
#5837=VECTOR('',#20808,2.05475);
#5838=VECTOR('',#20811,2.05475);
#5839=VECTOR('',#20814,2.05475);
#5840=VECTOR('',#20817,2.05475);
#5841=VECTOR('',#20820,2.05475);
#5842=VECTOR('',#20823,2.05475);
#5843=VECTOR('',#20826,2.05475);
#5844=VECTOR('',#20829,2.05475);
#5845=VECTOR('',#20832,2.05475);
#5846=VECTOR('',#20837,3.);
#5847=VECTOR('',#20842,3.);
#5848=VECTOR('',#20845,3.);
#5849=VECTOR('',#20848,3.);
#5850=VECTOR('',#20851,3.);
#5851=VECTOR('',#20854,3.);
#5852=VECTOR('',#20857,3.);
#5853=VECTOR('',#20860,3.);
#5854=VECTOR('',#20863,3.07350000000001);
#5855=VECTOR('',#20868,3.07350000000001);
#5856=VECTOR('',#20871,3.07350000000001);
#5857=VECTOR('',#20874,3.07350000000001);
#5858=VECTOR('',#20877,3.07350000000001);
#5859=VECTOR('',#20880,3.07350000000001);
#5860=VECTOR('',#20883,3.07350000000001);
#5861=VECTOR('',#20886,3.07350000000001);
#5862=VECTOR('',#20889,3.);
#5863=VECTOR('',#20894,3.);
#5864=VECTOR('',#20897,3.);
#5865=VECTOR('',#20900,3.);
#5866=VECTOR('',#20903,3.);
#5867=VECTOR('',#20906,3.);
#5868=VECTOR('',#20909,3.);
#5869=VECTOR('',#20912,3.);
#5870=VECTOR('',#20915,3.);
#5871=VECTOR('',#20920,3.);
#5872=VECTOR('',#20923,3.);
#5873=VECTOR('',#20926,3.);
#5874=VECTOR('',#20929,3.);
#5875=VECTOR('',#20932,3.);
#5876=VECTOR('',#20935,3.);
#5877=VECTOR('',#20938,3.);
#5878=VECTOR('',#20941,3.);
#5879=VECTOR('',#20946,3.);
#5880=VECTOR('',#20949,3.);
#5881=VECTOR('',#20952,3.);
#5882=VECTOR('',#20955,3.);
#5883=VECTOR('',#20958,3.);
#5884=VECTOR('',#20961,3.);
#5885=VECTOR('',#20964,3.);
#5886=VECTOR('',#20967,3.07350000000001);
#5887=VECTOR('',#20972,3.07350000000001);
#5888=VECTOR('',#20975,3.07350000000001);
#5889=VECTOR('',#20978,3.07350000000001);
#5890=VECTOR('',#20981,3.07350000000001);
#5891=VECTOR('',#20984,3.07350000000001);
#5892=VECTOR('',#20987,3.07350000000001);
#5893=VECTOR('',#20990,3.07350000000001);
#5894=VECTOR('',#20993,3.0735);
#5895=VECTOR('',#20998,3.0735);
#5896=VECTOR('',#21001,3.0735);
#5897=VECTOR('',#21004,3.0735);
#5898=VECTOR('',#21007,3.0735);
#5899=VECTOR('',#21010,3.0735);
#5900=VECTOR('',#21013,3.0735);
#5901=VECTOR('',#21016,3.0735);
#5902=VECTOR('',#21019,3.0735);
#5903=VECTOR('',#21024,3.0735);
#5904=VECTOR('',#21027,3.0735);
#5905=VECTOR('',#21030,3.0735);
#5906=VECTOR('',#21033,3.0735);
#5907=VECTOR('',#21036,3.0735);
#5908=VECTOR('',#21039,3.0735);
#5909=VECTOR('',#21042,3.0735);
#5910=VECTOR('',#21167,60.);
#5911=VECTOR('',#21174,70.);
#6438=VERTEX_POINT('',#23378);
#6439=VERTEX_POINT('',#23379);
#6440=VERTEX_POINT('',#23381);
#6441=VERTEX_POINT('',#23404);
#6442=VERTEX_POINT('',#23406);
#6443=VERTEX_POINT('',#23414);
#6444=VERTEX_POINT('',#23440);
#6445=VERTEX_POINT('',#23441);
#6446=VERTEX_POINT('',#23491);
#6447=VERTEX_POINT('',#23492);
#6448=VERTEX_POINT('',#23539);
#6449=VERTEX_POINT('',#23540);
#6450=VERTEX_POINT('',#23587);
#6451=VERTEX_POINT('',#23588);
#6452=VERTEX_POINT('',#23638);
#6453=VERTEX_POINT('',#23639);
#6454=VERTEX_POINT('',#23686);
#6455=VERTEX_POINT('',#23687);
#6456=VERTEX_POINT('',#23734);
#6457=VERTEX_POINT('',#23735);
#6458=VERTEX_POINT('',#23785);
#6459=VERTEX_POINT('',#23786);
#6460=VERTEX_POINT('',#23836);
#6461=VERTEX_POINT('',#23837);
#6462=VERTEX_POINT('',#23884);
#6463=VERTEX_POINT('',#23885);
#6464=VERTEX_POINT('',#23935);
#6465=VERTEX_POINT('',#23936);
#6466=VERTEX_POINT('',#23938);
#6467=VERTEX_POINT('',#23952);
#6468=VERTEX_POINT('',#23974);
#6469=VERTEX_POINT('',#23975);
#6470=VERTEX_POINT('',#23977);
#6471=VERTEX_POINT('',#23985);
#6472=VERTEX_POINT('',#23996);
#6473=VERTEX_POINT('',#23997);
#6474=VERTEX_POINT('',#24020);
#6475=VERTEX_POINT('',#24021);
#6476=VERTEX_POINT('',#24045);
#6477=VERTEX_POINT('',#24046);
#6478=VERTEX_POINT('',#24070);
#6479=VERTEX_POINT('',#24071);
#6480=VERTEX_POINT('',#24094);
#6481=VERTEX_POINT('',#24095);
#6482=VERTEX_POINT('',#24119);
#6483=VERTEX_POINT('',#24120);
#6484=VERTEX_POINT('',#24143);
#6485=VERTEX_POINT('',#24144);
#6486=VERTEX_POINT('',#24168);
#6487=VERTEX_POINT('',#24169);
#6488=VERTEX_POINT('',#24192);
#6489=VERTEX_POINT('',#24193);
#6490=VERTEX_POINT('',#24217);
#6491=VERTEX_POINT('',#24218);
#6492=VERTEX_POINT('',#24242);
#6493=VERTEX_POINT('',#24243);
#6494=VERTEX_POINT('',#24266);
#6495=VERTEX_POINT('',#24267);
#6496=VERTEX_POINT('',#24269);
#6497=VERTEX_POINT('',#24275);
#6498=VERTEX_POINT('',#24283);
#6499=VERTEX_POINT('',#24284);
#6500=VERTEX_POINT('',#24286);
#6501=VERTEX_POINT('',#24309);
#6502=VERTEX_POINT('',#24311);
#6503=VERTEX_POINT('',#24319);
#6504=VERTEX_POINT('',#24345);
#6505=VERTEX_POINT('',#24346);
#6506=VERTEX_POINT('',#24396);
#6507=VERTEX_POINT('',#24397);
#6508=VERTEX_POINT('',#24444);
#6509=VERTEX_POINT('',#24445);
#6510=VERTEX_POINT('',#24492);
#6511=VERTEX_POINT('',#24493);
#6512=VERTEX_POINT('',#24543);
#6513=VERTEX_POINT('',#24544);
#6514=VERTEX_POINT('',#24591);
#6515=VERTEX_POINT('',#24592);
#6516=VERTEX_POINT('',#24639);
#6517=VERTEX_POINT('',#24640);
#6518=VERTEX_POINT('',#24690);
#6519=VERTEX_POINT('',#24691);
#6520=VERTEX_POINT('',#24741);
#6521=VERTEX_POINT('',#24742);
#6522=VERTEX_POINT('',#24789);
#6523=VERTEX_POINT('',#24790);
#6524=VERTEX_POINT('',#24840);
#6525=VERTEX_POINT('',#24841);
#6526=VERTEX_POINT('',#24843);
#6527=VERTEX_POINT('',#24857);
#6528=VERTEX_POINT('',#24879);
#6529=VERTEX_POINT('',#24880);
#6530=VERTEX_POINT('',#24882);
#6531=VERTEX_POINT('',#24890);
#6532=VERTEX_POINT('',#24901);
#6533=VERTEX_POINT('',#24902);
#6534=VERTEX_POINT('',#24925);
#6535=VERTEX_POINT('',#24926);
#6536=VERTEX_POINT('',#24950);
#6537=VERTEX_POINT('',#24951);
#6538=VERTEX_POINT('',#24975);
#6539=VERTEX_POINT('',#24976);
#6540=VERTEX_POINT('',#24999);
#6541=VERTEX_POINT('',#25000);
#6542=VERTEX_POINT('',#25024);
#6543=VERTEX_POINT('',#25025);
#6544=VERTEX_POINT('',#25048);
#6545=VERTEX_POINT('',#25049);
#6546=VERTEX_POINT('',#25073);
#6547=VERTEX_POINT('',#25074);
#6548=VERTEX_POINT('',#25097);
#6549=VERTEX_POINT('',#25098);
#6550=VERTEX_POINT('',#25122);
#6551=VERTEX_POINT('',#25123);
#6552=VERTEX_POINT('',#25147);
#6553=VERTEX_POINT('',#25148);
#6554=VERTEX_POINT('',#25171);
#6555=VERTEX_POINT('',#25172);
#6556=VERTEX_POINT('',#25174);
#6557=VERTEX_POINT('',#25180);
#6558=VERTEX_POINT('',#25188);
#6559=VERTEX_POINT('',#25189);
#6560=VERTEX_POINT('',#25191);
#6561=VERTEX_POINT('',#25214);
#6562=VERTEX_POINT('',#25216);
#6563=VERTEX_POINT('',#25224);
#6564=VERTEX_POINT('',#25250);
#6565=VERTEX_POINT('',#25251);
#6566=VERTEX_POINT('',#25301);
#6567=VERTEX_POINT('',#25302);
#6568=VERTEX_POINT('',#25349);
#6569=VERTEX_POINT('',#25350);
#6570=VERTEX_POINT('',#25397);
#6571=VERTEX_POINT('',#25398);
#6572=VERTEX_POINT('',#25448);
#6573=VERTEX_POINT('',#25449);
#6574=VERTEX_POINT('',#25496);
#6575=VERTEX_POINT('',#25497);
#6576=VERTEX_POINT('',#25544);
#6577=VERTEX_POINT('',#25545);
#6578=VERTEX_POINT('',#25595);
#6579=VERTEX_POINT('',#25596);
#6580=VERTEX_POINT('',#25646);
#6581=VERTEX_POINT('',#25647);
#6582=VERTEX_POINT('',#25694);
#6583=VERTEX_POINT('',#25695);
#6584=VERTEX_POINT('',#25745);
#6585=VERTEX_POINT('',#25746);
#6586=VERTEX_POINT('',#25748);
#6587=VERTEX_POINT('',#25762);
#6588=VERTEX_POINT('',#25784);
#6589=VERTEX_POINT('',#25785);
#6590=VERTEX_POINT('',#25787);
#6591=VERTEX_POINT('',#25795);
#6592=VERTEX_POINT('',#25806);
#6593=VERTEX_POINT('',#25807);
#6594=VERTEX_POINT('',#25830);
#6595=VERTEX_POINT('',#25831);
#6596=VERTEX_POINT('',#25855);
#6597=VERTEX_POINT('',#25856);
#6598=VERTEX_POINT('',#25880);
#6599=VERTEX_POINT('',#25881);
#6600=VERTEX_POINT('',#25904);
#6601=VERTEX_POINT('',#25905);
#6602=VERTEX_POINT('',#25929);
#6603=VERTEX_POINT('',#25930);
#6604=VERTEX_POINT('',#25953);
#6605=VERTEX_POINT('',#25954);
#6606=VERTEX_POINT('',#25978);
#6607=VERTEX_POINT('',#25979);
#6608=VERTEX_POINT('',#26002);
#6609=VERTEX_POINT('',#26003);
#6610=VERTEX_POINT('',#26027);
#6611=VERTEX_POINT('',#26028);
#6612=VERTEX_POINT('',#26052);
#6613=VERTEX_POINT('',#26053);
#6614=VERTEX_POINT('',#26076);
#6615=VERTEX_POINT('',#26077);
#6616=VERTEX_POINT('',#26079);
#6617=VERTEX_POINT('',#26085);
#6618=VERTEX_POINT('',#26093);
#6619=VERTEX_POINT('',#26094);
#6620=VERTEX_POINT('',#26096);
#6621=VERTEX_POINT('',#26119);
#6622=VERTEX_POINT('',#26121);
#6623=VERTEX_POINT('',#26129);
#6624=VERTEX_POINT('',#26155);
#6625=VERTEX_POINT('',#26156);
#6626=VERTEX_POINT('',#26206);
#6627=VERTEX_POINT('',#26207);
#6628=VERTEX_POINT('',#26254);
#6629=VERTEX_POINT('',#26255);
#6630=VERTEX_POINT('',#26302);
#6631=VERTEX_POINT('',#26303);
#6632=VERTEX_POINT('',#26353);
#6633=VERTEX_POINT('',#26354);
#6634=VERTEX_POINT('',#26401);
#6635=VERTEX_POINT('',#26402);
#6636=VERTEX_POINT('',#26449);
#6637=VERTEX_POINT('',#26450);
#6638=VERTEX_POINT('',#26500);
#6639=VERTEX_POINT('',#26501);
#6640=VERTEX_POINT('',#26551);
#6641=VERTEX_POINT('',#26552);
#6642=VERTEX_POINT('',#26599);
#6643=VERTEX_POINT('',#26600);
#6644=VERTEX_POINT('',#26650);
#6645=VERTEX_POINT('',#26651);
#6646=VERTEX_POINT('',#26653);
#6647=VERTEX_POINT('',#26667);
#6648=VERTEX_POINT('',#26689);
#6649=VERTEX_POINT('',#26690);
#6650=VERTEX_POINT('',#26692);
#6651=VERTEX_POINT('',#26700);
#6652=VERTEX_POINT('',#26711);
#6653=VERTEX_POINT('',#26712);
#6654=VERTEX_POINT('',#26735);
#6655=VERTEX_POINT('',#26736);
#6656=VERTEX_POINT('',#26760);
#6657=VERTEX_POINT('',#26761);
#6658=VERTEX_POINT('',#26785);
#6659=VERTEX_POINT('',#26786);
#6660=VERTEX_POINT('',#26809);
#6661=VERTEX_POINT('',#26810);
#6662=VERTEX_POINT('',#26834);
#6663=VERTEX_POINT('',#26835);
#6664=VERTEX_POINT('',#26858);
#6665=VERTEX_POINT('',#26859);
#6666=VERTEX_POINT('',#26883);
#6667=VERTEX_POINT('',#26884);
#6668=VERTEX_POINT('',#26907);
#6669=VERTEX_POINT('',#26908);
#6670=VERTEX_POINT('',#26932);
#6671=VERTEX_POINT('',#26933);
#6672=VERTEX_POINT('',#26957);
#6673=VERTEX_POINT('',#26958);
#6674=VERTEX_POINT('',#26981);
#6675=VERTEX_POINT('',#26982);
#6676=VERTEX_POINT('',#26984);
#6677=VERTEX_POINT('',#26990);
#6678=VERTEX_POINT('',#26998);
#6679=VERTEX_POINT('',#26999);
#6680=VERTEX_POINT('',#27001);
#6681=VERTEX_POINT('',#27024);
#6682=VERTEX_POINT('',#27026);
#6683=VERTEX_POINT('',#27034);
#6684=VERTEX_POINT('',#27060);
#6685=VERTEX_POINT('',#27061);
#6686=VERTEX_POINT('',#27111);
#6687=VERTEX_POINT('',#27112);
#6688=VERTEX_POINT('',#27159);
#6689=VERTEX_POINT('',#27160);
#6690=VERTEX_POINT('',#27207);
#6691=VERTEX_POINT('',#27208);
#6692=VERTEX_POINT('',#27258);
#6693=VERTEX_POINT('',#27259);
#6694=VERTEX_POINT('',#27306);
#6695=VERTEX_POINT('',#27307);
#6696=VERTEX_POINT('',#27354);
#6697=VERTEX_POINT('',#27355);
#6698=VERTEX_POINT('',#27405);
#6699=VERTEX_POINT('',#27406);
#6700=VERTEX_POINT('',#27456);
#6701=VERTEX_POINT('',#27457);
#6702=VERTEX_POINT('',#27504);
#6703=VERTEX_POINT('',#27505);
#6704=VERTEX_POINT('',#27555);
#6705=VERTEX_POINT('',#27556);
#6706=VERTEX_POINT('',#27558);
#6707=VERTEX_POINT('',#27572);
#6708=VERTEX_POINT('',#27594);
#6709=VERTEX_POINT('',#27595);
#6710=VERTEX_POINT('',#27597);
#6711=VERTEX_POINT('',#27605);
#6712=VERTEX_POINT('',#27616);
#6713=VERTEX_POINT('',#27617);
#6714=VERTEX_POINT('',#27640);
#6715=VERTEX_POINT('',#27641);
#6716=VERTEX_POINT('',#27665);
#6717=VERTEX_POINT('',#27666);
#6718=VERTEX_POINT('',#27690);
#6719=VERTEX_POINT('',#27691);
#6720=VERTEX_POINT('',#27714);
#6721=VERTEX_POINT('',#27715);
#6722=VERTEX_POINT('',#27739);
#6723=VERTEX_POINT('',#27740);
#6724=VERTEX_POINT('',#27763);
#6725=VERTEX_POINT('',#27764);
#6726=VERTEX_POINT('',#27788);
#6727=VERTEX_POINT('',#27789);
#6728=VERTEX_POINT('',#27812);
#6729=VERTEX_POINT('',#27813);
#6730=VERTEX_POINT('',#27837);
#6731=VERTEX_POINT('',#27838);
#6732=VERTEX_POINT('',#27862);
#6733=VERTEX_POINT('',#27863);
#6734=VERTEX_POINT('',#27886);
#6735=VERTEX_POINT('',#27887);
#6736=VERTEX_POINT('',#27889);
#6737=VERTEX_POINT('',#27895);
#6738=VERTEX_POINT('',#27903);
#6739=VERTEX_POINT('',#27904);
#6740=VERTEX_POINT('',#27906);
#6741=VERTEX_POINT('',#27929);
#6742=VERTEX_POINT('',#27931);
#6743=VERTEX_POINT('',#27939);
#6744=VERTEX_POINT('',#27965);
#6745=VERTEX_POINT('',#27966);
#6746=VERTEX_POINT('',#28016);
#6747=VERTEX_POINT('',#28017);
#6748=VERTEX_POINT('',#28064);
#6749=VERTEX_POINT('',#28065);
#6750=VERTEX_POINT('',#28112);
#6751=VERTEX_POINT('',#28113);
#6752=VERTEX_POINT('',#28163);
#6753=VERTEX_POINT('',#28164);
#6754=VERTEX_POINT('',#28211);
#6755=VERTEX_POINT('',#28212);
#6756=VERTEX_POINT('',#28259);
#6757=VERTEX_POINT('',#28260);
#6758=VERTEX_POINT('',#28310);
#6759=VERTEX_POINT('',#28311);
#6760=VERTEX_POINT('',#28361);
#6761=VERTEX_POINT('',#28362);
#6762=VERTEX_POINT('',#28409);
#6763=VERTEX_POINT('',#28410);
#6764=VERTEX_POINT('',#28460);
#6765=VERTEX_POINT('',#28461);
#6766=VERTEX_POINT('',#28463);
#6767=VERTEX_POINT('',#28477);
#6768=VERTEX_POINT('',#28499);
#6769=VERTEX_POINT('',#28500);
#6770=VERTEX_POINT('',#28502);
#6771=VERTEX_POINT('',#28510);
#6772=VERTEX_POINT('',#28521);
#6773=VERTEX_POINT('',#28522);
#6774=VERTEX_POINT('',#28545);
#6775=VERTEX_POINT('',#28546);
#6776=VERTEX_POINT('',#28570);
#6777=VERTEX_POINT('',#28571);
#6778=VERTEX_POINT('',#28595);
#6779=VERTEX_POINT('',#28596);
#6780=VERTEX_POINT('',#28619);
#6781=VERTEX_POINT('',#28620);
#6782=VERTEX_POINT('',#28644);
#6783=VERTEX_POINT('',#28645);
#6784=VERTEX_POINT('',#28668);
#6785=VERTEX_POINT('',#28669);
#6786=VERTEX_POINT('',#28693);
#6787=VERTEX_POINT('',#28694);
#6788=VERTEX_POINT('',#28717);
#6789=VERTEX_POINT('',#28718);
#6790=VERTEX_POINT('',#28742);
#6791=VERTEX_POINT('',#28743);
#6792=VERTEX_POINT('',#28767);
#6793=VERTEX_POINT('',#28768);
#6794=VERTEX_POINT('',#28791);
#6795=VERTEX_POINT('',#28792);
#6796=VERTEX_POINT('',#28794);
#6797=VERTEX_POINT('',#28800);
#6798=VERTEX_POINT('',#28808);
#6799=VERTEX_POINT('',#28809);
#6800=VERTEX_POINT('',#28811);
#6801=VERTEX_POINT('',#28834);
#6802=VERTEX_POINT('',#28836);
#6803=VERTEX_POINT('',#28844);
#6804=VERTEX_POINT('',#28870);
#6805=VERTEX_POINT('',#28871);
#6806=VERTEX_POINT('',#28921);
#6807=VERTEX_POINT('',#28922);
#6808=VERTEX_POINT('',#28969);
#6809=VERTEX_POINT('',#28970);
#6810=VERTEX_POINT('',#29017);
#6811=VERTEX_POINT('',#29018);
#6812=VERTEX_POINT('',#29068);
#6813=VERTEX_POINT('',#29069);
#6814=VERTEX_POINT('',#29116);
#6815=VERTEX_POINT('',#29117);
#6816=VERTEX_POINT('',#29164);
#6817=VERTEX_POINT('',#29165);
#6818=VERTEX_POINT('',#29215);
#6819=VERTEX_POINT('',#29216);
#6820=VERTEX_POINT('',#29266);
#6821=VERTEX_POINT('',#29267);
#6822=VERTEX_POINT('',#29314);
#6823=VERTEX_POINT('',#29315);
#6824=VERTEX_POINT('',#29365);
#6825=VERTEX_POINT('',#29366);
#6826=VERTEX_POINT('',#29368);
#6827=VERTEX_POINT('',#29382);
#6828=VERTEX_POINT('',#29404);
#6829=VERTEX_POINT('',#29405);
#6830=VERTEX_POINT('',#29407);
#6831=VERTEX_POINT('',#29415);
#6832=VERTEX_POINT('',#29426);
#6833=VERTEX_POINT('',#29427);
#6834=VERTEX_POINT('',#29450);
#6835=VERTEX_POINT('',#29451);
#6836=VERTEX_POINT('',#29475);
#6837=VERTEX_POINT('',#29476);
#6838=VERTEX_POINT('',#29500);
#6839=VERTEX_POINT('',#29501);
#6840=VERTEX_POINT('',#29524);
#6841=VERTEX_POINT('',#29525);
#6842=VERTEX_POINT('',#29549);
#6843=VERTEX_POINT('',#29550);
#6844=VERTEX_POINT('',#29573);
#6845=VERTEX_POINT('',#29574);
#6846=VERTEX_POINT('',#29598);
#6847=VERTEX_POINT('',#29599);
#6848=VERTEX_POINT('',#29622);
#6849=VERTEX_POINT('',#29623);
#6850=VERTEX_POINT('',#29647);
#6851=VERTEX_POINT('',#29648);
#6852=VERTEX_POINT('',#29672);
#6853=VERTEX_POINT('',#29673);
#6854=VERTEX_POINT('',#29696);
#6855=VERTEX_POINT('',#29697);
#6856=VERTEX_POINT('',#29699);
#6857=VERTEX_POINT('',#29705);
#6858=VERTEX_POINT('',#29713);
#6859=VERTEX_POINT('',#29714);
#6860=VERTEX_POINT('',#29716);
#6861=VERTEX_POINT('',#29739);
#6862=VERTEX_POINT('',#29741);
#6863=VERTEX_POINT('',#29749);
#6864=VERTEX_POINT('',#29775);
#6865=VERTEX_POINT('',#29776);
#6866=VERTEX_POINT('',#29826);
#6867=VERTEX_POINT('',#29827);
#6868=VERTEX_POINT('',#29874);
#6869=VERTEX_POINT('',#29875);
#6870=VERTEX_POINT('',#29922);
#6871=VERTEX_POINT('',#29923);
#6872=VERTEX_POINT('',#29973);
#6873=VERTEX_POINT('',#29974);
#6874=VERTEX_POINT('',#30021);
#6875=VERTEX_POINT('',#30022);
#6876=VERTEX_POINT('',#30069);
#6877=VERTEX_POINT('',#30070);
#6878=VERTEX_POINT('',#30120);
#6879=VERTEX_POINT('',#30121);
#6880=VERTEX_POINT('',#30171);
#6881=VERTEX_POINT('',#30172);
#6882=VERTEX_POINT('',#30219);
#6883=VERTEX_POINT('',#30220);
#6884=VERTEX_POINT('',#30270);
#6885=VERTEX_POINT('',#30271);
#6886=VERTEX_POINT('',#30273);
#6887=VERTEX_POINT('',#30287);
#6888=VERTEX_POINT('',#30309);
#6889=VERTEX_POINT('',#30310);
#6890=VERTEX_POINT('',#30312);
#6891=VERTEX_POINT('',#30320);
#6892=VERTEX_POINT('',#30331);
#6893=VERTEX_POINT('',#30332);
#6894=VERTEX_POINT('',#30355);
#6895=VERTEX_POINT('',#30356);
#6896=VERTEX_POINT('',#30380);
#6897=VERTEX_POINT('',#30381);
#6898=VERTEX_POINT('',#30405);
#6899=VERTEX_POINT('',#30406);
#6900=VERTEX_POINT('',#30429);
#6901=VERTEX_POINT('',#30430);
#6902=VERTEX_POINT('',#30454);
#6903=VERTEX_POINT('',#30455);
#6904=VERTEX_POINT('',#30478);
#6905=VERTEX_POINT('',#30479);
#6906=VERTEX_POINT('',#30503);
#6907=VERTEX_POINT('',#30504);
#6908=VERTEX_POINT('',#30527);
#6909=VERTEX_POINT('',#30528);
#6910=VERTEX_POINT('',#30552);
#6911=VERTEX_POINT('',#30553);
#6912=VERTEX_POINT('',#30577);
#6913=VERTEX_POINT('',#30578);
#6914=VERTEX_POINT('',#30601);
#6915=VERTEX_POINT('',#30602);
#6916=VERTEX_POINT('',#30604);
#6917=VERTEX_POINT('',#30610);
#6918=VERTEX_POINT('',#30618);
#6919=VERTEX_POINT('',#30619);
#6920=VERTEX_POINT('',#30621);
#6921=VERTEX_POINT('',#30644);
#6922=VERTEX_POINT('',#30646);
#6923=VERTEX_POINT('',#30654);
#6924=VERTEX_POINT('',#30680);
#6925=VERTEX_POINT('',#30681);
#6926=VERTEX_POINT('',#30731);
#6927=VERTEX_POINT('',#30732);
#6928=VERTEX_POINT('',#30779);
#6929=VERTEX_POINT('',#30780);
#6930=VERTEX_POINT('',#30827);
#6931=VERTEX_POINT('',#30828);
#6932=VERTEX_POINT('',#30878);
#6933=VERTEX_POINT('',#30879);
#6934=VERTEX_POINT('',#30926);
#6935=VERTEX_POINT('',#30927);
#6936=VERTEX_POINT('',#30974);
#6937=VERTEX_POINT('',#30975);
#6938=VERTEX_POINT('',#31025);
#6939=VERTEX_POINT('',#31026);
#6940=VERTEX_POINT('',#31076);
#6941=VERTEX_POINT('',#31077);
#6942=VERTEX_POINT('',#31124);
#6943=VERTEX_POINT('',#31125);
#6944=VERTEX_POINT('',#31175);
#6945=VERTEX_POINT('',#31176);
#6946=VERTEX_POINT('',#31178);
#6947=VERTEX_POINT('',#31192);
#6948=VERTEX_POINT('',#31214);
#6949=VERTEX_POINT('',#31215);
#6950=VERTEX_POINT('',#31217);
#6951=VERTEX_POINT('',#31225);
#6952=VERTEX_POINT('',#31236);
#6953=VERTEX_POINT('',#31237);
#6954=VERTEX_POINT('',#31260);
#6955=VERTEX_POINT('',#31261);
#6956=VERTEX_POINT('',#31285);
#6957=VERTEX_POINT('',#31286);
#6958=VERTEX_POINT('',#31310);
#6959=VERTEX_POINT('',#31311);
#6960=VERTEX_POINT('',#31334);
#6961=VERTEX_POINT('',#31335);
#6962=VERTEX_POINT('',#31359);
#6963=VERTEX_POINT('',#31360);
#6964=VERTEX_POINT('',#31383);
#6965=VERTEX_POINT('',#31384);
#6966=VERTEX_POINT('',#31408);
#6967=VERTEX_POINT('',#31409);
#6968=VERTEX_POINT('',#31432);
#6969=VERTEX_POINT('',#31433);
#6970=VERTEX_POINT('',#31457);
#6971=VERTEX_POINT('',#31458);
#6972=VERTEX_POINT('',#31482);
#6973=VERTEX_POINT('',#31483);
#6974=VERTEX_POINT('',#31506);
#6975=VERTEX_POINT('',#31507);
#6976=VERTEX_POINT('',#31509);
#6977=VERTEX_POINT('',#31515);
#6978=VERTEX_POINT('',#31523);
#6979=VERTEX_POINT('',#31524);
#6980=VERTEX_POINT('',#31526);
#6981=VERTEX_POINT('',#31549);
#6982=VERTEX_POINT('',#31551);
#6983=VERTEX_POINT('',#31559);
#6984=VERTEX_POINT('',#31585);
#6985=VERTEX_POINT('',#31586);
#6986=VERTEX_POINT('',#31636);
#6987=VERTEX_POINT('',#31637);
#6988=VERTEX_POINT('',#31684);
#6989=VERTEX_POINT('',#31685);
#6990=VERTEX_POINT('',#31732);
#6991=VERTEX_POINT('',#31733);
#6992=VERTEX_POINT('',#31783);
#6993=VERTEX_POINT('',#31784);
#6994=VERTEX_POINT('',#31831);
#6995=VERTEX_POINT('',#31832);
#6996=VERTEX_POINT('',#31879);
#6997=VERTEX_POINT('',#31880);
#6998=VERTEX_POINT('',#31930);
#6999=VERTEX_POINT('',#31931);
#7000=VERTEX_POINT('',#31981);
#7001=VERTEX_POINT('',#31982);
#7002=VERTEX_POINT('',#32029);
#7003=VERTEX_POINT('',#32030);
#7004=VERTEX_POINT('',#32080);
#7005=VERTEX_POINT('',#32081);
#7006=VERTEX_POINT('',#32083);
#7007=VERTEX_POINT('',#32097);
#7008=VERTEX_POINT('',#32119);
#7009=VERTEX_POINT('',#32120);
#7010=VERTEX_POINT('',#32122);
#7011=VERTEX_POINT('',#32130);
#7012=VERTEX_POINT('',#32141);
#7013=VERTEX_POINT('',#32142);
#7014=VERTEX_POINT('',#32165);
#7015=VERTEX_POINT('',#32166);
#7016=VERTEX_POINT('',#32190);
#7017=VERTEX_POINT('',#32191);
#7018=VERTEX_POINT('',#32215);
#7019=VERTEX_POINT('',#32216);
#7020=VERTEX_POINT('',#32239);
#7021=VERTEX_POINT('',#32240);
#7022=VERTEX_POINT('',#32264);
#7023=VERTEX_POINT('',#32265);
#7024=VERTEX_POINT('',#32288);
#7025=VERTEX_POINT('',#32289);
#7026=VERTEX_POINT('',#32313);
#7027=VERTEX_POINT('',#32314);
#7028=VERTEX_POINT('',#32337);
#7029=VERTEX_POINT('',#32338);
#7030=VERTEX_POINT('',#32362);
#7031=VERTEX_POINT('',#32363);
#7032=VERTEX_POINT('',#32387);
#7033=VERTEX_POINT('',#32388);
#7034=VERTEX_POINT('',#32411);
#7035=VERTEX_POINT('',#32412);
#7036=VERTEX_POINT('',#32414);
#7037=VERTEX_POINT('',#32420);
#7038=VERTEX_POINT('',#32428);
#7039=VERTEX_POINT('',#32429);
#7040=VERTEX_POINT('',#32431);
#7041=VERTEX_POINT('',#32454);
#7042=VERTEX_POINT('',#32456);
#7043=VERTEX_POINT('',#32464);
#7044=VERTEX_POINT('',#32490);
#7045=VERTEX_POINT('',#32491);
#7046=VERTEX_POINT('',#32541);
#7047=VERTEX_POINT('',#32542);
#7048=VERTEX_POINT('',#32589);
#7049=VERTEX_POINT('',#32590);
#7050=VERTEX_POINT('',#32637);
#7051=VERTEX_POINT('',#32638);
#7052=VERTEX_POINT('',#32688);
#7053=VERTEX_POINT('',#32689);
#7054=VERTEX_POINT('',#32736);
#7055=VERTEX_POINT('',#32737);
#7056=VERTEX_POINT('',#32784);
#7057=VERTEX_POINT('',#32785);
#7058=VERTEX_POINT('',#32835);
#7059=VERTEX_POINT('',#32836);
#7060=VERTEX_POINT('',#32886);
#7061=VERTEX_POINT('',#32887);
#7062=VERTEX_POINT('',#32934);
#7063=VERTEX_POINT('',#32935);
#7064=VERTEX_POINT('',#32985);
#7065=VERTEX_POINT('',#32986);
#7066=VERTEX_POINT('',#32988);
#7067=VERTEX_POINT('',#33002);
#7068=VERTEX_POINT('',#33024);
#7069=VERTEX_POINT('',#33025);
#7070=VERTEX_POINT('',#33027);
#7071=VERTEX_POINT('',#33035);
#7072=VERTEX_POINT('',#33046);
#7073=VERTEX_POINT('',#33047);
#7074=VERTEX_POINT('',#33070);
#7075=VERTEX_POINT('',#33071);
#7076=VERTEX_POINT('',#33095);
#7077=VERTEX_POINT('',#33096);
#7078=VERTEX_POINT('',#33120);
#7079=VERTEX_POINT('',#33121);
#7080=VERTEX_POINT('',#33144);
#7081=VERTEX_POINT('',#33145);
#7082=VERTEX_POINT('',#33169);
#7083=VERTEX_POINT('',#33170);
#7084=VERTEX_POINT('',#33193);
#7085=VERTEX_POINT('',#33194);
#7086=VERTEX_POINT('',#33218);
#7087=VERTEX_POINT('',#33219);
#7088=VERTEX_POINT('',#33242);
#7089=VERTEX_POINT('',#33243);
#7090=VERTEX_POINT('',#33267);
#7091=VERTEX_POINT('',#33268);
#7092=VERTEX_POINT('',#33292);
#7093=VERTEX_POINT('',#33293);
#7094=VERTEX_POINT('',#33316);
#7095=VERTEX_POINT('',#33317);
#7096=VERTEX_POINT('',#33319);
#7097=VERTEX_POINT('',#33325);
#7098=VERTEX_POINT('',#33333);
#7099=VERTEX_POINT('',#33334);
#7100=VERTEX_POINT('',#33336);
#7101=VERTEX_POINT('',#33359);
#7102=VERTEX_POINT('',#33361);
#7103=VERTEX_POINT('',#33369);
#7104=VERTEX_POINT('',#33395);
#7105=VERTEX_POINT('',#33396);
#7106=VERTEX_POINT('',#33446);
#7107=VERTEX_POINT('',#33447);
#7108=VERTEX_POINT('',#33494);
#7109=VERTEX_POINT('',#33495);
#7110=VERTEX_POINT('',#33542);
#7111=VERTEX_POINT('',#33543);
#7112=VERTEX_POINT('',#33593);
#7113=VERTEX_POINT('',#33594);
#7114=VERTEX_POINT('',#33641);
#7115=VERTEX_POINT('',#33642);
#7116=VERTEX_POINT('',#33689);
#7117=VERTEX_POINT('',#33690);
#7118=VERTEX_POINT('',#33740);
#7119=VERTEX_POINT('',#33741);
#7120=VERTEX_POINT('',#33791);
#7121=VERTEX_POINT('',#33792);
#7122=VERTEX_POINT('',#33839);
#7123=VERTEX_POINT('',#33840);
#7124=VERTEX_POINT('',#33890);
#7125=VERTEX_POINT('',#33891);
#7126=VERTEX_POINT('',#33893);
#7127=VERTEX_POINT('',#33907);
#7128=VERTEX_POINT('',#33929);
#7129=VERTEX_POINT('',#33930);
#7130=VERTEX_POINT('',#33932);
#7131=VERTEX_POINT('',#33940);
#7132=VERTEX_POINT('',#33951);
#7133=VERTEX_POINT('',#33952);
#7134=VERTEX_POINT('',#33975);
#7135=VERTEX_POINT('',#33976);
#7136=VERTEX_POINT('',#34000);
#7137=VERTEX_POINT('',#34001);
#7138=VERTEX_POINT('',#34025);
#7139=VERTEX_POINT('',#34026);
#7140=VERTEX_POINT('',#34049);
#7141=VERTEX_POINT('',#34050);
#7142=VERTEX_POINT('',#34074);
#7143=VERTEX_POINT('',#34075);
#7144=VERTEX_POINT('',#34098);
#7145=VERTEX_POINT('',#34099);
#7146=VERTEX_POINT('',#34123);
#7147=VERTEX_POINT('',#34124);
#7148=VERTEX_POINT('',#34147);
#7149=VERTEX_POINT('',#34148);
#7150=VERTEX_POINT('',#34172);
#7151=VERTEX_POINT('',#34173);
#7152=VERTEX_POINT('',#34197);
#7153=VERTEX_POINT('',#34198);
#7154=VERTEX_POINT('',#34221);
#7155=VERTEX_POINT('',#34222);
#7156=VERTEX_POINT('',#34224);
#7157=VERTEX_POINT('',#34230);
#7158=VERTEX_POINT('',#34238);
#7159=VERTEX_POINT('',#34239);
#7160=VERTEX_POINT('',#34241);
#7161=VERTEX_POINT('',#34246);
#7162=VERTEX_POINT('',#34259);
#7163=VERTEX_POINT('',#34260);
#7164=VERTEX_POINT('',#34310);
#7165=VERTEX_POINT('',#34311);
#7166=VERTEX_POINT('',#34361);
#7167=VERTEX_POINT('',#34362);
#7168=VERTEX_POINT('',#34409);
#7169=VERTEX_POINT('',#34410);
#7170=VERTEX_POINT('',#34463);
#7171=VERTEX_POINT('',#34464);
#7172=VERTEX_POINT('',#34511);
#7173=VERTEX_POINT('',#34512);
#7174=VERTEX_POINT('',#34559);
#7175=VERTEX_POINT('',#34560);
#7176=VERTEX_POINT('',#34562);
#7177=VERTEX_POINT('',#34576);
#7178=VERTEX_POINT('',#34609);
#7179=VERTEX_POINT('',#34610);
#7180=VERTEX_POINT('',#34612);
#7181=VERTEX_POINT('',#34621);
#7182=VERTEX_POINT('',#34633);
#7183=VERTEX_POINT('',#34634);
#7184=VERTEX_POINT('',#34657);
#7185=VERTEX_POINT('',#34658);
#7186=VERTEX_POINT('',#34682);
#7187=VERTEX_POINT('',#34683);
#7188=VERTEX_POINT('',#34707);
#7189=VERTEX_POINT('',#34708);
#7190=VERTEX_POINT('',#34732);
#7191=VERTEX_POINT('',#34733);
#7192=VERTEX_POINT('',#34756);
#7193=VERTEX_POINT('',#34757);
#7194=VERTEX_POINT('',#34781);
#7195=VERTEX_POINT('',#34782);
#7196=VERTEX_POINT('',#34784);
#7197=VERTEX_POINT('',#34790);
#7198=VERTEX_POINT('',#34795);
#7199=VERTEX_POINT('',#34807);
#7200=VERTEX_POINT('',#34808);
#7201=VERTEX_POINT('',#34810);
#7202=VERTEX_POINT('',#34815);
#7203=VERTEX_POINT('',#34828);
#7204=VERTEX_POINT('',#34829);
#7205=VERTEX_POINT('',#34879);
#7206=VERTEX_POINT('',#34880);
#7207=VERTEX_POINT('',#34930);
#7208=VERTEX_POINT('',#34931);
#7209=VERTEX_POINT('',#34978);
#7210=VERTEX_POINT('',#34979);
#7211=VERTEX_POINT('',#35032);
#7212=VERTEX_POINT('',#35033);
#7213=VERTEX_POINT('',#35080);
#7214=VERTEX_POINT('',#35081);
#7215=VERTEX_POINT('',#35128);
#7216=VERTEX_POINT('',#35129);
#7217=VERTEX_POINT('',#35131);
#7218=VERTEX_POINT('',#35145);
#7219=VERTEX_POINT('',#35178);
#7220=VERTEX_POINT('',#35179);
#7221=VERTEX_POINT('',#35181);
#7222=VERTEX_POINT('',#35186);
#7223=VERTEX_POINT('',#35199);
#7224=VERTEX_POINT('',#35200);
#7225=VERTEX_POINT('',#35250);
#7226=VERTEX_POINT('',#35251);
#7227=VERTEX_POINT('',#35301);
#7228=VERTEX_POINT('',#35302);
#7229=VERTEX_POINT('',#35349);
#7230=VERTEX_POINT('',#35350);
#7231=VERTEX_POINT('',#35403);
#7232=VERTEX_POINT('',#35404);
#7233=VERTEX_POINT('',#35451);
#7234=VERTEX_POINT('',#35452);
#7235=VERTEX_POINT('',#35499);
#7236=VERTEX_POINT('',#35500);
#7237=VERTEX_POINT('',#35502);
#7238=VERTEX_POINT('',#35516);
#7239=VERTEX_POINT('',#35549);
#7240=VERTEX_POINT('',#35550);
#7241=VERTEX_POINT('',#35552);
#7242=VERTEX_POINT('',#35557);
#7243=VERTEX_POINT('',#35570);
#7244=VERTEX_POINT('',#35571);
#7245=VERTEX_POINT('',#35621);
#7246=VERTEX_POINT('',#35622);
#7247=VERTEX_POINT('',#35672);
#7248=VERTEX_POINT('',#35673);
#7249=VERTEX_POINT('',#35720);
#7250=VERTEX_POINT('',#35721);
#7251=VERTEX_POINT('',#35774);
#7252=VERTEX_POINT('',#35775);
#7253=VERTEX_POINT('',#35822);
#7254=VERTEX_POINT('',#35823);
#7255=VERTEX_POINT('',#35870);
#7256=VERTEX_POINT('',#35871);
#7257=VERTEX_POINT('',#35873);
#7258=VERTEX_POINT('',#35887);
#7259=VERTEX_POINT('',#35920);
#7260=VERTEX_POINT('',#35921);
#7261=VERTEX_POINT('',#35923);
#7262=VERTEX_POINT('',#35932);
#7263=VERTEX_POINT('',#35944);
#7264=VERTEX_POINT('',#35945);
#7265=VERTEX_POINT('',#35968);
#7266=VERTEX_POINT('',#35969);
#7267=VERTEX_POINT('',#35993);
#7268=VERTEX_POINT('',#35994);
#7269=VERTEX_POINT('',#36018);
#7270=VERTEX_POINT('',#36019);
#7271=VERTEX_POINT('',#36043);
#7272=VERTEX_POINT('',#36044);
#7273=VERTEX_POINT('',#36067);
#7274=VERTEX_POINT('',#36068);
#7275=VERTEX_POINT('',#36092);
#7276=VERTEX_POINT('',#36093);
#7277=VERTEX_POINT('',#36095);
#7278=VERTEX_POINT('',#36101);
#7279=VERTEX_POINT('',#36106);
#7280=VERTEX_POINT('',#36118);
#7281=VERTEX_POINT('',#36119);
#7282=VERTEX_POINT('',#36121);
#7283=VERTEX_POINT('',#36130);
#7284=VERTEX_POINT('',#36142);
#7285=VERTEX_POINT('',#36143);
#7286=VERTEX_POINT('',#36166);
#7287=VERTEX_POINT('',#36167);
#7288=VERTEX_POINT('',#36191);
#7289=VERTEX_POINT('',#36192);
#7290=VERTEX_POINT('',#36216);
#7291=VERTEX_POINT('',#36217);
#7292=VERTEX_POINT('',#36241);
#7293=VERTEX_POINT('',#36242);
#7294=VERTEX_POINT('',#36265);
#7295=VERTEX_POINT('',#36266);
#7296=VERTEX_POINT('',#36290);
#7297=VERTEX_POINT('',#36291);
#7298=VERTEX_POINT('',#36293);
#7299=VERTEX_POINT('',#36299);
#7300=VERTEX_POINT('',#36304);
#7301=VERTEX_POINT('',#36316);
#7302=VERTEX_POINT('',#36317);
#7303=VERTEX_POINT('',#36319);
#7304=VERTEX_POINT('',#36328);
#7305=VERTEX_POINT('',#36340);
#7306=VERTEX_POINT('',#36341);
#7307=VERTEX_POINT('',#36364);
#7308=VERTEX_POINT('',#36365);
#7309=VERTEX_POINT('',#36389);
#7310=VERTEX_POINT('',#36390);
#7311=VERTEX_POINT('',#36414);
#7312=VERTEX_POINT('',#36415);
#7313=VERTEX_POINT('',#36439);
#7314=VERTEX_POINT('',#36440);
#7315=VERTEX_POINT('',#36463);
#7316=VERTEX_POINT('',#36464);
#7317=VERTEX_POINT('',#36488);
#7318=VERTEX_POINT('',#36489);
#7319=VERTEX_POINT('',#36491);
#7320=VERTEX_POINT('',#36497);
#7321=VERTEX_POINT('',#36502);
#7322=VERTEX_POINT('',#52658);
#7323=VERTEX_POINT('',#52660);
#7324=VERTEX_POINT('',#52664);
#7325=VERTEX_POINT('',#52666);
#8261=EDGE_CURVE('',#6438,#6439,#4630,.T.);
#8262=EDGE_CURVE('',#6439,#6440,#3113,.T.);
#8263=EDGE_CURVE('',#6440,#6441,#2777,.T.);
#8264=EDGE_CURVE('',#6441,#6442,#3114,.T.);
#8265=EDGE_CURVE('',#6442,#6443,#4631,.T.);
#8266=EDGE_CURVE('',#6443,#6443,#2778,.F.);
#8267=EDGE_CURVE('',#6442,#6438,#3115,.T.);
#8268=EDGE_CURVE('',#6444,#6445,#4632,.T.);
#8269=EDGE_CURVE('',#6445,#6439,#3116,.T.);
#8270=EDGE_CURVE('',#6438,#6444,#3117,.T.);
#8271=EDGE_CURVE('',#6446,#6447,#4633,.T.);
#8272=EDGE_CURVE('',#6447,#6445,#3118,.T.);
#8273=EDGE_CURVE('',#6444,#6446,#3119,.T.);
#8274=EDGE_CURVE('',#6448,#6449,#4634,.T.);
#8275=EDGE_CURVE('',#6449,#6447,#3120,.T.);
#8276=EDGE_CURVE('',#6446,#6448,#3121,.T.);
#8277=EDGE_CURVE('',#6450,#6451,#4635,.T.);
#8278=EDGE_CURVE('',#6451,#6449,#3122,.T.);
#8279=EDGE_CURVE('',#6448,#6450,#3123,.T.);
#8280=EDGE_CURVE('',#6452,#6453,#4636,.T.);
#8281=EDGE_CURVE('',#6453,#6451,#3124,.T.);
#8282=EDGE_CURVE('',#6450,#6452,#3125,.T.);
#8283=EDGE_CURVE('',#6454,#6455,#4637,.T.);
#8284=EDGE_CURVE('',#6455,#6453,#3126,.T.);
#8285=EDGE_CURVE('',#6452,#6454,#3127,.T.);
#8286=EDGE_CURVE('',#6456,#6457,#4638,.T.);
#8287=EDGE_CURVE('',#6457,#6455,#3128,.T.);
#8288=EDGE_CURVE('',#6454,#6456,#3129,.T.);
#8289=EDGE_CURVE('',#6458,#6459,#4639,.T.);
#8290=EDGE_CURVE('',#6459,#6457,#3130,.T.);
#8291=EDGE_CURVE('',#6456,#6458,#3131,.T.);
#8292=EDGE_CURVE('',#6460,#6461,#4640,.T.);
#8293=EDGE_CURVE('',#6461,#6459,#3132,.T.);
#8294=EDGE_CURVE('',#6458,#6460,#3133,.T.);
#8295=EDGE_CURVE('',#6462,#6463,#4641,.T.);
#8296=EDGE_CURVE('',#6463,#6461,#3134,.T.);
#8297=EDGE_CURVE('',#6460,#6462,#3135,.T.);
#8298=EDGE_CURVE('',#6464,#6465,#4642,.T.);
#8299=EDGE_CURVE('',#6464,#6466,#3136,.T.);
#8300=EDGE_CURVE('',#6467,#6466,#2779,.T.);
#8301=EDGE_CURVE('',#6467,#6465,#3137,.T.);
#8302=EDGE_CURVE('',#6468,#6469,#4643,.T.);
#8303=EDGE_CURVE('',#6469,#6470,#3138,.T.);
#8304=EDGE_CURVE('',#6471,#6470,#2780,.T.);
#8305=EDGE_CURVE('',#6468,#6471,#3139,.T.);
#8306=EDGE_CURVE('',#6472,#6473,#4644,.T.);
#8307=EDGE_CURVE('',#6473,#6469,#3140,.T.);
#8308=EDGE_CURVE('',#6472,#6468,#3141,.T.);
#8309=EDGE_CURVE('',#6474,#6475,#4645,.T.);
#8310=EDGE_CURVE('',#6475,#6473,#3142,.T.);
#8311=EDGE_CURVE('',#6474,#6472,#3143,.T.);
#8312=EDGE_CURVE('',#6476,#6477,#4646,.T.);
#8313=EDGE_CURVE('',#6477,#6475,#3144,.T.);
#8314=EDGE_CURVE('',#6476,#6474,#3145,.T.);
#8315=EDGE_CURVE('',#6478,#6479,#4647,.T.);
#8316=EDGE_CURVE('',#6479,#6477,#3146,.T.);
#8317=EDGE_CURVE('',#6478,#6476,#3147,.T.);
#8318=EDGE_CURVE('',#6480,#6481,#4648,.T.);
#8319=EDGE_CURVE('',#6481,#6479,#3148,.T.);
#8320=EDGE_CURVE('',#6480,#6478,#3149,.T.);
#8321=EDGE_CURVE('',#6482,#6483,#4649,.T.);
#8322=EDGE_CURVE('',#6483,#6481,#3150,.T.);
#8323=EDGE_CURVE('',#6482,#6480,#3151,.T.);
#8324=EDGE_CURVE('',#6484,#6485,#4650,.T.);
#8325=EDGE_CURVE('',#6485,#6483,#3152,.T.);
#8326=EDGE_CURVE('',#6484,#6482,#3153,.T.);
#8327=EDGE_CURVE('',#6486,#6487,#4651,.T.);
#8328=EDGE_CURVE('',#6487,#6485,#3154,.T.);
#8329=EDGE_CURVE('',#6486,#6484,#3155,.T.);
#8330=EDGE_CURVE('',#6488,#6489,#4652,.T.);
#8331=EDGE_CURVE('',#6489,#6487,#3156,.T.);
#8332=EDGE_CURVE('',#6488,#6486,#3157,.T.);
#8333=EDGE_CURVE('',#6490,#6491,#4653,.T.);
#8334=EDGE_CURVE('',#6491,#6489,#3158,.T.);
#8335=EDGE_CURVE('',#6490,#6488,#3159,.T.);
#8336=EDGE_CURVE('',#6492,#6493,#4654,.T.);
#8337=EDGE_CURVE('',#6493,#6491,#3160,.T.);
#8338=EDGE_CURVE('',#6492,#6490,#3161,.T.);
#8339=EDGE_CURVE('',#6494,#6495,#4655,.T.);
#8340=EDGE_CURVE('',#6496,#6494,#3162,.T.);
#8341=EDGE_CURVE('',#6497,#6496,#2781,.T.);
#8342=EDGE_CURVE('',#6497,#6495,#3163,.T.);
#8343=EDGE_CURVE('',#6498,#6499,#4656,.T.);
#8344=EDGE_CURVE('',#6499,#6500,#3164,.T.);
#8345=EDGE_CURVE('',#6500,#6501,#2782,.T.);
#8346=EDGE_CURVE('',#6501,#6502,#3165,.T.);
#8347=EDGE_CURVE('',#6502,#6503,#4657,.T.);
#8348=EDGE_CURVE('',#6503,#6503,#2783,.F.);
#8349=EDGE_CURVE('',#6502,#6498,#3166,.T.);
#8350=EDGE_CURVE('',#6504,#6505,#4658,.T.);
#8351=EDGE_CURVE('',#6505,#6499,#3167,.T.);
#8352=EDGE_CURVE('',#6498,#6504,#3168,.T.);
#8353=EDGE_CURVE('',#6506,#6507,#4659,.T.);
#8354=EDGE_CURVE('',#6507,#6505,#3169,.T.);
#8355=EDGE_CURVE('',#6504,#6506,#3170,.T.);
#8356=EDGE_CURVE('',#6508,#6509,#4660,.T.);
#8357=EDGE_CURVE('',#6509,#6507,#3171,.T.);
#8358=EDGE_CURVE('',#6506,#6508,#3172,.T.);
#8359=EDGE_CURVE('',#6510,#6511,#4661,.T.);
#8360=EDGE_CURVE('',#6511,#6509,#3173,.T.);
#8361=EDGE_CURVE('',#6508,#6510,#3174,.T.);
#8362=EDGE_CURVE('',#6512,#6513,#4662,.T.);
#8363=EDGE_CURVE('',#6513,#6511,#3175,.T.);
#8364=EDGE_CURVE('',#6510,#6512,#3176,.T.);
#8365=EDGE_CURVE('',#6514,#6515,#4663,.T.);
#8366=EDGE_CURVE('',#6515,#6513,#3177,.T.);
#8367=EDGE_CURVE('',#6512,#6514,#3178,.T.);
#8368=EDGE_CURVE('',#6516,#6517,#4664,.T.);
#8369=EDGE_CURVE('',#6517,#6515,#3179,.T.);
#8370=EDGE_CURVE('',#6514,#6516,#3180,.T.);
#8371=EDGE_CURVE('',#6518,#6519,#4665,.T.);
#8372=EDGE_CURVE('',#6519,#6517,#3181,.T.);
#8373=EDGE_CURVE('',#6516,#6518,#3182,.T.);
#8374=EDGE_CURVE('',#6520,#6521,#4666,.T.);
#8375=EDGE_CURVE('',#6521,#6519,#3183,.T.);
#8376=EDGE_CURVE('',#6518,#6520,#3184,.T.);
#8377=EDGE_CURVE('',#6522,#6523,#4667,.T.);
#8378=EDGE_CURVE('',#6523,#6521,#3185,.T.);
#8379=EDGE_CURVE('',#6520,#6522,#3186,.T.);
#8380=EDGE_CURVE('',#6524,#6525,#4668,.T.);
#8381=EDGE_CURVE('',#6524,#6526,#3187,.T.);
#8382=EDGE_CURVE('',#6527,#6526,#2784,.F.);
#8383=EDGE_CURVE('',#6527,#6525,#3188,.T.);
#8384=EDGE_CURVE('',#6528,#6529,#4669,.T.);
#8385=EDGE_CURVE('',#6529,#6530,#3189,.T.);
#8386=EDGE_CURVE('',#6531,#6530,#2785,.T.);
#8387=EDGE_CURVE('',#6528,#6531,#3190,.T.);
#8388=EDGE_CURVE('',#6532,#6533,#4670,.T.);
#8389=EDGE_CURVE('',#6533,#6529,#3191,.T.);
#8390=EDGE_CURVE('',#6532,#6528,#3192,.T.);
#8391=EDGE_CURVE('',#6534,#6535,#4671,.T.);
#8392=EDGE_CURVE('',#6535,#6533,#3193,.T.);
#8393=EDGE_CURVE('',#6534,#6532,#3194,.T.);
#8394=EDGE_CURVE('',#6536,#6537,#4672,.T.);
#8395=EDGE_CURVE('',#6537,#6535,#3195,.T.);
#8396=EDGE_CURVE('',#6536,#6534,#3196,.T.);
#8397=EDGE_CURVE('',#6538,#6539,#4673,.T.);
#8398=EDGE_CURVE('',#6539,#6537,#3197,.T.);
#8399=EDGE_CURVE('',#6538,#6536,#3198,.T.);
#8400=EDGE_CURVE('',#6540,#6541,#4674,.T.);
#8401=EDGE_CURVE('',#6541,#6539,#3199,.T.);
#8402=EDGE_CURVE('',#6540,#6538,#3200,.T.);
#8403=EDGE_CURVE('',#6542,#6543,#4675,.T.);
#8404=EDGE_CURVE('',#6543,#6541,#3201,.T.);
#8405=EDGE_CURVE('',#6542,#6540,#3202,.T.);
#8406=EDGE_CURVE('',#6544,#6545,#4676,.T.);
#8407=EDGE_CURVE('',#6545,#6543,#3203,.T.);
#8408=EDGE_CURVE('',#6544,#6542,#3204,.T.);
#8409=EDGE_CURVE('',#6546,#6547,#4677,.T.);
#8410=EDGE_CURVE('',#6547,#6545,#3205,.T.);
#8411=EDGE_CURVE('',#6546,#6544,#3206,.T.);
#8412=EDGE_CURVE('',#6548,#6549,#4678,.T.);
#8413=EDGE_CURVE('',#6549,#6547,#3207,.T.);
#8414=EDGE_CURVE('',#6548,#6546,#3208,.T.);
#8415=EDGE_CURVE('',#6550,#6551,#4679,.T.);
#8416=EDGE_CURVE('',#6551,#6549,#3209,.T.);
#8417=EDGE_CURVE('',#6550,#6548,#3210,.T.);
#8418=EDGE_CURVE('',#6552,#6553,#4680,.T.);
#8419=EDGE_CURVE('',#6553,#6551,#3211,.T.);
#8420=EDGE_CURVE('',#6552,#6550,#3212,.T.);
#8421=EDGE_CURVE('',#6554,#6555,#4681,.T.);
#8422=EDGE_CURVE('',#6556,#6554,#3213,.T.);
#8423=EDGE_CURVE('',#6557,#6556,#2786,.T.);
#8424=EDGE_CURVE('',#6557,#6555,#3214,.T.);
#8425=EDGE_CURVE('',#6558,#6559,#4682,.T.);
#8426=EDGE_CURVE('',#6559,#6560,#3215,.T.);
#8427=EDGE_CURVE('',#6560,#6561,#2787,.T.);
#8428=EDGE_CURVE('',#6561,#6562,#3216,.T.);
#8429=EDGE_CURVE('',#6562,#6563,#4683,.T.);
#8430=EDGE_CURVE('',#6563,#6563,#2788,.F.);
#8431=EDGE_CURVE('',#6562,#6558,#3217,.T.);
#8432=EDGE_CURVE('',#6564,#6565,#4684,.T.);
#8433=EDGE_CURVE('',#6565,#6559,#3218,.T.);
#8434=EDGE_CURVE('',#6558,#6564,#3219,.T.);
#8435=EDGE_CURVE('',#6566,#6567,#4685,.T.);
#8436=EDGE_CURVE('',#6567,#6565,#3220,.T.);
#8437=EDGE_CURVE('',#6564,#6566,#3221,.T.);
#8438=EDGE_CURVE('',#6568,#6569,#4686,.T.);
#8439=EDGE_CURVE('',#6569,#6567,#3222,.T.);
#8440=EDGE_CURVE('',#6566,#6568,#3223,.T.);
#8441=EDGE_CURVE('',#6570,#6571,#4687,.T.);
#8442=EDGE_CURVE('',#6571,#6569,#3224,.T.);
#8443=EDGE_CURVE('',#6568,#6570,#3225,.T.);
#8444=EDGE_CURVE('',#6572,#6573,#4688,.T.);
#8445=EDGE_CURVE('',#6573,#6571,#3226,.T.);
#8446=EDGE_CURVE('',#6570,#6572,#3227,.T.);
#8447=EDGE_CURVE('',#6574,#6575,#4689,.T.);
#8448=EDGE_CURVE('',#6575,#6573,#3228,.T.);
#8449=EDGE_CURVE('',#6572,#6574,#3229,.T.);
#8450=EDGE_CURVE('',#6576,#6577,#4690,.T.);
#8451=EDGE_CURVE('',#6577,#6575,#3230,.T.);
#8452=EDGE_CURVE('',#6574,#6576,#3231,.T.);
#8453=EDGE_CURVE('',#6578,#6579,#4691,.T.);
#8454=EDGE_CURVE('',#6579,#6577,#3232,.T.);
#8455=EDGE_CURVE('',#6576,#6578,#3233,.T.);
#8456=EDGE_CURVE('',#6580,#6581,#4692,.T.);
#8457=EDGE_CURVE('',#6581,#6579,#3234,.T.);
#8458=EDGE_CURVE('',#6578,#6580,#3235,.T.);
#8459=EDGE_CURVE('',#6582,#6583,#4693,.T.);
#8460=EDGE_CURVE('',#6583,#6581,#3236,.T.);
#8461=EDGE_CURVE('',#6580,#6582,#3237,.T.);
#8462=EDGE_CURVE('',#6584,#6585,#4694,.T.);
#8463=EDGE_CURVE('',#6584,#6586,#3238,.T.);
#8464=EDGE_CURVE('',#6587,#6586,#2789,.T.);
#8465=EDGE_CURVE('',#6587,#6585,#3239,.T.);
#8466=EDGE_CURVE('',#6588,#6589,#4695,.T.);
#8467=EDGE_CURVE('',#6589,#6590,#3240,.T.);
#8468=EDGE_CURVE('',#6591,#6590,#2790,.T.);
#8469=EDGE_CURVE('',#6588,#6591,#3241,.T.);
#8470=EDGE_CURVE('',#6592,#6593,#4696,.T.);
#8471=EDGE_CURVE('',#6593,#6589,#3242,.T.);
#8472=EDGE_CURVE('',#6592,#6588,#3243,.T.);
#8473=EDGE_CURVE('',#6594,#6595,#4697,.T.);
#8474=EDGE_CURVE('',#6595,#6593,#3244,.T.);
#8475=EDGE_CURVE('',#6594,#6592,#3245,.T.);
#8476=EDGE_CURVE('',#6596,#6597,#4698,.T.);
#8477=EDGE_CURVE('',#6597,#6595,#3246,.T.);
#8478=EDGE_CURVE('',#6596,#6594,#3247,.T.);
#8479=EDGE_CURVE('',#6598,#6599,#4699,.T.);
#8480=EDGE_CURVE('',#6599,#6597,#3248,.T.);
#8481=EDGE_CURVE('',#6598,#6596,#3249,.T.);
#8482=EDGE_CURVE('',#6600,#6601,#4700,.T.);
#8483=EDGE_CURVE('',#6601,#6599,#3250,.T.);
#8484=EDGE_CURVE('',#6600,#6598,#3251,.T.);
#8485=EDGE_CURVE('',#6602,#6603,#4701,.T.);
#8486=EDGE_CURVE('',#6603,#6601,#3252,.T.);
#8487=EDGE_CURVE('',#6602,#6600,#3253,.T.);
#8488=EDGE_CURVE('',#6604,#6605,#4702,.T.);
#8489=EDGE_CURVE('',#6605,#6603,#3254,.T.);
#8490=EDGE_CURVE('',#6604,#6602,#3255,.T.);
#8491=EDGE_CURVE('',#6606,#6607,#4703,.T.);
#8492=EDGE_CURVE('',#6607,#6605,#3256,.T.);
#8493=EDGE_CURVE('',#6606,#6604,#3257,.T.);
#8494=EDGE_CURVE('',#6608,#6609,#4704,.T.);
#8495=EDGE_CURVE('',#6609,#6607,#3258,.T.);
#8496=EDGE_CURVE('',#6608,#6606,#3259,.T.);
#8497=EDGE_CURVE('',#6610,#6611,#4705,.T.);
#8498=EDGE_CURVE('',#6611,#6609,#3260,.T.);
#8499=EDGE_CURVE('',#6610,#6608,#3261,.T.);
#8500=EDGE_CURVE('',#6612,#6613,#4706,.T.);
#8501=EDGE_CURVE('',#6613,#6611,#3262,.T.);
#8502=EDGE_CURVE('',#6612,#6610,#3263,.T.);
#8503=EDGE_CURVE('',#6614,#6615,#4707,.T.);
#8504=EDGE_CURVE('',#6616,#6614,#3264,.T.);
#8505=EDGE_CURVE('',#6617,#6616,#2791,.T.);
#8506=EDGE_CURVE('',#6617,#6615,#3265,.T.);
#8507=EDGE_CURVE('',#6618,#6619,#4708,.T.);
#8508=EDGE_CURVE('',#6619,#6620,#3266,.T.);
#8509=EDGE_CURVE('',#6620,#6621,#2792,.T.);
#8510=EDGE_CURVE('',#6621,#6622,#3267,.T.);
#8511=EDGE_CURVE('',#6622,#6623,#4709,.T.);
#8512=EDGE_CURVE('',#6623,#6623,#2793,.F.);
#8513=EDGE_CURVE('',#6622,#6618,#3268,.T.);
#8514=EDGE_CURVE('',#6624,#6625,#4710,.T.);
#8515=EDGE_CURVE('',#6625,#6619,#3269,.T.);
#8516=EDGE_CURVE('',#6618,#6624,#3270,.T.);
#8517=EDGE_CURVE('',#6626,#6627,#4711,.T.);
#8518=EDGE_CURVE('',#6627,#6625,#3271,.T.);
#8519=EDGE_CURVE('',#6624,#6626,#3272,.T.);
#8520=EDGE_CURVE('',#6628,#6629,#4712,.T.);
#8521=EDGE_CURVE('',#6629,#6627,#3273,.T.);
#8522=EDGE_CURVE('',#6626,#6628,#3274,.T.);
#8523=EDGE_CURVE('',#6630,#6631,#4713,.T.);
#8524=EDGE_CURVE('',#6631,#6629,#3275,.T.);
#8525=EDGE_CURVE('',#6628,#6630,#3276,.T.);
#8526=EDGE_CURVE('',#6632,#6633,#4714,.T.);
#8527=EDGE_CURVE('',#6633,#6631,#3277,.T.);
#8528=EDGE_CURVE('',#6630,#6632,#3278,.T.);
#8529=EDGE_CURVE('',#6634,#6635,#4715,.T.);
#8530=EDGE_CURVE('',#6635,#6633,#3279,.T.);
#8531=EDGE_CURVE('',#6632,#6634,#3280,.T.);
#8532=EDGE_CURVE('',#6636,#6637,#4716,.T.);
#8533=EDGE_CURVE('',#6637,#6635,#3281,.T.);
#8534=EDGE_CURVE('',#6634,#6636,#3282,.T.);
#8535=EDGE_CURVE('',#6638,#6639,#4717,.T.);
#8536=EDGE_CURVE('',#6639,#6637,#3283,.T.);
#8537=EDGE_CURVE('',#6636,#6638,#3284,.T.);
#8538=EDGE_CURVE('',#6640,#6641,#4718,.T.);
#8539=EDGE_CURVE('',#6641,#6639,#3285,.T.);
#8540=EDGE_CURVE('',#6638,#6640,#3286,.T.);
#8541=EDGE_CURVE('',#6642,#6643,#4719,.T.);
#8542=EDGE_CURVE('',#6643,#6641,#3287,.T.);
#8543=EDGE_CURVE('',#6640,#6642,#3288,.T.);
#8544=EDGE_CURVE('',#6644,#6645,#4720,.T.);
#8545=EDGE_CURVE('',#6644,#6646,#3289,.T.);
#8546=EDGE_CURVE('',#6647,#6646,#2794,.T.);
#8547=EDGE_CURVE('',#6647,#6645,#3290,.T.);
#8548=EDGE_CURVE('',#6648,#6649,#4721,.T.);
#8549=EDGE_CURVE('',#6649,#6650,#3291,.T.);
#8550=EDGE_CURVE('',#6651,#6650,#2795,.T.);
#8551=EDGE_CURVE('',#6648,#6651,#3292,.T.);
#8552=EDGE_CURVE('',#6652,#6653,#4722,.T.);
#8553=EDGE_CURVE('',#6653,#6649,#3293,.T.);
#8554=EDGE_CURVE('',#6652,#6648,#3294,.T.);
#8555=EDGE_CURVE('',#6654,#6655,#4723,.T.);
#8556=EDGE_CURVE('',#6655,#6653,#3295,.T.);
#8557=EDGE_CURVE('',#6654,#6652,#3296,.T.);
#8558=EDGE_CURVE('',#6656,#6657,#4724,.T.);
#8559=EDGE_CURVE('',#6657,#6655,#3297,.T.);
#8560=EDGE_CURVE('',#6656,#6654,#3298,.T.);
#8561=EDGE_CURVE('',#6658,#6659,#4725,.T.);
#8562=EDGE_CURVE('',#6659,#6657,#3299,.T.);
#8563=EDGE_CURVE('',#6658,#6656,#3300,.T.);
#8564=EDGE_CURVE('',#6660,#6661,#4726,.T.);
#8565=EDGE_CURVE('',#6661,#6659,#3301,.T.);
#8566=EDGE_CURVE('',#6660,#6658,#3302,.T.);
#8567=EDGE_CURVE('',#6662,#6663,#4727,.T.);
#8568=EDGE_CURVE('',#6663,#6661,#3303,.T.);
#8569=EDGE_CURVE('',#6662,#6660,#3304,.T.);
#8570=EDGE_CURVE('',#6664,#6665,#4728,.T.);
#8571=EDGE_CURVE('',#6665,#6663,#3305,.T.);
#8572=EDGE_CURVE('',#6664,#6662,#3306,.T.);
#8573=EDGE_CURVE('',#6666,#6667,#4729,.T.);
#8574=EDGE_CURVE('',#6667,#6665,#3307,.T.);
#8575=EDGE_CURVE('',#6666,#6664,#3308,.T.);
#8576=EDGE_CURVE('',#6668,#6669,#4730,.T.);
#8577=EDGE_CURVE('',#6669,#6667,#3309,.T.);
#8578=EDGE_CURVE('',#6668,#6666,#3310,.T.);
#8579=EDGE_CURVE('',#6670,#6671,#4731,.T.);
#8580=EDGE_CURVE('',#6671,#6669,#3311,.T.);
#8581=EDGE_CURVE('',#6670,#6668,#3312,.T.);
#8582=EDGE_CURVE('',#6672,#6673,#4732,.T.);
#8583=EDGE_CURVE('',#6673,#6671,#3313,.T.);
#8584=EDGE_CURVE('',#6672,#6670,#3314,.T.);
#8585=EDGE_CURVE('',#6674,#6675,#4733,.T.);
#8586=EDGE_CURVE('',#6676,#6674,#3315,.T.);
#8587=EDGE_CURVE('',#6677,#6676,#2796,.T.);
#8588=EDGE_CURVE('',#6677,#6675,#3316,.T.);
#8589=EDGE_CURVE('',#6678,#6679,#4734,.T.);
#8590=EDGE_CURVE('',#6679,#6680,#3317,.T.);
#8591=EDGE_CURVE('',#6680,#6681,#2797,.T.);
#8592=EDGE_CURVE('',#6681,#6682,#3318,.T.);
#8593=EDGE_CURVE('',#6682,#6683,#4735,.T.);
#8594=EDGE_CURVE('',#6683,#6683,#2798,.F.);
#8595=EDGE_CURVE('',#6682,#6678,#3319,.T.);
#8596=EDGE_CURVE('',#6684,#6685,#4736,.T.);
#8597=EDGE_CURVE('',#6685,#6679,#3320,.T.);
#8598=EDGE_CURVE('',#6678,#6684,#3321,.T.);
#8599=EDGE_CURVE('',#6686,#6687,#4737,.T.);
#8600=EDGE_CURVE('',#6687,#6685,#3322,.T.);
#8601=EDGE_CURVE('',#6684,#6686,#3323,.T.);
#8602=EDGE_CURVE('',#6688,#6689,#4738,.T.);
#8603=EDGE_CURVE('',#6689,#6687,#3324,.T.);
#8604=EDGE_CURVE('',#6686,#6688,#3325,.T.);
#8605=EDGE_CURVE('',#6690,#6691,#4739,.T.);
#8606=EDGE_CURVE('',#6691,#6689,#3326,.T.);
#8607=EDGE_CURVE('',#6688,#6690,#3327,.T.);
#8608=EDGE_CURVE('',#6692,#6693,#4740,.T.);
#8609=EDGE_CURVE('',#6693,#6691,#3328,.T.);
#8610=EDGE_CURVE('',#6690,#6692,#3329,.T.);
#8611=EDGE_CURVE('',#6694,#6695,#4741,.T.);
#8612=EDGE_CURVE('',#6695,#6693,#3330,.T.);
#8613=EDGE_CURVE('',#6692,#6694,#3331,.T.);
#8614=EDGE_CURVE('',#6696,#6697,#4742,.T.);
#8615=EDGE_CURVE('',#6697,#6695,#3332,.T.);
#8616=EDGE_CURVE('',#6694,#6696,#3333,.T.);
#8617=EDGE_CURVE('',#6698,#6699,#4743,.T.);
#8618=EDGE_CURVE('',#6699,#6697,#3334,.T.);
#8619=EDGE_CURVE('',#6696,#6698,#3335,.T.);
#8620=EDGE_CURVE('',#6700,#6701,#4744,.T.);
#8621=EDGE_CURVE('',#6701,#6699,#3336,.T.);
#8622=EDGE_CURVE('',#6698,#6700,#3337,.T.);
#8623=EDGE_CURVE('',#6702,#6703,#4745,.T.);
#8624=EDGE_CURVE('',#6703,#6701,#3338,.T.);
#8625=EDGE_CURVE('',#6700,#6702,#3339,.T.);
#8626=EDGE_CURVE('',#6704,#6705,#4746,.T.);
#8627=EDGE_CURVE('',#6704,#6706,#3340,.T.);
#8628=EDGE_CURVE('',#6707,#6706,#2799,.T.);
#8629=EDGE_CURVE('',#6707,#6705,#3341,.T.);
#8630=EDGE_CURVE('',#6708,#6709,#4747,.T.);
#8631=EDGE_CURVE('',#6709,#6710,#3342,.T.);
#8632=EDGE_CURVE('',#6711,#6710,#2800,.T.);
#8633=EDGE_CURVE('',#6708,#6711,#3343,.T.);
#8634=EDGE_CURVE('',#6712,#6713,#4748,.T.);
#8635=EDGE_CURVE('',#6713,#6709,#3344,.T.);
#8636=EDGE_CURVE('',#6712,#6708,#3345,.T.);
#8637=EDGE_CURVE('',#6714,#6715,#4749,.T.);
#8638=EDGE_CURVE('',#6715,#6713,#3346,.T.);
#8639=EDGE_CURVE('',#6714,#6712,#3347,.T.);
#8640=EDGE_CURVE('',#6716,#6717,#4750,.T.);
#8641=EDGE_CURVE('',#6717,#6715,#3348,.T.);
#8642=EDGE_CURVE('',#6716,#6714,#3349,.T.);
#8643=EDGE_CURVE('',#6718,#6719,#4751,.T.);
#8644=EDGE_CURVE('',#6719,#6717,#3350,.T.);
#8645=EDGE_CURVE('',#6718,#6716,#3351,.T.);
#8646=EDGE_CURVE('',#6720,#6721,#4752,.T.);
#8647=EDGE_CURVE('',#6721,#6719,#3352,.T.);
#8648=EDGE_CURVE('',#6720,#6718,#3353,.T.);
#8649=EDGE_CURVE('',#6722,#6723,#4753,.T.);
#8650=EDGE_CURVE('',#6723,#6721,#3354,.T.);
#8651=EDGE_CURVE('',#6722,#6720,#3355,.T.);
#8652=EDGE_CURVE('',#6724,#6725,#4754,.T.);
#8653=EDGE_CURVE('',#6725,#6723,#3356,.T.);
#8654=EDGE_CURVE('',#6724,#6722,#3357,.T.);
#8655=EDGE_CURVE('',#6726,#6727,#4755,.T.);
#8656=EDGE_CURVE('',#6727,#6725,#3358,.T.);
#8657=EDGE_CURVE('',#6726,#6724,#3359,.T.);
#8658=EDGE_CURVE('',#6728,#6729,#4756,.T.);
#8659=EDGE_CURVE('',#6729,#6727,#3360,.T.);
#8660=EDGE_CURVE('',#6728,#6726,#3361,.T.);
#8661=EDGE_CURVE('',#6730,#6731,#4757,.T.);
#8662=EDGE_CURVE('',#6731,#6729,#3362,.T.);
#8663=EDGE_CURVE('',#6730,#6728,#3363,.T.);
#8664=EDGE_CURVE('',#6732,#6733,#4758,.T.);
#8665=EDGE_CURVE('',#6733,#6731,#3364,.T.);
#8666=EDGE_CURVE('',#6732,#6730,#3365,.T.);
#8667=EDGE_CURVE('',#6734,#6735,#4759,.T.);
#8668=EDGE_CURVE('',#6736,#6734,#3366,.T.);
#8669=EDGE_CURVE('',#6737,#6736,#2801,.T.);
#8670=EDGE_CURVE('',#6737,#6735,#3367,.T.);
#8671=EDGE_CURVE('',#6738,#6739,#4760,.T.);
#8672=EDGE_CURVE('',#6739,#6740,#3368,.T.);
#8673=EDGE_CURVE('',#6740,#6741,#2802,.T.);
#8674=EDGE_CURVE('',#6741,#6742,#3369,.T.);
#8675=EDGE_CURVE('',#6742,#6743,#4761,.T.);
#8676=EDGE_CURVE('',#6743,#6743,#2803,.F.);
#8677=EDGE_CURVE('',#6742,#6738,#3370,.T.);
#8678=EDGE_CURVE('',#6744,#6745,#4762,.T.);
#8679=EDGE_CURVE('',#6745,#6739,#3371,.T.);
#8680=EDGE_CURVE('',#6738,#6744,#3372,.T.);
#8681=EDGE_CURVE('',#6746,#6747,#4763,.T.);
#8682=EDGE_CURVE('',#6747,#6745,#3373,.T.);
#8683=EDGE_CURVE('',#6744,#6746,#3374,.T.);
#8684=EDGE_CURVE('',#6748,#6749,#4764,.T.);
#8685=EDGE_CURVE('',#6749,#6747,#3375,.T.);
#8686=EDGE_CURVE('',#6746,#6748,#3376,.T.);
#8687=EDGE_CURVE('',#6750,#6751,#4765,.T.);
#8688=EDGE_CURVE('',#6751,#6749,#3377,.T.);
#8689=EDGE_CURVE('',#6748,#6750,#3378,.T.);
#8690=EDGE_CURVE('',#6752,#6753,#4766,.T.);
#8691=EDGE_CURVE('',#6753,#6751,#3379,.T.);
#8692=EDGE_CURVE('',#6750,#6752,#3380,.T.);
#8693=EDGE_CURVE('',#6754,#6755,#4767,.T.);
#8694=EDGE_CURVE('',#6755,#6753,#3381,.T.);
#8695=EDGE_CURVE('',#6752,#6754,#3382,.T.);
#8696=EDGE_CURVE('',#6756,#6757,#4768,.T.);
#8697=EDGE_CURVE('',#6757,#6755,#3383,.T.);
#8698=EDGE_CURVE('',#6754,#6756,#3384,.T.);
#8699=EDGE_CURVE('',#6758,#6759,#4769,.T.);
#8700=EDGE_CURVE('',#6759,#6757,#3385,.T.);
#8701=EDGE_CURVE('',#6756,#6758,#3386,.T.);
#8702=EDGE_CURVE('',#6760,#6761,#4770,.T.);
#8703=EDGE_CURVE('',#6761,#6759,#3387,.T.);
#8704=EDGE_CURVE('',#6758,#6760,#3388,.T.);
#8705=EDGE_CURVE('',#6762,#6763,#4771,.T.);
#8706=EDGE_CURVE('',#6763,#6761,#3389,.T.);
#8707=EDGE_CURVE('',#6760,#6762,#3390,.T.);
#8708=EDGE_CURVE('',#6764,#6765,#4772,.T.);
#8709=EDGE_CURVE('',#6764,#6766,#3391,.T.);
#8710=EDGE_CURVE('',#6767,#6766,#2804,.T.);
#8711=EDGE_CURVE('',#6767,#6765,#3392,.T.);
#8712=EDGE_CURVE('',#6768,#6769,#4773,.T.);
#8713=EDGE_CURVE('',#6769,#6770,#3393,.T.);
#8714=EDGE_CURVE('',#6771,#6770,#2805,.T.);
#8715=EDGE_CURVE('',#6768,#6771,#3394,.T.);
#8716=EDGE_CURVE('',#6772,#6773,#4774,.T.);
#8717=EDGE_CURVE('',#6773,#6769,#3395,.T.);
#8718=EDGE_CURVE('',#6772,#6768,#3396,.T.);
#8719=EDGE_CURVE('',#6774,#6775,#4775,.T.);
#8720=EDGE_CURVE('',#6775,#6773,#3397,.T.);
#8721=EDGE_CURVE('',#6774,#6772,#3398,.T.);
#8722=EDGE_CURVE('',#6776,#6777,#4776,.T.);
#8723=EDGE_CURVE('',#6777,#6775,#3399,.T.);
#8724=EDGE_CURVE('',#6776,#6774,#3400,.T.);
#8725=EDGE_CURVE('',#6778,#6779,#4777,.T.);
#8726=EDGE_CURVE('',#6779,#6777,#3401,.T.);
#8727=EDGE_CURVE('',#6778,#6776,#3402,.T.);
#8728=EDGE_CURVE('',#6780,#6781,#4778,.T.);
#8729=EDGE_CURVE('',#6781,#6779,#3403,.T.);
#8730=EDGE_CURVE('',#6780,#6778,#3404,.T.);
#8731=EDGE_CURVE('',#6782,#6783,#4779,.T.);
#8732=EDGE_CURVE('',#6783,#6781,#3405,.T.);
#8733=EDGE_CURVE('',#6782,#6780,#3406,.T.);
#8734=EDGE_CURVE('',#6784,#6785,#4780,.T.);
#8735=EDGE_CURVE('',#6785,#6783,#3407,.T.);
#8736=EDGE_CURVE('',#6784,#6782,#3408,.T.);
#8737=EDGE_CURVE('',#6786,#6787,#4781,.T.);
#8738=EDGE_CURVE('',#6787,#6785,#3409,.T.);
#8739=EDGE_CURVE('',#6786,#6784,#3410,.T.);
#8740=EDGE_CURVE('',#6788,#6789,#4782,.T.);
#8741=EDGE_CURVE('',#6789,#6787,#3411,.T.);
#8742=EDGE_CURVE('',#6788,#6786,#3412,.T.);
#8743=EDGE_CURVE('',#6790,#6791,#4783,.T.);
#8744=EDGE_CURVE('',#6791,#6789,#3413,.T.);
#8745=EDGE_CURVE('',#6790,#6788,#3414,.T.);
#8746=EDGE_CURVE('',#6792,#6793,#4784,.T.);
#8747=EDGE_CURVE('',#6793,#6791,#3415,.T.);
#8748=EDGE_CURVE('',#6792,#6790,#3416,.T.);
#8749=EDGE_CURVE('',#6794,#6795,#4785,.T.);
#8750=EDGE_CURVE('',#6796,#6794,#3417,.T.);
#8751=EDGE_CURVE('',#6797,#6796,#2806,.T.);
#8752=EDGE_CURVE('',#6797,#6795,#3418,.T.);
#8753=EDGE_CURVE('',#6798,#6799,#4786,.T.);
#8754=EDGE_CURVE('',#6799,#6800,#3419,.T.);
#8755=EDGE_CURVE('',#6800,#6801,#2807,.T.);
#8756=EDGE_CURVE('',#6801,#6802,#3420,.T.);
#8757=EDGE_CURVE('',#6802,#6803,#4787,.T.);
#8758=EDGE_CURVE('',#6803,#6803,#2808,.F.);
#8759=EDGE_CURVE('',#6802,#6798,#3421,.T.);
#8760=EDGE_CURVE('',#6804,#6805,#4788,.T.);
#8761=EDGE_CURVE('',#6805,#6799,#3422,.T.);
#8762=EDGE_CURVE('',#6798,#6804,#3423,.T.);
#8763=EDGE_CURVE('',#6806,#6807,#4789,.T.);
#8764=EDGE_CURVE('',#6807,#6805,#3424,.T.);
#8765=EDGE_CURVE('',#6804,#6806,#3425,.T.);
#8766=EDGE_CURVE('',#6808,#6809,#4790,.T.);
#8767=EDGE_CURVE('',#6809,#6807,#3426,.T.);
#8768=EDGE_CURVE('',#6806,#6808,#3427,.T.);
#8769=EDGE_CURVE('',#6810,#6811,#4791,.T.);
#8770=EDGE_CURVE('',#6811,#6809,#3428,.T.);
#8771=EDGE_CURVE('',#6808,#6810,#3429,.T.);
#8772=EDGE_CURVE('',#6812,#6813,#4792,.T.);
#8773=EDGE_CURVE('',#6813,#6811,#3430,.T.);
#8774=EDGE_CURVE('',#6810,#6812,#3431,.T.);
#8775=EDGE_CURVE('',#6814,#6815,#4793,.T.);
#8776=EDGE_CURVE('',#6815,#6813,#3432,.T.);
#8777=EDGE_CURVE('',#6812,#6814,#3433,.T.);
#8778=EDGE_CURVE('',#6816,#6817,#4794,.T.);
#8779=EDGE_CURVE('',#6817,#6815,#3434,.T.);
#8780=EDGE_CURVE('',#6814,#6816,#3435,.T.);
#8781=EDGE_CURVE('',#6818,#6819,#4795,.T.);
#8782=EDGE_CURVE('',#6819,#6817,#3436,.T.);
#8783=EDGE_CURVE('',#6816,#6818,#3437,.T.);
#8784=EDGE_CURVE('',#6820,#6821,#4796,.T.);
#8785=EDGE_CURVE('',#6821,#6819,#3438,.T.);
#8786=EDGE_CURVE('',#6818,#6820,#3439,.T.);
#8787=EDGE_CURVE('',#6822,#6823,#4797,.T.);
#8788=EDGE_CURVE('',#6823,#6821,#3440,.T.);
#8789=EDGE_CURVE('',#6820,#6822,#3441,.T.);
#8790=EDGE_CURVE('',#6824,#6825,#4798,.T.);
#8791=EDGE_CURVE('',#6824,#6826,#3442,.T.);
#8792=EDGE_CURVE('',#6827,#6826,#2809,.T.);
#8793=EDGE_CURVE('',#6827,#6825,#3443,.T.);
#8794=EDGE_CURVE('',#6828,#6829,#4799,.T.);
#8795=EDGE_CURVE('',#6829,#6830,#3444,.T.);
#8796=EDGE_CURVE('',#6831,#6830,#2810,.T.);
#8797=EDGE_CURVE('',#6828,#6831,#3445,.T.);
#8798=EDGE_CURVE('',#6832,#6833,#4800,.T.);
#8799=EDGE_CURVE('',#6833,#6829,#3446,.T.);
#8800=EDGE_CURVE('',#6832,#6828,#3447,.T.);
#8801=EDGE_CURVE('',#6834,#6835,#4801,.T.);
#8802=EDGE_CURVE('',#6835,#6833,#3448,.T.);
#8803=EDGE_CURVE('',#6834,#6832,#3449,.T.);
#8804=EDGE_CURVE('',#6836,#6837,#4802,.T.);
#8805=EDGE_CURVE('',#6837,#6835,#3450,.T.);
#8806=EDGE_CURVE('',#6836,#6834,#3451,.T.);
#8807=EDGE_CURVE('',#6838,#6839,#4803,.T.);
#8808=EDGE_CURVE('',#6839,#6837,#3452,.T.);
#8809=EDGE_CURVE('',#6838,#6836,#3453,.T.);
#8810=EDGE_CURVE('',#6840,#6841,#4804,.T.);
#8811=EDGE_CURVE('',#6841,#6839,#3454,.T.);
#8812=EDGE_CURVE('',#6840,#6838,#3455,.T.);
#8813=EDGE_CURVE('',#6842,#6843,#4805,.T.);
#8814=EDGE_CURVE('',#6843,#6841,#3456,.T.);
#8815=EDGE_CURVE('',#6842,#6840,#3457,.T.);
#8816=EDGE_CURVE('',#6844,#6845,#4806,.T.);
#8817=EDGE_CURVE('',#6845,#6843,#3458,.T.);
#8818=EDGE_CURVE('',#6844,#6842,#3459,.T.);
#8819=EDGE_CURVE('',#6846,#6847,#4807,.T.);
#8820=EDGE_CURVE('',#6847,#6845,#3460,.T.);
#8821=EDGE_CURVE('',#6846,#6844,#3461,.T.);
#8822=EDGE_CURVE('',#6848,#6849,#4808,.T.);
#8823=EDGE_CURVE('',#6849,#6847,#3462,.T.);
#8824=EDGE_CURVE('',#6848,#6846,#3463,.T.);
#8825=EDGE_CURVE('',#6850,#6851,#4809,.T.);
#8826=EDGE_CURVE('',#6851,#6849,#3464,.T.);
#8827=EDGE_CURVE('',#6850,#6848,#3465,.T.);
#8828=EDGE_CURVE('',#6852,#6853,#4810,.T.);
#8829=EDGE_CURVE('',#6853,#6851,#3466,.T.);
#8830=EDGE_CURVE('',#6852,#6850,#3467,.T.);
#8831=EDGE_CURVE('',#6854,#6855,#4811,.T.);
#8832=EDGE_CURVE('',#6856,#6854,#3468,.T.);
#8833=EDGE_CURVE('',#6857,#6856,#2811,.T.);
#8834=EDGE_CURVE('',#6857,#6855,#3469,.T.);
#8835=EDGE_CURVE('',#6858,#6859,#4812,.T.);
#8836=EDGE_CURVE('',#6859,#6860,#3470,.T.);
#8837=EDGE_CURVE('',#6860,#6861,#2812,.T.);
#8838=EDGE_CURVE('',#6861,#6862,#3471,.T.);
#8839=EDGE_CURVE('',#6862,#6863,#4813,.T.);
#8840=EDGE_CURVE('',#6863,#6863,#2813,.F.);
#8841=EDGE_CURVE('',#6862,#6858,#3472,.T.);
#8842=EDGE_CURVE('',#6864,#6865,#4814,.T.);
#8843=EDGE_CURVE('',#6865,#6859,#3473,.T.);
#8844=EDGE_CURVE('',#6858,#6864,#3474,.T.);
#8845=EDGE_CURVE('',#6866,#6867,#4815,.T.);
#8846=EDGE_CURVE('',#6867,#6865,#3475,.T.);
#8847=EDGE_CURVE('',#6864,#6866,#3476,.T.);
#8848=EDGE_CURVE('',#6868,#6869,#4816,.T.);
#8849=EDGE_CURVE('',#6869,#6867,#3477,.T.);
#8850=EDGE_CURVE('',#6866,#6868,#3478,.T.);
#8851=EDGE_CURVE('',#6870,#6871,#4817,.T.);
#8852=EDGE_CURVE('',#6871,#6869,#3479,.T.);
#8853=EDGE_CURVE('',#6868,#6870,#3480,.T.);
#8854=EDGE_CURVE('',#6872,#6873,#4818,.T.);
#8855=EDGE_CURVE('',#6873,#6871,#3481,.T.);
#8856=EDGE_CURVE('',#6870,#6872,#3482,.T.);
#8857=EDGE_CURVE('',#6874,#6875,#4819,.T.);
#8858=EDGE_CURVE('',#6875,#6873,#3483,.T.);
#8859=EDGE_CURVE('',#6872,#6874,#3484,.T.);
#8860=EDGE_CURVE('',#6876,#6877,#4820,.T.);
#8861=EDGE_CURVE('',#6877,#6875,#3485,.T.);
#8862=EDGE_CURVE('',#6874,#6876,#3486,.T.);
#8863=EDGE_CURVE('',#6878,#6879,#4821,.T.);
#8864=EDGE_CURVE('',#6879,#6877,#3487,.T.);
#8865=EDGE_CURVE('',#6876,#6878,#3488,.T.);
#8866=EDGE_CURVE('',#6880,#6881,#4822,.T.);
#8867=EDGE_CURVE('',#6881,#6879,#3489,.T.);
#8868=EDGE_CURVE('',#6878,#6880,#3490,.T.);
#8869=EDGE_CURVE('',#6882,#6883,#4823,.T.);
#8870=EDGE_CURVE('',#6883,#6881,#3491,.T.);
#8871=EDGE_CURVE('',#6880,#6882,#3492,.T.);
#8872=EDGE_CURVE('',#6884,#6885,#4824,.T.);
#8873=EDGE_CURVE('',#6884,#6886,#3493,.T.);
#8874=EDGE_CURVE('',#6887,#6886,#2814,.F.);
#8875=EDGE_CURVE('',#6887,#6885,#3494,.T.);
#8876=EDGE_CURVE('',#6888,#6889,#4825,.T.);
#8877=EDGE_CURVE('',#6889,#6890,#3495,.T.);
#8878=EDGE_CURVE('',#6891,#6890,#2815,.T.);
#8879=EDGE_CURVE('',#6888,#6891,#3496,.T.);
#8880=EDGE_CURVE('',#6892,#6893,#4826,.T.);
#8881=EDGE_CURVE('',#6893,#6889,#3497,.T.);
#8882=EDGE_CURVE('',#6892,#6888,#3498,.T.);
#8883=EDGE_CURVE('',#6894,#6895,#4827,.T.);
#8884=EDGE_CURVE('',#6895,#6893,#3499,.T.);
#8885=EDGE_CURVE('',#6894,#6892,#3500,.T.);
#8886=EDGE_CURVE('',#6896,#6897,#4828,.T.);
#8887=EDGE_CURVE('',#6897,#6895,#3501,.T.);
#8888=EDGE_CURVE('',#6896,#6894,#3502,.T.);
#8889=EDGE_CURVE('',#6898,#6899,#4829,.T.);
#8890=EDGE_CURVE('',#6899,#6897,#3503,.T.);
#8891=EDGE_CURVE('',#6898,#6896,#3504,.T.);
#8892=EDGE_CURVE('',#6900,#6901,#4830,.T.);
#8893=EDGE_CURVE('',#6901,#6899,#3505,.T.);
#8894=EDGE_CURVE('',#6900,#6898,#3506,.T.);
#8895=EDGE_CURVE('',#6902,#6903,#4831,.T.);
#8896=EDGE_CURVE('',#6903,#6901,#3507,.T.);
#8897=EDGE_CURVE('',#6902,#6900,#3508,.T.);
#8898=EDGE_CURVE('',#6904,#6905,#4832,.T.);
#8899=EDGE_CURVE('',#6905,#6903,#3509,.T.);
#8900=EDGE_CURVE('',#6904,#6902,#3510,.T.);
#8901=EDGE_CURVE('',#6906,#6907,#4833,.T.);
#8902=EDGE_CURVE('',#6907,#6905,#3511,.T.);
#8903=EDGE_CURVE('',#6906,#6904,#3512,.T.);
#8904=EDGE_CURVE('',#6908,#6909,#4834,.T.);
#8905=EDGE_CURVE('',#6909,#6907,#3513,.T.);
#8906=EDGE_CURVE('',#6908,#6906,#3514,.T.);
#8907=EDGE_CURVE('',#6910,#6911,#4835,.T.);
#8908=EDGE_CURVE('',#6911,#6909,#3515,.T.);
#8909=EDGE_CURVE('',#6910,#6908,#3516,.T.);
#8910=EDGE_CURVE('',#6912,#6913,#4836,.T.);
#8911=EDGE_CURVE('',#6913,#6911,#3517,.T.);
#8912=EDGE_CURVE('',#6912,#6910,#3518,.T.);
#8913=EDGE_CURVE('',#6914,#6915,#4837,.T.);
#8914=EDGE_CURVE('',#6916,#6914,#3519,.T.);
#8915=EDGE_CURVE('',#6917,#6916,#2816,.T.);
#8916=EDGE_CURVE('',#6917,#6915,#3520,.T.);
#8917=EDGE_CURVE('',#6918,#6919,#4838,.T.);
#8918=EDGE_CURVE('',#6919,#6920,#3521,.T.);
#8919=EDGE_CURVE('',#6920,#6921,#2817,.T.);
#8920=EDGE_CURVE('',#6921,#6922,#3522,.T.);
#8921=EDGE_CURVE('',#6922,#6923,#4839,.T.);
#8922=EDGE_CURVE('',#6923,#6923,#2818,.F.);
#8923=EDGE_CURVE('',#6922,#6918,#3523,.T.);
#8924=EDGE_CURVE('',#6924,#6925,#4840,.T.);
#8925=EDGE_CURVE('',#6925,#6919,#3524,.T.);
#8926=EDGE_CURVE('',#6918,#6924,#3525,.T.);
#8927=EDGE_CURVE('',#6926,#6927,#4841,.T.);
#8928=EDGE_CURVE('',#6927,#6925,#3526,.T.);
#8929=EDGE_CURVE('',#6924,#6926,#3527,.T.);
#8930=EDGE_CURVE('',#6928,#6929,#4842,.T.);
#8931=EDGE_CURVE('',#6929,#6927,#3528,.T.);
#8932=EDGE_CURVE('',#6926,#6928,#3529,.T.);
#8933=EDGE_CURVE('',#6930,#6931,#4843,.T.);
#8934=EDGE_CURVE('',#6931,#6929,#3530,.T.);
#8935=EDGE_CURVE('',#6928,#6930,#3531,.T.);
#8936=EDGE_CURVE('',#6932,#6933,#4844,.T.);
#8937=EDGE_CURVE('',#6933,#6931,#3532,.T.);
#8938=EDGE_CURVE('',#6930,#6932,#3533,.T.);
#8939=EDGE_CURVE('',#6934,#6935,#4845,.T.);
#8940=EDGE_CURVE('',#6935,#6933,#3534,.T.);
#8941=EDGE_CURVE('',#6932,#6934,#3535,.T.);
#8942=EDGE_CURVE('',#6936,#6937,#4846,.T.);
#8943=EDGE_CURVE('',#6937,#6935,#3536,.T.);
#8944=EDGE_CURVE('',#6934,#6936,#3537,.T.);
#8945=EDGE_CURVE('',#6938,#6939,#4847,.T.);
#8946=EDGE_CURVE('',#6939,#6937,#3538,.T.);
#8947=EDGE_CURVE('',#6936,#6938,#3539,.T.);
#8948=EDGE_CURVE('',#6940,#6941,#4848,.T.);
#8949=EDGE_CURVE('',#6941,#6939,#3540,.T.);
#8950=EDGE_CURVE('',#6938,#6940,#3541,.T.);
#8951=EDGE_CURVE('',#6942,#6943,#4849,.T.);
#8952=EDGE_CURVE('',#6943,#6941,#3542,.T.);
#8953=EDGE_CURVE('',#6940,#6942,#3543,.T.);
#8954=EDGE_CURVE('',#6944,#6945,#4850,.T.);
#8955=EDGE_CURVE('',#6944,#6946,#3544,.T.);
#8956=EDGE_CURVE('',#6947,#6946,#2819,.F.);
#8957=EDGE_CURVE('',#6947,#6945,#3545,.T.);
#8958=EDGE_CURVE('',#6948,#6949,#4851,.T.);
#8959=EDGE_CURVE('',#6949,#6950,#3546,.T.);
#8960=EDGE_CURVE('',#6951,#6950,#2820,.T.);
#8961=EDGE_CURVE('',#6948,#6951,#3547,.T.);
#8962=EDGE_CURVE('',#6952,#6953,#4852,.T.);
#8963=EDGE_CURVE('',#6953,#6949,#3548,.T.);
#8964=EDGE_CURVE('',#6952,#6948,#3549,.T.);
#8965=EDGE_CURVE('',#6954,#6955,#4853,.T.);
#8966=EDGE_CURVE('',#6955,#6953,#3550,.T.);
#8967=EDGE_CURVE('',#6954,#6952,#3551,.T.);
#8968=EDGE_CURVE('',#6956,#6957,#4854,.T.);
#8969=EDGE_CURVE('',#6957,#6955,#3552,.T.);
#8970=EDGE_CURVE('',#6956,#6954,#3553,.T.);
#8971=EDGE_CURVE('',#6958,#6959,#4855,.T.);
#8972=EDGE_CURVE('',#6959,#6957,#3554,.T.);
#8973=EDGE_CURVE('',#6958,#6956,#3555,.T.);
#8974=EDGE_CURVE('',#6960,#6961,#4856,.T.);
#8975=EDGE_CURVE('',#6961,#6959,#3556,.T.);
#8976=EDGE_CURVE('',#6960,#6958,#3557,.T.);
#8977=EDGE_CURVE('',#6962,#6963,#4857,.T.);
#8978=EDGE_CURVE('',#6963,#6961,#3558,.T.);
#8979=EDGE_CURVE('',#6962,#6960,#3559,.T.);
#8980=EDGE_CURVE('',#6964,#6965,#4858,.T.);
#8981=EDGE_CURVE('',#6965,#6963,#3560,.T.);
#8982=EDGE_CURVE('',#6964,#6962,#3561,.T.);
#8983=EDGE_CURVE('',#6966,#6967,#4859,.T.);
#8984=EDGE_CURVE('',#6967,#6965,#3562,.T.);
#8985=EDGE_CURVE('',#6966,#6964,#3563,.T.);
#8986=EDGE_CURVE('',#6968,#6969,#4860,.T.);
#8987=EDGE_CURVE('',#6969,#6967,#3564,.T.);
#8988=EDGE_CURVE('',#6968,#6966,#3565,.T.);
#8989=EDGE_CURVE('',#6970,#6971,#4861,.T.);
#8990=EDGE_CURVE('',#6971,#6969,#3566,.T.);
#8991=EDGE_CURVE('',#6970,#6968,#3567,.T.);
#8992=EDGE_CURVE('',#6972,#6973,#4862,.T.);
#8993=EDGE_CURVE('',#6973,#6971,#3568,.T.);
#8994=EDGE_CURVE('',#6972,#6970,#3569,.T.);
#8995=EDGE_CURVE('',#6974,#6975,#4863,.T.);
#8996=EDGE_CURVE('',#6976,#6974,#3570,.T.);
#8997=EDGE_CURVE('',#6977,#6976,#2821,.T.);
#8998=EDGE_CURVE('',#6977,#6975,#3571,.T.);
#8999=EDGE_CURVE('',#6978,#6979,#4864,.T.);
#9000=EDGE_CURVE('',#6979,#6980,#3572,.T.);
#9001=EDGE_CURVE('',#6980,#6981,#2822,.T.);
#9002=EDGE_CURVE('',#6981,#6982,#3573,.T.);
#9003=EDGE_CURVE('',#6982,#6983,#4865,.T.);
#9004=EDGE_CURVE('',#6983,#6983,#2823,.F.);
#9005=EDGE_CURVE('',#6982,#6978,#3574,.T.);
#9006=EDGE_CURVE('',#6984,#6985,#4866,.T.);
#9007=EDGE_CURVE('',#6985,#6979,#3575,.T.);
#9008=EDGE_CURVE('',#6978,#6984,#3576,.T.);
#9009=EDGE_CURVE('',#6986,#6987,#4867,.T.);
#9010=EDGE_CURVE('',#6987,#6985,#3577,.T.);
#9011=EDGE_CURVE('',#6984,#6986,#3578,.T.);
#9012=EDGE_CURVE('',#6988,#6989,#4868,.T.);
#9013=EDGE_CURVE('',#6989,#6987,#3579,.T.);
#9014=EDGE_CURVE('',#6986,#6988,#3580,.T.);
#9015=EDGE_CURVE('',#6990,#6991,#4869,.T.);
#9016=EDGE_CURVE('',#6991,#6989,#3581,.T.);
#9017=EDGE_CURVE('',#6988,#6990,#3582,.T.);
#9018=EDGE_CURVE('',#6992,#6993,#4870,.T.);
#9019=EDGE_CURVE('',#6993,#6991,#3583,.T.);
#9020=EDGE_CURVE('',#6990,#6992,#3584,.T.);
#9021=EDGE_CURVE('',#6994,#6995,#4871,.T.);
#9022=EDGE_CURVE('',#6995,#6993,#3585,.T.);
#9023=EDGE_CURVE('',#6992,#6994,#3586,.T.);
#9024=EDGE_CURVE('',#6996,#6997,#4872,.T.);
#9025=EDGE_CURVE('',#6997,#6995,#3587,.T.);
#9026=EDGE_CURVE('',#6994,#6996,#3588,.T.);
#9027=EDGE_CURVE('',#6998,#6999,#4873,.T.);
#9028=EDGE_CURVE('',#6999,#6997,#3589,.T.);
#9029=EDGE_CURVE('',#6996,#6998,#3590,.T.);
#9030=EDGE_CURVE('',#7000,#7001,#4874,.T.);
#9031=EDGE_CURVE('',#7001,#6999,#3591,.T.);
#9032=EDGE_CURVE('',#6998,#7000,#3592,.T.);
#9033=EDGE_CURVE('',#7002,#7003,#4875,.T.);
#9034=EDGE_CURVE('',#7003,#7001,#3593,.T.);
#9035=EDGE_CURVE('',#7000,#7002,#3594,.T.);
#9036=EDGE_CURVE('',#7004,#7005,#4876,.T.);
#9037=EDGE_CURVE('',#7004,#7006,#3595,.T.);
#9038=EDGE_CURVE('',#7007,#7006,#2824,.F.);
#9039=EDGE_CURVE('',#7007,#7005,#3596,.T.);
#9040=EDGE_CURVE('',#7008,#7009,#4877,.T.);
#9041=EDGE_CURVE('',#7009,#7010,#3597,.T.);
#9042=EDGE_CURVE('',#7011,#7010,#2825,.T.);
#9043=EDGE_CURVE('',#7008,#7011,#3598,.T.);
#9044=EDGE_CURVE('',#7012,#7013,#4878,.T.);
#9045=EDGE_CURVE('',#7013,#7009,#3599,.T.);
#9046=EDGE_CURVE('',#7012,#7008,#3600,.T.);
#9047=EDGE_CURVE('',#7014,#7015,#4879,.T.);
#9048=EDGE_CURVE('',#7015,#7013,#3601,.T.);
#9049=EDGE_CURVE('',#7014,#7012,#3602,.T.);
#9050=EDGE_CURVE('',#7016,#7017,#4880,.T.);
#9051=EDGE_CURVE('',#7017,#7015,#3603,.T.);
#9052=EDGE_CURVE('',#7016,#7014,#3604,.T.);
#9053=EDGE_CURVE('',#7018,#7019,#4881,.T.);
#9054=EDGE_CURVE('',#7019,#7017,#3605,.T.);
#9055=EDGE_CURVE('',#7018,#7016,#3606,.T.);
#9056=EDGE_CURVE('',#7020,#7021,#4882,.T.);
#9057=EDGE_CURVE('',#7021,#7019,#3607,.T.);
#9058=EDGE_CURVE('',#7020,#7018,#3608,.T.);
#9059=EDGE_CURVE('',#7022,#7023,#4883,.T.);
#9060=EDGE_CURVE('',#7023,#7021,#3609,.T.);
#9061=EDGE_CURVE('',#7022,#7020,#3610,.T.);
#9062=EDGE_CURVE('',#7024,#7025,#4884,.T.);
#9063=EDGE_CURVE('',#7025,#7023,#3611,.T.);
#9064=EDGE_CURVE('',#7024,#7022,#3612,.T.);
#9065=EDGE_CURVE('',#7026,#7027,#4885,.T.);
#9066=EDGE_CURVE('',#7027,#7025,#3613,.T.);
#9067=EDGE_CURVE('',#7026,#7024,#3614,.T.);
#9068=EDGE_CURVE('',#7028,#7029,#4886,.T.);
#9069=EDGE_CURVE('',#7029,#7027,#3615,.T.);
#9070=EDGE_CURVE('',#7028,#7026,#3616,.T.);
#9071=EDGE_CURVE('',#7030,#7031,#4887,.T.);
#9072=EDGE_CURVE('',#7031,#7029,#3617,.T.);
#9073=EDGE_CURVE('',#7030,#7028,#3618,.T.);
#9074=EDGE_CURVE('',#7032,#7033,#4888,.T.);
#9075=EDGE_CURVE('',#7033,#7031,#3619,.T.);
#9076=EDGE_CURVE('',#7032,#7030,#3620,.T.);
#9077=EDGE_CURVE('',#7034,#7035,#4889,.T.);
#9078=EDGE_CURVE('',#7036,#7034,#3621,.T.);
#9079=EDGE_CURVE('',#7037,#7036,#2826,.T.);
#9080=EDGE_CURVE('',#7037,#7035,#3622,.T.);
#9081=EDGE_CURVE('',#7038,#7039,#4890,.T.);
#9082=EDGE_CURVE('',#7039,#7040,#3623,.T.);
#9083=EDGE_CURVE('',#7040,#7041,#2827,.T.);
#9084=EDGE_CURVE('',#7041,#7042,#3624,.T.);
#9085=EDGE_CURVE('',#7042,#7043,#4891,.T.);
#9086=EDGE_CURVE('',#7043,#7043,#2828,.F.);
#9087=EDGE_CURVE('',#7042,#7038,#3625,.T.);
#9088=EDGE_CURVE('',#7044,#7045,#4892,.T.);
#9089=EDGE_CURVE('',#7045,#7039,#3626,.T.);
#9090=EDGE_CURVE('',#7038,#7044,#3627,.T.);
#9091=EDGE_CURVE('',#7046,#7047,#4893,.T.);
#9092=EDGE_CURVE('',#7047,#7045,#3628,.T.);
#9093=EDGE_CURVE('',#7044,#7046,#3629,.T.);
#9094=EDGE_CURVE('',#7048,#7049,#4894,.T.);
#9095=EDGE_CURVE('',#7049,#7047,#3630,.T.);
#9096=EDGE_CURVE('',#7046,#7048,#3631,.T.);
#9097=EDGE_CURVE('',#7050,#7051,#4895,.T.);
#9098=EDGE_CURVE('',#7051,#7049,#3632,.T.);
#9099=EDGE_CURVE('',#7048,#7050,#3633,.T.);
#9100=EDGE_CURVE('',#7052,#7053,#4896,.T.);
#9101=EDGE_CURVE('',#7053,#7051,#3634,.T.);
#9102=EDGE_CURVE('',#7050,#7052,#3635,.T.);
#9103=EDGE_CURVE('',#7054,#7055,#4897,.T.);
#9104=EDGE_CURVE('',#7055,#7053,#3636,.T.);
#9105=EDGE_CURVE('',#7052,#7054,#3637,.T.);
#9106=EDGE_CURVE('',#7056,#7057,#4898,.T.);
#9107=EDGE_CURVE('',#7057,#7055,#3638,.T.);
#9108=EDGE_CURVE('',#7054,#7056,#3639,.T.);
#9109=EDGE_CURVE('',#7058,#7059,#4899,.T.);
#9110=EDGE_CURVE('',#7059,#7057,#3640,.T.);
#9111=EDGE_CURVE('',#7056,#7058,#3641,.T.);
#9112=EDGE_CURVE('',#7060,#7061,#4900,.T.);
#9113=EDGE_CURVE('',#7061,#7059,#3642,.T.);
#9114=EDGE_CURVE('',#7058,#7060,#3643,.T.);
#9115=EDGE_CURVE('',#7062,#7063,#4901,.T.);
#9116=EDGE_CURVE('',#7063,#7061,#3644,.T.);
#9117=EDGE_CURVE('',#7060,#7062,#3645,.T.);
#9118=EDGE_CURVE('',#7064,#7065,#4902,.T.);
#9119=EDGE_CURVE('',#7064,#7066,#3646,.T.);
#9120=EDGE_CURVE('',#7067,#7066,#2829,.F.);
#9121=EDGE_CURVE('',#7067,#7065,#3647,.T.);
#9122=EDGE_CURVE('',#7068,#7069,#4903,.T.);
#9123=EDGE_CURVE('',#7069,#7070,#3648,.T.);
#9124=EDGE_CURVE('',#7071,#7070,#2830,.T.);
#9125=EDGE_CURVE('',#7068,#7071,#3649,.T.);
#9126=EDGE_CURVE('',#7072,#7073,#4904,.T.);
#9127=EDGE_CURVE('',#7073,#7069,#3650,.T.);
#9128=EDGE_CURVE('',#7072,#7068,#3651,.T.);
#9129=EDGE_CURVE('',#7074,#7075,#4905,.T.);
#9130=EDGE_CURVE('',#7075,#7073,#3652,.T.);
#9131=EDGE_CURVE('',#7074,#7072,#3653,.T.);
#9132=EDGE_CURVE('',#7076,#7077,#4906,.T.);
#9133=EDGE_CURVE('',#7077,#7075,#3654,.T.);
#9134=EDGE_CURVE('',#7076,#7074,#3655,.T.);
#9135=EDGE_CURVE('',#7078,#7079,#4907,.T.);
#9136=EDGE_CURVE('',#7079,#7077,#3656,.T.);
#9137=EDGE_CURVE('',#7078,#7076,#3657,.T.);
#9138=EDGE_CURVE('',#7080,#7081,#4908,.T.);
#9139=EDGE_CURVE('',#7081,#7079,#3658,.T.);
#9140=EDGE_CURVE('',#7080,#7078,#3659,.T.);
#9141=EDGE_CURVE('',#7082,#7083,#4909,.T.);
#9142=EDGE_CURVE('',#7083,#7081,#3660,.T.);
#9143=EDGE_CURVE('',#7082,#7080,#3661,.T.);
#9144=EDGE_CURVE('',#7084,#7085,#4910,.T.);
#9145=EDGE_CURVE('',#7085,#7083,#3662,.T.);
#9146=EDGE_CURVE('',#7084,#7082,#3663,.T.);
#9147=EDGE_CURVE('',#7086,#7087,#4911,.T.);
#9148=EDGE_CURVE('',#7087,#7085,#3664,.T.);
#9149=EDGE_CURVE('',#7086,#7084,#3665,.T.);
#9150=EDGE_CURVE('',#7088,#7089,#4912,.T.);
#9151=EDGE_CURVE('',#7089,#7087,#3666,.T.);
#9152=EDGE_CURVE('',#7088,#7086,#3667,.T.);
#9153=EDGE_CURVE('',#7090,#7091,#4913,.T.);
#9154=EDGE_CURVE('',#7091,#7089,#3668,.T.);
#9155=EDGE_CURVE('',#7090,#7088,#3669,.T.);
#9156=EDGE_CURVE('',#7092,#7093,#4914,.T.);
#9157=EDGE_CURVE('',#7093,#7091,#3670,.T.);
#9158=EDGE_CURVE('',#7092,#7090,#3671,.T.);
#9159=EDGE_CURVE('',#7094,#7095,#4915,.T.);
#9160=EDGE_CURVE('',#7096,#7094,#3672,.T.);
#9161=EDGE_CURVE('',#7097,#7096,#2831,.T.);
#9162=EDGE_CURVE('',#7097,#7095,#3673,.T.);
#9163=EDGE_CURVE('',#7098,#7099,#4916,.T.);
#9164=EDGE_CURVE('',#7099,#7100,#3674,.T.);
#9165=EDGE_CURVE('',#7100,#7101,#2832,.T.);
#9166=EDGE_CURVE('',#7101,#7102,#3675,.T.);
#9167=EDGE_CURVE('',#7102,#7103,#4917,.T.);
#9168=EDGE_CURVE('',#7103,#7103,#2833,.F.);
#9169=EDGE_CURVE('',#7102,#7098,#3676,.T.);
#9170=EDGE_CURVE('',#7104,#7105,#4918,.T.);
#9171=EDGE_CURVE('',#7105,#7099,#3677,.T.);
#9172=EDGE_CURVE('',#7098,#7104,#3678,.T.);
#9173=EDGE_CURVE('',#7106,#7107,#4919,.T.);
#9174=EDGE_CURVE('',#7107,#7105,#3679,.T.);
#9175=EDGE_CURVE('',#7104,#7106,#3680,.T.);
#9176=EDGE_CURVE('',#7108,#7109,#4920,.T.);
#9177=EDGE_CURVE('',#7109,#7107,#3681,.T.);
#9178=EDGE_CURVE('',#7106,#7108,#3682,.T.);
#9179=EDGE_CURVE('',#7110,#7111,#4921,.T.);
#9180=EDGE_CURVE('',#7111,#7109,#3683,.T.);
#9181=EDGE_CURVE('',#7108,#7110,#3684,.T.);
#9182=EDGE_CURVE('',#7112,#7113,#4922,.T.);
#9183=EDGE_CURVE('',#7113,#7111,#3685,.T.);
#9184=EDGE_CURVE('',#7110,#7112,#3686,.T.);
#9185=EDGE_CURVE('',#7114,#7115,#4923,.T.);
#9186=EDGE_CURVE('',#7115,#7113,#3687,.T.);
#9187=EDGE_CURVE('',#7112,#7114,#3688,.T.);
#9188=EDGE_CURVE('',#7116,#7117,#4924,.T.);
#9189=EDGE_CURVE('',#7117,#7115,#3689,.T.);
#9190=EDGE_CURVE('',#7114,#7116,#3690,.T.);
#9191=EDGE_CURVE('',#7118,#7119,#4925,.T.);
#9192=EDGE_CURVE('',#7119,#7117,#3691,.T.);
#9193=EDGE_CURVE('',#7116,#7118,#3692,.T.);
#9194=EDGE_CURVE('',#7120,#7121,#4926,.T.);
#9195=EDGE_CURVE('',#7121,#7119,#3693,.T.);
#9196=EDGE_CURVE('',#7118,#7120,#3694,.T.);
#9197=EDGE_CURVE('',#7122,#7123,#4927,.T.);
#9198=EDGE_CURVE('',#7123,#7121,#3695,.T.);
#9199=EDGE_CURVE('',#7120,#7122,#3696,.T.);
#9200=EDGE_CURVE('',#7124,#7125,#4928,.T.);
#9201=EDGE_CURVE('',#7124,#7126,#3697,.T.);
#9202=EDGE_CURVE('',#7127,#7126,#2834,.F.);
#9203=EDGE_CURVE('',#7127,#7125,#3698,.T.);
#9204=EDGE_CURVE('',#7128,#7129,#4929,.T.);
#9205=EDGE_CURVE('',#7129,#7130,#3699,.T.);
#9206=EDGE_CURVE('',#7131,#7130,#2835,.T.);
#9207=EDGE_CURVE('',#7128,#7131,#3700,.T.);
#9208=EDGE_CURVE('',#7132,#7133,#4930,.T.);
#9209=EDGE_CURVE('',#7133,#7129,#3701,.T.);
#9210=EDGE_CURVE('',#7132,#7128,#3702,.T.);
#9211=EDGE_CURVE('',#7134,#7135,#4931,.T.);
#9212=EDGE_CURVE('',#7135,#7133,#3703,.T.);
#9213=EDGE_CURVE('',#7134,#7132,#3704,.T.);
#9214=EDGE_CURVE('',#7136,#7137,#4932,.T.);
#9215=EDGE_CURVE('',#7137,#7135,#3705,.T.);
#9216=EDGE_CURVE('',#7136,#7134,#3706,.T.);
#9217=EDGE_CURVE('',#7138,#7139,#4933,.T.);
#9218=EDGE_CURVE('',#7139,#7137,#3707,.T.);
#9219=EDGE_CURVE('',#7138,#7136,#3708,.T.);
#9220=EDGE_CURVE('',#7140,#7141,#4934,.T.);
#9221=EDGE_CURVE('',#7141,#7139,#3709,.T.);
#9222=EDGE_CURVE('',#7140,#7138,#3710,.T.);
#9223=EDGE_CURVE('',#7142,#7143,#4935,.T.);
#9224=EDGE_CURVE('',#7143,#7141,#3711,.T.);
#9225=EDGE_CURVE('',#7142,#7140,#3712,.T.);
#9226=EDGE_CURVE('',#7144,#7145,#4936,.T.);
#9227=EDGE_CURVE('',#7145,#7143,#3713,.T.);
#9228=EDGE_CURVE('',#7144,#7142,#3714,.T.);
#9229=EDGE_CURVE('',#7146,#7147,#4937,.T.);
#9230=EDGE_CURVE('',#7147,#7145,#3715,.T.);
#9231=EDGE_CURVE('',#7146,#7144,#3716,.T.);
#9232=EDGE_CURVE('',#7148,#7149,#4938,.T.);
#9233=EDGE_CURVE('',#7149,#7147,#3717,.T.);
#9234=EDGE_CURVE('',#7148,#7146,#3718,.T.);
#9235=EDGE_CURVE('',#7150,#7151,#4939,.T.);
#9236=EDGE_CURVE('',#7151,#7149,#3719,.T.);
#9237=EDGE_CURVE('',#7150,#7148,#3720,.T.);
#9238=EDGE_CURVE('',#7152,#7153,#4940,.T.);
#9239=EDGE_CURVE('',#7153,#7151,#3721,.T.);
#9240=EDGE_CURVE('',#7152,#7150,#3722,.T.);
#9241=EDGE_CURVE('',#7154,#7155,#4941,.T.);
#9242=EDGE_CURVE('',#7156,#7154,#3723,.T.);
#9243=EDGE_CURVE('',#7157,#7156,#2836,.T.);
#9244=EDGE_CURVE('',#7157,#7155,#3724,.T.);
#9245=EDGE_CURVE('',#7158,#7159,#4942,.T.);
#9246=EDGE_CURVE('',#7159,#7160,#3725,.T.);
#9247=EDGE_CURVE('',#7160,#7161,#2837,.F.);
#9248=EDGE_CURVE('',#7161,#7158,#3726,.T.);
#9249=EDGE_CURVE('',#7162,#7163,#4943,.T.);
#9250=EDGE_CURVE('',#7163,#7159,#3727,.T.);
#9251=EDGE_CURVE('',#7158,#7162,#3728,.T.);
#9252=EDGE_CURVE('',#7164,#7165,#4944,.T.);
#9253=EDGE_CURVE('',#7165,#7163,#3729,.T.);
#9254=EDGE_CURVE('',#7162,#7164,#3730,.T.);
#9255=EDGE_CURVE('',#7166,#7167,#4945,.T.);
#9256=EDGE_CURVE('',#7167,#7165,#3731,.T.);
#9257=EDGE_CURVE('',#7164,#7166,#3732,.T.);
#9258=EDGE_CURVE('',#7168,#7169,#4946,.T.);
#9259=EDGE_CURVE('',#7169,#7167,#3733,.T.);
#9260=EDGE_CURVE('',#7166,#7168,#3734,.T.);
#9261=EDGE_CURVE('',#7170,#7171,#4947,.T.);
#9262=EDGE_CURVE('',#7171,#7169,#3735,.T.);
#9263=EDGE_CURVE('',#7168,#7170,#3736,.T.);
#9264=EDGE_CURVE('',#7172,#7173,#4948,.T.);
#9265=EDGE_CURVE('',#7173,#7171,#3737,.T.);
#9266=EDGE_CURVE('',#7170,#7172,#3738,.T.);
#9267=EDGE_CURVE('',#7174,#7175,#4949,.T.);
#9268=EDGE_CURVE('',#7174,#7176,#3739,.T.);
#9269=EDGE_CURVE('',#7177,#7176,#3740,.T.);
#9270=EDGE_CURVE('',#7177,#7175,#3741,.T.);
#9271=EDGE_CURVE('',#7178,#7179,#4950,.T.);
#9272=EDGE_CURVE('',#7179,#7180,#3742,.T.);
#9273=EDGE_CURVE('',#7181,#7180,#2838,.T.);
#9274=EDGE_CURVE('',#7178,#7181,#3743,.T.);
#9275=EDGE_CURVE('',#7182,#7183,#4951,.T.);
#9276=EDGE_CURVE('',#7183,#7179,#3744,.T.);
#9277=EDGE_CURVE('',#7182,#7178,#3745,.T.);
#9278=EDGE_CURVE('',#7184,#7185,#4952,.T.);
#9279=EDGE_CURVE('',#7185,#7183,#3746,.T.);
#9280=EDGE_CURVE('',#7184,#7182,#3747,.T.);
#9281=EDGE_CURVE('',#7186,#7187,#4953,.T.);
#9282=EDGE_CURVE('',#7187,#7185,#3748,.T.);
#9283=EDGE_CURVE('',#7186,#7184,#3749,.T.);
#9284=EDGE_CURVE('',#7188,#7189,#4954,.T.);
#9285=EDGE_CURVE('',#7189,#7187,#3750,.T.);
#9286=EDGE_CURVE('',#7188,#7186,#3751,.T.);
#9287=EDGE_CURVE('',#7190,#7191,#4955,.T.);
#9288=EDGE_CURVE('',#7191,#7189,#3752,.T.);
#9289=EDGE_CURVE('',#7190,#7188,#3753,.T.);
#9290=EDGE_CURVE('',#7192,#7193,#4956,.T.);
#9291=EDGE_CURVE('',#7193,#7191,#3754,.T.);
#9292=EDGE_CURVE('',#7192,#7190,#3755,.T.);
#9293=EDGE_CURVE('',#7194,#7195,#4957,.T.);
#9294=EDGE_CURVE('',#7196,#7194,#3756,.T.);
#9295=EDGE_CURVE('',#7197,#7196,#3757,.T.);
#9296=EDGE_CURVE('',#7198,#7197,#3758,.T.);
#9297=EDGE_CURVE('',#7198,#7195,#3759,.T.);
#9298=EDGE_CURVE('',#7199,#7200,#4958,.T.);
#9299=EDGE_CURVE('',#7200,#7201,#3760,.T.);
#9300=EDGE_CURVE('',#7201,#7202,#2839,.F.);
#9301=EDGE_CURVE('',#7202,#7199,#3761,.T.);
#9302=EDGE_CURVE('',#7203,#7204,#4959,.T.);
#9303=EDGE_CURVE('',#7204,#7200,#3762,.T.);
#9304=EDGE_CURVE('',#7199,#7203,#3763,.T.);
#9305=EDGE_CURVE('',#7205,#7206,#4960,.T.);
#9306=EDGE_CURVE('',#7206,#7204,#3764,.T.);
#9307=EDGE_CURVE('',#7203,#7205,#3765,.T.);
#9308=EDGE_CURVE('',#7207,#7208,#4961,.T.);
#9309=EDGE_CURVE('',#7208,#7206,#3766,.T.);
#9310=EDGE_CURVE('',#7205,#7207,#3767,.T.);
#9311=EDGE_CURVE('',#7209,#7210,#4962,.T.);
#9312=EDGE_CURVE('',#7210,#7208,#3768,.T.);
#9313=EDGE_CURVE('',#7207,#7209,#3769,.T.);
#9314=EDGE_CURVE('',#7211,#7212,#4963,.T.);
#9315=EDGE_CURVE('',#7212,#7210,#3770,.T.);
#9316=EDGE_CURVE('',#7209,#7211,#3771,.T.);
#9317=EDGE_CURVE('',#7213,#7214,#4964,.T.);
#9318=EDGE_CURVE('',#7214,#7212,#3772,.T.);
#9319=EDGE_CURVE('',#7211,#7213,#3773,.T.);
#9320=EDGE_CURVE('',#7215,#7216,#4965,.T.);
#9321=EDGE_CURVE('',#7215,#7217,#3774,.T.);
#9322=EDGE_CURVE('',#7218,#7217,#3775,.T.);
#9323=EDGE_CURVE('',#7218,#7216,#3776,.T.);
#9324=EDGE_CURVE('',#7219,#7220,#4966,.T.);
#9325=EDGE_CURVE('',#7220,#7221,#3777,.T.);
#9326=EDGE_CURVE('',#7221,#7222,#2840,.F.);
#9327=EDGE_CURVE('',#7222,#7219,#3778,.T.);
#9328=EDGE_CURVE('',#7223,#7224,#4967,.T.);
#9329=EDGE_CURVE('',#7224,#7220,#3779,.T.);
#9330=EDGE_CURVE('',#7219,#7223,#3780,.T.);
#9331=EDGE_CURVE('',#7225,#7226,#4968,.T.);
#9332=EDGE_CURVE('',#7226,#7224,#3781,.T.);
#9333=EDGE_CURVE('',#7223,#7225,#3782,.T.);
#9334=EDGE_CURVE('',#7227,#7228,#4969,.T.);
#9335=EDGE_CURVE('',#7228,#7226,#3783,.T.);
#9336=EDGE_CURVE('',#7225,#7227,#3784,.T.);
#9337=EDGE_CURVE('',#7229,#7230,#4970,.T.);
#9338=EDGE_CURVE('',#7230,#7228,#3785,.T.);
#9339=EDGE_CURVE('',#7227,#7229,#3786,.T.);
#9340=EDGE_CURVE('',#7231,#7232,#4971,.T.);
#9341=EDGE_CURVE('',#7232,#7230,#3787,.T.);
#9342=EDGE_CURVE('',#7229,#7231,#3788,.T.);
#9343=EDGE_CURVE('',#7233,#7234,#4972,.T.);
#9344=EDGE_CURVE('',#7234,#7232,#3789,.T.);
#9345=EDGE_CURVE('',#7231,#7233,#3790,.T.);
#9346=EDGE_CURVE('',#7235,#7236,#4973,.T.);
#9347=EDGE_CURVE('',#7235,#7237,#3791,.T.);
#9348=EDGE_CURVE('',#7238,#7237,#3792,.T.);
#9349=EDGE_CURVE('',#7238,#7236,#3793,.T.);
#9350=EDGE_CURVE('',#7239,#7240,#4974,.T.);
#9351=EDGE_CURVE('',#7240,#7241,#3794,.T.);
#9352=EDGE_CURVE('',#7241,#7242,#2841,.F.);
#9353=EDGE_CURVE('',#7242,#7239,#3795,.T.);
#9354=EDGE_CURVE('',#7243,#7244,#4975,.T.);
#9355=EDGE_CURVE('',#7244,#7240,#3796,.T.);
#9356=EDGE_CURVE('',#7239,#7243,#3797,.T.);
#9357=EDGE_CURVE('',#7245,#7246,#4976,.T.);
#9358=EDGE_CURVE('',#7246,#7244,#3798,.T.);
#9359=EDGE_CURVE('',#7243,#7245,#3799,.T.);
#9360=EDGE_CURVE('',#7247,#7248,#4977,.T.);
#9361=EDGE_CURVE('',#7248,#7246,#3800,.T.);
#9362=EDGE_CURVE('',#7245,#7247,#3801,.T.);
#9363=EDGE_CURVE('',#7249,#7250,#4978,.T.);
#9364=EDGE_CURVE('',#7250,#7248,#3802,.T.);
#9365=EDGE_CURVE('',#7247,#7249,#3803,.T.);
#9366=EDGE_CURVE('',#7251,#7252,#4979,.T.);
#9367=EDGE_CURVE('',#7252,#7250,#3804,.T.);
#9368=EDGE_CURVE('',#7249,#7251,#3805,.T.);
#9369=EDGE_CURVE('',#7253,#7254,#4980,.T.);
#9370=EDGE_CURVE('',#7254,#7252,#3806,.T.);
#9371=EDGE_CURVE('',#7251,#7253,#3807,.T.);
#9372=EDGE_CURVE('',#7255,#7256,#4981,.T.);
#9373=EDGE_CURVE('',#7255,#7257,#3808,.T.);
#9374=EDGE_CURVE('',#7258,#7257,#3809,.T.);
#9375=EDGE_CURVE('',#7258,#7256,#3810,.T.);
#9376=EDGE_CURVE('',#7259,#7260,#4982,.T.);
#9377=EDGE_CURVE('',#7260,#7261,#3811,.T.);
#9378=EDGE_CURVE('',#7262,#7261,#2842,.T.);
#9379=EDGE_CURVE('',#7259,#7262,#3812,.T.);
#9380=EDGE_CURVE('',#7263,#7264,#4983,.T.);
#9381=EDGE_CURVE('',#7264,#7260,#3813,.T.);
#9382=EDGE_CURVE('',#7263,#7259,#3814,.T.);
#9383=EDGE_CURVE('',#7265,#7266,#4984,.T.);
#9384=EDGE_CURVE('',#7266,#7264,#3815,.T.);
#9385=EDGE_CURVE('',#7265,#7263,#3816,.T.);
#9386=EDGE_CURVE('',#7267,#7268,#4985,.T.);
#9387=EDGE_CURVE('',#7268,#7266,#3817,.T.);
#9388=EDGE_CURVE('',#7267,#7265,#3818,.T.);
#9389=EDGE_CURVE('',#7269,#7270,#4986,.T.);
#9390=EDGE_CURVE('',#7270,#7268,#3819,.T.);
#9391=EDGE_CURVE('',#7269,#7267,#3820,.T.);
#9392=EDGE_CURVE('',#7271,#7272,#4987,.T.);
#9393=EDGE_CURVE('',#7272,#7270,#3821,.T.);
#9394=EDGE_CURVE('',#7271,#7269,#3822,.T.);
#9395=EDGE_CURVE('',#7273,#7274,#4988,.T.);
#9396=EDGE_CURVE('',#7274,#7272,#3823,.T.);
#9397=EDGE_CURVE('',#7273,#7271,#3824,.T.);
#9398=EDGE_CURVE('',#7275,#7276,#4989,.T.);
#9399=EDGE_CURVE('',#7277,#7275,#3825,.T.);
#9400=EDGE_CURVE('',#7278,#7277,#3826,.T.);
#9401=EDGE_CURVE('',#7279,#7278,#3827,.T.);
#9402=EDGE_CURVE('',#7279,#7276,#3828,.T.);
#9403=EDGE_CURVE('',#7280,#7281,#4990,.T.);
#9404=EDGE_CURVE('',#7281,#7282,#3829,.T.);
#9405=EDGE_CURVE('',#7283,#7282,#2843,.T.);
#9406=EDGE_CURVE('',#7280,#7283,#3830,.T.);
#9407=EDGE_CURVE('',#7284,#7285,#4991,.T.);
#9408=EDGE_CURVE('',#7285,#7281,#3831,.T.);
#9409=EDGE_CURVE('',#7284,#7280,#3832,.T.);
#9410=EDGE_CURVE('',#7286,#7287,#4992,.T.);
#9411=EDGE_CURVE('',#7287,#7285,#3833,.T.);
#9412=EDGE_CURVE('',#7286,#7284,#3834,.T.);
#9413=EDGE_CURVE('',#7288,#7289,#4993,.T.);
#9414=EDGE_CURVE('',#7289,#7287,#3835,.T.);
#9415=EDGE_CURVE('',#7288,#7286,#3836,.T.);
#9416=EDGE_CURVE('',#7290,#7291,#4994,.T.);
#9417=EDGE_CURVE('',#7291,#7289,#3837,.T.);
#9418=EDGE_CURVE('',#7290,#7288,#3838,.T.);
#9419=EDGE_CURVE('',#7292,#7293,#4995,.T.);
#9420=EDGE_CURVE('',#7293,#7291,#3839,.T.);
#9421=EDGE_CURVE('',#7292,#7290,#3840,.T.);
#9422=EDGE_CURVE('',#7294,#7295,#4996,.T.);
#9423=EDGE_CURVE('',#7295,#7293,#3841,.T.);
#9424=EDGE_CURVE('',#7294,#7292,#3842,.T.);
#9425=EDGE_CURVE('',#7296,#7297,#4997,.T.);
#9426=EDGE_CURVE('',#7298,#7296,#3843,.T.);
#9427=EDGE_CURVE('',#7299,#7298,#3844,.T.);
#9428=EDGE_CURVE('',#7300,#7299,#3845,.T.);
#9429=EDGE_CURVE('',#7300,#7297,#3846,.T.);
#9430=EDGE_CURVE('',#7301,#7302,#4998,.T.);
#9431=EDGE_CURVE('',#7302,#7303,#3847,.T.);
#9432=EDGE_CURVE('',#7304,#7303,#2844,.T.);
#9433=EDGE_CURVE('',#7301,#7304,#3848,.T.);
#9434=EDGE_CURVE('',#7305,#7306,#4999,.T.);
#9435=EDGE_CURVE('',#7306,#7302,#3849,.T.);
#9436=EDGE_CURVE('',#7305,#7301,#3850,.T.);
#9437=EDGE_CURVE('',#7307,#7308,#5000,.T.);
#9438=EDGE_CURVE('',#7308,#7306,#3851,.T.);
#9439=EDGE_CURVE('',#7307,#7305,#3852,.T.);
#9440=EDGE_CURVE('',#7309,#7310,#5001,.T.);
#9441=EDGE_CURVE('',#7310,#7308,#3853,.T.);
#9442=EDGE_CURVE('',#7309,#7307,#3854,.T.);
#9443=EDGE_CURVE('',#7311,#7312,#5002,.T.);
#9444=EDGE_CURVE('',#7312,#7310,#3855,.T.);
#9445=EDGE_CURVE('',#7311,#7309,#3856,.T.);
#9446=EDGE_CURVE('',#7313,#7314,#5003,.T.);
#9447=EDGE_CURVE('',#7314,#7312,#3857,.T.);
#9448=EDGE_CURVE('',#7313,#7311,#3858,.T.);
#9449=EDGE_CURVE('',#7315,#7316,#5004,.T.);
#9450=EDGE_CURVE('',#7316,#7314,#3859,.T.);
#9451=EDGE_CURVE('',#7315,#7313,#3860,.T.);
#9452=EDGE_CURVE('',#7317,#7318,#5005,.T.);
#9453=EDGE_CURVE('',#7319,#7317,#3861,.T.);
#9454=EDGE_CURVE('',#7320,#7319,#3862,.T.);
#9455=EDGE_CURVE('',#7321,#7320,#3863,.T.);
#9456=EDGE_CURVE('',#7321,#7318,#3864,.T.);
#9457=EDGE_CURVE('',#7257,#7321,#3865,.T.);
#9458=EDGE_CURVE('',#7253,#7255,#3866,.T.);
#9459=EDGE_CURVE('',#7303,#7242,#3867,.T.);
#9460=EDGE_CURVE('',#7318,#7316,#3868,.T.);
#9461=EDGE_CURVE('',#7317,#7315,#3869,.T.);
#9462=EDGE_CURVE('',#7319,#7258,#3870,.T.);
#9463=EDGE_CURVE('',#7241,#7304,#3871,.T.);
#9464=EDGE_CURVE('',#7256,#7254,#3872,.T.);
#9465=EDGE_CURVE('',#7237,#7300,#3873,.T.);
#9466=EDGE_CURVE('',#7233,#7235,#3874,.T.);
#9467=EDGE_CURVE('',#7282,#7222,#3875,.T.);
#9468=EDGE_CURVE('',#7297,#7295,#3876,.T.);
#9469=EDGE_CURVE('',#7296,#7294,#3877,.T.);
#9470=EDGE_CURVE('',#7298,#7238,#3878,.T.);
#9471=EDGE_CURVE('',#7221,#7283,#3879,.T.);
#9472=EDGE_CURVE('',#7236,#7234,#3880,.T.);
#9473=EDGE_CURVE('',#7217,#7279,#3881,.T.);
#9474=EDGE_CURVE('',#7213,#7215,#3882,.T.);
#9475=EDGE_CURVE('',#7261,#7202,#3883,.T.);
#9476=EDGE_CURVE('',#7276,#7274,#3884,.T.);
#9477=EDGE_CURVE('',#7275,#7273,#3885,.T.);
#9478=EDGE_CURVE('',#7277,#7218,#3886,.T.);
#9479=EDGE_CURVE('',#7201,#7262,#3887,.T.);
#9480=EDGE_CURVE('',#7216,#7214,#3888,.T.);
#9481=EDGE_CURVE('',#7176,#7198,#3889,.T.);
#9482=EDGE_CURVE('',#7172,#7174,#3890,.T.);
#9483=EDGE_CURVE('',#7180,#7161,#3891,.T.);
#9484=EDGE_CURVE('',#7195,#7193,#3892,.T.);
#9485=EDGE_CURVE('',#7194,#7192,#3893,.T.);
#9486=EDGE_CURVE('',#7196,#7177,#3894,.T.);
#9487=EDGE_CURVE('',#7160,#7181,#3895,.T.);
#9488=EDGE_CURVE('',#7175,#7173,#3896,.T.);
#9489=EDGE_CURVE('',#7100,#7131,#3897,.T.);
#9490=EDGE_CURVE('',#7130,#7101,#3898,.T.);
#9491=EDGE_CURVE('',#7155,#7153,#3899,.T.);
#9492=EDGE_CURVE('',#7154,#7152,#3900,.T.);
#9493=EDGE_CURVE('',#7126,#7157,#3901,.T.);
#9494=EDGE_CURVE('',#7122,#7124,#3902,.T.);
#9495=EDGE_CURVE('',#7125,#7123,#3903,.T.);
#9496=EDGE_CURVE('',#7156,#7127,#3904,.T.);
#9497=EDGE_CURVE('',#7040,#7071,#3905,.T.);
#9498=EDGE_CURVE('',#7070,#7041,#3906,.T.);
#9499=EDGE_CURVE('',#7095,#7093,#3907,.T.);
#9500=EDGE_CURVE('',#7094,#7092,#3908,.T.);
#9501=EDGE_CURVE('',#7066,#7097,#3909,.T.);
#9502=EDGE_CURVE('',#7062,#7064,#3910,.T.);
#9503=EDGE_CURVE('',#7065,#7063,#3911,.T.);
#9504=EDGE_CURVE('',#7096,#7067,#3912,.T.);
#9505=EDGE_CURVE('',#6980,#7011,#3913,.T.);
#9506=EDGE_CURVE('',#7010,#6981,#3914,.T.);
#9507=EDGE_CURVE('',#7035,#7033,#3915,.T.);
#9508=EDGE_CURVE('',#7034,#7032,#3916,.T.);
#9509=EDGE_CURVE('',#7006,#7037,#3917,.T.);
#9510=EDGE_CURVE('',#7002,#7004,#3918,.T.);
#9511=EDGE_CURVE('',#7005,#7003,#3919,.T.);
#9512=EDGE_CURVE('',#7036,#7007,#3920,.T.);
#9513=EDGE_CURVE('',#6920,#6951,#3921,.T.);
#9514=EDGE_CURVE('',#6950,#6921,#3922,.T.);
#9515=EDGE_CURVE('',#6975,#6973,#3923,.T.);
#9516=EDGE_CURVE('',#6974,#6972,#3924,.T.);
#9517=EDGE_CURVE('',#6946,#6977,#3925,.T.);
#9518=EDGE_CURVE('',#6942,#6944,#3926,.T.);
#9519=EDGE_CURVE('',#6945,#6943,#3927,.T.);
#9520=EDGE_CURVE('',#6976,#6947,#3928,.T.);
#9521=EDGE_CURVE('',#6860,#6891,#3929,.T.);
#9522=EDGE_CURVE('',#6890,#6861,#3930,.T.);
#9523=EDGE_CURVE('',#6915,#6913,#3931,.T.);
#9524=EDGE_CURVE('',#6914,#6912,#3932,.T.);
#9525=EDGE_CURVE('',#6886,#6917,#3933,.T.);
#9526=EDGE_CURVE('',#6882,#6884,#3934,.T.);
#9527=EDGE_CURVE('',#6885,#6883,#3935,.T.);
#9528=EDGE_CURVE('',#6916,#6887,#3936,.T.);
#9529=EDGE_CURVE('',#6800,#6831,#3937,.T.);
#9530=EDGE_CURVE('',#6830,#6801,#3938,.T.);
#9531=EDGE_CURVE('',#6855,#6853,#3939,.T.);
#9532=EDGE_CURVE('',#6854,#6852,#3940,.T.);
#9533=EDGE_CURVE('',#6826,#6857,#3941,.T.);
#9534=EDGE_CURVE('',#6822,#6824,#3942,.T.);
#9535=EDGE_CURVE('',#6825,#6823,#3943,.T.);
#9536=EDGE_CURVE('',#6856,#6827,#3944,.T.);
#9537=EDGE_CURVE('',#6740,#6771,#3945,.T.);
#9538=EDGE_CURVE('',#6770,#6741,#3946,.T.);
#9539=EDGE_CURVE('',#6795,#6793,#3947,.T.);
#9540=EDGE_CURVE('',#6794,#6792,#3948,.T.);
#9541=EDGE_CURVE('',#6766,#6797,#3949,.T.);
#9542=EDGE_CURVE('',#6762,#6764,#3950,.T.);
#9543=EDGE_CURVE('',#6765,#6763,#3951,.T.);
#9544=EDGE_CURVE('',#6796,#6767,#3952,.T.);
#9545=EDGE_CURVE('',#6680,#6711,#3953,.T.);
#9546=EDGE_CURVE('',#6710,#6681,#3954,.T.);
#9547=EDGE_CURVE('',#6735,#6733,#3955,.T.);
#9548=EDGE_CURVE('',#6734,#6732,#3956,.T.);
#9549=EDGE_CURVE('',#6706,#6737,#3957,.T.);
#9550=EDGE_CURVE('',#6702,#6704,#3958,.T.);
#9551=EDGE_CURVE('',#6705,#6703,#3959,.T.);
#9552=EDGE_CURVE('',#6736,#6707,#3960,.T.);
#9553=EDGE_CURVE('',#6620,#6651,#3961,.T.);
#9554=EDGE_CURVE('',#6650,#6621,#3962,.T.);
#9555=EDGE_CURVE('',#6675,#6673,#3963,.T.);
#9556=EDGE_CURVE('',#6674,#6672,#3964,.T.);
#9557=EDGE_CURVE('',#6646,#6677,#3965,.T.);
#9558=EDGE_CURVE('',#6642,#6644,#3966,.T.);
#9559=EDGE_CURVE('',#6645,#6643,#3967,.T.);
#9560=EDGE_CURVE('',#6676,#6647,#3968,.T.);
#9561=EDGE_CURVE('',#6560,#6591,#3969,.T.);
#9562=EDGE_CURVE('',#6590,#6561,#3970,.T.);
#9563=EDGE_CURVE('',#6615,#6613,#3971,.T.);
#9564=EDGE_CURVE('',#6614,#6612,#3972,.T.);
#9565=EDGE_CURVE('',#6586,#6617,#3973,.T.);
#9566=EDGE_CURVE('',#6582,#6584,#3974,.T.);
#9567=EDGE_CURVE('',#6585,#6583,#3975,.T.);
#9568=EDGE_CURVE('',#6616,#6587,#3976,.T.);
#9569=EDGE_CURVE('',#6500,#6531,#3977,.T.);
#9570=EDGE_CURVE('',#6530,#6501,#3978,.T.);
#9571=EDGE_CURVE('',#6555,#6553,#3979,.T.);
#9572=EDGE_CURVE('',#6554,#6552,#3980,.T.);
#9573=EDGE_CURVE('',#6526,#6557,#3981,.T.);
#9574=EDGE_CURVE('',#6522,#6524,#3982,.T.);
#9575=EDGE_CURVE('',#6525,#6523,#3983,.T.);
#9576=EDGE_CURVE('',#6556,#6527,#3984,.T.);
#9577=EDGE_CURVE('',#6440,#6471,#3985,.T.);
#9578=EDGE_CURVE('',#6470,#6441,#3986,.T.);
#9579=EDGE_CURVE('',#6495,#6493,#3987,.T.);
#9580=EDGE_CURVE('',#6494,#6492,#3988,.T.);
#9581=EDGE_CURVE('',#6466,#6497,#3989,.T.);
#9582=EDGE_CURVE('',#6462,#6464,#3990,.T.);
#9583=EDGE_CURVE('',#6465,#6463,#3991,.T.);
#9584=EDGE_CURVE('',#6496,#6467,#3992,.T.);
#9585=EDGE_CURVE('',#7322,#7322,#2845,.T.);
#9586=EDGE_CURVE('',#7322,#7323,#5006,.T.);
#9587=EDGE_CURVE('',#7323,#7323,#2846,.T.);
#9588=EDGE_CURVE('',#7324,#7324,#2847,.T.);
#9589=EDGE_CURVE('',#7324,#7325,#5007,.T.);
#9590=EDGE_CURVE('',#7325,#7325,#2848,.T.);
#11018=ORIENTED_EDGE('',*,*,#8261,.T.);
#11019=ORIENTED_EDGE('',*,*,#8262,.T.);
#11020=ORIENTED_EDGE('',*,*,#8263,.T.);
#11021=ORIENTED_EDGE('',*,*,#8264,.T.);
#11022=ORIENTED_EDGE('',*,*,#8265,.T.);
#11023=ORIENTED_EDGE('',*,*,#8266,.T.);
#11024=ORIENTED_EDGE('',*,*,#8265,.F.);
#11025=ORIENTED_EDGE('',*,*,#8267,.T.);
#11026=ORIENTED_EDGE('',*,*,#8268,.T.);
#11027=ORIENTED_EDGE('',*,*,#8269,.T.);
#11028=ORIENTED_EDGE('',*,*,#8261,.F.);
#11029=ORIENTED_EDGE('',*,*,#8270,.T.);
#11030=ORIENTED_EDGE('',*,*,#8271,.T.);
#11031=ORIENTED_EDGE('',*,*,#8272,.T.);
#11032=ORIENTED_EDGE('',*,*,#8268,.F.);
#11033=ORIENTED_EDGE('',*,*,#8273,.T.);
#11034=ORIENTED_EDGE('',*,*,#8274,.T.);
#11035=ORIENTED_EDGE('',*,*,#8275,.T.);
#11036=ORIENTED_EDGE('',*,*,#8271,.F.);
#11037=ORIENTED_EDGE('',*,*,#8276,.T.);
#11038=ORIENTED_EDGE('',*,*,#8277,.T.);
#11039=ORIENTED_EDGE('',*,*,#8278,.T.);
#11040=ORIENTED_EDGE('',*,*,#8274,.F.);
#11041=ORIENTED_EDGE('',*,*,#8279,.T.);
#11042=ORIENTED_EDGE('',*,*,#8280,.T.);
#11043=ORIENTED_EDGE('',*,*,#8281,.T.);
#11044=ORIENTED_EDGE('',*,*,#8277,.F.);
#11045=ORIENTED_EDGE('',*,*,#8282,.T.);
#11046=ORIENTED_EDGE('',*,*,#8283,.T.);
#11047=ORIENTED_EDGE('',*,*,#8284,.T.);
#11048=ORIENTED_EDGE('',*,*,#8280,.F.);
#11049=ORIENTED_EDGE('',*,*,#8285,.T.);
#11050=ORIENTED_EDGE('',*,*,#8286,.T.);
#11051=ORIENTED_EDGE('',*,*,#8287,.T.);
#11052=ORIENTED_EDGE('',*,*,#8283,.F.);
#11053=ORIENTED_EDGE('',*,*,#8288,.T.);
#11054=ORIENTED_EDGE('',*,*,#8289,.T.);
#11055=ORIENTED_EDGE('',*,*,#8290,.T.);
#11056=ORIENTED_EDGE('',*,*,#8286,.F.);
#11057=ORIENTED_EDGE('',*,*,#8291,.T.);
#11058=ORIENTED_EDGE('',*,*,#8292,.T.);
#11059=ORIENTED_EDGE('',*,*,#8293,.T.);
#11060=ORIENTED_EDGE('',*,*,#8289,.F.);
#11061=ORIENTED_EDGE('',*,*,#8294,.T.);
#11062=ORIENTED_EDGE('',*,*,#8295,.T.);
#11063=ORIENTED_EDGE('',*,*,#8296,.T.);
#11064=ORIENTED_EDGE('',*,*,#8292,.F.);
#11065=ORIENTED_EDGE('',*,*,#8297,.T.);
#11066=ORIENTED_EDGE('',*,*,#8298,.F.);
#11067=ORIENTED_EDGE('',*,*,#8299,.T.);
#11068=ORIENTED_EDGE('',*,*,#8300,.F.);
#11069=ORIENTED_EDGE('',*,*,#8301,.T.);
#11070=ORIENTED_EDGE('',*,*,#8302,.T.);
#11071=ORIENTED_EDGE('',*,*,#8303,.T.);
#11072=ORIENTED_EDGE('',*,*,#8304,.F.);
#11073=ORIENTED_EDGE('',*,*,#8305,.F.);
#11074=ORIENTED_EDGE('',*,*,#8306,.T.);
#11075=ORIENTED_EDGE('',*,*,#8307,.T.);
#11076=ORIENTED_EDGE('',*,*,#8302,.F.);
#11077=ORIENTED_EDGE('',*,*,#8308,.F.);
#11078=ORIENTED_EDGE('',*,*,#8309,.T.);
#11079=ORIENTED_EDGE('',*,*,#8310,.T.);
#11080=ORIENTED_EDGE('',*,*,#8306,.F.);
#11081=ORIENTED_EDGE('',*,*,#8311,.F.);
#11082=ORIENTED_EDGE('',*,*,#8312,.T.);
#11083=ORIENTED_EDGE('',*,*,#8313,.T.);
#11084=ORIENTED_EDGE('',*,*,#8309,.F.);
#11085=ORIENTED_EDGE('',*,*,#8314,.F.);
#11086=ORIENTED_EDGE('',*,*,#8315,.T.);
#11087=ORIENTED_EDGE('',*,*,#8316,.T.);
#11088=ORIENTED_EDGE('',*,*,#8312,.F.);
#11089=ORIENTED_EDGE('',*,*,#8317,.F.);
#11090=ORIENTED_EDGE('',*,*,#8318,.T.);
#11091=ORIENTED_EDGE('',*,*,#8319,.T.);
#11092=ORIENTED_EDGE('',*,*,#8315,.F.);
#11093=ORIENTED_EDGE('',*,*,#8320,.F.);
#11094=ORIENTED_EDGE('',*,*,#8321,.T.);
#11095=ORIENTED_EDGE('',*,*,#8322,.T.);
#11096=ORIENTED_EDGE('',*,*,#8318,.F.);
#11097=ORIENTED_EDGE('',*,*,#8323,.F.);
#11098=ORIENTED_EDGE('',*,*,#8324,.T.);
#11099=ORIENTED_EDGE('',*,*,#8325,.T.);
#11100=ORIENTED_EDGE('',*,*,#8321,.F.);
#11101=ORIENTED_EDGE('',*,*,#8326,.F.);
#11102=ORIENTED_EDGE('',*,*,#8327,.T.);
#11103=ORIENTED_EDGE('',*,*,#8328,.T.);
#11104=ORIENTED_EDGE('',*,*,#8324,.F.);
#11105=ORIENTED_EDGE('',*,*,#8329,.F.);
#11106=ORIENTED_EDGE('',*,*,#8330,.T.);
#11107=ORIENTED_EDGE('',*,*,#8331,.T.);
#11108=ORIENTED_EDGE('',*,*,#8327,.F.);
#11109=ORIENTED_EDGE('',*,*,#8332,.F.);
#11110=ORIENTED_EDGE('',*,*,#8333,.T.);
#11111=ORIENTED_EDGE('',*,*,#8334,.T.);
#11112=ORIENTED_EDGE('',*,*,#8330,.F.);
#11113=ORIENTED_EDGE('',*,*,#8335,.F.);
#11114=ORIENTED_EDGE('',*,*,#8336,.T.);
#11115=ORIENTED_EDGE('',*,*,#8337,.T.);
#11116=ORIENTED_EDGE('',*,*,#8333,.F.);
#11117=ORIENTED_EDGE('',*,*,#8338,.F.);
#11118=ORIENTED_EDGE('',*,*,#8339,.F.);
#11119=ORIENTED_EDGE('',*,*,#8340,.F.);
#11120=ORIENTED_EDGE('',*,*,#8341,.F.);
#11121=ORIENTED_EDGE('',*,*,#8342,.T.);
#11122=ORIENTED_EDGE('',*,*,#8343,.T.);
#11123=ORIENTED_EDGE('',*,*,#8344,.T.);
#11124=ORIENTED_EDGE('',*,*,#8345,.T.);
#11125=ORIENTED_EDGE('',*,*,#8346,.T.);
#11126=ORIENTED_EDGE('',*,*,#8347,.T.);
#11127=ORIENTED_EDGE('',*,*,#8348,.T.);
#11128=ORIENTED_EDGE('',*,*,#8347,.F.);
#11129=ORIENTED_EDGE('',*,*,#8349,.T.);
#11130=ORIENTED_EDGE('',*,*,#8350,.T.);
#11131=ORIENTED_EDGE('',*,*,#8351,.T.);
#11132=ORIENTED_EDGE('',*,*,#8343,.F.);
#11133=ORIENTED_EDGE('',*,*,#8352,.T.);
#11134=ORIENTED_EDGE('',*,*,#8353,.T.);
#11135=ORIENTED_EDGE('',*,*,#8354,.T.);
#11136=ORIENTED_EDGE('',*,*,#8350,.F.);
#11137=ORIENTED_EDGE('',*,*,#8355,.T.);
#11138=ORIENTED_EDGE('',*,*,#8356,.T.);
#11139=ORIENTED_EDGE('',*,*,#8357,.T.);
#11140=ORIENTED_EDGE('',*,*,#8353,.F.);
#11141=ORIENTED_EDGE('',*,*,#8358,.T.);
#11142=ORIENTED_EDGE('',*,*,#8359,.T.);
#11143=ORIENTED_EDGE('',*,*,#8360,.T.);
#11144=ORIENTED_EDGE('',*,*,#8356,.F.);
#11145=ORIENTED_EDGE('',*,*,#8361,.T.);
#11146=ORIENTED_EDGE('',*,*,#8362,.T.);
#11147=ORIENTED_EDGE('',*,*,#8363,.T.);
#11148=ORIENTED_EDGE('',*,*,#8359,.F.);
#11149=ORIENTED_EDGE('',*,*,#8364,.T.);
#11150=ORIENTED_EDGE('',*,*,#8365,.T.);
#11151=ORIENTED_EDGE('',*,*,#8366,.T.);
#11152=ORIENTED_EDGE('',*,*,#8362,.F.);
#11153=ORIENTED_EDGE('',*,*,#8367,.T.);
#11154=ORIENTED_EDGE('',*,*,#8368,.T.);
#11155=ORIENTED_EDGE('',*,*,#8369,.T.);
#11156=ORIENTED_EDGE('',*,*,#8365,.F.);
#11157=ORIENTED_EDGE('',*,*,#8370,.T.);
#11158=ORIENTED_EDGE('',*,*,#8371,.T.);
#11159=ORIENTED_EDGE('',*,*,#8372,.T.);
#11160=ORIENTED_EDGE('',*,*,#8368,.F.);
#11161=ORIENTED_EDGE('',*,*,#8373,.T.);
#11162=ORIENTED_EDGE('',*,*,#8374,.T.);
#11163=ORIENTED_EDGE('',*,*,#8375,.T.);
#11164=ORIENTED_EDGE('',*,*,#8371,.F.);
#11165=ORIENTED_EDGE('',*,*,#8376,.T.);
#11166=ORIENTED_EDGE('',*,*,#8377,.T.);
#11167=ORIENTED_EDGE('',*,*,#8378,.T.);
#11168=ORIENTED_EDGE('',*,*,#8374,.F.);
#11169=ORIENTED_EDGE('',*,*,#8379,.T.);
#11170=ORIENTED_EDGE('',*,*,#8380,.F.);
#11171=ORIENTED_EDGE('',*,*,#8381,.T.);
#11172=ORIENTED_EDGE('',*,*,#8382,.F.);
#11173=ORIENTED_EDGE('',*,*,#8383,.T.);
#11174=ORIENTED_EDGE('',*,*,#8384,.T.);
#11175=ORIENTED_EDGE('',*,*,#8385,.T.);
#11176=ORIENTED_EDGE('',*,*,#8386,.F.);
#11177=ORIENTED_EDGE('',*,*,#8387,.F.);
#11178=ORIENTED_EDGE('',*,*,#8388,.T.);
#11179=ORIENTED_EDGE('',*,*,#8389,.T.);
#11180=ORIENTED_EDGE('',*,*,#8384,.F.);
#11181=ORIENTED_EDGE('',*,*,#8390,.F.);
#11182=ORIENTED_EDGE('',*,*,#8391,.T.);
#11183=ORIENTED_EDGE('',*,*,#8392,.T.);
#11184=ORIENTED_EDGE('',*,*,#8388,.F.);
#11185=ORIENTED_EDGE('',*,*,#8393,.F.);
#11186=ORIENTED_EDGE('',*,*,#8394,.T.);
#11187=ORIENTED_EDGE('',*,*,#8395,.T.);
#11188=ORIENTED_EDGE('',*,*,#8391,.F.);
#11189=ORIENTED_EDGE('',*,*,#8396,.F.);
#11190=ORIENTED_EDGE('',*,*,#8397,.T.);
#11191=ORIENTED_EDGE('',*,*,#8398,.T.);
#11192=ORIENTED_EDGE('',*,*,#8394,.F.);
#11193=ORIENTED_EDGE('',*,*,#8399,.F.);
#11194=ORIENTED_EDGE('',*,*,#8400,.T.);
#11195=ORIENTED_EDGE('',*,*,#8401,.T.);
#11196=ORIENTED_EDGE('',*,*,#8397,.F.);
#11197=ORIENTED_EDGE('',*,*,#8402,.F.);
#11198=ORIENTED_EDGE('',*,*,#8403,.T.);
#11199=ORIENTED_EDGE('',*,*,#8404,.T.);
#11200=ORIENTED_EDGE('',*,*,#8400,.F.);
#11201=ORIENTED_EDGE('',*,*,#8405,.F.);
#11202=ORIENTED_EDGE('',*,*,#8406,.T.);
#11203=ORIENTED_EDGE('',*,*,#8407,.T.);
#11204=ORIENTED_EDGE('',*,*,#8403,.F.);
#11205=ORIENTED_EDGE('',*,*,#8408,.F.);
#11206=ORIENTED_EDGE('',*,*,#8409,.T.);
#11207=ORIENTED_EDGE('',*,*,#8410,.T.);
#11208=ORIENTED_EDGE('',*,*,#8406,.F.);
#11209=ORIENTED_EDGE('',*,*,#8411,.F.);
#11210=ORIENTED_EDGE('',*,*,#8412,.T.);
#11211=ORIENTED_EDGE('',*,*,#8413,.T.);
#11212=ORIENTED_EDGE('',*,*,#8409,.F.);
#11213=ORIENTED_EDGE('',*,*,#8414,.F.);
#11214=ORIENTED_EDGE('',*,*,#8415,.T.);
#11215=ORIENTED_EDGE('',*,*,#8416,.T.);
#11216=ORIENTED_EDGE('',*,*,#8412,.F.);
#11217=ORIENTED_EDGE('',*,*,#8417,.F.);
#11218=ORIENTED_EDGE('',*,*,#8418,.T.);
#11219=ORIENTED_EDGE('',*,*,#8419,.T.);
#11220=ORIENTED_EDGE('',*,*,#8415,.F.);
#11221=ORIENTED_EDGE('',*,*,#8420,.F.);
#11222=ORIENTED_EDGE('',*,*,#8421,.F.);
#11223=ORIENTED_EDGE('',*,*,#8422,.F.);
#11224=ORIENTED_EDGE('',*,*,#8423,.F.);
#11225=ORIENTED_EDGE('',*,*,#8424,.T.);
#11226=ORIENTED_EDGE('',*,*,#8425,.T.);
#11227=ORIENTED_EDGE('',*,*,#8426,.T.);
#11228=ORIENTED_EDGE('',*,*,#8427,.T.);
#11229=ORIENTED_EDGE('',*,*,#8428,.T.);
#11230=ORIENTED_EDGE('',*,*,#8429,.T.);
#11231=ORIENTED_EDGE('',*,*,#8430,.T.);
#11232=ORIENTED_EDGE('',*,*,#8429,.F.);
#11233=ORIENTED_EDGE('',*,*,#8431,.T.);
#11234=ORIENTED_EDGE('',*,*,#8432,.T.);
#11235=ORIENTED_EDGE('',*,*,#8433,.T.);
#11236=ORIENTED_EDGE('',*,*,#8425,.F.);
#11237=ORIENTED_EDGE('',*,*,#8434,.T.);
#11238=ORIENTED_EDGE('',*,*,#8435,.T.);
#11239=ORIENTED_EDGE('',*,*,#8436,.T.);
#11240=ORIENTED_EDGE('',*,*,#8432,.F.);
#11241=ORIENTED_EDGE('',*,*,#8437,.T.);
#11242=ORIENTED_EDGE('',*,*,#8438,.T.);
#11243=ORIENTED_EDGE('',*,*,#8439,.T.);
#11244=ORIENTED_EDGE('',*,*,#8435,.F.);
#11245=ORIENTED_EDGE('',*,*,#8440,.T.);
#11246=ORIENTED_EDGE('',*,*,#8441,.T.);
#11247=ORIENTED_EDGE('',*,*,#8442,.T.);
#11248=ORIENTED_EDGE('',*,*,#8438,.F.);
#11249=ORIENTED_EDGE('',*,*,#8443,.T.);
#11250=ORIENTED_EDGE('',*,*,#8444,.T.);
#11251=ORIENTED_EDGE('',*,*,#8445,.T.);
#11252=ORIENTED_EDGE('',*,*,#8441,.F.);
#11253=ORIENTED_EDGE('',*,*,#8446,.T.);
#11254=ORIENTED_EDGE('',*,*,#8447,.T.);
#11255=ORIENTED_EDGE('',*,*,#8448,.T.);
#11256=ORIENTED_EDGE('',*,*,#8444,.F.);
#11257=ORIENTED_EDGE('',*,*,#8449,.T.);
#11258=ORIENTED_EDGE('',*,*,#8450,.T.);
#11259=ORIENTED_EDGE('',*,*,#8451,.T.);
#11260=ORIENTED_EDGE('',*,*,#8447,.F.);
#11261=ORIENTED_EDGE('',*,*,#8452,.T.);
#11262=ORIENTED_EDGE('',*,*,#8453,.T.);
#11263=ORIENTED_EDGE('',*,*,#8454,.T.);
#11264=ORIENTED_EDGE('',*,*,#8450,.F.);
#11265=ORIENTED_EDGE('',*,*,#8455,.T.);
#11266=ORIENTED_EDGE('',*,*,#8456,.T.);
#11267=ORIENTED_EDGE('',*,*,#8457,.T.);
#11268=ORIENTED_EDGE('',*,*,#8453,.F.);
#11269=ORIENTED_EDGE('',*,*,#8458,.T.);
#11270=ORIENTED_EDGE('',*,*,#8459,.T.);
#11271=ORIENTED_EDGE('',*,*,#8460,.T.);
#11272=ORIENTED_EDGE('',*,*,#8456,.F.);
#11273=ORIENTED_EDGE('',*,*,#8461,.T.);
#11274=ORIENTED_EDGE('',*,*,#8462,.F.);
#11275=ORIENTED_EDGE('',*,*,#8463,.T.);
#11276=ORIENTED_EDGE('',*,*,#8464,.F.);
#11277=ORIENTED_EDGE('',*,*,#8465,.T.);
#11278=ORIENTED_EDGE('',*,*,#8466,.T.);
#11279=ORIENTED_EDGE('',*,*,#8467,.T.);
#11280=ORIENTED_EDGE('',*,*,#8468,.F.);
#11281=ORIENTED_EDGE('',*,*,#8469,.F.);
#11282=ORIENTED_EDGE('',*,*,#8470,.T.);
#11283=ORIENTED_EDGE('',*,*,#8471,.T.);
#11284=ORIENTED_EDGE('',*,*,#8466,.F.);
#11285=ORIENTED_EDGE('',*,*,#8472,.F.);
#11286=ORIENTED_EDGE('',*,*,#8473,.T.);
#11287=ORIENTED_EDGE('',*,*,#8474,.T.);
#11288=ORIENTED_EDGE('',*,*,#8470,.F.);
#11289=ORIENTED_EDGE('',*,*,#8475,.F.);
#11290=ORIENTED_EDGE('',*,*,#8476,.T.);
#11291=ORIENTED_EDGE('',*,*,#8477,.T.);
#11292=ORIENTED_EDGE('',*,*,#8473,.F.);
#11293=ORIENTED_EDGE('',*,*,#8478,.F.);
#11294=ORIENTED_EDGE('',*,*,#8479,.T.);
#11295=ORIENTED_EDGE('',*,*,#8480,.T.);
#11296=ORIENTED_EDGE('',*,*,#8476,.F.);
#11297=ORIENTED_EDGE('',*,*,#8481,.F.);
#11298=ORIENTED_EDGE('',*,*,#8482,.T.);
#11299=ORIENTED_EDGE('',*,*,#8483,.T.);
#11300=ORIENTED_EDGE('',*,*,#8479,.F.);
#11301=ORIENTED_EDGE('',*,*,#8484,.F.);
#11302=ORIENTED_EDGE('',*,*,#8485,.T.);
#11303=ORIENTED_EDGE('',*,*,#8486,.T.);
#11304=ORIENTED_EDGE('',*,*,#8482,.F.);
#11305=ORIENTED_EDGE('',*,*,#8487,.F.);
#11306=ORIENTED_EDGE('',*,*,#8488,.T.);
#11307=ORIENTED_EDGE('',*,*,#8489,.T.);
#11308=ORIENTED_EDGE('',*,*,#8485,.F.);
#11309=ORIENTED_EDGE('',*,*,#8490,.F.);
#11310=ORIENTED_EDGE('',*,*,#8491,.T.);
#11311=ORIENTED_EDGE('',*,*,#8492,.T.);
#11312=ORIENTED_EDGE('',*,*,#8488,.F.);
#11313=ORIENTED_EDGE('',*,*,#8493,.F.);
#11314=ORIENTED_EDGE('',*,*,#8494,.T.);
#11315=ORIENTED_EDGE('',*,*,#8495,.T.);
#11316=ORIENTED_EDGE('',*,*,#8491,.F.);
#11317=ORIENTED_EDGE('',*,*,#8496,.F.);
#11318=ORIENTED_EDGE('',*,*,#8497,.T.);
#11319=ORIENTED_EDGE('',*,*,#8498,.T.);
#11320=ORIENTED_EDGE('',*,*,#8494,.F.);
#11321=ORIENTED_EDGE('',*,*,#8499,.F.);
#11322=ORIENTED_EDGE('',*,*,#8500,.T.);
#11323=ORIENTED_EDGE('',*,*,#8501,.T.);
#11324=ORIENTED_EDGE('',*,*,#8497,.F.);
#11325=ORIENTED_EDGE('',*,*,#8502,.F.);
#11326=ORIENTED_EDGE('',*,*,#8503,.F.);
#11327=ORIENTED_EDGE('',*,*,#8504,.F.);
#11328=ORIENTED_EDGE('',*,*,#8505,.F.);
#11329=ORIENTED_EDGE('',*,*,#8506,.T.);
#11330=ORIENTED_EDGE('',*,*,#8507,.T.);
#11331=ORIENTED_EDGE('',*,*,#8508,.T.);
#11332=ORIENTED_EDGE('',*,*,#8509,.T.);
#11333=ORIENTED_EDGE('',*,*,#8510,.T.);
#11334=ORIENTED_EDGE('',*,*,#8511,.T.);
#11335=ORIENTED_EDGE('',*,*,#8512,.T.);
#11336=ORIENTED_EDGE('',*,*,#8511,.F.);
#11337=ORIENTED_EDGE('',*,*,#8513,.T.);
#11338=ORIENTED_EDGE('',*,*,#8514,.T.);
#11339=ORIENTED_EDGE('',*,*,#8515,.T.);
#11340=ORIENTED_EDGE('',*,*,#8507,.F.);
#11341=ORIENTED_EDGE('',*,*,#8516,.T.);
#11342=ORIENTED_EDGE('',*,*,#8517,.T.);
#11343=ORIENTED_EDGE('',*,*,#8518,.T.);
#11344=ORIENTED_EDGE('',*,*,#8514,.F.);
#11345=ORIENTED_EDGE('',*,*,#8519,.T.);
#11346=ORIENTED_EDGE('',*,*,#8520,.T.);
#11347=ORIENTED_EDGE('',*,*,#8521,.T.);
#11348=ORIENTED_EDGE('',*,*,#8517,.F.);
#11349=ORIENTED_EDGE('',*,*,#8522,.T.);
#11350=ORIENTED_EDGE('',*,*,#8523,.T.);
#11351=ORIENTED_EDGE('',*,*,#8524,.T.);
#11352=ORIENTED_EDGE('',*,*,#8520,.F.);
#11353=ORIENTED_EDGE('',*,*,#8525,.T.);
#11354=ORIENTED_EDGE('',*,*,#8526,.T.);
#11355=ORIENTED_EDGE('',*,*,#8527,.T.);
#11356=ORIENTED_EDGE('',*,*,#8523,.F.);
#11357=ORIENTED_EDGE('',*,*,#8528,.T.);
#11358=ORIENTED_EDGE('',*,*,#8529,.T.);
#11359=ORIENTED_EDGE('',*,*,#8530,.T.);
#11360=ORIENTED_EDGE('',*,*,#8526,.F.);
#11361=ORIENTED_EDGE('',*,*,#8531,.T.);
#11362=ORIENTED_EDGE('',*,*,#8532,.T.);
#11363=ORIENTED_EDGE('',*,*,#8533,.T.);
#11364=ORIENTED_EDGE('',*,*,#8529,.F.);
#11365=ORIENTED_EDGE('',*,*,#8534,.T.);
#11366=ORIENTED_EDGE('',*,*,#8535,.T.);
#11367=ORIENTED_EDGE('',*,*,#8536,.T.);
#11368=ORIENTED_EDGE('',*,*,#8532,.F.);
#11369=ORIENTED_EDGE('',*,*,#8537,.T.);
#11370=ORIENTED_EDGE('',*,*,#8538,.T.);
#11371=ORIENTED_EDGE('',*,*,#8539,.T.);
#11372=ORIENTED_EDGE('',*,*,#8535,.F.);
#11373=ORIENTED_EDGE('',*,*,#8540,.T.);
#11374=ORIENTED_EDGE('',*,*,#8541,.T.);
#11375=ORIENTED_EDGE('',*,*,#8542,.T.);
#11376=ORIENTED_EDGE('',*,*,#8538,.F.);
#11377=ORIENTED_EDGE('',*,*,#8543,.T.);
#11378=ORIENTED_EDGE('',*,*,#8544,.F.);
#11379=ORIENTED_EDGE('',*,*,#8545,.T.);
#11380=ORIENTED_EDGE('',*,*,#8546,.F.);
#11381=ORIENTED_EDGE('',*,*,#8547,.T.);
#11382=ORIENTED_EDGE('',*,*,#8548,.T.);
#11383=ORIENTED_EDGE('',*,*,#8549,.T.);
#11384=ORIENTED_EDGE('',*,*,#8550,.F.);
#11385=ORIENTED_EDGE('',*,*,#8551,.F.);
#11386=ORIENTED_EDGE('',*,*,#8552,.T.);
#11387=ORIENTED_EDGE('',*,*,#8553,.T.);
#11388=ORIENTED_EDGE('',*,*,#8548,.F.);
#11389=ORIENTED_EDGE('',*,*,#8554,.F.);
#11390=ORIENTED_EDGE('',*,*,#8555,.T.);
#11391=ORIENTED_EDGE('',*,*,#8556,.T.);
#11392=ORIENTED_EDGE('',*,*,#8552,.F.);
#11393=ORIENTED_EDGE('',*,*,#8557,.F.);
#11394=ORIENTED_EDGE('',*,*,#8558,.T.);
#11395=ORIENTED_EDGE('',*,*,#8559,.T.);
#11396=ORIENTED_EDGE('',*,*,#8555,.F.);
#11397=ORIENTED_EDGE('',*,*,#8560,.F.);
#11398=ORIENTED_EDGE('',*,*,#8561,.T.);
#11399=ORIENTED_EDGE('',*,*,#8562,.T.);
#11400=ORIENTED_EDGE('',*,*,#8558,.F.);
#11401=ORIENTED_EDGE('',*,*,#8563,.F.);
#11402=ORIENTED_EDGE('',*,*,#8564,.T.);
#11403=ORIENTED_EDGE('',*,*,#8565,.T.);
#11404=ORIENTED_EDGE('',*,*,#8561,.F.);
#11405=ORIENTED_EDGE('',*,*,#8566,.F.);
#11406=ORIENTED_EDGE('',*,*,#8567,.T.);
#11407=ORIENTED_EDGE('',*,*,#8568,.T.);
#11408=ORIENTED_EDGE('',*,*,#8564,.F.);
#11409=ORIENTED_EDGE('',*,*,#8569,.F.);
#11410=ORIENTED_EDGE('',*,*,#8570,.T.);
#11411=ORIENTED_EDGE('',*,*,#8571,.T.);
#11412=ORIENTED_EDGE('',*,*,#8567,.F.);
#11413=ORIENTED_EDGE('',*,*,#8572,.F.);
#11414=ORIENTED_EDGE('',*,*,#8573,.T.);
#11415=ORIENTED_EDGE('',*,*,#8574,.T.);
#11416=ORIENTED_EDGE('',*,*,#8570,.F.);
#11417=ORIENTED_EDGE('',*,*,#8575,.F.);
#11418=ORIENTED_EDGE('',*,*,#8576,.T.);
#11419=ORIENTED_EDGE('',*,*,#8577,.T.);
#11420=ORIENTED_EDGE('',*,*,#8573,.F.);
#11421=ORIENTED_EDGE('',*,*,#8578,.F.);
#11422=ORIENTED_EDGE('',*,*,#8579,.T.);
#11423=ORIENTED_EDGE('',*,*,#8580,.T.);
#11424=ORIENTED_EDGE('',*,*,#8576,.F.);
#11425=ORIENTED_EDGE('',*,*,#8581,.F.);
#11426=ORIENTED_EDGE('',*,*,#8582,.T.);
#11427=ORIENTED_EDGE('',*,*,#8583,.T.);
#11428=ORIENTED_EDGE('',*,*,#8579,.F.);
#11429=ORIENTED_EDGE('',*,*,#8584,.F.);
#11430=ORIENTED_EDGE('',*,*,#8585,.F.);
#11431=ORIENTED_EDGE('',*,*,#8586,.F.);
#11432=ORIENTED_EDGE('',*,*,#8587,.F.);
#11433=ORIENTED_EDGE('',*,*,#8588,.T.);
#11434=ORIENTED_EDGE('',*,*,#8589,.T.);
#11435=ORIENTED_EDGE('',*,*,#8590,.T.);
#11436=ORIENTED_EDGE('',*,*,#8591,.T.);
#11437=ORIENTED_EDGE('',*,*,#8592,.T.);
#11438=ORIENTED_EDGE('',*,*,#8593,.T.);
#11439=ORIENTED_EDGE('',*,*,#8594,.T.);
#11440=ORIENTED_EDGE('',*,*,#8593,.F.);
#11441=ORIENTED_EDGE('',*,*,#8595,.T.);
#11442=ORIENTED_EDGE('',*,*,#8596,.T.);
#11443=ORIENTED_EDGE('',*,*,#8597,.T.);
#11444=ORIENTED_EDGE('',*,*,#8589,.F.);
#11445=ORIENTED_EDGE('',*,*,#8598,.T.);
#11446=ORIENTED_EDGE('',*,*,#8599,.T.);
#11447=ORIENTED_EDGE('',*,*,#8600,.T.);
#11448=ORIENTED_EDGE('',*,*,#8596,.F.);
#11449=ORIENTED_EDGE('',*,*,#8601,.T.);
#11450=ORIENTED_EDGE('',*,*,#8602,.T.);
#11451=ORIENTED_EDGE('',*,*,#8603,.T.);
#11452=ORIENTED_EDGE('',*,*,#8599,.F.);
#11453=ORIENTED_EDGE('',*,*,#8604,.T.);
#11454=ORIENTED_EDGE('',*,*,#8605,.T.);
#11455=ORIENTED_EDGE('',*,*,#8606,.T.);
#11456=ORIENTED_EDGE('',*,*,#8602,.F.);
#11457=ORIENTED_EDGE('',*,*,#8607,.T.);
#11458=ORIENTED_EDGE('',*,*,#8608,.T.);
#11459=ORIENTED_EDGE('',*,*,#8609,.T.);
#11460=ORIENTED_EDGE('',*,*,#8605,.F.);
#11461=ORIENTED_EDGE('',*,*,#8610,.T.);
#11462=ORIENTED_EDGE('',*,*,#8611,.T.);
#11463=ORIENTED_EDGE('',*,*,#8612,.T.);
#11464=ORIENTED_EDGE('',*,*,#8608,.F.);
#11465=ORIENTED_EDGE('',*,*,#8613,.T.);
#11466=ORIENTED_EDGE('',*,*,#8614,.T.);
#11467=ORIENTED_EDGE('',*,*,#8615,.T.);
#11468=ORIENTED_EDGE('',*,*,#8611,.F.);
#11469=ORIENTED_EDGE('',*,*,#8616,.T.);
#11470=ORIENTED_EDGE('',*,*,#8617,.T.);
#11471=ORIENTED_EDGE('',*,*,#8618,.T.);
#11472=ORIENTED_EDGE('',*,*,#8614,.F.);
#11473=ORIENTED_EDGE('',*,*,#8619,.T.);
#11474=ORIENTED_EDGE('',*,*,#8620,.T.);
#11475=ORIENTED_EDGE('',*,*,#8621,.T.);
#11476=ORIENTED_EDGE('',*,*,#8617,.F.);
#11477=ORIENTED_EDGE('',*,*,#8622,.T.);
#11478=ORIENTED_EDGE('',*,*,#8623,.T.);
#11479=ORIENTED_EDGE('',*,*,#8624,.T.);
#11480=ORIENTED_EDGE('',*,*,#8620,.F.);
#11481=ORIENTED_EDGE('',*,*,#8625,.T.);
#11482=ORIENTED_EDGE('',*,*,#8626,.F.);
#11483=ORIENTED_EDGE('',*,*,#8627,.T.);
#11484=ORIENTED_EDGE('',*,*,#8628,.F.);
#11485=ORIENTED_EDGE('',*,*,#8629,.T.);
#11486=ORIENTED_EDGE('',*,*,#8630,.T.);
#11487=ORIENTED_EDGE('',*,*,#8631,.T.);
#11488=ORIENTED_EDGE('',*,*,#8632,.F.);
#11489=ORIENTED_EDGE('',*,*,#8633,.F.);
#11490=ORIENTED_EDGE('',*,*,#8634,.T.);
#11491=ORIENTED_EDGE('',*,*,#8635,.T.);
#11492=ORIENTED_EDGE('',*,*,#8630,.F.);
#11493=ORIENTED_EDGE('',*,*,#8636,.F.);
#11494=ORIENTED_EDGE('',*,*,#8637,.T.);
#11495=ORIENTED_EDGE('',*,*,#8638,.T.);
#11496=ORIENTED_EDGE('',*,*,#8634,.F.);
#11497=ORIENTED_EDGE('',*,*,#8639,.F.);
#11498=ORIENTED_EDGE('',*,*,#8640,.T.);
#11499=ORIENTED_EDGE('',*,*,#8641,.T.);
#11500=ORIENTED_EDGE('',*,*,#8637,.F.);
#11501=ORIENTED_EDGE('',*,*,#8642,.F.);
#11502=ORIENTED_EDGE('',*,*,#8643,.T.);
#11503=ORIENTED_EDGE('',*,*,#8644,.T.);
#11504=ORIENTED_EDGE('',*,*,#8640,.F.);
#11505=ORIENTED_EDGE('',*,*,#8645,.F.);
#11506=ORIENTED_EDGE('',*,*,#8646,.T.);
#11507=ORIENTED_EDGE('',*,*,#8647,.T.);
#11508=ORIENTED_EDGE('',*,*,#8643,.F.);
#11509=ORIENTED_EDGE('',*,*,#8648,.F.);
#11510=ORIENTED_EDGE('',*,*,#8649,.T.);
#11511=ORIENTED_EDGE('',*,*,#8650,.T.);
#11512=ORIENTED_EDGE('',*,*,#8646,.F.);
#11513=ORIENTED_EDGE('',*,*,#8651,.F.);
#11514=ORIENTED_EDGE('',*,*,#8652,.T.);
#11515=ORIENTED_EDGE('',*,*,#8653,.T.);
#11516=ORIENTED_EDGE('',*,*,#8649,.F.);
#11517=ORIENTED_EDGE('',*,*,#8654,.F.);
#11518=ORIENTED_EDGE('',*,*,#8655,.T.);
#11519=ORIENTED_EDGE('',*,*,#8656,.T.);
#11520=ORIENTED_EDGE('',*,*,#8652,.F.);
#11521=ORIENTED_EDGE('',*,*,#8657,.F.);
#11522=ORIENTED_EDGE('',*,*,#8658,.T.);
#11523=ORIENTED_EDGE('',*,*,#8659,.T.);
#11524=ORIENTED_EDGE('',*,*,#8655,.F.);
#11525=ORIENTED_EDGE('',*,*,#8660,.F.);
#11526=ORIENTED_EDGE('',*,*,#8661,.T.);
#11527=ORIENTED_EDGE('',*,*,#8662,.T.);
#11528=ORIENTED_EDGE('',*,*,#8658,.F.);
#11529=ORIENTED_EDGE('',*,*,#8663,.F.);
#11530=ORIENTED_EDGE('',*,*,#8664,.T.);
#11531=ORIENTED_EDGE('',*,*,#8665,.T.);
#11532=ORIENTED_EDGE('',*,*,#8661,.F.);
#11533=ORIENTED_EDGE('',*,*,#8666,.F.);
#11534=ORIENTED_EDGE('',*,*,#8667,.F.);
#11535=ORIENTED_EDGE('',*,*,#8668,.F.);
#11536=ORIENTED_EDGE('',*,*,#8669,.F.);
#11537=ORIENTED_EDGE('',*,*,#8670,.T.);
#11538=ORIENTED_EDGE('',*,*,#8671,.T.);
#11539=ORIENTED_EDGE('',*,*,#8672,.T.);
#11540=ORIENTED_EDGE('',*,*,#8673,.T.);
#11541=ORIENTED_EDGE('',*,*,#8674,.T.);
#11542=ORIENTED_EDGE('',*,*,#8675,.T.);
#11543=ORIENTED_EDGE('',*,*,#8676,.T.);
#11544=ORIENTED_EDGE('',*,*,#8675,.F.);
#11545=ORIENTED_EDGE('',*,*,#8677,.T.);
#11546=ORIENTED_EDGE('',*,*,#8678,.T.);
#11547=ORIENTED_EDGE('',*,*,#8679,.T.);
#11548=ORIENTED_EDGE('',*,*,#8671,.F.);
#11549=ORIENTED_EDGE('',*,*,#8680,.T.);
#11550=ORIENTED_EDGE('',*,*,#8681,.T.);
#11551=ORIENTED_EDGE('',*,*,#8682,.T.);
#11552=ORIENTED_EDGE('',*,*,#8678,.F.);
#11553=ORIENTED_EDGE('',*,*,#8683,.T.);
#11554=ORIENTED_EDGE('',*,*,#8684,.T.);
#11555=ORIENTED_EDGE('',*,*,#8685,.T.);
#11556=ORIENTED_EDGE('',*,*,#8681,.F.);
#11557=ORIENTED_EDGE('',*,*,#8686,.T.);
#11558=ORIENTED_EDGE('',*,*,#8687,.T.);
#11559=ORIENTED_EDGE('',*,*,#8688,.T.);
#11560=ORIENTED_EDGE('',*,*,#8684,.F.);
#11561=ORIENTED_EDGE('',*,*,#8689,.T.);
#11562=ORIENTED_EDGE('',*,*,#8690,.T.);
#11563=ORIENTED_EDGE('',*,*,#8691,.T.);
#11564=ORIENTED_EDGE('',*,*,#8687,.F.);
#11565=ORIENTED_EDGE('',*,*,#8692,.T.);
#11566=ORIENTED_EDGE('',*,*,#8693,.T.);
#11567=ORIENTED_EDGE('',*,*,#8694,.T.);
#11568=ORIENTED_EDGE('',*,*,#8690,.F.);
#11569=ORIENTED_EDGE('',*,*,#8695,.T.);
#11570=ORIENTED_EDGE('',*,*,#8696,.T.);
#11571=ORIENTED_EDGE('',*,*,#8697,.T.);
#11572=ORIENTED_EDGE('',*,*,#8693,.F.);
#11573=ORIENTED_EDGE('',*,*,#8698,.T.);
#11574=ORIENTED_EDGE('',*,*,#8699,.T.);
#11575=ORIENTED_EDGE('',*,*,#8700,.T.);
#11576=ORIENTED_EDGE('',*,*,#8696,.F.);
#11577=ORIENTED_EDGE('',*,*,#8701,.T.);
#11578=ORIENTED_EDGE('',*,*,#8702,.T.);
#11579=ORIENTED_EDGE('',*,*,#8703,.T.);
#11580=ORIENTED_EDGE('',*,*,#8699,.F.);
#11581=ORIENTED_EDGE('',*,*,#8704,.T.);
#11582=ORIENTED_EDGE('',*,*,#8705,.T.);
#11583=ORIENTED_EDGE('',*,*,#8706,.T.);
#11584=ORIENTED_EDGE('',*,*,#8702,.F.);
#11585=ORIENTED_EDGE('',*,*,#8707,.T.);
#11586=ORIENTED_EDGE('',*,*,#8708,.F.);
#11587=ORIENTED_EDGE('',*,*,#8709,.T.);
#11588=ORIENTED_EDGE('',*,*,#8710,.F.);
#11589=ORIENTED_EDGE('',*,*,#8711,.T.);
#11590=ORIENTED_EDGE('',*,*,#8712,.T.);
#11591=ORIENTED_EDGE('',*,*,#8713,.T.);
#11592=ORIENTED_EDGE('',*,*,#8714,.F.);
#11593=ORIENTED_EDGE('',*,*,#8715,.F.);
#11594=ORIENTED_EDGE('',*,*,#8716,.T.);
#11595=ORIENTED_EDGE('',*,*,#8717,.T.);
#11596=ORIENTED_EDGE('',*,*,#8712,.F.);
#11597=ORIENTED_EDGE('',*,*,#8718,.F.);
#11598=ORIENTED_EDGE('',*,*,#8719,.T.);
#11599=ORIENTED_EDGE('',*,*,#8720,.T.);
#11600=ORIENTED_EDGE('',*,*,#8716,.F.);
#11601=ORIENTED_EDGE('',*,*,#8721,.F.);
#11602=ORIENTED_EDGE('',*,*,#8722,.T.);
#11603=ORIENTED_EDGE('',*,*,#8723,.T.);
#11604=ORIENTED_EDGE('',*,*,#8719,.F.);
#11605=ORIENTED_EDGE('',*,*,#8724,.F.);
#11606=ORIENTED_EDGE('',*,*,#8725,.T.);
#11607=ORIENTED_EDGE('',*,*,#8726,.T.);
#11608=ORIENTED_EDGE('',*,*,#8722,.F.);
#11609=ORIENTED_EDGE('',*,*,#8727,.F.);
#11610=ORIENTED_EDGE('',*,*,#8728,.T.);
#11611=ORIENTED_EDGE('',*,*,#8729,.T.);
#11612=ORIENTED_EDGE('',*,*,#8725,.F.);
#11613=ORIENTED_EDGE('',*,*,#8730,.F.);
#11614=ORIENTED_EDGE('',*,*,#8731,.T.);
#11615=ORIENTED_EDGE('',*,*,#8732,.T.);
#11616=ORIENTED_EDGE('',*,*,#8728,.F.);
#11617=ORIENTED_EDGE('',*,*,#8733,.F.);
#11618=ORIENTED_EDGE('',*,*,#8734,.T.);
#11619=ORIENTED_EDGE('',*,*,#8735,.T.);
#11620=ORIENTED_EDGE('',*,*,#8731,.F.);
#11621=ORIENTED_EDGE('',*,*,#8736,.F.);
#11622=ORIENTED_EDGE('',*,*,#8737,.T.);
#11623=ORIENTED_EDGE('',*,*,#8738,.T.);
#11624=ORIENTED_EDGE('',*,*,#8734,.F.);
#11625=ORIENTED_EDGE('',*,*,#8739,.F.);
#11626=ORIENTED_EDGE('',*,*,#8740,.T.);
#11627=ORIENTED_EDGE('',*,*,#8741,.T.);
#11628=ORIENTED_EDGE('',*,*,#8737,.F.);
#11629=ORIENTED_EDGE('',*,*,#8742,.F.);
#11630=ORIENTED_EDGE('',*,*,#8743,.T.);
#11631=ORIENTED_EDGE('',*,*,#8744,.T.);
#11632=ORIENTED_EDGE('',*,*,#8740,.F.);
#11633=ORIENTED_EDGE('',*,*,#8745,.F.);
#11634=ORIENTED_EDGE('',*,*,#8746,.T.);
#11635=ORIENTED_EDGE('',*,*,#8747,.T.);
#11636=ORIENTED_EDGE('',*,*,#8743,.F.);
#11637=ORIENTED_EDGE('',*,*,#8748,.F.);
#11638=ORIENTED_EDGE('',*,*,#8749,.F.);
#11639=ORIENTED_EDGE('',*,*,#8750,.F.);
#11640=ORIENTED_EDGE('',*,*,#8751,.F.);
#11641=ORIENTED_EDGE('',*,*,#8752,.T.);
#11642=ORIENTED_EDGE('',*,*,#8753,.T.);
#11643=ORIENTED_EDGE('',*,*,#8754,.T.);
#11644=ORIENTED_EDGE('',*,*,#8755,.T.);
#11645=ORIENTED_EDGE('',*,*,#8756,.T.);
#11646=ORIENTED_EDGE('',*,*,#8757,.T.);
#11647=ORIENTED_EDGE('',*,*,#8758,.T.);
#11648=ORIENTED_EDGE('',*,*,#8757,.F.);
#11649=ORIENTED_EDGE('',*,*,#8759,.T.);
#11650=ORIENTED_EDGE('',*,*,#8760,.T.);
#11651=ORIENTED_EDGE('',*,*,#8761,.T.);
#11652=ORIENTED_EDGE('',*,*,#8753,.F.);
#11653=ORIENTED_EDGE('',*,*,#8762,.T.);
#11654=ORIENTED_EDGE('',*,*,#8763,.T.);
#11655=ORIENTED_EDGE('',*,*,#8764,.T.);
#11656=ORIENTED_EDGE('',*,*,#8760,.F.);
#11657=ORIENTED_EDGE('',*,*,#8765,.T.);
#11658=ORIENTED_EDGE('',*,*,#8766,.T.);
#11659=ORIENTED_EDGE('',*,*,#8767,.T.);
#11660=ORIENTED_EDGE('',*,*,#8763,.F.);
#11661=ORIENTED_EDGE('',*,*,#8768,.T.);
#11662=ORIENTED_EDGE('',*,*,#8769,.T.);
#11663=ORIENTED_EDGE('',*,*,#8770,.T.);
#11664=ORIENTED_EDGE('',*,*,#8766,.F.);
#11665=ORIENTED_EDGE('',*,*,#8771,.T.);
#11666=ORIENTED_EDGE('',*,*,#8772,.T.);
#11667=ORIENTED_EDGE('',*,*,#8773,.T.);
#11668=ORIENTED_EDGE('',*,*,#8769,.F.);
#11669=ORIENTED_EDGE('',*,*,#8774,.T.);
#11670=ORIENTED_EDGE('',*,*,#8775,.T.);
#11671=ORIENTED_EDGE('',*,*,#8776,.T.);
#11672=ORIENTED_EDGE('',*,*,#8772,.F.);
#11673=ORIENTED_EDGE('',*,*,#8777,.T.);
#11674=ORIENTED_EDGE('',*,*,#8778,.T.);
#11675=ORIENTED_EDGE('',*,*,#8779,.T.);
#11676=ORIENTED_EDGE('',*,*,#8775,.F.);
#11677=ORIENTED_EDGE('',*,*,#8780,.T.);
#11678=ORIENTED_EDGE('',*,*,#8781,.T.);
#11679=ORIENTED_EDGE('',*,*,#8782,.T.);
#11680=ORIENTED_EDGE('',*,*,#8778,.F.);
#11681=ORIENTED_EDGE('',*,*,#8783,.T.);
#11682=ORIENTED_EDGE('',*,*,#8784,.T.);
#11683=ORIENTED_EDGE('',*,*,#8785,.T.);
#11684=ORIENTED_EDGE('',*,*,#8781,.F.);
#11685=ORIENTED_EDGE('',*,*,#8786,.T.);
#11686=ORIENTED_EDGE('',*,*,#8787,.T.);
#11687=ORIENTED_EDGE('',*,*,#8788,.T.);
#11688=ORIENTED_EDGE('',*,*,#8784,.F.);
#11689=ORIENTED_EDGE('',*,*,#8789,.T.);
#11690=ORIENTED_EDGE('',*,*,#8790,.F.);
#11691=ORIENTED_EDGE('',*,*,#8791,.T.);
#11692=ORIENTED_EDGE('',*,*,#8792,.F.);
#11693=ORIENTED_EDGE('',*,*,#8793,.T.);
#11694=ORIENTED_EDGE('',*,*,#8794,.T.);
#11695=ORIENTED_EDGE('',*,*,#8795,.T.);
#11696=ORIENTED_EDGE('',*,*,#8796,.F.);
#11697=ORIENTED_EDGE('',*,*,#8797,.F.);
#11698=ORIENTED_EDGE('',*,*,#8798,.T.);
#11699=ORIENTED_EDGE('',*,*,#8799,.T.);
#11700=ORIENTED_EDGE('',*,*,#8794,.F.);
#11701=ORIENTED_EDGE('',*,*,#8800,.F.);
#11702=ORIENTED_EDGE('',*,*,#8801,.T.);
#11703=ORIENTED_EDGE('',*,*,#8802,.T.);
#11704=ORIENTED_EDGE('',*,*,#8798,.F.);
#11705=ORIENTED_EDGE('',*,*,#8803,.F.);
#11706=ORIENTED_EDGE('',*,*,#8804,.T.);
#11707=ORIENTED_EDGE('',*,*,#8805,.T.);
#11708=ORIENTED_EDGE('',*,*,#8801,.F.);
#11709=ORIENTED_EDGE('',*,*,#8806,.F.);
#11710=ORIENTED_EDGE('',*,*,#8807,.T.);
#11711=ORIENTED_EDGE('',*,*,#8808,.T.);
#11712=ORIENTED_EDGE('',*,*,#8804,.F.);
#11713=ORIENTED_EDGE('',*,*,#8809,.F.);
#11714=ORIENTED_EDGE('',*,*,#8810,.T.);
#11715=ORIENTED_EDGE('',*,*,#8811,.T.);
#11716=ORIENTED_EDGE('',*,*,#8807,.F.);
#11717=ORIENTED_EDGE('',*,*,#8812,.F.);
#11718=ORIENTED_EDGE('',*,*,#8813,.T.);
#11719=ORIENTED_EDGE('',*,*,#8814,.T.);
#11720=ORIENTED_EDGE('',*,*,#8810,.F.);
#11721=ORIENTED_EDGE('',*,*,#8815,.F.);
#11722=ORIENTED_EDGE('',*,*,#8816,.T.);
#11723=ORIENTED_EDGE('',*,*,#8817,.T.);
#11724=ORIENTED_EDGE('',*,*,#8813,.F.);
#11725=ORIENTED_EDGE('',*,*,#8818,.F.);
#11726=ORIENTED_EDGE('',*,*,#8819,.T.);
#11727=ORIENTED_EDGE('',*,*,#8820,.T.);
#11728=ORIENTED_EDGE('',*,*,#8816,.F.);
#11729=ORIENTED_EDGE('',*,*,#8821,.F.);
#11730=ORIENTED_EDGE('',*,*,#8822,.T.);
#11731=ORIENTED_EDGE('',*,*,#8823,.T.);
#11732=ORIENTED_EDGE('',*,*,#8819,.F.);
#11733=ORIENTED_EDGE('',*,*,#8824,.F.);
#11734=ORIENTED_EDGE('',*,*,#8825,.T.);
#11735=ORIENTED_EDGE('',*,*,#8826,.T.);
#11736=ORIENTED_EDGE('',*,*,#8822,.F.);
#11737=ORIENTED_EDGE('',*,*,#8827,.F.);
#11738=ORIENTED_EDGE('',*,*,#8828,.T.);
#11739=ORIENTED_EDGE('',*,*,#8829,.T.);
#11740=ORIENTED_EDGE('',*,*,#8825,.F.);
#11741=ORIENTED_EDGE('',*,*,#8830,.F.);
#11742=ORIENTED_EDGE('',*,*,#8831,.F.);
#11743=ORIENTED_EDGE('',*,*,#8832,.F.);
#11744=ORIENTED_EDGE('',*,*,#8833,.F.);
#11745=ORIENTED_EDGE('',*,*,#8834,.T.);
#11746=ORIENTED_EDGE('',*,*,#8835,.T.);
#11747=ORIENTED_EDGE('',*,*,#8836,.T.);
#11748=ORIENTED_EDGE('',*,*,#8837,.T.);
#11749=ORIENTED_EDGE('',*,*,#8838,.T.);
#11750=ORIENTED_EDGE('',*,*,#8839,.T.);
#11751=ORIENTED_EDGE('',*,*,#8840,.T.);
#11752=ORIENTED_EDGE('',*,*,#8839,.F.);
#11753=ORIENTED_EDGE('',*,*,#8841,.T.);
#11754=ORIENTED_EDGE('',*,*,#8842,.T.);
#11755=ORIENTED_EDGE('',*,*,#8843,.T.);
#11756=ORIENTED_EDGE('',*,*,#8835,.F.);
#11757=ORIENTED_EDGE('',*,*,#8844,.T.);
#11758=ORIENTED_EDGE('',*,*,#8845,.T.);
#11759=ORIENTED_EDGE('',*,*,#8846,.T.);
#11760=ORIENTED_EDGE('',*,*,#8842,.F.);
#11761=ORIENTED_EDGE('',*,*,#8847,.T.);
#11762=ORIENTED_EDGE('',*,*,#8848,.T.);
#11763=ORIENTED_EDGE('',*,*,#8849,.T.);
#11764=ORIENTED_EDGE('',*,*,#8845,.F.);
#11765=ORIENTED_EDGE('',*,*,#8850,.T.);
#11766=ORIENTED_EDGE('',*,*,#8851,.T.);
#11767=ORIENTED_EDGE('',*,*,#8852,.T.);
#11768=ORIENTED_EDGE('',*,*,#8848,.F.);
#11769=ORIENTED_EDGE('',*,*,#8853,.T.);
#11770=ORIENTED_EDGE('',*,*,#8854,.T.);
#11771=ORIENTED_EDGE('',*,*,#8855,.T.);
#11772=ORIENTED_EDGE('',*,*,#8851,.F.);
#11773=ORIENTED_EDGE('',*,*,#8856,.T.);
#11774=ORIENTED_EDGE('',*,*,#8857,.T.);
#11775=ORIENTED_EDGE('',*,*,#8858,.T.);
#11776=ORIENTED_EDGE('',*,*,#8854,.F.);
#11777=ORIENTED_EDGE('',*,*,#8859,.T.);
#11778=ORIENTED_EDGE('',*,*,#8860,.T.);
#11779=ORIENTED_EDGE('',*,*,#8861,.T.);
#11780=ORIENTED_EDGE('',*,*,#8857,.F.);
#11781=ORIENTED_EDGE('',*,*,#8862,.T.);
#11782=ORIENTED_EDGE('',*,*,#8863,.T.);
#11783=ORIENTED_EDGE('',*,*,#8864,.T.);
#11784=ORIENTED_EDGE('',*,*,#8860,.F.);
#11785=ORIENTED_EDGE('',*,*,#8865,.T.);
#11786=ORIENTED_EDGE('',*,*,#8866,.T.);
#11787=ORIENTED_EDGE('',*,*,#8867,.T.);
#11788=ORIENTED_EDGE('',*,*,#8863,.F.);
#11789=ORIENTED_EDGE('',*,*,#8868,.T.);
#11790=ORIENTED_EDGE('',*,*,#8869,.T.);
#11791=ORIENTED_EDGE('',*,*,#8870,.T.);
#11792=ORIENTED_EDGE('',*,*,#8866,.F.);
#11793=ORIENTED_EDGE('',*,*,#8871,.T.);
#11794=ORIENTED_EDGE('',*,*,#8872,.F.);
#11795=ORIENTED_EDGE('',*,*,#8873,.T.);
#11796=ORIENTED_EDGE('',*,*,#8874,.F.);
#11797=ORIENTED_EDGE('',*,*,#8875,.T.);
#11798=ORIENTED_EDGE('',*,*,#8876,.T.);
#11799=ORIENTED_EDGE('',*,*,#8877,.T.);
#11800=ORIENTED_EDGE('',*,*,#8878,.F.);
#11801=ORIENTED_EDGE('',*,*,#8879,.F.);
#11802=ORIENTED_EDGE('',*,*,#8880,.T.);
#11803=ORIENTED_EDGE('',*,*,#8881,.T.);
#11804=ORIENTED_EDGE('',*,*,#8876,.F.);
#11805=ORIENTED_EDGE('',*,*,#8882,.F.);
#11806=ORIENTED_EDGE('',*,*,#8883,.T.);
#11807=ORIENTED_EDGE('',*,*,#8884,.T.);
#11808=ORIENTED_EDGE('',*,*,#8880,.F.);
#11809=ORIENTED_EDGE('',*,*,#8885,.F.);
#11810=ORIENTED_EDGE('',*,*,#8886,.T.);
#11811=ORIENTED_EDGE('',*,*,#8887,.T.);
#11812=ORIENTED_EDGE('',*,*,#8883,.F.);
#11813=ORIENTED_EDGE('',*,*,#8888,.F.);
#11814=ORIENTED_EDGE('',*,*,#8889,.T.);
#11815=ORIENTED_EDGE('',*,*,#8890,.T.);
#11816=ORIENTED_EDGE('',*,*,#8886,.F.);
#11817=ORIENTED_EDGE('',*,*,#8891,.F.);
#11818=ORIENTED_EDGE('',*,*,#8892,.T.);
#11819=ORIENTED_EDGE('',*,*,#8893,.T.);
#11820=ORIENTED_EDGE('',*,*,#8889,.F.);
#11821=ORIENTED_EDGE('',*,*,#8894,.F.);
#11822=ORIENTED_EDGE('',*,*,#8895,.T.);
#11823=ORIENTED_EDGE('',*,*,#8896,.T.);
#11824=ORIENTED_EDGE('',*,*,#8892,.F.);
#11825=ORIENTED_EDGE('',*,*,#8897,.F.);
#11826=ORIENTED_EDGE('',*,*,#8898,.T.);
#11827=ORIENTED_EDGE('',*,*,#8899,.T.);
#11828=ORIENTED_EDGE('',*,*,#8895,.F.);
#11829=ORIENTED_EDGE('',*,*,#8900,.F.);
#11830=ORIENTED_EDGE('',*,*,#8901,.T.);
#11831=ORIENTED_EDGE('',*,*,#8902,.T.);
#11832=ORIENTED_EDGE('',*,*,#8898,.F.);
#11833=ORIENTED_EDGE('',*,*,#8903,.F.);
#11834=ORIENTED_EDGE('',*,*,#8904,.T.);
#11835=ORIENTED_EDGE('',*,*,#8905,.T.);
#11836=ORIENTED_EDGE('',*,*,#8901,.F.);
#11837=ORIENTED_EDGE('',*,*,#8906,.F.);
#11838=ORIENTED_EDGE('',*,*,#8907,.T.);
#11839=ORIENTED_EDGE('',*,*,#8908,.T.);
#11840=ORIENTED_EDGE('',*,*,#8904,.F.);
#11841=ORIENTED_EDGE('',*,*,#8909,.F.);
#11842=ORIENTED_EDGE('',*,*,#8910,.T.);
#11843=ORIENTED_EDGE('',*,*,#8911,.T.);
#11844=ORIENTED_EDGE('',*,*,#8907,.F.);
#11845=ORIENTED_EDGE('',*,*,#8912,.F.);
#11846=ORIENTED_EDGE('',*,*,#8913,.F.);
#11847=ORIENTED_EDGE('',*,*,#8914,.F.);
#11848=ORIENTED_EDGE('',*,*,#8915,.F.);
#11849=ORIENTED_EDGE('',*,*,#8916,.T.);
#11850=ORIENTED_EDGE('',*,*,#8917,.T.);
#11851=ORIENTED_EDGE('',*,*,#8918,.T.);
#11852=ORIENTED_EDGE('',*,*,#8919,.T.);
#11853=ORIENTED_EDGE('',*,*,#8920,.T.);
#11854=ORIENTED_EDGE('',*,*,#8921,.T.);
#11855=ORIENTED_EDGE('',*,*,#8922,.T.);
#11856=ORIENTED_EDGE('',*,*,#8921,.F.);
#11857=ORIENTED_EDGE('',*,*,#8923,.T.);
#11858=ORIENTED_EDGE('',*,*,#8924,.T.);
#11859=ORIENTED_EDGE('',*,*,#8925,.T.);
#11860=ORIENTED_EDGE('',*,*,#8917,.F.);
#11861=ORIENTED_EDGE('',*,*,#8926,.T.);
#11862=ORIENTED_EDGE('',*,*,#8927,.T.);
#11863=ORIENTED_EDGE('',*,*,#8928,.T.);
#11864=ORIENTED_EDGE('',*,*,#8924,.F.);
#11865=ORIENTED_EDGE('',*,*,#8929,.T.);
#11866=ORIENTED_EDGE('',*,*,#8930,.T.);
#11867=ORIENTED_EDGE('',*,*,#8931,.T.);
#11868=ORIENTED_EDGE('',*,*,#8927,.F.);
#11869=ORIENTED_EDGE('',*,*,#8932,.T.);
#11870=ORIENTED_EDGE('',*,*,#8933,.T.);
#11871=ORIENTED_EDGE('',*,*,#8934,.T.);
#11872=ORIENTED_EDGE('',*,*,#8930,.F.);
#11873=ORIENTED_EDGE('',*,*,#8935,.T.);
#11874=ORIENTED_EDGE('',*,*,#8936,.T.);
#11875=ORIENTED_EDGE('',*,*,#8937,.T.);
#11876=ORIENTED_EDGE('',*,*,#8933,.F.);
#11877=ORIENTED_EDGE('',*,*,#8938,.T.);
#11878=ORIENTED_EDGE('',*,*,#8939,.T.);
#11879=ORIENTED_EDGE('',*,*,#8940,.T.);
#11880=ORIENTED_EDGE('',*,*,#8936,.F.);
#11881=ORIENTED_EDGE('',*,*,#8941,.T.);
#11882=ORIENTED_EDGE('',*,*,#8942,.T.);
#11883=ORIENTED_EDGE('',*,*,#8943,.T.);
#11884=ORIENTED_EDGE('',*,*,#8939,.F.);
#11885=ORIENTED_EDGE('',*,*,#8944,.T.);
#11886=ORIENTED_EDGE('',*,*,#8945,.T.);
#11887=ORIENTED_EDGE('',*,*,#8946,.T.);
#11888=ORIENTED_EDGE('',*,*,#8942,.F.);
#11889=ORIENTED_EDGE('',*,*,#8947,.T.);
#11890=ORIENTED_EDGE('',*,*,#8948,.T.);
#11891=ORIENTED_EDGE('',*,*,#8949,.T.);
#11892=ORIENTED_EDGE('',*,*,#8945,.F.);
#11893=ORIENTED_EDGE('',*,*,#8950,.T.);
#11894=ORIENTED_EDGE('',*,*,#8951,.T.);
#11895=ORIENTED_EDGE('',*,*,#8952,.T.);
#11896=ORIENTED_EDGE('',*,*,#8948,.F.);
#11897=ORIENTED_EDGE('',*,*,#8953,.T.);
#11898=ORIENTED_EDGE('',*,*,#8954,.F.);
#11899=ORIENTED_EDGE('',*,*,#8955,.T.);
#11900=ORIENTED_EDGE('',*,*,#8956,.F.);
#11901=ORIENTED_EDGE('',*,*,#8957,.T.);
#11902=ORIENTED_EDGE('',*,*,#8958,.T.);
#11903=ORIENTED_EDGE('',*,*,#8959,.T.);
#11904=ORIENTED_EDGE('',*,*,#8960,.F.);
#11905=ORIENTED_EDGE('',*,*,#8961,.F.);
#11906=ORIENTED_EDGE('',*,*,#8962,.T.);
#11907=ORIENTED_EDGE('',*,*,#8963,.T.);
#11908=ORIENTED_EDGE('',*,*,#8958,.F.);
#11909=ORIENTED_EDGE('',*,*,#8964,.F.);
#11910=ORIENTED_EDGE('',*,*,#8965,.T.);
#11911=ORIENTED_EDGE('',*,*,#8966,.T.);
#11912=ORIENTED_EDGE('',*,*,#8962,.F.);
#11913=ORIENTED_EDGE('',*,*,#8967,.F.);
#11914=ORIENTED_EDGE('',*,*,#8968,.T.);
#11915=ORIENTED_EDGE('',*,*,#8969,.T.);
#11916=ORIENTED_EDGE('',*,*,#8965,.F.);
#11917=ORIENTED_EDGE('',*,*,#8970,.F.);
#11918=ORIENTED_EDGE('',*,*,#8971,.T.);
#11919=ORIENTED_EDGE('',*,*,#8972,.T.);
#11920=ORIENTED_EDGE('',*,*,#8968,.F.);
#11921=ORIENTED_EDGE('',*,*,#8973,.F.);
#11922=ORIENTED_EDGE('',*,*,#8974,.T.);
#11923=ORIENTED_EDGE('',*,*,#8975,.T.);
#11924=ORIENTED_EDGE('',*,*,#8971,.F.);
#11925=ORIENTED_EDGE('',*,*,#8976,.F.);
#11926=ORIENTED_EDGE('',*,*,#8977,.T.);
#11927=ORIENTED_EDGE('',*,*,#8978,.T.);
#11928=ORIENTED_EDGE('',*,*,#8974,.F.);
#11929=ORIENTED_EDGE('',*,*,#8979,.F.);
#11930=ORIENTED_EDGE('',*,*,#8980,.T.);
#11931=ORIENTED_EDGE('',*,*,#8981,.T.);
#11932=ORIENTED_EDGE('',*,*,#8977,.F.);
#11933=ORIENTED_EDGE('',*,*,#8982,.F.);
#11934=ORIENTED_EDGE('',*,*,#8983,.T.);
#11935=ORIENTED_EDGE('',*,*,#8984,.T.);
#11936=ORIENTED_EDGE('',*,*,#8980,.F.);
#11937=ORIENTED_EDGE('',*,*,#8985,.F.);
#11938=ORIENTED_EDGE('',*,*,#8986,.T.);
#11939=ORIENTED_EDGE('',*,*,#8987,.T.);
#11940=ORIENTED_EDGE('',*,*,#8983,.F.);
#11941=ORIENTED_EDGE('',*,*,#8988,.F.);
#11942=ORIENTED_EDGE('',*,*,#8989,.T.);
#11943=ORIENTED_EDGE('',*,*,#8990,.T.);
#11944=ORIENTED_EDGE('',*,*,#8986,.F.);
#11945=ORIENTED_EDGE('',*,*,#8991,.F.);
#11946=ORIENTED_EDGE('',*,*,#8992,.T.);
#11947=ORIENTED_EDGE('',*,*,#8993,.T.);
#11948=ORIENTED_EDGE('',*,*,#8989,.F.);
#11949=ORIENTED_EDGE('',*,*,#8994,.F.);
#11950=ORIENTED_EDGE('',*,*,#8995,.F.);
#11951=ORIENTED_EDGE('',*,*,#8996,.F.);
#11952=ORIENTED_EDGE('',*,*,#8997,.F.);
#11953=ORIENTED_EDGE('',*,*,#8998,.T.);
#11954=ORIENTED_EDGE('',*,*,#8999,.T.);
#11955=ORIENTED_EDGE('',*,*,#9000,.T.);
#11956=ORIENTED_EDGE('',*,*,#9001,.T.);
#11957=ORIENTED_EDGE('',*,*,#9002,.T.);
#11958=ORIENTED_EDGE('',*,*,#9003,.T.);
#11959=ORIENTED_EDGE('',*,*,#9004,.T.);
#11960=ORIENTED_EDGE('',*,*,#9003,.F.);
#11961=ORIENTED_EDGE('',*,*,#9005,.T.);
#11962=ORIENTED_EDGE('',*,*,#9006,.T.);
#11963=ORIENTED_EDGE('',*,*,#9007,.T.);
#11964=ORIENTED_EDGE('',*,*,#8999,.F.);
#11965=ORIENTED_EDGE('',*,*,#9008,.T.);
#11966=ORIENTED_EDGE('',*,*,#9009,.T.);
#11967=ORIENTED_EDGE('',*,*,#9010,.T.);
#11968=ORIENTED_EDGE('',*,*,#9006,.F.);
#11969=ORIENTED_EDGE('',*,*,#9011,.T.);
#11970=ORIENTED_EDGE('',*,*,#9012,.T.);
#11971=ORIENTED_EDGE('',*,*,#9013,.T.);
#11972=ORIENTED_EDGE('',*,*,#9009,.F.);
#11973=ORIENTED_EDGE('',*,*,#9014,.T.);
#11974=ORIENTED_EDGE('',*,*,#9015,.T.);
#11975=ORIENTED_EDGE('',*,*,#9016,.T.);
#11976=ORIENTED_EDGE('',*,*,#9012,.F.);
#11977=ORIENTED_EDGE('',*,*,#9017,.T.);
#11978=ORIENTED_EDGE('',*,*,#9018,.T.);
#11979=ORIENTED_EDGE('',*,*,#9019,.T.);
#11980=ORIENTED_EDGE('',*,*,#9015,.F.);
#11981=ORIENTED_EDGE('',*,*,#9020,.T.);
#11982=ORIENTED_EDGE('',*,*,#9021,.T.);
#11983=ORIENTED_EDGE('',*,*,#9022,.T.);
#11984=ORIENTED_EDGE('',*,*,#9018,.F.);
#11985=ORIENTED_EDGE('',*,*,#9023,.T.);
#11986=ORIENTED_EDGE('',*,*,#9024,.T.);
#11987=ORIENTED_EDGE('',*,*,#9025,.T.);
#11988=ORIENTED_EDGE('',*,*,#9021,.F.);
#11989=ORIENTED_EDGE('',*,*,#9026,.T.);
#11990=ORIENTED_EDGE('',*,*,#9027,.T.);
#11991=ORIENTED_EDGE('',*,*,#9028,.T.);
#11992=ORIENTED_EDGE('',*,*,#9024,.F.);
#11993=ORIENTED_EDGE('',*,*,#9029,.T.);
#11994=ORIENTED_EDGE('',*,*,#9030,.T.);
#11995=ORIENTED_EDGE('',*,*,#9031,.T.);
#11996=ORIENTED_EDGE('',*,*,#9027,.F.);
#11997=ORIENTED_EDGE('',*,*,#9032,.T.);
#11998=ORIENTED_EDGE('',*,*,#9033,.T.);
#11999=ORIENTED_EDGE('',*,*,#9034,.T.);
#12000=ORIENTED_EDGE('',*,*,#9030,.F.);
#12001=ORIENTED_EDGE('',*,*,#9035,.T.);
#12002=ORIENTED_EDGE('',*,*,#9036,.F.);
#12003=ORIENTED_EDGE('',*,*,#9037,.T.);
#12004=ORIENTED_EDGE('',*,*,#9038,.F.);
#12005=ORIENTED_EDGE('',*,*,#9039,.T.);
#12006=ORIENTED_EDGE('',*,*,#9040,.T.);
#12007=ORIENTED_EDGE('',*,*,#9041,.T.);
#12008=ORIENTED_EDGE('',*,*,#9042,.F.);
#12009=ORIENTED_EDGE('',*,*,#9043,.F.);
#12010=ORIENTED_EDGE('',*,*,#9044,.T.);
#12011=ORIENTED_EDGE('',*,*,#9045,.T.);
#12012=ORIENTED_EDGE('',*,*,#9040,.F.);
#12013=ORIENTED_EDGE('',*,*,#9046,.F.);
#12014=ORIENTED_EDGE('',*,*,#9047,.T.);
#12015=ORIENTED_EDGE('',*,*,#9048,.T.);
#12016=ORIENTED_EDGE('',*,*,#9044,.F.);
#12017=ORIENTED_EDGE('',*,*,#9049,.F.);
#12018=ORIENTED_EDGE('',*,*,#9050,.T.);
#12019=ORIENTED_EDGE('',*,*,#9051,.T.);
#12020=ORIENTED_EDGE('',*,*,#9047,.F.);
#12021=ORIENTED_EDGE('',*,*,#9052,.F.);
#12022=ORIENTED_EDGE('',*,*,#9053,.T.);
#12023=ORIENTED_EDGE('',*,*,#9054,.T.);
#12024=ORIENTED_EDGE('',*,*,#9050,.F.);
#12025=ORIENTED_EDGE('',*,*,#9055,.F.);
#12026=ORIENTED_EDGE('',*,*,#9056,.T.);
#12027=ORIENTED_EDGE('',*,*,#9057,.T.);
#12028=ORIENTED_EDGE('',*,*,#9053,.F.);
#12029=ORIENTED_EDGE('',*,*,#9058,.F.);
#12030=ORIENTED_EDGE('',*,*,#9059,.T.);
#12031=ORIENTED_EDGE('',*,*,#9060,.T.);
#12032=ORIENTED_EDGE('',*,*,#9056,.F.);
#12033=ORIENTED_EDGE('',*,*,#9061,.F.);
#12034=ORIENTED_EDGE('',*,*,#9062,.T.);
#12035=ORIENTED_EDGE('',*,*,#9063,.T.);
#12036=ORIENTED_EDGE('',*,*,#9059,.F.);
#12037=ORIENTED_EDGE('',*,*,#9064,.F.);
#12038=ORIENTED_EDGE('',*,*,#9065,.T.);
#12039=ORIENTED_EDGE('',*,*,#9066,.T.);
#12040=ORIENTED_EDGE('',*,*,#9062,.F.);
#12041=ORIENTED_EDGE('',*,*,#9067,.F.);
#12042=ORIENTED_EDGE('',*,*,#9068,.T.);
#12043=ORIENTED_EDGE('',*,*,#9069,.T.);
#12044=ORIENTED_EDGE('',*,*,#9065,.F.);
#12045=ORIENTED_EDGE('',*,*,#9070,.F.);
#12046=ORIENTED_EDGE('',*,*,#9071,.T.);
#12047=ORIENTED_EDGE('',*,*,#9072,.T.);
#12048=ORIENTED_EDGE('',*,*,#9068,.F.);
#12049=ORIENTED_EDGE('',*,*,#9073,.F.);
#12050=ORIENTED_EDGE('',*,*,#9074,.T.);
#12051=ORIENTED_EDGE('',*,*,#9075,.T.);
#12052=ORIENTED_EDGE('',*,*,#9071,.F.);
#12053=ORIENTED_EDGE('',*,*,#9076,.F.);
#12054=ORIENTED_EDGE('',*,*,#9077,.F.);
#12055=ORIENTED_EDGE('',*,*,#9078,.F.);
#12056=ORIENTED_EDGE('',*,*,#9079,.F.);
#12057=ORIENTED_EDGE('',*,*,#9080,.T.);
#12058=ORIENTED_EDGE('',*,*,#9081,.T.);
#12059=ORIENTED_EDGE('',*,*,#9082,.T.);
#12060=ORIENTED_EDGE('',*,*,#9083,.T.);
#12061=ORIENTED_EDGE('',*,*,#9084,.T.);
#12062=ORIENTED_EDGE('',*,*,#9085,.T.);
#12063=ORIENTED_EDGE('',*,*,#9086,.T.);
#12064=ORIENTED_EDGE('',*,*,#9085,.F.);
#12065=ORIENTED_EDGE('',*,*,#9087,.T.);
#12066=ORIENTED_EDGE('',*,*,#9088,.T.);
#12067=ORIENTED_EDGE('',*,*,#9089,.T.);
#12068=ORIENTED_EDGE('',*,*,#9081,.F.);
#12069=ORIENTED_EDGE('',*,*,#9090,.T.);
#12070=ORIENTED_EDGE('',*,*,#9091,.T.);
#12071=ORIENTED_EDGE('',*,*,#9092,.T.);
#12072=ORIENTED_EDGE('',*,*,#9088,.F.);
#12073=ORIENTED_EDGE('',*,*,#9093,.T.);
#12074=ORIENTED_EDGE('',*,*,#9094,.T.);
#12075=ORIENTED_EDGE('',*,*,#9095,.T.);
#12076=ORIENTED_EDGE('',*,*,#9091,.F.);
#12077=ORIENTED_EDGE('',*,*,#9096,.T.);
#12078=ORIENTED_EDGE('',*,*,#9097,.T.);
#12079=ORIENTED_EDGE('',*,*,#9098,.T.);
#12080=ORIENTED_EDGE('',*,*,#9094,.F.);
#12081=ORIENTED_EDGE('',*,*,#9099,.T.);
#12082=ORIENTED_EDGE('',*,*,#9100,.T.);
#12083=ORIENTED_EDGE('',*,*,#9101,.T.);
#12084=ORIENTED_EDGE('',*,*,#9097,.F.);
#12085=ORIENTED_EDGE('',*,*,#9102,.T.);
#12086=ORIENTED_EDGE('',*,*,#9103,.T.);
#12087=ORIENTED_EDGE('',*,*,#9104,.T.);
#12088=ORIENTED_EDGE('',*,*,#9100,.F.);
#12089=ORIENTED_EDGE('',*,*,#9105,.T.);
#12090=ORIENTED_EDGE('',*,*,#9106,.T.);
#12091=ORIENTED_EDGE('',*,*,#9107,.T.);
#12092=ORIENTED_EDGE('',*,*,#9103,.F.);
#12093=ORIENTED_EDGE('',*,*,#9108,.T.);
#12094=ORIENTED_EDGE('',*,*,#9109,.T.);
#12095=ORIENTED_EDGE('',*,*,#9110,.T.);
#12096=ORIENTED_EDGE('',*,*,#9106,.F.);
#12097=ORIENTED_EDGE('',*,*,#9111,.T.);
#12098=ORIENTED_EDGE('',*,*,#9112,.T.);
#12099=ORIENTED_EDGE('',*,*,#9113,.T.);
#12100=ORIENTED_EDGE('',*,*,#9109,.F.);
#12101=ORIENTED_EDGE('',*,*,#9114,.T.);
#12102=ORIENTED_EDGE('',*,*,#9115,.T.);
#12103=ORIENTED_EDGE('',*,*,#9116,.T.);
#12104=ORIENTED_EDGE('',*,*,#9112,.F.);
#12105=ORIENTED_EDGE('',*,*,#9117,.T.);
#12106=ORIENTED_EDGE('',*,*,#9118,.F.);
#12107=ORIENTED_EDGE('',*,*,#9119,.T.);
#12108=ORIENTED_EDGE('',*,*,#9120,.F.);
#12109=ORIENTED_EDGE('',*,*,#9121,.T.);
#12110=ORIENTED_EDGE('',*,*,#9122,.T.);
#12111=ORIENTED_EDGE('',*,*,#9123,.T.);
#12112=ORIENTED_EDGE('',*,*,#9124,.F.);
#12113=ORIENTED_EDGE('',*,*,#9125,.F.);
#12114=ORIENTED_EDGE('',*,*,#9126,.T.);
#12115=ORIENTED_EDGE('',*,*,#9127,.T.);
#12116=ORIENTED_EDGE('',*,*,#9122,.F.);
#12117=ORIENTED_EDGE('',*,*,#9128,.F.);
#12118=ORIENTED_EDGE('',*,*,#9129,.T.);
#12119=ORIENTED_EDGE('',*,*,#9130,.T.);
#12120=ORIENTED_EDGE('',*,*,#9126,.F.);
#12121=ORIENTED_EDGE('',*,*,#9131,.F.);
#12122=ORIENTED_EDGE('',*,*,#9132,.T.);
#12123=ORIENTED_EDGE('',*,*,#9133,.T.);
#12124=ORIENTED_EDGE('',*,*,#9129,.F.);
#12125=ORIENTED_EDGE('',*,*,#9134,.F.);
#12126=ORIENTED_EDGE('',*,*,#9135,.T.);
#12127=ORIENTED_EDGE('',*,*,#9136,.T.);
#12128=ORIENTED_EDGE('',*,*,#9132,.F.);
#12129=ORIENTED_EDGE('',*,*,#9137,.F.);
#12130=ORIENTED_EDGE('',*,*,#9138,.T.);
#12131=ORIENTED_EDGE('',*,*,#9139,.T.);
#12132=ORIENTED_EDGE('',*,*,#9135,.F.);
#12133=ORIENTED_EDGE('',*,*,#9140,.F.);
#12134=ORIENTED_EDGE('',*,*,#9141,.T.);
#12135=ORIENTED_EDGE('',*,*,#9142,.T.);
#12136=ORIENTED_EDGE('',*,*,#9138,.F.);
#12137=ORIENTED_EDGE('',*,*,#9143,.F.);
#12138=ORIENTED_EDGE('',*,*,#9144,.T.);
#12139=ORIENTED_EDGE('',*,*,#9145,.T.);
#12140=ORIENTED_EDGE('',*,*,#9141,.F.);
#12141=ORIENTED_EDGE('',*,*,#9146,.F.);
#12142=ORIENTED_EDGE('',*,*,#9147,.T.);
#12143=ORIENTED_EDGE('',*,*,#9148,.T.);
#12144=ORIENTED_EDGE('',*,*,#9144,.F.);
#12145=ORIENTED_EDGE('',*,*,#9149,.F.);
#12146=ORIENTED_EDGE('',*,*,#9150,.T.);
#12147=ORIENTED_EDGE('',*,*,#9151,.T.);
#12148=ORIENTED_EDGE('',*,*,#9147,.F.);
#12149=ORIENTED_EDGE('',*,*,#9152,.F.);
#12150=ORIENTED_EDGE('',*,*,#9153,.T.);
#12151=ORIENTED_EDGE('',*,*,#9154,.T.);
#12152=ORIENTED_EDGE('',*,*,#9150,.F.);
#12153=ORIENTED_EDGE('',*,*,#9155,.F.);
#12154=ORIENTED_EDGE('',*,*,#9156,.T.);
#12155=ORIENTED_EDGE('',*,*,#9157,.T.);
#12156=ORIENTED_EDGE('',*,*,#9153,.F.);
#12157=ORIENTED_EDGE('',*,*,#9158,.F.);
#12158=ORIENTED_EDGE('',*,*,#9159,.F.);
#12159=ORIENTED_EDGE('',*,*,#9160,.F.);
#12160=ORIENTED_EDGE('',*,*,#9161,.F.);
#12161=ORIENTED_EDGE('',*,*,#9162,.T.);
#12162=ORIENTED_EDGE('',*,*,#9163,.T.);
#12163=ORIENTED_EDGE('',*,*,#9164,.T.);
#12164=ORIENTED_EDGE('',*,*,#9165,.T.);
#12165=ORIENTED_EDGE('',*,*,#9166,.T.);
#12166=ORIENTED_EDGE('',*,*,#9167,.T.);
#12167=ORIENTED_EDGE('',*,*,#9168,.T.);
#12168=ORIENTED_EDGE('',*,*,#9167,.F.);
#12169=ORIENTED_EDGE('',*,*,#9169,.T.);
#12170=ORIENTED_EDGE('',*,*,#9170,.T.);
#12171=ORIENTED_EDGE('',*,*,#9171,.T.);
#12172=ORIENTED_EDGE('',*,*,#9163,.F.);
#12173=ORIENTED_EDGE('',*,*,#9172,.T.);
#12174=ORIENTED_EDGE('',*,*,#9173,.T.);
#12175=ORIENTED_EDGE('',*,*,#9174,.T.);
#12176=ORIENTED_EDGE('',*,*,#9170,.F.);
#12177=ORIENTED_EDGE('',*,*,#9175,.T.);
#12178=ORIENTED_EDGE('',*,*,#9176,.T.);
#12179=ORIENTED_EDGE('',*,*,#9177,.T.);
#12180=ORIENTED_EDGE('',*,*,#9173,.F.);
#12181=ORIENTED_EDGE('',*,*,#9178,.T.);
#12182=ORIENTED_EDGE('',*,*,#9179,.T.);
#12183=ORIENTED_EDGE('',*,*,#9180,.T.);
#12184=ORIENTED_EDGE('',*,*,#9176,.F.);
#12185=ORIENTED_EDGE('',*,*,#9181,.T.);
#12186=ORIENTED_EDGE('',*,*,#9182,.T.);
#12187=ORIENTED_EDGE('',*,*,#9183,.T.);
#12188=ORIENTED_EDGE('',*,*,#9179,.F.);
#12189=ORIENTED_EDGE('',*,*,#9184,.T.);
#12190=ORIENTED_EDGE('',*,*,#9185,.T.);
#12191=ORIENTED_EDGE('',*,*,#9186,.T.);
#12192=ORIENTED_EDGE('',*,*,#9182,.F.);
#12193=ORIENTED_EDGE('',*,*,#9187,.T.);
#12194=ORIENTED_EDGE('',*,*,#9188,.T.);
#12195=ORIENTED_EDGE('',*,*,#9189,.T.);
#12196=ORIENTED_EDGE('',*,*,#9185,.F.);
#12197=ORIENTED_EDGE('',*,*,#9190,.T.);
#12198=ORIENTED_EDGE('',*,*,#9191,.T.);
#12199=ORIENTED_EDGE('',*,*,#9192,.T.);
#12200=ORIENTED_EDGE('',*,*,#9188,.F.);
#12201=ORIENTED_EDGE('',*,*,#9193,.T.);
#12202=ORIENTED_EDGE('',*,*,#9194,.T.);
#12203=ORIENTED_EDGE('',*,*,#9195,.T.);
#12204=ORIENTED_EDGE('',*,*,#9191,.F.);
#12205=ORIENTED_EDGE('',*,*,#9196,.T.);
#12206=ORIENTED_EDGE('',*,*,#9197,.T.);
#12207=ORIENTED_EDGE('',*,*,#9198,.T.);
#12208=ORIENTED_EDGE('',*,*,#9194,.F.);
#12209=ORIENTED_EDGE('',*,*,#9199,.T.);
#12210=ORIENTED_EDGE('',*,*,#9200,.F.);
#12211=ORIENTED_EDGE('',*,*,#9201,.T.);
#12212=ORIENTED_EDGE('',*,*,#9202,.F.);
#12213=ORIENTED_EDGE('',*,*,#9203,.T.);
#12214=ORIENTED_EDGE('',*,*,#9204,.T.);
#12215=ORIENTED_EDGE('',*,*,#9205,.T.);
#12216=ORIENTED_EDGE('',*,*,#9206,.F.);
#12217=ORIENTED_EDGE('',*,*,#9207,.F.);
#12218=ORIENTED_EDGE('',*,*,#9208,.T.);
#12219=ORIENTED_EDGE('',*,*,#9209,.T.);
#12220=ORIENTED_EDGE('',*,*,#9204,.F.);
#12221=ORIENTED_EDGE('',*,*,#9210,.F.);
#12222=ORIENTED_EDGE('',*,*,#9211,.T.);
#12223=ORIENTED_EDGE('',*,*,#9212,.T.);
#12224=ORIENTED_EDGE('',*,*,#9208,.F.);
#12225=ORIENTED_EDGE('',*,*,#9213,.F.);
#12226=ORIENTED_EDGE('',*,*,#9214,.T.);
#12227=ORIENTED_EDGE('',*,*,#9215,.T.);
#12228=ORIENTED_EDGE('',*,*,#9211,.F.);
#12229=ORIENTED_EDGE('',*,*,#9216,.F.);
#12230=ORIENTED_EDGE('',*,*,#9217,.T.);
#12231=ORIENTED_EDGE('',*,*,#9218,.T.);
#12232=ORIENTED_EDGE('',*,*,#9214,.F.);
#12233=ORIENTED_EDGE('',*,*,#9219,.F.);
#12234=ORIENTED_EDGE('',*,*,#9220,.T.);
#12235=ORIENTED_EDGE('',*,*,#9221,.T.);
#12236=ORIENTED_EDGE('',*,*,#9217,.F.);
#12237=ORIENTED_EDGE('',*,*,#9222,.F.);
#12238=ORIENTED_EDGE('',*,*,#9223,.T.);
#12239=ORIENTED_EDGE('',*,*,#9224,.T.);
#12240=ORIENTED_EDGE('',*,*,#9220,.F.);
#12241=ORIENTED_EDGE('',*,*,#9225,.F.);
#12242=ORIENTED_EDGE('',*,*,#9226,.T.);
#12243=ORIENTED_EDGE('',*,*,#9227,.T.);
#12244=ORIENTED_EDGE('',*,*,#9223,.F.);
#12245=ORIENTED_EDGE('',*,*,#9228,.F.);
#12246=ORIENTED_EDGE('',*,*,#9229,.T.);
#12247=ORIENTED_EDGE('',*,*,#9230,.T.);
#12248=ORIENTED_EDGE('',*,*,#9226,.F.);
#12249=ORIENTED_EDGE('',*,*,#9231,.F.);
#12250=ORIENTED_EDGE('',*,*,#9232,.T.);
#12251=ORIENTED_EDGE('',*,*,#9233,.T.);
#12252=ORIENTED_EDGE('',*,*,#9229,.F.);
#12253=ORIENTED_EDGE('',*,*,#9234,.F.);
#12254=ORIENTED_EDGE('',*,*,#9235,.T.);
#12255=ORIENTED_EDGE('',*,*,#9236,.T.);
#12256=ORIENTED_EDGE('',*,*,#9232,.F.);
#12257=ORIENTED_EDGE('',*,*,#9237,.F.);
#12258=ORIENTED_EDGE('',*,*,#9238,.T.);
#12259=ORIENTED_EDGE('',*,*,#9239,.T.);
#12260=ORIENTED_EDGE('',*,*,#9235,.F.);
#12261=ORIENTED_EDGE('',*,*,#9240,.F.);
#12262=ORIENTED_EDGE('',*,*,#9241,.F.);
#12263=ORIENTED_EDGE('',*,*,#9242,.F.);
#12264=ORIENTED_EDGE('',*,*,#9243,.F.);
#12265=ORIENTED_EDGE('',*,*,#9244,.T.);
#12266=ORIENTED_EDGE('',*,*,#9245,.T.);
#12267=ORIENTED_EDGE('',*,*,#9246,.T.);
#12268=ORIENTED_EDGE('',*,*,#9247,.T.);
#12269=ORIENTED_EDGE('',*,*,#9248,.T.);
#12270=ORIENTED_EDGE('',*,*,#9249,.T.);
#12271=ORIENTED_EDGE('',*,*,#9250,.T.);
#12272=ORIENTED_EDGE('',*,*,#9245,.F.);
#12273=ORIENTED_EDGE('',*,*,#9251,.T.);
#12274=ORIENTED_EDGE('',*,*,#9252,.T.);
#12275=ORIENTED_EDGE('',*,*,#9253,.T.);
#12276=ORIENTED_EDGE('',*,*,#9249,.F.);
#12277=ORIENTED_EDGE('',*,*,#9254,.T.);
#12278=ORIENTED_EDGE('',*,*,#9255,.T.);
#12279=ORIENTED_EDGE('',*,*,#9256,.T.);
#12280=ORIENTED_EDGE('',*,*,#9252,.F.);
#12281=ORIENTED_EDGE('',*,*,#9257,.T.);
#12282=ORIENTED_EDGE('',*,*,#9258,.T.);
#12283=ORIENTED_EDGE('',*,*,#9259,.T.);
#12284=ORIENTED_EDGE('',*,*,#9255,.F.);
#12285=ORIENTED_EDGE('',*,*,#9260,.T.);
#12286=ORIENTED_EDGE('',*,*,#9261,.T.);
#12287=ORIENTED_EDGE('',*,*,#9262,.T.);
#12288=ORIENTED_EDGE('',*,*,#9258,.F.);
#12289=ORIENTED_EDGE('',*,*,#9263,.T.);
#12290=ORIENTED_EDGE('',*,*,#9264,.T.);
#12291=ORIENTED_EDGE('',*,*,#9265,.T.);
#12292=ORIENTED_EDGE('',*,*,#9261,.F.);
#12293=ORIENTED_EDGE('',*,*,#9266,.T.);
#12294=ORIENTED_EDGE('',*,*,#9267,.F.);
#12295=ORIENTED_EDGE('',*,*,#9268,.T.);
#12296=ORIENTED_EDGE('',*,*,#9269,.F.);
#12297=ORIENTED_EDGE('',*,*,#9270,.T.);
#12298=ORIENTED_EDGE('',*,*,#9271,.T.);
#12299=ORIENTED_EDGE('',*,*,#9272,.T.);
#12300=ORIENTED_EDGE('',*,*,#9273,.F.);
#12301=ORIENTED_EDGE('',*,*,#9274,.F.);
#12302=ORIENTED_EDGE('',*,*,#9275,.T.);
#12303=ORIENTED_EDGE('',*,*,#9276,.T.);
#12304=ORIENTED_EDGE('',*,*,#9271,.F.);
#12305=ORIENTED_EDGE('',*,*,#9277,.F.);
#12306=ORIENTED_EDGE('',*,*,#9278,.T.);
#12307=ORIENTED_EDGE('',*,*,#9279,.T.);
#12308=ORIENTED_EDGE('',*,*,#9275,.F.);
#12309=ORIENTED_EDGE('',*,*,#9280,.F.);
#12310=ORIENTED_EDGE('',*,*,#9281,.T.);
#12311=ORIENTED_EDGE('',*,*,#9282,.T.);
#12312=ORIENTED_EDGE('',*,*,#9278,.F.);
#12313=ORIENTED_EDGE('',*,*,#9283,.F.);
#12314=ORIENTED_EDGE('',*,*,#9284,.T.);
#12315=ORIENTED_EDGE('',*,*,#9285,.T.);
#12316=ORIENTED_EDGE('',*,*,#9281,.F.);
#12317=ORIENTED_EDGE('',*,*,#9286,.F.);
#12318=ORIENTED_EDGE('',*,*,#9287,.T.);
#12319=ORIENTED_EDGE('',*,*,#9288,.T.);
#12320=ORIENTED_EDGE('',*,*,#9284,.F.);
#12321=ORIENTED_EDGE('',*,*,#9289,.F.);
#12322=ORIENTED_EDGE('',*,*,#9290,.T.);
#12323=ORIENTED_EDGE('',*,*,#9291,.T.);
#12324=ORIENTED_EDGE('',*,*,#9287,.F.);
#12325=ORIENTED_EDGE('',*,*,#9292,.F.);
#12326=ORIENTED_EDGE('',*,*,#9293,.F.);
#12327=ORIENTED_EDGE('',*,*,#9294,.F.);
#12328=ORIENTED_EDGE('',*,*,#9295,.F.);
#12329=ORIENTED_EDGE('',*,*,#9296,.F.);
#12330=ORIENTED_EDGE('',*,*,#9297,.T.);
#12331=ORIENTED_EDGE('',*,*,#9298,.T.);
#12332=ORIENTED_EDGE('',*,*,#9299,.T.);
#12333=ORIENTED_EDGE('',*,*,#9300,.T.);
#12334=ORIENTED_EDGE('',*,*,#9301,.T.);
#12335=ORIENTED_EDGE('',*,*,#9302,.T.);
#12336=ORIENTED_EDGE('',*,*,#9303,.T.);
#12337=ORIENTED_EDGE('',*,*,#9298,.F.);
#12338=ORIENTED_EDGE('',*,*,#9304,.T.);
#12339=ORIENTED_EDGE('',*,*,#9305,.T.);
#12340=ORIENTED_EDGE('',*,*,#9306,.T.);
#12341=ORIENTED_EDGE('',*,*,#9302,.F.);
#12342=ORIENTED_EDGE('',*,*,#9307,.T.);
#12343=ORIENTED_EDGE('',*,*,#9308,.T.);
#12344=ORIENTED_EDGE('',*,*,#9309,.T.);
#12345=ORIENTED_EDGE('',*,*,#9305,.F.);
#12346=ORIENTED_EDGE('',*,*,#9310,.T.);
#12347=ORIENTED_EDGE('',*,*,#9311,.T.);
#12348=ORIENTED_EDGE('',*,*,#9312,.T.);
#12349=ORIENTED_EDGE('',*,*,#9308,.F.);
#12350=ORIENTED_EDGE('',*,*,#9313,.T.);
#12351=ORIENTED_EDGE('',*,*,#9314,.T.);
#12352=ORIENTED_EDGE('',*,*,#9315,.T.);
#12353=ORIENTED_EDGE('',*,*,#9311,.F.);
#12354=ORIENTED_EDGE('',*,*,#9316,.T.);
#12355=ORIENTED_EDGE('',*,*,#9317,.T.);
#12356=ORIENTED_EDGE('',*,*,#9318,.T.);
#12357=ORIENTED_EDGE('',*,*,#9314,.F.);
#12358=ORIENTED_EDGE('',*,*,#9319,.T.);
#12359=ORIENTED_EDGE('',*,*,#9320,.F.);
#12360=ORIENTED_EDGE('',*,*,#9321,.T.);
#12361=ORIENTED_EDGE('',*,*,#9322,.F.);
#12362=ORIENTED_EDGE('',*,*,#9323,.T.);
#12363=ORIENTED_EDGE('',*,*,#9324,.T.);
#12364=ORIENTED_EDGE('',*,*,#9325,.T.);
#12365=ORIENTED_EDGE('',*,*,#9326,.T.);
#12366=ORIENTED_EDGE('',*,*,#9327,.T.);
#12367=ORIENTED_EDGE('',*,*,#9328,.T.);
#12368=ORIENTED_EDGE('',*,*,#9329,.T.);
#12369=ORIENTED_EDGE('',*,*,#9324,.F.);
#12370=ORIENTED_EDGE('',*,*,#9330,.T.);
#12371=ORIENTED_EDGE('',*,*,#9331,.T.);
#12372=ORIENTED_EDGE('',*,*,#9332,.T.);
#12373=ORIENTED_EDGE('',*,*,#9328,.F.);
#12374=ORIENTED_EDGE('',*,*,#9333,.T.);
#12375=ORIENTED_EDGE('',*,*,#9334,.T.);
#12376=ORIENTED_EDGE('',*,*,#9335,.T.);
#12377=ORIENTED_EDGE('',*,*,#9331,.F.);
#12378=ORIENTED_EDGE('',*,*,#9336,.T.);
#12379=ORIENTED_EDGE('',*,*,#9337,.T.);
#12380=ORIENTED_EDGE('',*,*,#9338,.T.);
#12381=ORIENTED_EDGE('',*,*,#9334,.F.);
#12382=ORIENTED_EDGE('',*,*,#9339,.T.);
#12383=ORIENTED_EDGE('',*,*,#9340,.T.);
#12384=ORIENTED_EDGE('',*,*,#9341,.T.);
#12385=ORIENTED_EDGE('',*,*,#9337,.F.);
#12386=ORIENTED_EDGE('',*,*,#9342,.T.);
#12387=ORIENTED_EDGE('',*,*,#9343,.T.);
#12388=ORIENTED_EDGE('',*,*,#9344,.T.);
#12389=ORIENTED_EDGE('',*,*,#9340,.F.);
#12390=ORIENTED_EDGE('',*,*,#9345,.T.);
#12391=ORIENTED_EDGE('',*,*,#9346,.F.);
#12392=ORIENTED_EDGE('',*,*,#9347,.T.);
#12393=ORIENTED_EDGE('',*,*,#9348,.F.);
#12394=ORIENTED_EDGE('',*,*,#9349,.T.);
#12395=ORIENTED_EDGE('',*,*,#9350,.T.);
#12396=ORIENTED_EDGE('',*,*,#9351,.T.);
#12397=ORIENTED_EDGE('',*,*,#9352,.T.);
#12398=ORIENTED_EDGE('',*,*,#9353,.T.);
#12399=ORIENTED_EDGE('',*,*,#9354,.T.);
#12400=ORIENTED_EDGE('',*,*,#9355,.T.);
#12401=ORIENTED_EDGE('',*,*,#9350,.F.);
#12402=ORIENTED_EDGE('',*,*,#9356,.T.);
#12403=ORIENTED_EDGE('',*,*,#9357,.T.);
#12404=ORIENTED_EDGE('',*,*,#9358,.T.);
#12405=ORIENTED_EDGE('',*,*,#9354,.F.);
#12406=ORIENTED_EDGE('',*,*,#9359,.T.);
#12407=ORIENTED_EDGE('',*,*,#9360,.T.);
#12408=ORIENTED_EDGE('',*,*,#9361,.T.);
#12409=ORIENTED_EDGE('',*,*,#9357,.F.);
#12410=ORIENTED_EDGE('',*,*,#9362,.T.);
#12411=ORIENTED_EDGE('',*,*,#9363,.T.);
#12412=ORIENTED_EDGE('',*,*,#9364,.T.);
#12413=ORIENTED_EDGE('',*,*,#9360,.F.);
#12414=ORIENTED_EDGE('',*,*,#9365,.T.);
#12415=ORIENTED_EDGE('',*,*,#9366,.T.);
#12416=ORIENTED_EDGE('',*,*,#9367,.T.);
#12417=ORIENTED_EDGE('',*,*,#9363,.F.);
#12418=ORIENTED_EDGE('',*,*,#9368,.T.);
#12419=ORIENTED_EDGE('',*,*,#9369,.T.);
#12420=ORIENTED_EDGE('',*,*,#9370,.T.);
#12421=ORIENTED_EDGE('',*,*,#9366,.F.);
#12422=ORIENTED_EDGE('',*,*,#9371,.T.);
#12423=ORIENTED_EDGE('',*,*,#9372,.F.);
#12424=ORIENTED_EDGE('',*,*,#9373,.T.);
#12425=ORIENTED_EDGE('',*,*,#9374,.F.);
#12426=ORIENTED_EDGE('',*,*,#9375,.T.);
#12427=ORIENTED_EDGE('',*,*,#9376,.T.);
#12428=ORIENTED_EDGE('',*,*,#9377,.T.);
#12429=ORIENTED_EDGE('',*,*,#9378,.F.);
#12430=ORIENTED_EDGE('',*,*,#9379,.F.);
#12431=ORIENTED_EDGE('',*,*,#9380,.T.);
#12432=ORIENTED_EDGE('',*,*,#9381,.T.);
#12433=ORIENTED_EDGE('',*,*,#9376,.F.);
#12434=ORIENTED_EDGE('',*,*,#9382,.F.);
#12435=ORIENTED_EDGE('',*,*,#9383,.T.);
#12436=ORIENTED_EDGE('',*,*,#9384,.T.);
#12437=ORIENTED_EDGE('',*,*,#9380,.F.);
#12438=ORIENTED_EDGE('',*,*,#9385,.F.);
#12439=ORIENTED_EDGE('',*,*,#9386,.T.);
#12440=ORIENTED_EDGE('',*,*,#9387,.T.);
#12441=ORIENTED_EDGE('',*,*,#9383,.F.);
#12442=ORIENTED_EDGE('',*,*,#9388,.F.);
#12443=ORIENTED_EDGE('',*,*,#9389,.T.);
#12444=ORIENTED_EDGE('',*,*,#9390,.T.);
#12445=ORIENTED_EDGE('',*,*,#9386,.F.);
#12446=ORIENTED_EDGE('',*,*,#9391,.F.);
#12447=ORIENTED_EDGE('',*,*,#9392,.T.);
#12448=ORIENTED_EDGE('',*,*,#9393,.T.);
#12449=ORIENTED_EDGE('',*,*,#9389,.F.);
#12450=ORIENTED_EDGE('',*,*,#9394,.F.);
#12451=ORIENTED_EDGE('',*,*,#9395,.T.);
#12452=ORIENTED_EDGE('',*,*,#9396,.T.);
#12453=ORIENTED_EDGE('',*,*,#9392,.F.);
#12454=ORIENTED_EDGE('',*,*,#9397,.F.);
#12455=ORIENTED_EDGE('',*,*,#9398,.F.);
#12456=ORIENTED_EDGE('',*,*,#9399,.F.);
#12457=ORIENTED_EDGE('',*,*,#9400,.F.);
#12458=ORIENTED_EDGE('',*,*,#9401,.F.);
#12459=ORIENTED_EDGE('',*,*,#9402,.T.);
#12460=ORIENTED_EDGE('',*,*,#9403,.T.);
#12461=ORIENTED_EDGE('',*,*,#9404,.T.);
#12462=ORIENTED_EDGE('',*,*,#9405,.F.);
#12463=ORIENTED_EDGE('',*,*,#9406,.F.);
#12464=ORIENTED_EDGE('',*,*,#9407,.T.);
#12465=ORIENTED_EDGE('',*,*,#9408,.T.);
#12466=ORIENTED_EDGE('',*,*,#9403,.F.);
#12467=ORIENTED_EDGE('',*,*,#9409,.F.);
#12468=ORIENTED_EDGE('',*,*,#9410,.T.);
#12469=ORIENTED_EDGE('',*,*,#9411,.T.);
#12470=ORIENTED_EDGE('',*,*,#9407,.F.);
#12471=ORIENTED_EDGE('',*,*,#9412,.F.);
#12472=ORIENTED_EDGE('',*,*,#9413,.T.);
#12473=ORIENTED_EDGE('',*,*,#9414,.T.);
#12474=ORIENTED_EDGE('',*,*,#9410,.F.);
#12475=ORIENTED_EDGE('',*,*,#9415,.F.);
#12476=ORIENTED_EDGE('',*,*,#9416,.T.);
#12477=ORIENTED_EDGE('',*,*,#9417,.T.);
#12478=ORIENTED_EDGE('',*,*,#9413,.F.);
#12479=ORIENTED_EDGE('',*,*,#9418,.F.);
#12480=ORIENTED_EDGE('',*,*,#9419,.T.);
#12481=ORIENTED_EDGE('',*,*,#9420,.T.);
#12482=ORIENTED_EDGE('',*,*,#9416,.F.);
#12483=ORIENTED_EDGE('',*,*,#9421,.F.);
#12484=ORIENTED_EDGE('',*,*,#9422,.T.);
#12485=ORIENTED_EDGE('',*,*,#9423,.T.);
#12486=ORIENTED_EDGE('',*,*,#9419,.F.);
#12487=ORIENTED_EDGE('',*,*,#9424,.F.);
#12488=ORIENTED_EDGE('',*,*,#9425,.F.);
#12489=ORIENTED_EDGE('',*,*,#9426,.F.);
#12490=ORIENTED_EDGE('',*,*,#9427,.F.);
#12491=ORIENTED_EDGE('',*,*,#9428,.F.);
#12492=ORIENTED_EDGE('',*,*,#9429,.T.);
#12493=ORIENTED_EDGE('',*,*,#9430,.T.);
#12494=ORIENTED_EDGE('',*,*,#9431,.T.);
#12495=ORIENTED_EDGE('',*,*,#9432,.F.);
#12496=ORIENTED_EDGE('',*,*,#9433,.F.);
#12497=ORIENTED_EDGE('',*,*,#9434,.T.);
#12498=ORIENTED_EDGE('',*,*,#9435,.T.);
#12499=ORIENTED_EDGE('',*,*,#9430,.F.);
#12500=ORIENTED_EDGE('',*,*,#9436,.F.);
#12501=ORIENTED_EDGE('',*,*,#9437,.T.);
#12502=ORIENTED_EDGE('',*,*,#9438,.T.);
#12503=ORIENTED_EDGE('',*,*,#9434,.F.);
#12504=ORIENTED_EDGE('',*,*,#9439,.F.);
#12505=ORIENTED_EDGE('',*,*,#9440,.T.);
#12506=ORIENTED_EDGE('',*,*,#9441,.T.);
#12507=ORIENTED_EDGE('',*,*,#9437,.F.);
#12508=ORIENTED_EDGE('',*,*,#9442,.F.);
#12509=ORIENTED_EDGE('',*,*,#9443,.T.);
#12510=ORIENTED_EDGE('',*,*,#9444,.T.);
#12511=ORIENTED_EDGE('',*,*,#9440,.F.);
#12512=ORIENTED_EDGE('',*,*,#9445,.F.);
#12513=ORIENTED_EDGE('',*,*,#9446,.T.);
#12514=ORIENTED_EDGE('',*,*,#9447,.T.);
#12515=ORIENTED_EDGE('',*,*,#9443,.F.);
#12516=ORIENTED_EDGE('',*,*,#9448,.F.);
#12517=ORIENTED_EDGE('',*,*,#9449,.T.);
#12518=ORIENTED_EDGE('',*,*,#9450,.T.);
#12519=ORIENTED_EDGE('',*,*,#9446,.F.);
#12520=ORIENTED_EDGE('',*,*,#9451,.F.);
#12521=ORIENTED_EDGE('',*,*,#9452,.F.);
#12522=ORIENTED_EDGE('',*,*,#9453,.F.);
#12523=ORIENTED_EDGE('',*,*,#9454,.F.);
#12524=ORIENTED_EDGE('',*,*,#9455,.F.);
#12525=ORIENTED_EDGE('',*,*,#9456,.T.);
#12526=ORIENTED_EDGE('',*,*,#9457,.F.);
#12527=ORIENTED_EDGE('',*,*,#9373,.F.);
#12528=ORIENTED_EDGE('',*,*,#9458,.F.);
#12529=ORIENTED_EDGE('',*,*,#9371,.F.);
#12530=ORIENTED_EDGE('',*,*,#9368,.F.);
#12531=ORIENTED_EDGE('',*,*,#9365,.F.);
#12532=ORIENTED_EDGE('',*,*,#9362,.F.);
#12533=ORIENTED_EDGE('',*,*,#9359,.F.);
#12534=ORIENTED_EDGE('',*,*,#9356,.F.);
#12535=ORIENTED_EDGE('',*,*,#9353,.F.);
#12536=ORIENTED_EDGE('',*,*,#9459,.F.);
#12537=ORIENTED_EDGE('',*,*,#9431,.F.);
#12538=ORIENTED_EDGE('',*,*,#9435,.F.);
#12539=ORIENTED_EDGE('',*,*,#9438,.F.);
#12540=ORIENTED_EDGE('',*,*,#9441,.F.);
#12541=ORIENTED_EDGE('',*,*,#9444,.F.);
#12542=ORIENTED_EDGE('',*,*,#9447,.F.);
#12543=ORIENTED_EDGE('',*,*,#9450,.F.);
#12544=ORIENTED_EDGE('',*,*,#9460,.F.);
#12545=ORIENTED_EDGE('',*,*,#9456,.F.);
#12546=ORIENTED_EDGE('',*,*,#9452,.T.);
#12547=ORIENTED_EDGE('',*,*,#9460,.T.);
#12548=ORIENTED_EDGE('',*,*,#9449,.F.);
#12549=ORIENTED_EDGE('',*,*,#9461,.F.);
#12550=ORIENTED_EDGE('',*,*,#9462,.F.);
#12551=ORIENTED_EDGE('',*,*,#9453,.T.);
#12552=ORIENTED_EDGE('',*,*,#9461,.T.);
#12553=ORIENTED_EDGE('',*,*,#9451,.T.);
#12554=ORIENTED_EDGE('',*,*,#9448,.T.);
#12555=ORIENTED_EDGE('',*,*,#9445,.T.);
#12556=ORIENTED_EDGE('',*,*,#9442,.T.);
#12557=ORIENTED_EDGE('',*,*,#9439,.T.);
#12558=ORIENTED_EDGE('',*,*,#9436,.T.);
#12559=ORIENTED_EDGE('',*,*,#9433,.T.);
#12560=ORIENTED_EDGE('',*,*,#9463,.F.);
#12561=ORIENTED_EDGE('',*,*,#9351,.F.);
#12562=ORIENTED_EDGE('',*,*,#9355,.F.);
#12563=ORIENTED_EDGE('',*,*,#9358,.F.);
#12564=ORIENTED_EDGE('',*,*,#9361,.F.);
#12565=ORIENTED_EDGE('',*,*,#9364,.F.);
#12566=ORIENTED_EDGE('',*,*,#9367,.F.);
#12567=ORIENTED_EDGE('',*,*,#9370,.F.);
#12568=ORIENTED_EDGE('',*,*,#9464,.F.);
#12569=ORIENTED_EDGE('',*,*,#9375,.F.);
#12570=ORIENTED_EDGE('',*,*,#9465,.F.);
#12571=ORIENTED_EDGE('',*,*,#9347,.F.);
#12572=ORIENTED_EDGE('',*,*,#9466,.F.);
#12573=ORIENTED_EDGE('',*,*,#9345,.F.);
#12574=ORIENTED_EDGE('',*,*,#9342,.F.);
#12575=ORIENTED_EDGE('',*,*,#9339,.F.);
#12576=ORIENTED_EDGE('',*,*,#9336,.F.);
#12577=ORIENTED_EDGE('',*,*,#9333,.F.);
#12578=ORIENTED_EDGE('',*,*,#9330,.F.);
#12579=ORIENTED_EDGE('',*,*,#9327,.F.);
#12580=ORIENTED_EDGE('',*,*,#9467,.F.);
#12581=ORIENTED_EDGE('',*,*,#9404,.F.);
#12582=ORIENTED_EDGE('',*,*,#9408,.F.);
#12583=ORIENTED_EDGE('',*,*,#9411,.F.);
#12584=ORIENTED_EDGE('',*,*,#9414,.F.);
#12585=ORIENTED_EDGE('',*,*,#9417,.F.);
#12586=ORIENTED_EDGE('',*,*,#9420,.F.);
#12587=ORIENTED_EDGE('',*,*,#9423,.F.);
#12588=ORIENTED_EDGE('',*,*,#9468,.F.);
#12589=ORIENTED_EDGE('',*,*,#9429,.F.);
#12590=ORIENTED_EDGE('',*,*,#9425,.T.);
#12591=ORIENTED_EDGE('',*,*,#9468,.T.);
#12592=ORIENTED_EDGE('',*,*,#9422,.F.);
#12593=ORIENTED_EDGE('',*,*,#9469,.F.);
#12594=ORIENTED_EDGE('',*,*,#9470,.F.);
#12595=ORIENTED_EDGE('',*,*,#9426,.T.);
#12596=ORIENTED_EDGE('',*,*,#9469,.T.);
#12597=ORIENTED_EDGE('',*,*,#9424,.T.);
#12598=ORIENTED_EDGE('',*,*,#9421,.T.);
#12599=ORIENTED_EDGE('',*,*,#9418,.T.);
#12600=ORIENTED_EDGE('',*,*,#9415,.T.);
#12601=ORIENTED_EDGE('',*,*,#9412,.T.);
#12602=ORIENTED_EDGE('',*,*,#9409,.T.);
#12603=ORIENTED_EDGE('',*,*,#9406,.T.);
#12604=ORIENTED_EDGE('',*,*,#9471,.F.);
#12605=ORIENTED_EDGE('',*,*,#9325,.F.);
#12606=ORIENTED_EDGE('',*,*,#9329,.F.);
#12607=ORIENTED_EDGE('',*,*,#9332,.F.);
#12608=ORIENTED_EDGE('',*,*,#9335,.F.);
#12609=ORIENTED_EDGE('',*,*,#9338,.F.);
#12610=ORIENTED_EDGE('',*,*,#9341,.F.);
#12611=ORIENTED_EDGE('',*,*,#9344,.F.);
#12612=ORIENTED_EDGE('',*,*,#9472,.F.);
#12613=ORIENTED_EDGE('',*,*,#9349,.F.);
#12614=ORIENTED_EDGE('',*,*,#9473,.F.);
#12615=ORIENTED_EDGE('',*,*,#9321,.F.);
#12616=ORIENTED_EDGE('',*,*,#9474,.F.);
#12617=ORIENTED_EDGE('',*,*,#9319,.F.);
#12618=ORIENTED_EDGE('',*,*,#9316,.F.);
#12619=ORIENTED_EDGE('',*,*,#9313,.F.);
#12620=ORIENTED_EDGE('',*,*,#9310,.F.);
#12621=ORIENTED_EDGE('',*,*,#9307,.F.);
#12622=ORIENTED_EDGE('',*,*,#9304,.F.);
#12623=ORIENTED_EDGE('',*,*,#9301,.F.);
#12624=ORIENTED_EDGE('',*,*,#9475,.F.);
#12625=ORIENTED_EDGE('',*,*,#9377,.F.);
#12626=ORIENTED_EDGE('',*,*,#9381,.F.);
#12627=ORIENTED_EDGE('',*,*,#9384,.F.);
#12628=ORIENTED_EDGE('',*,*,#9387,.F.);
#12629=ORIENTED_EDGE('',*,*,#9390,.F.);
#12630=ORIENTED_EDGE('',*,*,#9393,.F.);
#12631=ORIENTED_EDGE('',*,*,#9396,.F.);
#12632=ORIENTED_EDGE('',*,*,#9476,.F.);
#12633=ORIENTED_EDGE('',*,*,#9402,.F.);
#12634=ORIENTED_EDGE('',*,*,#9398,.T.);
#12635=ORIENTED_EDGE('',*,*,#9476,.T.);
#12636=ORIENTED_EDGE('',*,*,#9395,.F.);
#12637=ORIENTED_EDGE('',*,*,#9477,.F.);
#12638=ORIENTED_EDGE('',*,*,#9478,.F.);
#12639=ORIENTED_EDGE('',*,*,#9399,.T.);
#12640=ORIENTED_EDGE('',*,*,#9477,.T.);
#12641=ORIENTED_EDGE('',*,*,#9397,.T.);
#12642=ORIENTED_EDGE('',*,*,#9394,.T.);
#12643=ORIENTED_EDGE('',*,*,#9391,.T.);
#12644=ORIENTED_EDGE('',*,*,#9388,.T.);
#12645=ORIENTED_EDGE('',*,*,#9385,.T.);
#12646=ORIENTED_EDGE('',*,*,#9382,.T.);
#12647=ORIENTED_EDGE('',*,*,#9379,.T.);
#12648=ORIENTED_EDGE('',*,*,#9479,.F.);
#12649=ORIENTED_EDGE('',*,*,#9299,.F.);
#12650=ORIENTED_EDGE('',*,*,#9303,.F.);
#12651=ORIENTED_EDGE('',*,*,#9306,.F.);
#12652=ORIENTED_EDGE('',*,*,#9309,.F.);
#12653=ORIENTED_EDGE('',*,*,#9312,.F.);
#12654=ORIENTED_EDGE('',*,*,#9315,.F.);
#12655=ORIENTED_EDGE('',*,*,#9318,.F.);
#12656=ORIENTED_EDGE('',*,*,#9480,.F.);
#12657=ORIENTED_EDGE('',*,*,#9323,.F.);
#12658=ORIENTED_EDGE('',*,*,#9372,.T.);
#12659=ORIENTED_EDGE('',*,*,#9464,.T.);
#12660=ORIENTED_EDGE('',*,*,#9369,.F.);
#12661=ORIENTED_EDGE('',*,*,#9458,.T.);
#12662=ORIENTED_EDGE('',*,*,#9463,.T.);
#12663=ORIENTED_EDGE('',*,*,#9432,.T.);
#12664=ORIENTED_EDGE('',*,*,#9459,.T.);
#12665=ORIENTED_EDGE('',*,*,#9352,.F.);
#12666=ORIENTED_EDGE('',*,*,#9346,.T.);
#12667=ORIENTED_EDGE('',*,*,#9472,.T.);
#12668=ORIENTED_EDGE('',*,*,#9343,.F.);
#12669=ORIENTED_EDGE('',*,*,#9466,.T.);
#12670=ORIENTED_EDGE('',*,*,#9471,.T.);
#12671=ORIENTED_EDGE('',*,*,#9405,.T.);
#12672=ORIENTED_EDGE('',*,*,#9467,.T.);
#12673=ORIENTED_EDGE('',*,*,#9326,.F.);
#12674=ORIENTED_EDGE('',*,*,#9320,.T.);
#12675=ORIENTED_EDGE('',*,*,#9480,.T.);
#12676=ORIENTED_EDGE('',*,*,#9317,.F.);
#12677=ORIENTED_EDGE('',*,*,#9474,.T.);
#12678=ORIENTED_EDGE('',*,*,#9479,.T.);
#12679=ORIENTED_EDGE('',*,*,#9378,.T.);
#12680=ORIENTED_EDGE('',*,*,#9475,.T.);
#12681=ORIENTED_EDGE('',*,*,#9300,.F.);
#12682=ORIENTED_EDGE('',*,*,#9481,.F.);
#12683=ORIENTED_EDGE('',*,*,#9268,.F.);
#12684=ORIENTED_EDGE('',*,*,#9482,.F.);
#12685=ORIENTED_EDGE('',*,*,#9266,.F.);
#12686=ORIENTED_EDGE('',*,*,#9263,.F.);
#12687=ORIENTED_EDGE('',*,*,#9260,.F.);
#12688=ORIENTED_EDGE('',*,*,#9257,.F.);
#12689=ORIENTED_EDGE('',*,*,#9254,.F.);
#12690=ORIENTED_EDGE('',*,*,#9251,.F.);
#12691=ORIENTED_EDGE('',*,*,#9248,.F.);
#12692=ORIENTED_EDGE('',*,*,#9483,.F.);
#12693=ORIENTED_EDGE('',*,*,#9272,.F.);
#12694=ORIENTED_EDGE('',*,*,#9276,.F.);
#12695=ORIENTED_EDGE('',*,*,#9279,.F.);
#12696=ORIENTED_EDGE('',*,*,#9282,.F.);
#12697=ORIENTED_EDGE('',*,*,#9285,.F.);
#12698=ORIENTED_EDGE('',*,*,#9288,.F.);
#12699=ORIENTED_EDGE('',*,*,#9291,.F.);
#12700=ORIENTED_EDGE('',*,*,#9484,.F.);
#12701=ORIENTED_EDGE('',*,*,#9297,.F.);
#12702=ORIENTED_EDGE('',*,*,#9293,.T.);
#12703=ORIENTED_EDGE('',*,*,#9484,.T.);
#12704=ORIENTED_EDGE('',*,*,#9290,.F.);
#12705=ORIENTED_EDGE('',*,*,#9485,.F.);
#12706=ORIENTED_EDGE('',*,*,#9486,.F.);
#12707=ORIENTED_EDGE('',*,*,#9294,.T.);
#12708=ORIENTED_EDGE('',*,*,#9485,.T.);
#12709=ORIENTED_EDGE('',*,*,#9292,.T.);
#12710=ORIENTED_EDGE('',*,*,#9289,.T.);
#12711=ORIENTED_EDGE('',*,*,#9286,.T.);
#12712=ORIENTED_EDGE('',*,*,#9283,.T.);
#12713=ORIENTED_EDGE('',*,*,#9280,.T.);
#12714=ORIENTED_EDGE('',*,*,#9277,.T.);
#12715=ORIENTED_EDGE('',*,*,#9274,.T.);
#12716=ORIENTED_EDGE('',*,*,#9487,.F.);
#12717=ORIENTED_EDGE('',*,*,#9246,.F.);
#12718=ORIENTED_EDGE('',*,*,#9250,.F.);
#12719=ORIENTED_EDGE('',*,*,#9253,.F.);
#12720=ORIENTED_EDGE('',*,*,#9256,.F.);
#12721=ORIENTED_EDGE('',*,*,#9259,.F.);
#12722=ORIENTED_EDGE('',*,*,#9262,.F.);
#12723=ORIENTED_EDGE('',*,*,#9265,.F.);
#12724=ORIENTED_EDGE('',*,*,#9488,.F.);
#12725=ORIENTED_EDGE('',*,*,#9270,.F.);
#12726=ORIENTED_EDGE('',*,*,#9267,.T.);
#12727=ORIENTED_EDGE('',*,*,#9488,.T.);
#12728=ORIENTED_EDGE('',*,*,#9264,.F.);
#12729=ORIENTED_EDGE('',*,*,#9482,.T.);
#12730=ORIENTED_EDGE('',*,*,#9487,.T.);
#12731=ORIENTED_EDGE('',*,*,#9273,.T.);
#12732=ORIENTED_EDGE('',*,*,#9483,.T.);
#12733=ORIENTED_EDGE('',*,*,#9247,.F.);
#12734=ORIENTED_EDGE('',*,*,#9165,.F.);
#12735=ORIENTED_EDGE('',*,*,#9489,.T.);
#12736=ORIENTED_EDGE('',*,*,#9206,.T.);
#12737=ORIENTED_EDGE('',*,*,#9490,.T.);
#12738=ORIENTED_EDGE('',*,*,#9241,.T.);
#12739=ORIENTED_EDGE('',*,*,#9491,.T.);
#12740=ORIENTED_EDGE('',*,*,#9238,.F.);
#12741=ORIENTED_EDGE('',*,*,#9492,.F.);
#12742=ORIENTED_EDGE('',*,*,#9490,.F.);
#12743=ORIENTED_EDGE('',*,*,#9205,.F.);
#12744=ORIENTED_EDGE('',*,*,#9209,.F.);
#12745=ORIENTED_EDGE('',*,*,#9212,.F.);
#12746=ORIENTED_EDGE('',*,*,#9215,.F.);
#12747=ORIENTED_EDGE('',*,*,#9218,.F.);
#12748=ORIENTED_EDGE('',*,*,#9221,.F.);
#12749=ORIENTED_EDGE('',*,*,#9224,.F.);
#12750=ORIENTED_EDGE('',*,*,#9227,.F.);
#12751=ORIENTED_EDGE('',*,*,#9230,.F.);
#12752=ORIENTED_EDGE('',*,*,#9233,.F.);
#12753=ORIENTED_EDGE('',*,*,#9236,.F.);
#12754=ORIENTED_EDGE('',*,*,#9239,.F.);
#12755=ORIENTED_EDGE('',*,*,#9491,.F.);
#12756=ORIENTED_EDGE('',*,*,#9244,.F.);
#12757=ORIENTED_EDGE('',*,*,#9493,.F.);
#12758=ORIENTED_EDGE('',*,*,#9201,.F.);
#12759=ORIENTED_EDGE('',*,*,#9494,.F.);
#12760=ORIENTED_EDGE('',*,*,#9199,.F.);
#12761=ORIENTED_EDGE('',*,*,#9196,.F.);
#12762=ORIENTED_EDGE('',*,*,#9193,.F.);
#12763=ORIENTED_EDGE('',*,*,#9190,.F.);
#12764=ORIENTED_EDGE('',*,*,#9187,.F.);
#12765=ORIENTED_EDGE('',*,*,#9184,.F.);
#12766=ORIENTED_EDGE('',*,*,#9181,.F.);
#12767=ORIENTED_EDGE('',*,*,#9178,.F.);
#12768=ORIENTED_EDGE('',*,*,#9175,.F.);
#12769=ORIENTED_EDGE('',*,*,#9172,.F.);
#12770=ORIENTED_EDGE('',*,*,#9169,.F.);
#12771=ORIENTED_EDGE('',*,*,#9166,.F.);
#12772=ORIENTED_EDGE('',*,*,#9489,.F.);
#12773=ORIENTED_EDGE('',*,*,#9164,.F.);
#12774=ORIENTED_EDGE('',*,*,#9171,.F.);
#12775=ORIENTED_EDGE('',*,*,#9174,.F.);
#12776=ORIENTED_EDGE('',*,*,#9177,.F.);
#12777=ORIENTED_EDGE('',*,*,#9180,.F.);
#12778=ORIENTED_EDGE('',*,*,#9183,.F.);
#12779=ORIENTED_EDGE('',*,*,#9186,.F.);
#12780=ORIENTED_EDGE('',*,*,#9189,.F.);
#12781=ORIENTED_EDGE('',*,*,#9192,.F.);
#12782=ORIENTED_EDGE('',*,*,#9195,.F.);
#12783=ORIENTED_EDGE('',*,*,#9198,.F.);
#12784=ORIENTED_EDGE('',*,*,#9495,.F.);
#12785=ORIENTED_EDGE('',*,*,#9203,.F.);
#12786=ORIENTED_EDGE('',*,*,#9496,.F.);
#12787=ORIENTED_EDGE('',*,*,#9242,.T.);
#12788=ORIENTED_EDGE('',*,*,#9492,.T.);
#12789=ORIENTED_EDGE('',*,*,#9240,.T.);
#12790=ORIENTED_EDGE('',*,*,#9237,.T.);
#12791=ORIENTED_EDGE('',*,*,#9234,.T.);
#12792=ORIENTED_EDGE('',*,*,#9231,.T.);
#12793=ORIENTED_EDGE('',*,*,#9228,.T.);
#12794=ORIENTED_EDGE('',*,*,#9225,.T.);
#12795=ORIENTED_EDGE('',*,*,#9222,.T.);
#12796=ORIENTED_EDGE('',*,*,#9219,.T.);
#12797=ORIENTED_EDGE('',*,*,#9216,.T.);
#12798=ORIENTED_EDGE('',*,*,#9213,.T.);
#12799=ORIENTED_EDGE('',*,*,#9210,.T.);
#12800=ORIENTED_EDGE('',*,*,#9207,.T.);
#12801=ORIENTED_EDGE('',*,*,#9200,.T.);
#12802=ORIENTED_EDGE('',*,*,#9495,.T.);
#12803=ORIENTED_EDGE('',*,*,#9197,.F.);
#12804=ORIENTED_EDGE('',*,*,#9494,.T.);
#12805=ORIENTED_EDGE('',*,*,#9083,.F.);
#12806=ORIENTED_EDGE('',*,*,#9497,.T.);
#12807=ORIENTED_EDGE('',*,*,#9124,.T.);
#12808=ORIENTED_EDGE('',*,*,#9498,.T.);
#12809=ORIENTED_EDGE('',*,*,#9159,.T.);
#12810=ORIENTED_EDGE('',*,*,#9499,.T.);
#12811=ORIENTED_EDGE('',*,*,#9156,.F.);
#12812=ORIENTED_EDGE('',*,*,#9500,.F.);
#12813=ORIENTED_EDGE('',*,*,#9498,.F.);
#12814=ORIENTED_EDGE('',*,*,#9123,.F.);
#12815=ORIENTED_EDGE('',*,*,#9127,.F.);
#12816=ORIENTED_EDGE('',*,*,#9130,.F.);
#12817=ORIENTED_EDGE('',*,*,#9133,.F.);
#12818=ORIENTED_EDGE('',*,*,#9136,.F.);
#12819=ORIENTED_EDGE('',*,*,#9139,.F.);
#12820=ORIENTED_EDGE('',*,*,#9142,.F.);
#12821=ORIENTED_EDGE('',*,*,#9145,.F.);
#12822=ORIENTED_EDGE('',*,*,#9148,.F.);
#12823=ORIENTED_EDGE('',*,*,#9151,.F.);
#12824=ORIENTED_EDGE('',*,*,#9154,.F.);
#12825=ORIENTED_EDGE('',*,*,#9157,.F.);
#12826=ORIENTED_EDGE('',*,*,#9499,.F.);
#12827=ORIENTED_EDGE('',*,*,#9162,.F.);
#12828=ORIENTED_EDGE('',*,*,#9501,.F.);
#12829=ORIENTED_EDGE('',*,*,#9119,.F.);
#12830=ORIENTED_EDGE('',*,*,#9502,.F.);
#12831=ORIENTED_EDGE('',*,*,#9117,.F.);
#12832=ORIENTED_EDGE('',*,*,#9114,.F.);
#12833=ORIENTED_EDGE('',*,*,#9111,.F.);
#12834=ORIENTED_EDGE('',*,*,#9108,.F.);
#12835=ORIENTED_EDGE('',*,*,#9105,.F.);
#12836=ORIENTED_EDGE('',*,*,#9102,.F.);
#12837=ORIENTED_EDGE('',*,*,#9099,.F.);
#12838=ORIENTED_EDGE('',*,*,#9096,.F.);
#12839=ORIENTED_EDGE('',*,*,#9093,.F.);
#12840=ORIENTED_EDGE('',*,*,#9090,.F.);
#12841=ORIENTED_EDGE('',*,*,#9087,.F.);
#12842=ORIENTED_EDGE('',*,*,#9084,.F.);
#12843=ORIENTED_EDGE('',*,*,#9497,.F.);
#12844=ORIENTED_EDGE('',*,*,#9082,.F.);
#12845=ORIENTED_EDGE('',*,*,#9089,.F.);
#12846=ORIENTED_EDGE('',*,*,#9092,.F.);
#12847=ORIENTED_EDGE('',*,*,#9095,.F.);
#12848=ORIENTED_EDGE('',*,*,#9098,.F.);
#12849=ORIENTED_EDGE('',*,*,#9101,.F.);
#12850=ORIENTED_EDGE('',*,*,#9104,.F.);
#12851=ORIENTED_EDGE('',*,*,#9107,.F.);
#12852=ORIENTED_EDGE('',*,*,#9110,.F.);
#12853=ORIENTED_EDGE('',*,*,#9113,.F.);
#12854=ORIENTED_EDGE('',*,*,#9116,.F.);
#12855=ORIENTED_EDGE('',*,*,#9503,.F.);
#12856=ORIENTED_EDGE('',*,*,#9121,.F.);
#12857=ORIENTED_EDGE('',*,*,#9504,.F.);
#12858=ORIENTED_EDGE('',*,*,#9160,.T.);
#12859=ORIENTED_EDGE('',*,*,#9500,.T.);
#12860=ORIENTED_EDGE('',*,*,#9158,.T.);
#12861=ORIENTED_EDGE('',*,*,#9155,.T.);
#12862=ORIENTED_EDGE('',*,*,#9152,.T.);
#12863=ORIENTED_EDGE('',*,*,#9149,.T.);
#12864=ORIENTED_EDGE('',*,*,#9146,.T.);
#12865=ORIENTED_EDGE('',*,*,#9143,.T.);
#12866=ORIENTED_EDGE('',*,*,#9140,.T.);
#12867=ORIENTED_EDGE('',*,*,#9137,.T.);
#12868=ORIENTED_EDGE('',*,*,#9134,.T.);
#12869=ORIENTED_EDGE('',*,*,#9131,.T.);
#12870=ORIENTED_EDGE('',*,*,#9128,.T.);
#12871=ORIENTED_EDGE('',*,*,#9125,.T.);
#12872=ORIENTED_EDGE('',*,*,#9118,.T.);
#12873=ORIENTED_EDGE('',*,*,#9503,.T.);
#12874=ORIENTED_EDGE('',*,*,#9115,.F.);
#12875=ORIENTED_EDGE('',*,*,#9502,.T.);
#12876=ORIENTED_EDGE('',*,*,#9001,.F.);
#12877=ORIENTED_EDGE('',*,*,#9505,.T.);
#12878=ORIENTED_EDGE('',*,*,#9042,.T.);
#12879=ORIENTED_EDGE('',*,*,#9506,.T.);
#12880=ORIENTED_EDGE('',*,*,#9077,.T.);
#12881=ORIENTED_EDGE('',*,*,#9507,.T.);
#12882=ORIENTED_EDGE('',*,*,#9074,.F.);
#12883=ORIENTED_EDGE('',*,*,#9508,.F.);
#12884=ORIENTED_EDGE('',*,*,#9506,.F.);
#12885=ORIENTED_EDGE('',*,*,#9041,.F.);
#12886=ORIENTED_EDGE('',*,*,#9045,.F.);
#12887=ORIENTED_EDGE('',*,*,#9048,.F.);
#12888=ORIENTED_EDGE('',*,*,#9051,.F.);
#12889=ORIENTED_EDGE('',*,*,#9054,.F.);
#12890=ORIENTED_EDGE('',*,*,#9057,.F.);
#12891=ORIENTED_EDGE('',*,*,#9060,.F.);
#12892=ORIENTED_EDGE('',*,*,#9063,.F.);
#12893=ORIENTED_EDGE('',*,*,#9066,.F.);
#12894=ORIENTED_EDGE('',*,*,#9069,.F.);
#12895=ORIENTED_EDGE('',*,*,#9072,.F.);
#12896=ORIENTED_EDGE('',*,*,#9075,.F.);
#12897=ORIENTED_EDGE('',*,*,#9507,.F.);
#12898=ORIENTED_EDGE('',*,*,#9080,.F.);
#12899=ORIENTED_EDGE('',*,*,#9509,.F.);
#12900=ORIENTED_EDGE('',*,*,#9037,.F.);
#12901=ORIENTED_EDGE('',*,*,#9510,.F.);
#12902=ORIENTED_EDGE('',*,*,#9035,.F.);
#12903=ORIENTED_EDGE('',*,*,#9032,.F.);
#12904=ORIENTED_EDGE('',*,*,#9029,.F.);
#12905=ORIENTED_EDGE('',*,*,#9026,.F.);
#12906=ORIENTED_EDGE('',*,*,#9023,.F.);
#12907=ORIENTED_EDGE('',*,*,#9020,.F.);
#12908=ORIENTED_EDGE('',*,*,#9017,.F.);
#12909=ORIENTED_EDGE('',*,*,#9014,.F.);
#12910=ORIENTED_EDGE('',*,*,#9011,.F.);
#12911=ORIENTED_EDGE('',*,*,#9008,.F.);
#12912=ORIENTED_EDGE('',*,*,#9005,.F.);
#12913=ORIENTED_EDGE('',*,*,#9002,.F.);
#12914=ORIENTED_EDGE('',*,*,#9505,.F.);
#12915=ORIENTED_EDGE('',*,*,#9000,.F.);
#12916=ORIENTED_EDGE('',*,*,#9007,.F.);
#12917=ORIENTED_EDGE('',*,*,#9010,.F.);
#12918=ORIENTED_EDGE('',*,*,#9013,.F.);
#12919=ORIENTED_EDGE('',*,*,#9016,.F.);
#12920=ORIENTED_EDGE('',*,*,#9019,.F.);
#12921=ORIENTED_EDGE('',*,*,#9022,.F.);
#12922=ORIENTED_EDGE('',*,*,#9025,.F.);
#12923=ORIENTED_EDGE('',*,*,#9028,.F.);
#12924=ORIENTED_EDGE('',*,*,#9031,.F.);
#12925=ORIENTED_EDGE('',*,*,#9034,.F.);
#12926=ORIENTED_EDGE('',*,*,#9511,.F.);
#12927=ORIENTED_EDGE('',*,*,#9039,.F.);
#12928=ORIENTED_EDGE('',*,*,#9512,.F.);
#12929=ORIENTED_EDGE('',*,*,#9078,.T.);
#12930=ORIENTED_EDGE('',*,*,#9508,.T.);
#12931=ORIENTED_EDGE('',*,*,#9076,.T.);
#12932=ORIENTED_EDGE('',*,*,#9073,.T.);
#12933=ORIENTED_EDGE('',*,*,#9070,.T.);
#12934=ORIENTED_EDGE('',*,*,#9067,.T.);
#12935=ORIENTED_EDGE('',*,*,#9064,.T.);
#12936=ORIENTED_EDGE('',*,*,#9061,.T.);
#12937=ORIENTED_EDGE('',*,*,#9058,.T.);
#12938=ORIENTED_EDGE('',*,*,#9055,.T.);
#12939=ORIENTED_EDGE('',*,*,#9052,.T.);
#12940=ORIENTED_EDGE('',*,*,#9049,.T.);
#12941=ORIENTED_EDGE('',*,*,#9046,.T.);
#12942=ORIENTED_EDGE('',*,*,#9043,.T.);
#12943=ORIENTED_EDGE('',*,*,#9036,.T.);
#12944=ORIENTED_EDGE('',*,*,#9511,.T.);
#12945=ORIENTED_EDGE('',*,*,#9033,.F.);
#12946=ORIENTED_EDGE('',*,*,#9510,.T.);
#12947=ORIENTED_EDGE('',*,*,#8919,.F.);
#12948=ORIENTED_EDGE('',*,*,#9513,.T.);
#12949=ORIENTED_EDGE('',*,*,#8960,.T.);
#12950=ORIENTED_EDGE('',*,*,#9514,.T.);
#12951=ORIENTED_EDGE('',*,*,#8995,.T.);
#12952=ORIENTED_EDGE('',*,*,#9515,.T.);
#12953=ORIENTED_EDGE('',*,*,#8992,.F.);
#12954=ORIENTED_EDGE('',*,*,#9516,.F.);
#12955=ORIENTED_EDGE('',*,*,#9514,.F.);
#12956=ORIENTED_EDGE('',*,*,#8959,.F.);
#12957=ORIENTED_EDGE('',*,*,#8963,.F.);
#12958=ORIENTED_EDGE('',*,*,#8966,.F.);
#12959=ORIENTED_EDGE('',*,*,#8969,.F.);
#12960=ORIENTED_EDGE('',*,*,#8972,.F.);
#12961=ORIENTED_EDGE('',*,*,#8975,.F.);
#12962=ORIENTED_EDGE('',*,*,#8978,.F.);
#12963=ORIENTED_EDGE('',*,*,#8981,.F.);
#12964=ORIENTED_EDGE('',*,*,#8984,.F.);
#12965=ORIENTED_EDGE('',*,*,#8987,.F.);
#12966=ORIENTED_EDGE('',*,*,#8990,.F.);
#12967=ORIENTED_EDGE('',*,*,#8993,.F.);
#12968=ORIENTED_EDGE('',*,*,#9515,.F.);
#12969=ORIENTED_EDGE('',*,*,#8998,.F.);
#12970=ORIENTED_EDGE('',*,*,#9517,.F.);
#12971=ORIENTED_EDGE('',*,*,#8955,.F.);
#12972=ORIENTED_EDGE('',*,*,#9518,.F.);
#12973=ORIENTED_EDGE('',*,*,#8953,.F.);
#12974=ORIENTED_EDGE('',*,*,#8950,.F.);
#12975=ORIENTED_EDGE('',*,*,#8947,.F.);
#12976=ORIENTED_EDGE('',*,*,#8944,.F.);
#12977=ORIENTED_EDGE('',*,*,#8941,.F.);
#12978=ORIENTED_EDGE('',*,*,#8938,.F.);
#12979=ORIENTED_EDGE('',*,*,#8935,.F.);
#12980=ORIENTED_EDGE('',*,*,#8932,.F.);
#12981=ORIENTED_EDGE('',*,*,#8929,.F.);
#12982=ORIENTED_EDGE('',*,*,#8926,.F.);
#12983=ORIENTED_EDGE('',*,*,#8923,.F.);
#12984=ORIENTED_EDGE('',*,*,#8920,.F.);
#12985=ORIENTED_EDGE('',*,*,#9513,.F.);
#12986=ORIENTED_EDGE('',*,*,#8918,.F.);
#12987=ORIENTED_EDGE('',*,*,#8925,.F.);
#12988=ORIENTED_EDGE('',*,*,#8928,.F.);
#12989=ORIENTED_EDGE('',*,*,#8931,.F.);
#12990=ORIENTED_EDGE('',*,*,#8934,.F.);
#12991=ORIENTED_EDGE('',*,*,#8937,.F.);
#12992=ORIENTED_EDGE('',*,*,#8940,.F.);
#12993=ORIENTED_EDGE('',*,*,#8943,.F.);
#12994=ORIENTED_EDGE('',*,*,#8946,.F.);
#12995=ORIENTED_EDGE('',*,*,#8949,.F.);
#12996=ORIENTED_EDGE('',*,*,#8952,.F.);
#12997=ORIENTED_EDGE('',*,*,#9519,.F.);
#12998=ORIENTED_EDGE('',*,*,#8957,.F.);
#12999=ORIENTED_EDGE('',*,*,#9520,.F.);
#13000=ORIENTED_EDGE('',*,*,#8996,.T.);
#13001=ORIENTED_EDGE('',*,*,#9516,.T.);
#13002=ORIENTED_EDGE('',*,*,#8994,.T.);
#13003=ORIENTED_EDGE('',*,*,#8991,.T.);
#13004=ORIENTED_EDGE('',*,*,#8988,.T.);
#13005=ORIENTED_EDGE('',*,*,#8985,.T.);
#13006=ORIENTED_EDGE('',*,*,#8982,.T.);
#13007=ORIENTED_EDGE('',*,*,#8979,.T.);
#13008=ORIENTED_EDGE('',*,*,#8976,.T.);
#13009=ORIENTED_EDGE('',*,*,#8973,.T.);
#13010=ORIENTED_EDGE('',*,*,#8970,.T.);
#13011=ORIENTED_EDGE('',*,*,#8967,.T.);
#13012=ORIENTED_EDGE('',*,*,#8964,.T.);
#13013=ORIENTED_EDGE('',*,*,#8961,.T.);
#13014=ORIENTED_EDGE('',*,*,#8954,.T.);
#13015=ORIENTED_EDGE('',*,*,#9519,.T.);
#13016=ORIENTED_EDGE('',*,*,#8951,.F.);
#13017=ORIENTED_EDGE('',*,*,#9518,.T.);
#13018=ORIENTED_EDGE('',*,*,#8837,.F.);
#13019=ORIENTED_EDGE('',*,*,#9521,.T.);
#13020=ORIENTED_EDGE('',*,*,#8878,.T.);
#13021=ORIENTED_EDGE('',*,*,#9522,.T.);
#13022=ORIENTED_EDGE('',*,*,#8913,.T.);
#13023=ORIENTED_EDGE('',*,*,#9523,.T.);
#13024=ORIENTED_EDGE('',*,*,#8910,.F.);
#13025=ORIENTED_EDGE('',*,*,#9524,.F.);
#13026=ORIENTED_EDGE('',*,*,#9522,.F.);
#13027=ORIENTED_EDGE('',*,*,#8877,.F.);
#13028=ORIENTED_EDGE('',*,*,#8881,.F.);
#13029=ORIENTED_EDGE('',*,*,#8884,.F.);
#13030=ORIENTED_EDGE('',*,*,#8887,.F.);
#13031=ORIENTED_EDGE('',*,*,#8890,.F.);
#13032=ORIENTED_EDGE('',*,*,#8893,.F.);
#13033=ORIENTED_EDGE('',*,*,#8896,.F.);
#13034=ORIENTED_EDGE('',*,*,#8899,.F.);
#13035=ORIENTED_EDGE('',*,*,#8902,.F.);
#13036=ORIENTED_EDGE('',*,*,#8905,.F.);
#13037=ORIENTED_EDGE('',*,*,#8908,.F.);
#13038=ORIENTED_EDGE('',*,*,#8911,.F.);
#13039=ORIENTED_EDGE('',*,*,#9523,.F.);
#13040=ORIENTED_EDGE('',*,*,#8916,.F.);
#13041=ORIENTED_EDGE('',*,*,#9525,.F.);
#13042=ORIENTED_EDGE('',*,*,#8873,.F.);
#13043=ORIENTED_EDGE('',*,*,#9526,.F.);
#13044=ORIENTED_EDGE('',*,*,#8871,.F.);
#13045=ORIENTED_EDGE('',*,*,#8868,.F.);
#13046=ORIENTED_EDGE('',*,*,#8865,.F.);
#13047=ORIENTED_EDGE('',*,*,#8862,.F.);
#13048=ORIENTED_EDGE('',*,*,#8859,.F.);
#13049=ORIENTED_EDGE('',*,*,#8856,.F.);
#13050=ORIENTED_EDGE('',*,*,#8853,.F.);
#13051=ORIENTED_EDGE('',*,*,#8850,.F.);
#13052=ORIENTED_EDGE('',*,*,#8847,.F.);
#13053=ORIENTED_EDGE('',*,*,#8844,.F.);
#13054=ORIENTED_EDGE('',*,*,#8841,.F.);
#13055=ORIENTED_EDGE('',*,*,#8838,.F.);
#13056=ORIENTED_EDGE('',*,*,#9521,.F.);
#13057=ORIENTED_EDGE('',*,*,#8836,.F.);
#13058=ORIENTED_EDGE('',*,*,#8843,.F.);
#13059=ORIENTED_EDGE('',*,*,#8846,.F.);
#13060=ORIENTED_EDGE('',*,*,#8849,.F.);
#13061=ORIENTED_EDGE('',*,*,#8852,.F.);
#13062=ORIENTED_EDGE('',*,*,#8855,.F.);
#13063=ORIENTED_EDGE('',*,*,#8858,.F.);
#13064=ORIENTED_EDGE('',*,*,#8861,.F.);
#13065=ORIENTED_EDGE('',*,*,#8864,.F.);
#13066=ORIENTED_EDGE('',*,*,#8867,.F.);
#13067=ORIENTED_EDGE('',*,*,#8870,.F.);
#13068=ORIENTED_EDGE('',*,*,#9527,.F.);
#13069=ORIENTED_EDGE('',*,*,#8875,.F.);
#13070=ORIENTED_EDGE('',*,*,#9528,.F.);
#13071=ORIENTED_EDGE('',*,*,#8914,.T.);
#13072=ORIENTED_EDGE('',*,*,#9524,.T.);
#13073=ORIENTED_EDGE('',*,*,#8912,.T.);
#13074=ORIENTED_EDGE('',*,*,#8909,.T.);
#13075=ORIENTED_EDGE('',*,*,#8906,.T.);
#13076=ORIENTED_EDGE('',*,*,#8903,.T.);
#13077=ORIENTED_EDGE('',*,*,#8900,.T.);
#13078=ORIENTED_EDGE('',*,*,#8897,.T.);
#13079=ORIENTED_EDGE('',*,*,#8894,.T.);
#13080=ORIENTED_EDGE('',*,*,#8891,.T.);
#13081=ORIENTED_EDGE('',*,*,#8888,.T.);
#13082=ORIENTED_EDGE('',*,*,#8885,.T.);
#13083=ORIENTED_EDGE('',*,*,#8882,.T.);
#13084=ORIENTED_EDGE('',*,*,#8879,.T.);
#13085=ORIENTED_EDGE('',*,*,#8872,.T.);
#13086=ORIENTED_EDGE('',*,*,#9527,.T.);
#13087=ORIENTED_EDGE('',*,*,#8869,.F.);
#13088=ORIENTED_EDGE('',*,*,#9526,.T.);
#13089=ORIENTED_EDGE('',*,*,#9168,.F.);
#13090=ORIENTED_EDGE('',*,*,#9086,.F.);
#13091=ORIENTED_EDGE('',*,*,#9004,.F.);
#13092=ORIENTED_EDGE('',*,*,#8922,.F.);
#13093=ORIENTED_EDGE('',*,*,#8840,.F.);
#13094=ORIENTED_EDGE('',*,*,#8755,.F.);
#13095=ORIENTED_EDGE('',*,*,#9529,.T.);
#13096=ORIENTED_EDGE('',*,*,#8796,.T.);
#13097=ORIENTED_EDGE('',*,*,#9530,.T.);
#13098=ORIENTED_EDGE('',*,*,#8831,.T.);
#13099=ORIENTED_EDGE('',*,*,#9531,.T.);
#13100=ORIENTED_EDGE('',*,*,#8828,.F.);
#13101=ORIENTED_EDGE('',*,*,#9532,.F.);
#13102=ORIENTED_EDGE('',*,*,#9530,.F.);
#13103=ORIENTED_EDGE('',*,*,#8795,.F.);
#13104=ORIENTED_EDGE('',*,*,#8799,.F.);
#13105=ORIENTED_EDGE('',*,*,#8802,.F.);
#13106=ORIENTED_EDGE('',*,*,#8805,.F.);
#13107=ORIENTED_EDGE('',*,*,#8808,.F.);
#13108=ORIENTED_EDGE('',*,*,#8811,.F.);
#13109=ORIENTED_EDGE('',*,*,#8814,.F.);
#13110=ORIENTED_EDGE('',*,*,#8817,.F.);
#13111=ORIENTED_EDGE('',*,*,#8820,.F.);
#13112=ORIENTED_EDGE('',*,*,#8823,.F.);
#13113=ORIENTED_EDGE('',*,*,#8826,.F.);
#13114=ORIENTED_EDGE('',*,*,#8829,.F.);
#13115=ORIENTED_EDGE('',*,*,#9531,.F.);
#13116=ORIENTED_EDGE('',*,*,#8834,.F.);
#13117=ORIENTED_EDGE('',*,*,#9533,.F.);
#13118=ORIENTED_EDGE('',*,*,#8791,.F.);
#13119=ORIENTED_EDGE('',*,*,#9534,.F.);
#13120=ORIENTED_EDGE('',*,*,#8789,.F.);
#13121=ORIENTED_EDGE('',*,*,#8786,.F.);
#13122=ORIENTED_EDGE('',*,*,#8783,.F.);
#13123=ORIENTED_EDGE('',*,*,#8780,.F.);
#13124=ORIENTED_EDGE('',*,*,#8777,.F.);
#13125=ORIENTED_EDGE('',*,*,#8774,.F.);
#13126=ORIENTED_EDGE('',*,*,#8771,.F.);
#13127=ORIENTED_EDGE('',*,*,#8768,.F.);
#13128=ORIENTED_EDGE('',*,*,#8765,.F.);
#13129=ORIENTED_EDGE('',*,*,#8762,.F.);
#13130=ORIENTED_EDGE('',*,*,#8759,.F.);
#13131=ORIENTED_EDGE('',*,*,#8756,.F.);
#13132=ORIENTED_EDGE('',*,*,#9529,.F.);
#13133=ORIENTED_EDGE('',*,*,#8754,.F.);
#13134=ORIENTED_EDGE('',*,*,#8761,.F.);
#13135=ORIENTED_EDGE('',*,*,#8764,.F.);
#13136=ORIENTED_EDGE('',*,*,#8767,.F.);
#13137=ORIENTED_EDGE('',*,*,#8770,.F.);
#13138=ORIENTED_EDGE('',*,*,#8773,.F.);
#13139=ORIENTED_EDGE('',*,*,#8776,.F.);
#13140=ORIENTED_EDGE('',*,*,#8779,.F.);
#13141=ORIENTED_EDGE('',*,*,#8782,.F.);
#13142=ORIENTED_EDGE('',*,*,#8785,.F.);
#13143=ORIENTED_EDGE('',*,*,#8788,.F.);
#13144=ORIENTED_EDGE('',*,*,#9535,.F.);
#13145=ORIENTED_EDGE('',*,*,#8793,.F.);
#13146=ORIENTED_EDGE('',*,*,#9536,.F.);
#13147=ORIENTED_EDGE('',*,*,#8832,.T.);
#13148=ORIENTED_EDGE('',*,*,#9532,.T.);
#13149=ORIENTED_EDGE('',*,*,#8830,.T.);
#13150=ORIENTED_EDGE('',*,*,#8827,.T.);
#13151=ORIENTED_EDGE('',*,*,#8824,.T.);
#13152=ORIENTED_EDGE('',*,*,#8821,.T.);
#13153=ORIENTED_EDGE('',*,*,#8818,.T.);
#13154=ORIENTED_EDGE('',*,*,#8815,.T.);
#13155=ORIENTED_EDGE('',*,*,#8812,.T.);
#13156=ORIENTED_EDGE('',*,*,#8809,.T.);
#13157=ORIENTED_EDGE('',*,*,#8806,.T.);
#13158=ORIENTED_EDGE('',*,*,#8803,.T.);
#13159=ORIENTED_EDGE('',*,*,#8800,.T.);
#13160=ORIENTED_EDGE('',*,*,#8797,.T.);
#13161=ORIENTED_EDGE('',*,*,#8790,.T.);
#13162=ORIENTED_EDGE('',*,*,#9535,.T.);
#13163=ORIENTED_EDGE('',*,*,#8787,.F.);
#13164=ORIENTED_EDGE('',*,*,#9534,.T.);
#13165=ORIENTED_EDGE('',*,*,#8673,.F.);
#13166=ORIENTED_EDGE('',*,*,#9537,.T.);
#13167=ORIENTED_EDGE('',*,*,#8714,.T.);
#13168=ORIENTED_EDGE('',*,*,#9538,.T.);
#13169=ORIENTED_EDGE('',*,*,#8749,.T.);
#13170=ORIENTED_EDGE('',*,*,#9539,.T.);
#13171=ORIENTED_EDGE('',*,*,#8746,.F.);
#13172=ORIENTED_EDGE('',*,*,#9540,.F.);
#13173=ORIENTED_EDGE('',*,*,#9538,.F.);
#13174=ORIENTED_EDGE('',*,*,#8713,.F.);
#13175=ORIENTED_EDGE('',*,*,#8717,.F.);
#13176=ORIENTED_EDGE('',*,*,#8720,.F.);
#13177=ORIENTED_EDGE('',*,*,#8723,.F.);
#13178=ORIENTED_EDGE('',*,*,#8726,.F.);
#13179=ORIENTED_EDGE('',*,*,#8729,.F.);
#13180=ORIENTED_EDGE('',*,*,#8732,.F.);
#13181=ORIENTED_EDGE('',*,*,#8735,.F.);
#13182=ORIENTED_EDGE('',*,*,#8738,.F.);
#13183=ORIENTED_EDGE('',*,*,#8741,.F.);
#13184=ORIENTED_EDGE('',*,*,#8744,.F.);
#13185=ORIENTED_EDGE('',*,*,#8747,.F.);
#13186=ORIENTED_EDGE('',*,*,#9539,.F.);
#13187=ORIENTED_EDGE('',*,*,#8752,.F.);
#13188=ORIENTED_EDGE('',*,*,#9541,.F.);
#13189=ORIENTED_EDGE('',*,*,#8709,.F.);
#13190=ORIENTED_EDGE('',*,*,#9542,.F.);
#13191=ORIENTED_EDGE('',*,*,#8707,.F.);
#13192=ORIENTED_EDGE('',*,*,#8704,.F.);
#13193=ORIENTED_EDGE('',*,*,#8701,.F.);
#13194=ORIENTED_EDGE('',*,*,#8698,.F.);
#13195=ORIENTED_EDGE('',*,*,#8695,.F.);
#13196=ORIENTED_EDGE('',*,*,#8692,.F.);
#13197=ORIENTED_EDGE('',*,*,#8689,.F.);
#13198=ORIENTED_EDGE('',*,*,#8686,.F.);
#13199=ORIENTED_EDGE('',*,*,#8683,.F.);
#13200=ORIENTED_EDGE('',*,*,#8680,.F.);
#13201=ORIENTED_EDGE('',*,*,#8677,.F.);
#13202=ORIENTED_EDGE('',*,*,#8674,.F.);
#13203=ORIENTED_EDGE('',*,*,#9537,.F.);
#13204=ORIENTED_EDGE('',*,*,#8672,.F.);
#13205=ORIENTED_EDGE('',*,*,#8679,.F.);
#13206=ORIENTED_EDGE('',*,*,#8682,.F.);
#13207=ORIENTED_EDGE('',*,*,#8685,.F.);
#13208=ORIENTED_EDGE('',*,*,#8688,.F.);
#13209=ORIENTED_EDGE('',*,*,#8691,.F.);
#13210=ORIENTED_EDGE('',*,*,#8694,.F.);
#13211=ORIENTED_EDGE('',*,*,#8697,.F.);
#13212=ORIENTED_EDGE('',*,*,#8700,.F.);
#13213=ORIENTED_EDGE('',*,*,#8703,.F.);
#13214=ORIENTED_EDGE('',*,*,#8706,.F.);
#13215=ORIENTED_EDGE('',*,*,#9543,.F.);
#13216=ORIENTED_EDGE('',*,*,#8711,.F.);
#13217=ORIENTED_EDGE('',*,*,#9544,.F.);
#13218=ORIENTED_EDGE('',*,*,#8750,.T.);
#13219=ORIENTED_EDGE('',*,*,#9540,.T.);
#13220=ORIENTED_EDGE('',*,*,#8748,.T.);
#13221=ORIENTED_EDGE('',*,*,#8745,.T.);
#13222=ORIENTED_EDGE('',*,*,#8742,.T.);
#13223=ORIENTED_EDGE('',*,*,#8739,.T.);
#13224=ORIENTED_EDGE('',*,*,#8736,.T.);
#13225=ORIENTED_EDGE('',*,*,#8733,.T.);
#13226=ORIENTED_EDGE('',*,*,#8730,.T.);
#13227=ORIENTED_EDGE('',*,*,#8727,.T.);
#13228=ORIENTED_EDGE('',*,*,#8724,.T.);
#13229=ORIENTED_EDGE('',*,*,#8721,.T.);
#13230=ORIENTED_EDGE('',*,*,#8718,.T.);
#13231=ORIENTED_EDGE('',*,*,#8715,.T.);
#13232=ORIENTED_EDGE('',*,*,#8708,.T.);
#13233=ORIENTED_EDGE('',*,*,#9543,.T.);
#13234=ORIENTED_EDGE('',*,*,#8705,.F.);
#13235=ORIENTED_EDGE('',*,*,#9542,.T.);
#13236=ORIENTED_EDGE('',*,*,#8591,.F.);
#13237=ORIENTED_EDGE('',*,*,#9545,.T.);
#13238=ORIENTED_EDGE('',*,*,#8632,.T.);
#13239=ORIENTED_EDGE('',*,*,#9546,.T.);
#13240=ORIENTED_EDGE('',*,*,#8667,.T.);
#13241=ORIENTED_EDGE('',*,*,#9547,.T.);
#13242=ORIENTED_EDGE('',*,*,#8664,.F.);
#13243=ORIENTED_EDGE('',*,*,#9548,.F.);
#13244=ORIENTED_EDGE('',*,*,#9546,.F.);
#13245=ORIENTED_EDGE('',*,*,#8631,.F.);
#13246=ORIENTED_EDGE('',*,*,#8635,.F.);
#13247=ORIENTED_EDGE('',*,*,#8638,.F.);
#13248=ORIENTED_EDGE('',*,*,#8641,.F.);
#13249=ORIENTED_EDGE('',*,*,#8644,.F.);
#13250=ORIENTED_EDGE('',*,*,#8647,.F.);
#13251=ORIENTED_EDGE('',*,*,#8650,.F.);
#13252=ORIENTED_EDGE('',*,*,#8653,.F.);
#13253=ORIENTED_EDGE('',*,*,#8656,.F.);
#13254=ORIENTED_EDGE('',*,*,#8659,.F.);
#13255=ORIENTED_EDGE('',*,*,#8662,.F.);
#13256=ORIENTED_EDGE('',*,*,#8665,.F.);
#13257=ORIENTED_EDGE('',*,*,#9547,.F.);
#13258=ORIENTED_EDGE('',*,*,#8670,.F.);
#13259=ORIENTED_EDGE('',*,*,#9549,.F.);
#13260=ORIENTED_EDGE('',*,*,#8627,.F.);
#13261=ORIENTED_EDGE('',*,*,#9550,.F.);
#13262=ORIENTED_EDGE('',*,*,#8625,.F.);
#13263=ORIENTED_EDGE('',*,*,#8622,.F.);
#13264=ORIENTED_EDGE('',*,*,#8619,.F.);
#13265=ORIENTED_EDGE('',*,*,#8616,.F.);
#13266=ORIENTED_EDGE('',*,*,#8613,.F.);
#13267=ORIENTED_EDGE('',*,*,#8610,.F.);
#13268=ORIENTED_EDGE('',*,*,#8607,.F.);
#13269=ORIENTED_EDGE('',*,*,#8604,.F.);
#13270=ORIENTED_EDGE('',*,*,#8601,.F.);
#13271=ORIENTED_EDGE('',*,*,#8598,.F.);
#13272=ORIENTED_EDGE('',*,*,#8595,.F.);
#13273=ORIENTED_EDGE('',*,*,#8592,.F.);
#13274=ORIENTED_EDGE('',*,*,#9545,.F.);
#13275=ORIENTED_EDGE('',*,*,#8590,.F.);
#13276=ORIENTED_EDGE('',*,*,#8597,.F.);
#13277=ORIENTED_EDGE('',*,*,#8600,.F.);
#13278=ORIENTED_EDGE('',*,*,#8603,.F.);
#13279=ORIENTED_EDGE('',*,*,#8606,.F.);
#13280=ORIENTED_EDGE('',*,*,#8609,.F.);
#13281=ORIENTED_EDGE('',*,*,#8612,.F.);
#13282=ORIENTED_EDGE('',*,*,#8615,.F.);
#13283=ORIENTED_EDGE('',*,*,#8618,.F.);
#13284=ORIENTED_EDGE('',*,*,#8621,.F.);
#13285=ORIENTED_EDGE('',*,*,#8624,.F.);
#13286=ORIENTED_EDGE('',*,*,#9551,.F.);
#13287=ORIENTED_EDGE('',*,*,#8629,.F.);
#13288=ORIENTED_EDGE('',*,*,#9552,.F.);
#13289=ORIENTED_EDGE('',*,*,#8668,.T.);
#13290=ORIENTED_EDGE('',*,*,#9548,.T.);
#13291=ORIENTED_EDGE('',*,*,#8666,.T.);
#13292=ORIENTED_EDGE('',*,*,#8663,.T.);
#13293=ORIENTED_EDGE('',*,*,#8660,.T.);
#13294=ORIENTED_EDGE('',*,*,#8657,.T.);
#13295=ORIENTED_EDGE('',*,*,#8654,.T.);
#13296=ORIENTED_EDGE('',*,*,#8651,.T.);
#13297=ORIENTED_EDGE('',*,*,#8648,.T.);
#13298=ORIENTED_EDGE('',*,*,#8645,.T.);
#13299=ORIENTED_EDGE('',*,*,#8642,.T.);
#13300=ORIENTED_EDGE('',*,*,#8639,.T.);
#13301=ORIENTED_EDGE('',*,*,#8636,.T.);
#13302=ORIENTED_EDGE('',*,*,#8633,.T.);
#13303=ORIENTED_EDGE('',*,*,#8626,.T.);
#13304=ORIENTED_EDGE('',*,*,#9551,.T.);
#13305=ORIENTED_EDGE('',*,*,#8623,.F.);
#13306=ORIENTED_EDGE('',*,*,#9550,.T.);
#13307=ORIENTED_EDGE('',*,*,#8509,.F.);
#13308=ORIENTED_EDGE('',*,*,#9553,.T.);
#13309=ORIENTED_EDGE('',*,*,#8550,.T.);
#13310=ORIENTED_EDGE('',*,*,#9554,.T.);
#13311=ORIENTED_EDGE('',*,*,#8585,.T.);
#13312=ORIENTED_EDGE('',*,*,#9555,.T.);
#13313=ORIENTED_EDGE('',*,*,#8582,.F.);
#13314=ORIENTED_EDGE('',*,*,#9556,.F.);
#13315=ORIENTED_EDGE('',*,*,#9554,.F.);
#13316=ORIENTED_EDGE('',*,*,#8549,.F.);
#13317=ORIENTED_EDGE('',*,*,#8553,.F.);
#13318=ORIENTED_EDGE('',*,*,#8556,.F.);
#13319=ORIENTED_EDGE('',*,*,#8559,.F.);
#13320=ORIENTED_EDGE('',*,*,#8562,.F.);
#13321=ORIENTED_EDGE('',*,*,#8565,.F.);
#13322=ORIENTED_EDGE('',*,*,#8568,.F.);
#13323=ORIENTED_EDGE('',*,*,#8571,.F.);
#13324=ORIENTED_EDGE('',*,*,#8574,.F.);
#13325=ORIENTED_EDGE('',*,*,#8577,.F.);
#13326=ORIENTED_EDGE('',*,*,#8580,.F.);
#13327=ORIENTED_EDGE('',*,*,#8583,.F.);
#13328=ORIENTED_EDGE('',*,*,#9555,.F.);
#13329=ORIENTED_EDGE('',*,*,#8588,.F.);
#13330=ORIENTED_EDGE('',*,*,#9557,.F.);
#13331=ORIENTED_EDGE('',*,*,#8545,.F.);
#13332=ORIENTED_EDGE('',*,*,#9558,.F.);
#13333=ORIENTED_EDGE('',*,*,#8543,.F.);
#13334=ORIENTED_EDGE('',*,*,#8540,.F.);
#13335=ORIENTED_EDGE('',*,*,#8537,.F.);
#13336=ORIENTED_EDGE('',*,*,#8534,.F.);
#13337=ORIENTED_EDGE('',*,*,#8531,.F.);
#13338=ORIENTED_EDGE('',*,*,#8528,.F.);
#13339=ORIENTED_EDGE('',*,*,#8525,.F.);
#13340=ORIENTED_EDGE('',*,*,#8522,.F.);
#13341=ORIENTED_EDGE('',*,*,#8519,.F.);
#13342=ORIENTED_EDGE('',*,*,#8516,.F.);
#13343=ORIENTED_EDGE('',*,*,#8513,.F.);
#13344=ORIENTED_EDGE('',*,*,#8510,.F.);
#13345=ORIENTED_EDGE('',*,*,#9553,.F.);
#13346=ORIENTED_EDGE('',*,*,#8508,.F.);
#13347=ORIENTED_EDGE('',*,*,#8515,.F.);
#13348=ORIENTED_EDGE('',*,*,#8518,.F.);
#13349=ORIENTED_EDGE('',*,*,#8521,.F.);
#13350=ORIENTED_EDGE('',*,*,#8524,.F.);
#13351=ORIENTED_EDGE('',*,*,#8527,.F.);
#13352=ORIENTED_EDGE('',*,*,#8530,.F.);
#13353=ORIENTED_EDGE('',*,*,#8533,.F.);
#13354=ORIENTED_EDGE('',*,*,#8536,.F.);
#13355=ORIENTED_EDGE('',*,*,#8539,.F.);
#13356=ORIENTED_EDGE('',*,*,#8542,.F.);
#13357=ORIENTED_EDGE('',*,*,#9559,.F.);
#13358=ORIENTED_EDGE('',*,*,#8547,.F.);
#13359=ORIENTED_EDGE('',*,*,#9560,.F.);
#13360=ORIENTED_EDGE('',*,*,#8586,.T.);
#13361=ORIENTED_EDGE('',*,*,#9556,.T.);
#13362=ORIENTED_EDGE('',*,*,#8584,.T.);
#13363=ORIENTED_EDGE('',*,*,#8581,.T.);
#13364=ORIENTED_EDGE('',*,*,#8578,.T.);
#13365=ORIENTED_EDGE('',*,*,#8575,.T.);
#13366=ORIENTED_EDGE('',*,*,#8572,.T.);
#13367=ORIENTED_EDGE('',*,*,#8569,.T.);
#13368=ORIENTED_EDGE('',*,*,#8566,.T.);
#13369=ORIENTED_EDGE('',*,*,#8563,.T.);
#13370=ORIENTED_EDGE('',*,*,#8560,.T.);
#13371=ORIENTED_EDGE('',*,*,#8557,.T.);
#13372=ORIENTED_EDGE('',*,*,#8554,.T.);
#13373=ORIENTED_EDGE('',*,*,#8551,.T.);
#13374=ORIENTED_EDGE('',*,*,#8544,.T.);
#13375=ORIENTED_EDGE('',*,*,#9559,.T.);
#13376=ORIENTED_EDGE('',*,*,#8541,.F.);
#13377=ORIENTED_EDGE('',*,*,#9558,.T.);
#13378=ORIENTED_EDGE('',*,*,#8427,.F.);
#13379=ORIENTED_EDGE('',*,*,#9561,.T.);
#13380=ORIENTED_EDGE('',*,*,#8468,.T.);
#13381=ORIENTED_EDGE('',*,*,#9562,.T.);
#13382=ORIENTED_EDGE('',*,*,#8503,.T.);
#13383=ORIENTED_EDGE('',*,*,#9563,.T.);
#13384=ORIENTED_EDGE('',*,*,#8500,.F.);
#13385=ORIENTED_EDGE('',*,*,#9564,.F.);
#13386=ORIENTED_EDGE('',*,*,#9562,.F.);
#13387=ORIENTED_EDGE('',*,*,#8467,.F.);
#13388=ORIENTED_EDGE('',*,*,#8471,.F.);
#13389=ORIENTED_EDGE('',*,*,#8474,.F.);
#13390=ORIENTED_EDGE('',*,*,#8477,.F.);
#13391=ORIENTED_EDGE('',*,*,#8480,.F.);
#13392=ORIENTED_EDGE('',*,*,#8483,.F.);
#13393=ORIENTED_EDGE('',*,*,#8486,.F.);
#13394=ORIENTED_EDGE('',*,*,#8489,.F.);
#13395=ORIENTED_EDGE('',*,*,#8492,.F.);
#13396=ORIENTED_EDGE('',*,*,#8495,.F.);
#13397=ORIENTED_EDGE('',*,*,#8498,.F.);
#13398=ORIENTED_EDGE('',*,*,#8501,.F.);
#13399=ORIENTED_EDGE('',*,*,#9563,.F.);
#13400=ORIENTED_EDGE('',*,*,#8506,.F.);
#13401=ORIENTED_EDGE('',*,*,#9565,.F.);
#13402=ORIENTED_EDGE('',*,*,#8463,.F.);
#13403=ORIENTED_EDGE('',*,*,#9566,.F.);
#13404=ORIENTED_EDGE('',*,*,#8461,.F.);
#13405=ORIENTED_EDGE('',*,*,#8458,.F.);
#13406=ORIENTED_EDGE('',*,*,#8455,.F.);
#13407=ORIENTED_EDGE('',*,*,#8452,.F.);
#13408=ORIENTED_EDGE('',*,*,#8449,.F.);
#13409=ORIENTED_EDGE('',*,*,#8446,.F.);
#13410=ORIENTED_EDGE('',*,*,#8443,.F.);
#13411=ORIENTED_EDGE('',*,*,#8440,.F.);
#13412=ORIENTED_EDGE('',*,*,#8437,.F.);
#13413=ORIENTED_EDGE('',*,*,#8434,.F.);
#13414=ORIENTED_EDGE('',*,*,#8431,.F.);
#13415=ORIENTED_EDGE('',*,*,#8428,.F.);
#13416=ORIENTED_EDGE('',*,*,#9561,.F.);
#13417=ORIENTED_EDGE('',*,*,#8426,.F.);
#13418=ORIENTED_EDGE('',*,*,#8433,.F.);
#13419=ORIENTED_EDGE('',*,*,#8436,.F.);
#13420=ORIENTED_EDGE('',*,*,#8439,.F.);
#13421=ORIENTED_EDGE('',*,*,#8442,.F.);
#13422=ORIENTED_EDGE('',*,*,#8445,.F.);
#13423=ORIENTED_EDGE('',*,*,#8448,.F.);
#13424=ORIENTED_EDGE('',*,*,#8451,.F.);
#13425=ORIENTED_EDGE('',*,*,#8454,.F.);
#13426=ORIENTED_EDGE('',*,*,#8457,.F.);
#13427=ORIENTED_EDGE('',*,*,#8460,.F.);
#13428=ORIENTED_EDGE('',*,*,#9567,.F.);
#13429=ORIENTED_EDGE('',*,*,#8465,.F.);
#13430=ORIENTED_EDGE('',*,*,#9568,.F.);
#13431=ORIENTED_EDGE('',*,*,#8504,.T.);
#13432=ORIENTED_EDGE('',*,*,#9564,.T.);
#13433=ORIENTED_EDGE('',*,*,#8502,.T.);
#13434=ORIENTED_EDGE('',*,*,#8499,.T.);
#13435=ORIENTED_EDGE('',*,*,#8496,.T.);
#13436=ORIENTED_EDGE('',*,*,#8493,.T.);
#13437=ORIENTED_EDGE('',*,*,#8490,.T.);
#13438=ORIENTED_EDGE('',*,*,#8487,.T.);
#13439=ORIENTED_EDGE('',*,*,#8484,.T.);
#13440=ORIENTED_EDGE('',*,*,#8481,.T.);
#13441=ORIENTED_EDGE('',*,*,#8478,.T.);
#13442=ORIENTED_EDGE('',*,*,#8475,.T.);
#13443=ORIENTED_EDGE('',*,*,#8472,.T.);
#13444=ORIENTED_EDGE('',*,*,#8469,.T.);
#13445=ORIENTED_EDGE('',*,*,#8462,.T.);
#13446=ORIENTED_EDGE('',*,*,#9567,.T.);
#13447=ORIENTED_EDGE('',*,*,#8459,.F.);
#13448=ORIENTED_EDGE('',*,*,#9566,.T.);
#13449=ORIENTED_EDGE('',*,*,#8758,.F.);
#13450=ORIENTED_EDGE('',*,*,#8676,.F.);
#13451=ORIENTED_EDGE('',*,*,#8594,.F.);
#13452=ORIENTED_EDGE('',*,*,#8512,.F.);
#13453=ORIENTED_EDGE('',*,*,#8430,.F.);
#13454=ORIENTED_EDGE('',*,*,#8345,.F.);
#13455=ORIENTED_EDGE('',*,*,#9569,.T.);
#13456=ORIENTED_EDGE('',*,*,#8386,.T.);
#13457=ORIENTED_EDGE('',*,*,#9570,.T.);
#13458=ORIENTED_EDGE('',*,*,#8421,.T.);
#13459=ORIENTED_EDGE('',*,*,#9571,.T.);
#13460=ORIENTED_EDGE('',*,*,#8418,.F.);
#13461=ORIENTED_EDGE('',*,*,#9572,.F.);
#13462=ORIENTED_EDGE('',*,*,#9570,.F.);
#13463=ORIENTED_EDGE('',*,*,#8385,.F.);
#13464=ORIENTED_EDGE('',*,*,#8389,.F.);
#13465=ORIENTED_EDGE('',*,*,#8392,.F.);
#13466=ORIENTED_EDGE('',*,*,#8395,.F.);
#13467=ORIENTED_EDGE('',*,*,#8398,.F.);
#13468=ORIENTED_EDGE('',*,*,#8401,.F.);
#13469=ORIENTED_EDGE('',*,*,#8404,.F.);
#13470=ORIENTED_EDGE('',*,*,#8407,.F.);
#13471=ORIENTED_EDGE('',*,*,#8410,.F.);
#13472=ORIENTED_EDGE('',*,*,#8413,.F.);
#13473=ORIENTED_EDGE('',*,*,#8416,.F.);
#13474=ORIENTED_EDGE('',*,*,#8419,.F.);
#13475=ORIENTED_EDGE('',*,*,#9571,.F.);
#13476=ORIENTED_EDGE('',*,*,#8424,.F.);
#13477=ORIENTED_EDGE('',*,*,#9573,.F.);
#13478=ORIENTED_EDGE('',*,*,#8381,.F.);
#13479=ORIENTED_EDGE('',*,*,#9574,.F.);
#13480=ORIENTED_EDGE('',*,*,#8379,.F.);
#13481=ORIENTED_EDGE('',*,*,#8376,.F.);
#13482=ORIENTED_EDGE('',*,*,#8373,.F.);
#13483=ORIENTED_EDGE('',*,*,#8370,.F.);
#13484=ORIENTED_EDGE('',*,*,#8367,.F.);
#13485=ORIENTED_EDGE('',*,*,#8364,.F.);
#13486=ORIENTED_EDGE('',*,*,#8361,.F.);
#13487=ORIENTED_EDGE('',*,*,#8358,.F.);
#13488=ORIENTED_EDGE('',*,*,#8355,.F.);
#13489=ORIENTED_EDGE('',*,*,#8352,.F.);
#13490=ORIENTED_EDGE('',*,*,#8349,.F.);
#13491=ORIENTED_EDGE('',*,*,#8346,.F.);
#13492=ORIENTED_EDGE('',*,*,#9569,.F.);
#13493=ORIENTED_EDGE('',*,*,#8344,.F.);
#13494=ORIENTED_EDGE('',*,*,#8351,.F.);
#13495=ORIENTED_EDGE('',*,*,#8354,.F.);
#13496=ORIENTED_EDGE('',*,*,#8357,.F.);
#13497=ORIENTED_EDGE('',*,*,#8360,.F.);
#13498=ORIENTED_EDGE('',*,*,#8363,.F.);
#13499=ORIENTED_EDGE('',*,*,#8366,.F.);
#13500=ORIENTED_EDGE('',*,*,#8369,.F.);
#13501=ORIENTED_EDGE('',*,*,#8372,.F.);
#13502=ORIENTED_EDGE('',*,*,#8375,.F.);
#13503=ORIENTED_EDGE('',*,*,#8378,.F.);
#13504=ORIENTED_EDGE('',*,*,#9575,.F.);
#13505=ORIENTED_EDGE('',*,*,#8383,.F.);
#13506=ORIENTED_EDGE('',*,*,#9576,.F.);
#13507=ORIENTED_EDGE('',*,*,#8422,.T.);
#13508=ORIENTED_EDGE('',*,*,#9572,.T.);
#13509=ORIENTED_EDGE('',*,*,#8420,.T.);
#13510=ORIENTED_EDGE('',*,*,#8417,.T.);
#13511=ORIENTED_EDGE('',*,*,#8414,.T.);
#13512=ORIENTED_EDGE('',*,*,#8411,.T.);
#13513=ORIENTED_EDGE('',*,*,#8408,.T.);
#13514=ORIENTED_EDGE('',*,*,#8405,.T.);
#13515=ORIENTED_EDGE('',*,*,#8402,.T.);
#13516=ORIENTED_EDGE('',*,*,#8399,.T.);
#13517=ORIENTED_EDGE('',*,*,#8396,.T.);
#13518=ORIENTED_EDGE('',*,*,#8393,.T.);
#13519=ORIENTED_EDGE('',*,*,#8390,.T.);
#13520=ORIENTED_EDGE('',*,*,#8387,.T.);
#13521=ORIENTED_EDGE('',*,*,#8380,.T.);
#13522=ORIENTED_EDGE('',*,*,#9575,.T.);
#13523=ORIENTED_EDGE('',*,*,#8377,.F.);
#13524=ORIENTED_EDGE('',*,*,#9574,.T.);
#13525=ORIENTED_EDGE('',*,*,#8348,.F.);
#13526=ORIENTED_EDGE('',*,*,#8263,.F.);
#13527=ORIENTED_EDGE('',*,*,#9577,.T.);
#13528=ORIENTED_EDGE('',*,*,#8304,.T.);
#13529=ORIENTED_EDGE('',*,*,#9578,.T.);
#13530=ORIENTED_EDGE('',*,*,#8339,.T.);
#13531=ORIENTED_EDGE('',*,*,#9579,.T.);
#13532=ORIENTED_EDGE('',*,*,#8336,.F.);
#13533=ORIENTED_EDGE('',*,*,#9580,.F.);
#13534=ORIENTED_EDGE('',*,*,#9578,.F.);
#13535=ORIENTED_EDGE('',*,*,#8303,.F.);
#13536=ORIENTED_EDGE('',*,*,#8307,.F.);
#13537=ORIENTED_EDGE('',*,*,#8310,.F.);
#13538=ORIENTED_EDGE('',*,*,#8313,.F.);
#13539=ORIENTED_EDGE('',*,*,#8316,.F.);
#13540=ORIENTED_EDGE('',*,*,#8319,.F.);
#13541=ORIENTED_EDGE('',*,*,#8322,.F.);
#13542=ORIENTED_EDGE('',*,*,#8325,.F.);
#13543=ORIENTED_EDGE('',*,*,#8328,.F.);
#13544=ORIENTED_EDGE('',*,*,#8331,.F.);
#13545=ORIENTED_EDGE('',*,*,#8334,.F.);
#13546=ORIENTED_EDGE('',*,*,#8337,.F.);
#13547=ORIENTED_EDGE('',*,*,#9579,.F.);
#13548=ORIENTED_EDGE('',*,*,#8342,.F.);
#13549=ORIENTED_EDGE('',*,*,#9581,.F.);
#13550=ORIENTED_EDGE('',*,*,#8299,.F.);
#13551=ORIENTED_EDGE('',*,*,#9582,.F.);
#13552=ORIENTED_EDGE('',*,*,#8297,.F.);
#13553=ORIENTED_EDGE('',*,*,#8294,.F.);
#13554=ORIENTED_EDGE('',*,*,#8291,.F.);
#13555=ORIENTED_EDGE('',*,*,#8288,.F.);
#13556=ORIENTED_EDGE('',*,*,#8285,.F.);
#13557=ORIENTED_EDGE('',*,*,#8282,.F.);
#13558=ORIENTED_EDGE('',*,*,#8279,.F.);
#13559=ORIENTED_EDGE('',*,*,#8276,.F.);
#13560=ORIENTED_EDGE('',*,*,#8273,.F.);
#13561=ORIENTED_EDGE('',*,*,#8270,.F.);
#13562=ORIENTED_EDGE('',*,*,#8267,.F.);
#13563=ORIENTED_EDGE('',*,*,#8264,.F.);
#13564=ORIENTED_EDGE('',*,*,#9577,.F.);
#13565=ORIENTED_EDGE('',*,*,#8262,.F.);
#13566=ORIENTED_EDGE('',*,*,#8269,.F.);
#13567=ORIENTED_EDGE('',*,*,#8272,.F.);
#13568=ORIENTED_EDGE('',*,*,#8275,.F.);
#13569=ORIENTED_EDGE('',*,*,#8278,.F.);
#13570=ORIENTED_EDGE('',*,*,#8281,.F.);
#13571=ORIENTED_EDGE('',*,*,#8284,.F.);
#13572=ORIENTED_EDGE('',*,*,#8287,.F.);
#13573=ORIENTED_EDGE('',*,*,#8290,.F.);
#13574=ORIENTED_EDGE('',*,*,#8293,.F.);
#13575=ORIENTED_EDGE('',*,*,#8296,.F.);
#13576=ORIENTED_EDGE('',*,*,#9583,.F.);
#13577=ORIENTED_EDGE('',*,*,#8301,.F.);
#13578=ORIENTED_EDGE('',*,*,#9584,.F.);
#13579=ORIENTED_EDGE('',*,*,#8340,.T.);
#13580=ORIENTED_EDGE('',*,*,#9580,.T.);
#13581=ORIENTED_EDGE('',*,*,#8338,.T.);
#13582=ORIENTED_EDGE('',*,*,#8335,.T.);
#13583=ORIENTED_EDGE('',*,*,#8332,.T.);
#13584=ORIENTED_EDGE('',*,*,#8329,.T.);
#13585=ORIENTED_EDGE('',*,*,#8326,.T.);
#13586=ORIENTED_EDGE('',*,*,#8323,.T.);
#13587=ORIENTED_EDGE('',*,*,#8320,.T.);
#13588=ORIENTED_EDGE('',*,*,#8317,.T.);
#13589=ORIENTED_EDGE('',*,*,#8314,.T.);
#13590=ORIENTED_EDGE('',*,*,#8311,.T.);
#13591=ORIENTED_EDGE('',*,*,#8308,.T.);
#13592=ORIENTED_EDGE('',*,*,#8305,.T.);
#13593=ORIENTED_EDGE('',*,*,#8298,.T.);
#13594=ORIENTED_EDGE('',*,*,#9583,.T.);
#13595=ORIENTED_EDGE('',*,*,#8295,.F.);
#13596=ORIENTED_EDGE('',*,*,#9582,.T.);
#13597=ORIENTED_EDGE('',*,*,#8266,.F.);
#13598=ORIENTED_EDGE('',*,*,#9585,.F.);
#13599=ORIENTED_EDGE('',*,*,#9586,.T.);
#13600=ORIENTED_EDGE('',*,*,#9587,.T.);
#13601=ORIENTED_EDGE('',*,*,#9586,.F.);
#13602=ORIENTED_EDGE('',*,*,#9588,.F.);
#13603=ORIENTED_EDGE('',*,*,#9589,.T.);
#13604=ORIENTED_EDGE('',*,*,#9590,.T.);
#13605=ORIENTED_EDGE('',*,*,#9589,.F.);
#13606=ORIENTED_EDGE('',*,*,#9462,.T.);
#13607=ORIENTED_EDGE('',*,*,#9374,.T.);
#13608=ORIENTED_EDGE('',*,*,#9457,.T.);
#13609=ORIENTED_EDGE('',*,*,#9455,.T.);
#13610=ORIENTED_EDGE('',*,*,#9454,.T.);
#13611=ORIENTED_EDGE('',*,*,#9470,.T.);
#13612=ORIENTED_EDGE('',*,*,#9348,.T.);
#13613=ORIENTED_EDGE('',*,*,#9465,.T.);
#13614=ORIENTED_EDGE('',*,*,#9428,.T.);
#13615=ORIENTED_EDGE('',*,*,#9427,.T.);
#13616=ORIENTED_EDGE('',*,*,#9478,.T.);
#13617=ORIENTED_EDGE('',*,*,#9322,.T.);
#13618=ORIENTED_EDGE('',*,*,#9473,.T.);
#13619=ORIENTED_EDGE('',*,*,#9401,.T.);
#13620=ORIENTED_EDGE('',*,*,#9400,.T.);
#13621=ORIENTED_EDGE('',*,*,#9486,.T.);
#13622=ORIENTED_EDGE('',*,*,#9269,.T.);
#13623=ORIENTED_EDGE('',*,*,#9481,.T.);
#13624=ORIENTED_EDGE('',*,*,#9296,.T.);
#13625=ORIENTED_EDGE('',*,*,#9295,.T.);
#13626=ORIENTED_EDGE('',*,*,#9588,.T.);
#13627=ORIENTED_EDGE('',*,*,#9536,.T.);
#13628=ORIENTED_EDGE('',*,*,#8792,.T.);
#13629=ORIENTED_EDGE('',*,*,#9533,.T.);
#13630=ORIENTED_EDGE('',*,*,#8833,.T.);
#13631=ORIENTED_EDGE('',*,*,#9544,.T.);
#13632=ORIENTED_EDGE('',*,*,#8710,.T.);
#13633=ORIENTED_EDGE('',*,*,#9541,.T.);
#13634=ORIENTED_EDGE('',*,*,#8751,.T.);
#13635=ORIENTED_EDGE('',*,*,#9552,.T.);
#13636=ORIENTED_EDGE('',*,*,#8628,.T.);
#13637=ORIENTED_EDGE('',*,*,#9549,.T.);
#13638=ORIENTED_EDGE('',*,*,#8669,.T.);
#13639=ORIENTED_EDGE('',*,*,#9560,.T.);
#13640=ORIENTED_EDGE('',*,*,#8546,.T.);
#13641=ORIENTED_EDGE('',*,*,#9557,.T.);
#13642=ORIENTED_EDGE('',*,*,#8587,.T.);
#13643=ORIENTED_EDGE('',*,*,#9568,.T.);
#13644=ORIENTED_EDGE('',*,*,#8464,.T.);
#13645=ORIENTED_EDGE('',*,*,#9565,.T.);
#13646=ORIENTED_EDGE('',*,*,#8505,.T.);
#13647=ORIENTED_EDGE('',*,*,#9585,.T.);
#13648=ORIENTED_EDGE('',*,*,#9584,.T.);
#13649=ORIENTED_EDGE('',*,*,#8300,.T.);
#13650=ORIENTED_EDGE('',*,*,#9581,.T.);
#13651=ORIENTED_EDGE('',*,*,#8341,.T.);
#13652=ORIENTED_EDGE('',*,*,#9590,.F.);
#13653=ORIENTED_EDGE('',*,*,#9496,.T.);
#13654=ORIENTED_EDGE('',*,*,#9202,.T.);
#13655=ORIENTED_EDGE('',*,*,#9493,.T.);
#13656=ORIENTED_EDGE('',*,*,#9243,.T.);
#13657=ORIENTED_EDGE('',*,*,#9504,.T.);
#13658=ORIENTED_EDGE('',*,*,#9120,.T.);
#13659=ORIENTED_EDGE('',*,*,#9501,.T.);
#13660=ORIENTED_EDGE('',*,*,#9161,.T.);
#13661=ORIENTED_EDGE('',*,*,#9512,.T.);
#13662=ORIENTED_EDGE('',*,*,#9038,.T.);
#13663=ORIENTED_EDGE('',*,*,#9509,.T.);
#13664=ORIENTED_EDGE('',*,*,#9079,.T.);
#13665=ORIENTED_EDGE('',*,*,#9520,.T.);
#13666=ORIENTED_EDGE('',*,*,#8956,.T.);
#13667=ORIENTED_EDGE('',*,*,#9517,.T.);
#13668=ORIENTED_EDGE('',*,*,#8997,.T.);
#13669=ORIENTED_EDGE('',*,*,#9528,.T.);
#13670=ORIENTED_EDGE('',*,*,#8874,.T.);
#13671=ORIENTED_EDGE('',*,*,#9525,.T.);
#13672=ORIENTED_EDGE('',*,*,#8915,.T.);
#13673=ORIENTED_EDGE('',*,*,#9587,.F.);
#13674=ORIENTED_EDGE('',*,*,#9576,.T.);
#13675=ORIENTED_EDGE('',*,*,#8382,.T.);
#13676=ORIENTED_EDGE('',*,*,#9573,.T.);
#13677=ORIENTED_EDGE('',*,*,#8423,.T.);
#16532=CYLINDRICAL_SURFACE('',#18465,1.666);
#16533=CYLINDRICAL_SURFACE('',#18468,1.666);
#16534=CYLINDRICAL_SURFACE('',#18469,1.666);
#16535=CYLINDRICAL_SURFACE('',#18470,1.666);
#16536=CYLINDRICAL_SURFACE('',#18471,1.666);
#16537=CYLINDRICAL_SURFACE('',#18472,1.666);
#16538=CYLINDRICAL_SURFACE('',#18473,1.666);
#16539=CYLINDRICAL_SURFACE('',#18474,1.666);
#16540=CYLINDRICAL_SURFACE('',#18475,1.666);
#16541=CYLINDRICAL_SURFACE('',#18476,1.666);
#16542=CYLINDRICAL_SURFACE('',#18477,1.666);
#16543=CYLINDRICAL_SURFACE('',#18478,1.666);
#16544=CYLINDRICAL_SURFACE('',#18480,2.05475);
#16545=CYLINDRICAL_SURFACE('',#18482,2.05475);
#16546=CYLINDRICAL_SURFACE('',#18483,2.05475);
#16547=CYLINDRICAL_SURFACE('',#18484,2.05475);
#16548=CYLINDRICAL_SURFACE('',#18485,2.05475);
#16549=CYLINDRICAL_SURFACE('',#18486,2.05475);
#16550=CYLINDRICAL_SURFACE('',#18487,2.05475);
#16551=CYLINDRICAL_SURFACE('',#18488,2.05475);
#16552=CYLINDRICAL_SURFACE('',#18489,2.05475);
#16553=CYLINDRICAL_SURFACE('',#18490,2.05475);
#16554=CYLINDRICAL_SURFACE('',#18491,2.05475);
#16555=CYLINDRICAL_SURFACE('',#18492,2.05475);
#16556=CYLINDRICAL_SURFACE('',#18493,2.05475);
#16557=CYLINDRICAL_SURFACE('',#18495,1.666);
#16558=CYLINDRICAL_SURFACE('',#18498,1.666);
#16559=CYLINDRICAL_SURFACE('',#18499,1.666);
#16560=CYLINDRICAL_SURFACE('',#18500,1.666);
#16561=CYLINDRICAL_SURFACE('',#18501,1.666);
#16562=CYLINDRICAL_SURFACE('',#18502,1.666);
#16563=CYLINDRICAL_SURFACE('',#18503,1.666);
#16564=CYLINDRICAL_SURFACE('',#18504,1.666);
#16565=CYLINDRICAL_SURFACE('',#18505,1.666);
#16566=CYLINDRICAL_SURFACE('',#18506,1.666);
#16567=CYLINDRICAL_SURFACE('',#18507,1.666);
#16568=CYLINDRICAL_SURFACE('',#18508,1.666);
#16569=CYLINDRICAL_SURFACE('',#18510,2.05475);
#16570=CYLINDRICAL_SURFACE('',#18512,2.05475);
#16571=CYLINDRICAL_SURFACE('',#18513,2.05475);
#16572=CYLINDRICAL_SURFACE('',#18514,2.05475);
#16573=CYLINDRICAL_SURFACE('',#18515,2.05475);
#16574=CYLINDRICAL_SURFACE('',#18516,2.05475);
#16575=CYLINDRICAL_SURFACE('',#18517,2.05475);
#16576=CYLINDRICAL_SURFACE('',#18518,2.05475);
#16577=CYLINDRICAL_SURFACE('',#18519,2.05475);
#16578=CYLINDRICAL_SURFACE('',#18520,2.05475);
#16579=CYLINDRICAL_SURFACE('',#18521,2.05475);
#16580=CYLINDRICAL_SURFACE('',#18522,2.05475);
#16581=CYLINDRICAL_SURFACE('',#18523,2.05475);
#16582=CYLINDRICAL_SURFACE('',#18525,1.666);
#16583=CYLINDRICAL_SURFACE('',#18528,1.666);
#16584=CYLINDRICAL_SURFACE('',#18529,1.666);
#16585=CYLINDRICAL_SURFACE('',#18530,1.666);
#16586=CYLINDRICAL_SURFACE('',#18531,1.666);
#16587=CYLINDRICAL_SURFACE('',#18532,1.666);
#16588=CYLINDRICAL_SURFACE('',#18533,1.666);
#16589=CYLINDRICAL_SURFACE('',#18534,1.666);
#16590=CYLINDRICAL_SURFACE('',#18535,1.666);
#16591=CYLINDRICAL_SURFACE('',#18536,1.666);
#16592=CYLINDRICAL_SURFACE('',#18537,1.666);
#16593=CYLINDRICAL_SURFACE('',#18538,1.666);
#16594=CYLINDRICAL_SURFACE('',#18540,2.05475);
#16595=CYLINDRICAL_SURFACE('',#18542,2.05475);
#16596=CYLINDRICAL_SURFACE('',#18543,2.05475);
#16597=CYLINDRICAL_SURFACE('',#18544,2.05475);
#16598=CYLINDRICAL_SURFACE('',#18545,2.05475);
#16599=CYLINDRICAL_SURFACE('',#18546,2.05475);
#16600=CYLINDRICAL_SURFACE('',#18547,2.05475);
#16601=CYLINDRICAL_SURFACE('',#18548,2.05475);
#16602=CYLINDRICAL_SURFACE('',#18549,2.05475);
#16603=CYLINDRICAL_SURFACE('',#18550,2.05475);
#16604=CYLINDRICAL_SURFACE('',#18551,2.05475);
#16605=CYLINDRICAL_SURFACE('',#18552,2.05475);
#16606=CYLINDRICAL_SURFACE('',#18553,2.05475);
#16607=CYLINDRICAL_SURFACE('',#18555,1.666);
#16608=CYLINDRICAL_SURFACE('',#18558,1.666);
#16609=CYLINDRICAL_SURFACE('',#18559,1.666);
#16610=CYLINDRICAL_SURFACE('',#18560,1.666);
#16611=CYLINDRICAL_SURFACE('',#18561,1.666);
#16612=CYLINDRICAL_SURFACE('',#18562,1.666);
#16613=CYLINDRICAL_SURFACE('',#18563,1.666);
#16614=CYLINDRICAL_SURFACE('',#18564,1.666);
#16615=CYLINDRICAL_SURFACE('',#18565,1.666);
#16616=CYLINDRICAL_SURFACE('',#18566,1.666);
#16617=CYLINDRICAL_SURFACE('',#18567,1.666);
#16618=CYLINDRICAL_SURFACE('',#18568,1.666);
#16619=CYLINDRICAL_SURFACE('',#18570,2.05474999999998);
#16620=CYLINDRICAL_SURFACE('',#18572,2.05474999999998);
#16621=CYLINDRICAL_SURFACE('',#18573,2.05474999999998);
#16622=CYLINDRICAL_SURFACE('',#18574,2.05474999999998);
#16623=CYLINDRICAL_SURFACE('',#18575,2.05474999999998);
#16624=CYLINDRICAL_SURFACE('',#18576,2.05474999999998);
#16625=CYLINDRICAL_SURFACE('',#18577,2.05474999999998);
#16626=CYLINDRICAL_SURFACE('',#18578,2.05474999999998);
#16627=CYLINDRICAL_SURFACE('',#18579,2.05474999999998);
#16628=CYLINDRICAL_SURFACE('',#18580,2.05474999999998);
#16629=CYLINDRICAL_SURFACE('',#18581,2.05474999999998);
#16630=CYLINDRICAL_SURFACE('',#18582,2.05474999999998);
#16631=CYLINDRICAL_SURFACE('',#18583,2.05474999999998);
#16632=CYLINDRICAL_SURFACE('',#18585,1.666);
#16633=CYLINDRICAL_SURFACE('',#18588,1.666);
#16634=CYLINDRICAL_SURFACE('',#18589,1.666);
#16635=CYLINDRICAL_SURFACE('',#18590,1.666);
#16636=CYLINDRICAL_SURFACE('',#18591,1.666);
#16637=CYLINDRICAL_SURFACE('',#18592,1.666);
#16638=CYLINDRICAL_SURFACE('',#18593,1.666);
#16639=CYLINDRICAL_SURFACE('',#18594,1.666);
#16640=CYLINDRICAL_SURFACE('',#18595,1.666);
#16641=CYLINDRICAL_SURFACE('',#18596,1.666);
#16642=CYLINDRICAL_SURFACE('',#18597,1.666);
#16643=CYLINDRICAL_SURFACE('',#18598,1.666);
#16644=CYLINDRICAL_SURFACE('',#18600,2.05475);
#16645=CYLINDRICAL_SURFACE('',#18602,2.05475);
#16646=CYLINDRICAL_SURFACE('',#18603,2.05475);
#16647=CYLINDRICAL_SURFACE('',#18604,2.05475);
#16648=CYLINDRICAL_SURFACE('',#18605,2.05475);
#16649=CYLINDRICAL_SURFACE('',#18606,2.05475);
#16650=CYLINDRICAL_SURFACE('',#18607,2.05475);
#16651=CYLINDRICAL_SURFACE('',#18608,2.05475);
#16652=CYLINDRICAL_SURFACE('',#18609,2.05475);
#16653=CYLINDRICAL_SURFACE('',#18610,2.05475);
#16654=CYLINDRICAL_SURFACE('',#18611,2.05475);
#16655=CYLINDRICAL_SURFACE('',#18612,2.05475);
#16656=CYLINDRICAL_SURFACE('',#18613,2.05475);
#16657=CYLINDRICAL_SURFACE('',#18615,1.666);
#16658=CYLINDRICAL_SURFACE('',#18618,1.666);
#16659=CYLINDRICAL_SURFACE('',#18619,1.666);
#16660=CYLINDRICAL_SURFACE('',#18620,1.666);
#16661=CYLINDRICAL_SURFACE('',#18621,1.666);
#16662=CYLINDRICAL_SURFACE('',#18622,1.666);
#16663=CYLINDRICAL_SURFACE('',#18623,1.666);
#16664=CYLINDRICAL_SURFACE('',#18624,1.666);
#16665=CYLINDRICAL_SURFACE('',#18625,1.666);
#16666=CYLINDRICAL_SURFACE('',#18626,1.666);
#16667=CYLINDRICAL_SURFACE('',#18627,1.666);
#16668=CYLINDRICAL_SURFACE('',#18628,1.666);
#16669=CYLINDRICAL_SURFACE('',#18630,2.05474999999998);
#16670=CYLINDRICAL_SURFACE('',#18632,2.05474999999998);
#16671=CYLINDRICAL_SURFACE('',#18633,2.05474999999998);
#16672=CYLINDRICAL_SURFACE('',#18634,2.05474999999998);
#16673=CYLINDRICAL_SURFACE('',#18635,2.05474999999998);
#16674=CYLINDRICAL_SURFACE('',#18636,2.05474999999998);
#16675=CYLINDRICAL_SURFACE('',#18637,2.05474999999998);
#16676=CYLINDRICAL_SURFACE('',#18638,2.05474999999998);
#16677=CYLINDRICAL_SURFACE('',#18639,2.05474999999998);
#16678=CYLINDRICAL_SURFACE('',#18640,2.05474999999998);
#16679=CYLINDRICAL_SURFACE('',#18641,2.05474999999998);
#16680=CYLINDRICAL_SURFACE('',#18642,2.05474999999998);
#16681=CYLINDRICAL_SURFACE('',#18643,2.05474999999998);
#16682=CYLINDRICAL_SURFACE('',#18645,1.666);
#16683=CYLINDRICAL_SURFACE('',#18648,1.666);
#16684=CYLINDRICAL_SURFACE('',#18649,1.666);
#16685=CYLINDRICAL_SURFACE('',#18650,1.666);
#16686=CYLINDRICAL_SURFACE('',#18651,1.666);
#16687=CYLINDRICAL_SURFACE('',#18652,1.666);
#16688=CYLINDRICAL_SURFACE('',#18653,1.666);
#16689=CYLINDRICAL_SURFACE('',#18654,1.666);
#16690=CYLINDRICAL_SURFACE('',#18655,1.666);
#16691=CYLINDRICAL_SURFACE('',#18656,1.666);
#16692=CYLINDRICAL_SURFACE('',#18657,1.666);
#16693=CYLINDRICAL_SURFACE('',#18658,1.666);
#16694=CYLINDRICAL_SURFACE('',#18660,2.05474999999998);
#16695=CYLINDRICAL_SURFACE('',#18662,2.05474999999998);
#16696=CYLINDRICAL_SURFACE('',#18663,2.05474999999998);
#16697=CYLINDRICAL_SURFACE('',#18664,2.05474999999998);
#16698=CYLINDRICAL_SURFACE('',#18665,2.05474999999998);
#16699=CYLINDRICAL_SURFACE('',#18666,2.05474999999998);
#16700=CYLINDRICAL_SURFACE('',#18667,2.05474999999998);
#16701=CYLINDRICAL_SURFACE('',#18668,2.05474999999998);
#16702=CYLINDRICAL_SURFACE('',#18669,2.05474999999998);
#16703=CYLINDRICAL_SURFACE('',#18670,2.05474999999998);
#16704=CYLINDRICAL_SURFACE('',#18671,2.05474999999998);
#16705=CYLINDRICAL_SURFACE('',#18672,2.05474999999998);
#16706=CYLINDRICAL_SURFACE('',#18673,2.05474999999998);
#16707=CYLINDRICAL_SURFACE('',#18675,1.666);
#16708=CYLINDRICAL_SURFACE('',#18678,1.666);
#16709=CYLINDRICAL_SURFACE('',#18679,1.666);
#16710=CYLINDRICAL_SURFACE('',#18680,1.666);
#16711=CYLINDRICAL_SURFACE('',#18681,1.666);
#16712=CYLINDRICAL_SURFACE('',#18682,1.666);
#16713=CYLINDRICAL_SURFACE('',#18683,1.666);
#16714=CYLINDRICAL_SURFACE('',#18684,1.666);
#16715=CYLINDRICAL_SURFACE('',#18685,1.666);
#16716=CYLINDRICAL_SURFACE('',#18686,1.666);
#16717=CYLINDRICAL_SURFACE('',#18687,1.666);
#16718=CYLINDRICAL_SURFACE('',#18688,1.666);
#16719=CYLINDRICAL_SURFACE('',#18690,2.05475000000002);
#16720=CYLINDRICAL_SURFACE('',#18692,2.05475000000002);
#16721=CYLINDRICAL_SURFACE('',#18693,2.05475000000002);
#16722=CYLINDRICAL_SURFACE('',#18694,2.05475000000002);
#16723=CYLINDRICAL_SURFACE('',#18695,2.05475000000002);
#16724=CYLINDRICAL_SURFACE('',#18696,2.05475000000002);
#16725=CYLINDRICAL_SURFACE('',#18697,2.05475000000002);
#16726=CYLINDRICAL_SURFACE('',#18698,2.05475000000002);
#16727=CYLINDRICAL_SURFACE('',#18699,2.05475000000002);
#16728=CYLINDRICAL_SURFACE('',#18700,2.05475000000002);
#16729=CYLINDRICAL_SURFACE('',#18701,2.05475000000002);
#16730=CYLINDRICAL_SURFACE('',#18702,2.05475000000002);
#16731=CYLINDRICAL_SURFACE('',#18703,2.05475000000002);
#16732=CYLINDRICAL_SURFACE('',#18705,1.666);
#16733=CYLINDRICAL_SURFACE('',#18708,1.666);
#16734=CYLINDRICAL_SURFACE('',#18709,1.666);
#16735=CYLINDRICAL_SURFACE('',#18710,1.666);
#16736=CYLINDRICAL_SURFACE('',#18711,1.666);
#16737=CYLINDRICAL_SURFACE('',#18712,1.666);
#16738=CYLINDRICAL_SURFACE('',#18713,1.666);
#16739=CYLINDRICAL_SURFACE('',#18714,1.666);
#16740=CYLINDRICAL_SURFACE('',#18715,1.666);
#16741=CYLINDRICAL_SURFACE('',#18716,1.666);
#16742=CYLINDRICAL_SURFACE('',#18717,1.666);
#16743=CYLINDRICAL_SURFACE('',#18718,1.666);
#16744=CYLINDRICAL_SURFACE('',#18720,2.05474999999998);
#16745=CYLINDRICAL_SURFACE('',#18722,2.05474999999998);
#16746=CYLINDRICAL_SURFACE('',#18723,2.05474999999998);
#16747=CYLINDRICAL_SURFACE('',#18724,2.05474999999998);
#16748=CYLINDRICAL_SURFACE('',#18725,2.05474999999998);
#16749=CYLINDRICAL_SURFACE('',#18726,2.05474999999998);
#16750=CYLINDRICAL_SURFACE('',#18727,2.05474999999998);
#16751=CYLINDRICAL_SURFACE('',#18728,2.05474999999998);
#16752=CYLINDRICAL_SURFACE('',#18729,2.05474999999998);
#16753=CYLINDRICAL_SURFACE('',#18730,2.05474999999998);
#16754=CYLINDRICAL_SURFACE('',#18731,2.05474999999998);
#16755=CYLINDRICAL_SURFACE('',#18732,2.05474999999998);
#16756=CYLINDRICAL_SURFACE('',#18733,2.05474999999998);
#16757=CYLINDRICAL_SURFACE('',#18735,1.666);
#16758=CYLINDRICAL_SURFACE('',#18738,1.666);
#16759=CYLINDRICAL_SURFACE('',#18739,1.666);
#16760=CYLINDRICAL_SURFACE('',#18740,1.666);
#16761=CYLINDRICAL_SURFACE('',#18741,1.666);
#16762=CYLINDRICAL_SURFACE('',#18742,1.666);
#16763=CYLINDRICAL_SURFACE('',#18743,1.666);
#16764=CYLINDRICAL_SURFACE('',#18744,1.666);
#16765=CYLINDRICAL_SURFACE('',#18745,1.666);
#16766=CYLINDRICAL_SURFACE('',#18746,1.666);
#16767=CYLINDRICAL_SURFACE('',#18747,1.666);
#16768=CYLINDRICAL_SURFACE('',#18748,1.666);
#16769=CYLINDRICAL_SURFACE('',#18750,2.05475);
#16770=CYLINDRICAL_SURFACE('',#18752,2.05475);
#16771=CYLINDRICAL_SURFACE('',#18753,2.05475);
#16772=CYLINDRICAL_SURFACE('',#18754,2.05475);
#16773=CYLINDRICAL_SURFACE('',#18755,2.05475);
#16774=CYLINDRICAL_SURFACE('',#18756,2.05475);
#16775=CYLINDRICAL_SURFACE('',#18757,2.05475);
#16776=CYLINDRICAL_SURFACE('',#18758,2.05475);
#16777=CYLINDRICAL_SURFACE('',#18759,2.05475);
#16778=CYLINDRICAL_SURFACE('',#18760,2.05475);
#16779=CYLINDRICAL_SURFACE('',#18761,2.05475);
#16780=CYLINDRICAL_SURFACE('',#18762,2.05475);
#16781=CYLINDRICAL_SURFACE('',#18763,2.05475);
#16782=CYLINDRICAL_SURFACE('',#18765,1.666);
#16783=CYLINDRICAL_SURFACE('',#18768,1.666);
#16784=CYLINDRICAL_SURFACE('',#18769,1.666);
#16785=CYLINDRICAL_SURFACE('',#18770,1.666);
#16786=CYLINDRICAL_SURFACE('',#18771,1.666);
#16787=CYLINDRICAL_SURFACE('',#18772,1.666);
#16788=CYLINDRICAL_SURFACE('',#18773,1.666);
#16789=CYLINDRICAL_SURFACE('',#18774,1.666);
#16790=CYLINDRICAL_SURFACE('',#18775,1.666);
#16791=CYLINDRICAL_SURFACE('',#18776,1.666);
#16792=CYLINDRICAL_SURFACE('',#18777,1.666);
#16793=CYLINDRICAL_SURFACE('',#18778,1.666);
#16794=CYLINDRICAL_SURFACE('',#18780,2.05474999999999);
#16795=CYLINDRICAL_SURFACE('',#18782,2.05474999999999);
#16796=CYLINDRICAL_SURFACE('',#18783,2.05474999999999);
#16797=CYLINDRICAL_SURFACE('',#18784,2.05474999999999);
#16798=CYLINDRICAL_SURFACE('',#18785,2.05474999999999);
#16799=CYLINDRICAL_SURFACE('',#18786,2.05474999999999);
#16800=CYLINDRICAL_SURFACE('',#18787,2.05474999999999);
#16801=CYLINDRICAL_SURFACE('',#18788,2.05474999999999);
#16802=CYLINDRICAL_SURFACE('',#18789,2.05474999999999);
#16803=CYLINDRICAL_SURFACE('',#18790,2.05474999999999);
#16804=CYLINDRICAL_SURFACE('',#18791,2.05474999999999);
#16805=CYLINDRICAL_SURFACE('',#18792,2.05474999999999);
#16806=CYLINDRICAL_SURFACE('',#18793,2.05474999999999);
#16807=CYLINDRICAL_SURFACE('',#18795,1.666);
#16808=CYLINDRICAL_SURFACE('',#18798,1.666);
#16809=CYLINDRICAL_SURFACE('',#18799,1.666);
#16810=CYLINDRICAL_SURFACE('',#18800,1.666);
#16811=CYLINDRICAL_SURFACE('',#18801,1.666);
#16812=CYLINDRICAL_SURFACE('',#18802,1.666);
#16813=CYLINDRICAL_SURFACE('',#18803,1.666);
#16814=CYLINDRICAL_SURFACE('',#18804,1.666);
#16815=CYLINDRICAL_SURFACE('',#18805,1.666);
#16816=CYLINDRICAL_SURFACE('',#18806,1.666);
#16817=CYLINDRICAL_SURFACE('',#18807,1.666);
#16818=CYLINDRICAL_SURFACE('',#18808,1.666);
#16819=CYLINDRICAL_SURFACE('',#18810,2.05475);
#16820=CYLINDRICAL_SURFACE('',#18812,2.05475);
#16821=CYLINDRICAL_SURFACE('',#18813,2.05475);
#16822=CYLINDRICAL_SURFACE('',#18814,2.05475);
#16823=CYLINDRICAL_SURFACE('',#18815,2.05475);
#16824=CYLINDRICAL_SURFACE('',#18816,2.05475);
#16825=CYLINDRICAL_SURFACE('',#18817,2.05475);
#16826=CYLINDRICAL_SURFACE('',#18818,2.05475);
#16827=CYLINDRICAL_SURFACE('',#18819,2.05475);
#16828=CYLINDRICAL_SURFACE('',#18820,2.05475);
#16829=CYLINDRICAL_SURFACE('',#18821,2.05475);
#16830=CYLINDRICAL_SURFACE('',#18822,2.05475);
#16831=CYLINDRICAL_SURFACE('',#18823,2.05475);
#16832=CYLINDRICAL_SURFACE('',#18825,2.5175);
#16833=CYLINDRICAL_SURFACE('',#18827,2.5175);
#16834=CYLINDRICAL_SURFACE('',#18828,2.5175);
#16835=CYLINDRICAL_SURFACE('',#18829,2.5175);
#16836=CYLINDRICAL_SURFACE('',#18830,2.5175);
#16837=CYLINDRICAL_SURFACE('',#18831,2.5175);
#16838=CYLINDRICAL_SURFACE('',#18832,2.5175);
#16839=CYLINDRICAL_SURFACE('',#18833,2.5175);
#16840=CYLINDRICAL_SURFACE('',#18834,3.07350000000001);
#16841=CYLINDRICAL_SURFACE('',#18836,3.07350000000001);
#16842=CYLINDRICAL_SURFACE('',#18837,3.07350000000001);
#16843=CYLINDRICAL_SURFACE('',#18838,3.07350000000001);
#16844=CYLINDRICAL_SURFACE('',#18839,3.07350000000001);
#16845=CYLINDRICAL_SURFACE('',#18840,3.07350000000001);
#16846=CYLINDRICAL_SURFACE('',#18841,3.07350000000001);
#16847=CYLINDRICAL_SURFACE('',#18842,3.07350000000001);
#16848=CYLINDRICAL_SURFACE('',#18843,2.5175);
#16849=CYLINDRICAL_SURFACE('',#18845,2.5175);
#16850=CYLINDRICAL_SURFACE('',#18846,2.5175);
#16851=CYLINDRICAL_SURFACE('',#18847,2.5175);
#16852=CYLINDRICAL_SURFACE('',#18848,2.5175);
#16853=CYLINDRICAL_SURFACE('',#18849,2.5175);
#16854=CYLINDRICAL_SURFACE('',#18850,2.5175);
#16855=CYLINDRICAL_SURFACE('',#18851,2.5175);
#16856=CYLINDRICAL_SURFACE('',#18852,2.5175);
#16857=CYLINDRICAL_SURFACE('',#18854,2.5175);
#16858=CYLINDRICAL_SURFACE('',#18855,2.5175);
#16859=CYLINDRICAL_SURFACE('',#18856,2.5175);
#16860=CYLINDRICAL_SURFACE('',#18857,2.5175);
#16861=CYLINDRICAL_SURFACE('',#18858,2.5175);
#16862=CYLINDRICAL_SURFACE('',#18859,2.5175);
#16863=CYLINDRICAL_SURFACE('',#18860,2.5175);
#16864=CYLINDRICAL_SURFACE('',#18861,2.5175);
#16865=CYLINDRICAL_SURFACE('',#18863,2.5175);
#16866=CYLINDRICAL_SURFACE('',#18864,2.5175);
#16867=CYLINDRICAL_SURFACE('',#18865,2.5175);
#16868=CYLINDRICAL_SURFACE('',#18866,2.5175);
#16869=CYLINDRICAL_SURFACE('',#18867,2.5175);
#16870=CYLINDRICAL_SURFACE('',#18868,2.5175);
#16871=CYLINDRICAL_SURFACE('',#18869,2.5175);
#16872=CYLINDRICAL_SURFACE('',#18870,3.07350000000001);
#16873=CYLINDRICAL_SURFACE('',#18872,3.07350000000001);
#16874=CYLINDRICAL_SURFACE('',#18873,3.07350000000001);
#16875=CYLINDRICAL_SURFACE('',#18874,3.07350000000001);
#16876=CYLINDRICAL_SURFACE('',#18875,3.07350000000001);
#16877=CYLINDRICAL_SURFACE('',#18876,3.07350000000001);
#16878=CYLINDRICAL_SURFACE('',#18877,3.07350000000001);
#16879=CYLINDRICAL_SURFACE('',#18878,3.07350000000001);
#16880=CYLINDRICAL_SURFACE('',#18879,3.0735);
#16881=CYLINDRICAL_SURFACE('',#18881,3.0735);
#16882=CYLINDRICAL_SURFACE('',#18882,3.0735);
#16883=CYLINDRICAL_SURFACE('',#18883,3.0735);
#16884=CYLINDRICAL_SURFACE('',#18884,3.0735);
#16885=CYLINDRICAL_SURFACE('',#18885,3.0735);
#16886=CYLINDRICAL_SURFACE('',#18886,3.0735);
#16887=CYLINDRICAL_SURFACE('',#18887,3.0735);
#16888=CYLINDRICAL_SURFACE('',#18888,3.0735);
#16889=CYLINDRICAL_SURFACE('',#18890,3.0735);
#16890=CYLINDRICAL_SURFACE('',#18891,3.0735);
#16891=CYLINDRICAL_SURFACE('',#18892,3.0735);
#16892=CYLINDRICAL_SURFACE('',#18893,3.0735);
#16893=CYLINDRICAL_SURFACE('',#18894,3.0735);
#16894=CYLINDRICAL_SURFACE('',#18895,3.0735);
#16895=CYLINDRICAL_SURFACE('',#18896,3.0735);
#16896=CYLINDRICAL_SURFACE('',#18897,3.0735);
#16897=CYLINDRICAL_SURFACE('',#18898,3.0735);
#16898=CYLINDRICAL_SURFACE('',#18899,3.07350000000001);
#16899=CYLINDRICAL_SURFACE('',#18900,2.5175);
#16900=CYLINDRICAL_SURFACE('',#18902,2.5175);
#16901=CYLINDRICAL_SURFACE('',#18904,2.5175);
#16902=CYLINDRICAL_SURFACE('',#18906,3.07350000000001);
#16903=CYLINDRICAL_SURFACE('',#18907,2.5175);
#16904=CYLINDRICAL_SURFACE('',#18910,2.05475);
#16905=CYLINDRICAL_SURFACE('',#18911,1.666);
#16906=CYLINDRICAL_SURFACE('',#18913,2.05474999999999);
#16907=CYLINDRICAL_SURFACE('',#18914,1.666);
#16908=CYLINDRICAL_SURFACE('',#18916,2.05475);
#16909=CYLINDRICAL_SURFACE('',#18917,1.666);
#16910=CYLINDRICAL_SURFACE('',#18919,2.05474999999998);
#16911=CYLINDRICAL_SURFACE('',#18920,1.666);
#16912=CYLINDRICAL_SURFACE('',#18922,2.05475000000002);
#16913=CYLINDRICAL_SURFACE('',#18923,1.666);
#16914=CYLINDRICAL_SURFACE('',#18930,2.05474999999998);
#16915=CYLINDRICAL_SURFACE('',#18931,1.666);
#16916=CYLINDRICAL_SURFACE('',#18933,2.05474999999998);
#16917=CYLINDRICAL_SURFACE('',#18934,1.666);
#16918=CYLINDRICAL_SURFACE('',#18936,2.05475);
#16919=CYLINDRICAL_SURFACE('',#18937,1.666);
#16920=CYLINDRICAL_SURFACE('',#18939,2.05474999999998);
#16921=CYLINDRICAL_SURFACE('',#18940,1.666);
#16922=CYLINDRICAL_SURFACE('',#18942,2.05475);
#16923=CYLINDRICAL_SURFACE('',#18943,1.666);
#16924=CYLINDRICAL_SURFACE('',#18950,2.05475);
#16925=CYLINDRICAL_SURFACE('',#18951,1.666);
#16926=CYLINDRICAL_SURFACE('',#18954,2.05475);
#16927=CYLINDRICAL_SURFACE('',#18955,1.666);
#16928=CYLINDRICAL_SURFACE('',#18957,60.);
#16929=CYLINDRICAL_SURFACE('',#18960,70.);
#17273=ADVANCED_FACE('',(#675),#16532,.F.);
#17274=ADVANCED_FACE('',(#676),#16533,.F.);
#17275=ADVANCED_FACE('',(#677),#16534,.F.);
#17276=ADVANCED_FACE('',(#678),#16535,.F.);
#17277=ADVANCED_FACE('',(#679),#16536,.F.);
#17278=ADVANCED_FACE('',(#680),#16537,.F.);
#17279=ADVANCED_FACE('',(#681),#16538,.F.);
#17280=ADVANCED_FACE('',(#682),#16539,.F.);
#17281=ADVANCED_FACE('',(#683),#16540,.F.);
#17282=ADVANCED_FACE('',(#684),#16541,.F.);
#17283=ADVANCED_FACE('',(#685),#16542,.F.);
#17284=ADVANCED_FACE('',(#686),#16543,.F.);
#17285=ADVANCED_FACE('',(#687),#16544,.F.);
#17286=ADVANCED_FACE('',(#688),#16545,.F.);
#17287=ADVANCED_FACE('',(#689),#16546,.F.);
#17288=ADVANCED_FACE('',(#690),#16547,.F.);
#17289=ADVANCED_FACE('',(#691),#16548,.F.);
#17290=ADVANCED_FACE('',(#692),#16549,.F.);
#17291=ADVANCED_FACE('',(#693),#16550,.F.);
#17292=ADVANCED_FACE('',(#694),#16551,.F.);
#17293=ADVANCED_FACE('',(#695),#16552,.F.);
#17294=ADVANCED_FACE('',(#696),#16553,.F.);
#17295=ADVANCED_FACE('',(#697),#16554,.F.);
#17296=ADVANCED_FACE('',(#698),#16555,.F.);
#17297=ADVANCED_FACE('',(#699),#16556,.F.);
#17298=ADVANCED_FACE('',(#700),#16557,.F.);
#17299=ADVANCED_FACE('',(#701),#16558,.F.);
#17300=ADVANCED_FACE('',(#702),#16559,.F.);
#17301=ADVANCED_FACE('',(#703),#16560,.F.);
#17302=ADVANCED_FACE('',(#704),#16561,.F.);
#17303=ADVANCED_FACE('',(#705),#16562,.F.);
#17304=ADVANCED_FACE('',(#706),#16563,.F.);
#17305=ADVANCED_FACE('',(#707),#16564,.F.);
#17306=ADVANCED_FACE('',(#708),#16565,.F.);
#17307=ADVANCED_FACE('',(#709),#16566,.F.);
#17308=ADVANCED_FACE('',(#710),#16567,.F.);
#17309=ADVANCED_FACE('',(#711),#16568,.F.);
#17310=ADVANCED_FACE('',(#712),#16569,.F.);
#17311=ADVANCED_FACE('',(#713),#16570,.F.);
#17312=ADVANCED_FACE('',(#714),#16571,.F.);
#17313=ADVANCED_FACE('',(#715),#16572,.F.);
#17314=ADVANCED_FACE('',(#716),#16573,.F.);
#17315=ADVANCED_FACE('',(#717),#16574,.F.);
#17316=ADVANCED_FACE('',(#718),#16575,.F.);
#17317=ADVANCED_FACE('',(#719),#16576,.F.);
#17318=ADVANCED_FACE('',(#720),#16577,.F.);
#17319=ADVANCED_FACE('',(#721),#16578,.F.);
#17320=ADVANCED_FACE('',(#722),#16579,.F.);
#17321=ADVANCED_FACE('',(#723),#16580,.F.);
#17322=ADVANCED_FACE('',(#724),#16581,.F.);
#17323=ADVANCED_FACE('',(#725),#16582,.F.);
#17324=ADVANCED_FACE('',(#726),#16583,.F.);
#17325=ADVANCED_FACE('',(#727),#16584,.F.);
#17326=ADVANCED_FACE('',(#728),#16585,.F.);
#17327=ADVANCED_FACE('',(#729),#16586,.F.);
#17328=ADVANCED_FACE('',(#730),#16587,.F.);
#17329=ADVANCED_FACE('',(#731),#16588,.F.);
#17330=ADVANCED_FACE('',(#732),#16589,.F.);
#17331=ADVANCED_FACE('',(#733),#16590,.F.);
#17332=ADVANCED_FACE('',(#734),#16591,.F.);
#17333=ADVANCED_FACE('',(#735),#16592,.F.);
#17334=ADVANCED_FACE('',(#736),#16593,.F.);
#17335=ADVANCED_FACE('',(#737),#16594,.F.);
#17336=ADVANCED_FACE('',(#738),#16595,.F.);
#17337=ADVANCED_FACE('',(#739),#16596,.F.);
#17338=ADVANCED_FACE('',(#740),#16597,.F.);
#17339=ADVANCED_FACE('',(#741),#16598,.F.);
#17340=ADVANCED_FACE('',(#742),#16599,.F.);
#17341=ADVANCED_FACE('',(#743),#16600,.F.);
#17342=ADVANCED_FACE('',(#744),#16601,.F.);
#17343=ADVANCED_FACE('',(#745),#16602,.F.);
#17344=ADVANCED_FACE('',(#746),#16603,.F.);
#17345=ADVANCED_FACE('',(#747),#16604,.F.);
#17346=ADVANCED_FACE('',(#748),#16605,.F.);
#17347=ADVANCED_FACE('',(#749),#16606,.F.);
#17348=ADVANCED_FACE('',(#750),#16607,.F.);
#17349=ADVANCED_FACE('',(#751),#16608,.F.);
#17350=ADVANCED_FACE('',(#752),#16609,.F.);
#17351=ADVANCED_FACE('',(#753),#16610,.F.);
#17352=ADVANCED_FACE('',(#754),#16611,.F.);
#17353=ADVANCED_FACE('',(#755),#16612,.F.);
#17354=ADVANCED_FACE('',(#756),#16613,.F.);
#17355=ADVANCED_FACE('',(#757),#16614,.F.);
#17356=ADVANCED_FACE('',(#758),#16615,.F.);
#17357=ADVANCED_FACE('',(#759),#16616,.F.);
#17358=ADVANCED_FACE('',(#760),#16617,.F.);
#17359=ADVANCED_FACE('',(#761),#16618,.F.);
#17360=ADVANCED_FACE('',(#762),#16619,.F.);
#17361=ADVANCED_FACE('',(#763),#16620,.F.);
#17362=ADVANCED_FACE('',(#764),#16621,.F.);
#17363=ADVANCED_FACE('',(#765),#16622,.F.);
#17364=ADVANCED_FACE('',(#766),#16623,.F.);
#17365=ADVANCED_FACE('',(#767),#16624,.F.);
#17366=ADVANCED_FACE('',(#768),#16625,.F.);
#17367=ADVANCED_FACE('',(#769),#16626,.F.);
#17368=ADVANCED_FACE('',(#770),#16627,.F.);
#17369=ADVANCED_FACE('',(#771),#16628,.F.);
#17370=ADVANCED_FACE('',(#772),#16629,.F.);
#17371=ADVANCED_FACE('',(#773),#16630,.F.);
#17372=ADVANCED_FACE('',(#774),#16631,.F.);
#17373=ADVANCED_FACE('',(#775),#16632,.F.);
#17374=ADVANCED_FACE('',(#776),#16633,.F.);
#17375=ADVANCED_FACE('',(#777),#16634,.F.);
#17376=ADVANCED_FACE('',(#778),#16635,.F.);
#17377=ADVANCED_FACE('',(#779),#16636,.F.);
#17378=ADVANCED_FACE('',(#780),#16637,.F.);
#17379=ADVANCED_FACE('',(#781),#16638,.F.);
#17380=ADVANCED_FACE('',(#782),#16639,.F.);
#17381=ADVANCED_FACE('',(#783),#16640,.F.);
#17382=ADVANCED_FACE('',(#784),#16641,.F.);
#17383=ADVANCED_FACE('',(#785),#16642,.F.);
#17384=ADVANCED_FACE('',(#786),#16643,.F.);
#17385=ADVANCED_FACE('',(#787),#16644,.F.);
#17386=ADVANCED_FACE('',(#788),#16645,.F.);
#17387=ADVANCED_FACE('',(#789),#16646,.F.);
#17388=ADVANCED_FACE('',(#790),#16647,.F.);
#17389=ADVANCED_FACE('',(#791),#16648,.F.);
#17390=ADVANCED_FACE('',(#792),#16649,.F.);
#17391=ADVANCED_FACE('',(#793),#16650,.F.);
#17392=ADVANCED_FACE('',(#794),#16651,.F.);
#17393=ADVANCED_FACE('',(#795),#16652,.F.);
#17394=ADVANCED_FACE('',(#796),#16653,.F.);
#17395=ADVANCED_FACE('',(#797),#16654,.F.);
#17396=ADVANCED_FACE('',(#798),#16655,.F.);
#17397=ADVANCED_FACE('',(#799),#16656,.F.);
#17398=ADVANCED_FACE('',(#800),#16657,.F.);
#17399=ADVANCED_FACE('',(#801),#16658,.F.);
#17400=ADVANCED_FACE('',(#802),#16659,.F.);
#17401=ADVANCED_FACE('',(#803),#16660,.F.);
#17402=ADVANCED_FACE('',(#804),#16661,.F.);
#17403=ADVANCED_FACE('',(#805),#16662,.F.);
#17404=ADVANCED_FACE('',(#806),#16663,.F.);
#17405=ADVANCED_FACE('',(#807),#16664,.F.);
#17406=ADVANCED_FACE('',(#808),#16665,.F.);
#17407=ADVANCED_FACE('',(#809),#16666,.F.);
#17408=ADVANCED_FACE('',(#810),#16667,.F.);
#17409=ADVANCED_FACE('',(#811),#16668,.F.);
#17410=ADVANCED_FACE('',(#812),#16669,.F.);
#17411=ADVANCED_FACE('',(#813),#16670,.F.);
#17412=ADVANCED_FACE('',(#814),#16671,.F.);
#17413=ADVANCED_FACE('',(#815),#16672,.F.);
#17414=ADVANCED_FACE('',(#816),#16673,.F.);
#17415=ADVANCED_FACE('',(#817),#16674,.F.);
#17416=ADVANCED_FACE('',(#818),#16675,.F.);
#17417=ADVANCED_FACE('',(#819),#16676,.F.);
#17418=ADVANCED_FACE('',(#820),#16677,.F.);
#17419=ADVANCED_FACE('',(#821),#16678,.F.);
#17420=ADVANCED_FACE('',(#822),#16679,.F.);
#17421=ADVANCED_FACE('',(#823),#16680,.F.);
#17422=ADVANCED_FACE('',(#824),#16681,.F.);
#17423=ADVANCED_FACE('',(#825),#16682,.F.);
#17424=ADVANCED_FACE('',(#826),#16683,.F.);
#17425=ADVANCED_FACE('',(#827),#16684,.F.);
#17426=ADVANCED_FACE('',(#828),#16685,.F.);
#17427=ADVANCED_FACE('',(#829),#16686,.F.);
#17428=ADVANCED_FACE('',(#830),#16687,.F.);
#17429=ADVANCED_FACE('',(#831),#16688,.F.);
#17430=ADVANCED_FACE('',(#832),#16689,.F.);
#17431=ADVANCED_FACE('',(#833),#16690,.F.);
#17432=ADVANCED_FACE('',(#834),#16691,.F.);
#17433=ADVANCED_FACE('',(#835),#16692,.F.);
#17434=ADVANCED_FACE('',(#836),#16693,.F.);
#17435=ADVANCED_FACE('',(#837),#16694,.F.);
#17436=ADVANCED_FACE('',(#838),#16695,.F.);
#17437=ADVANCED_FACE('',(#839),#16696,.F.);
#17438=ADVANCED_FACE('',(#840),#16697,.F.);
#17439=ADVANCED_FACE('',(#841),#16698,.F.);
#17440=ADVANCED_FACE('',(#842),#16699,.F.);
#17441=ADVANCED_FACE('',(#843),#16700,.F.);
#17442=ADVANCED_FACE('',(#844),#16701,.F.);
#17443=ADVANCED_FACE('',(#845),#16702,.F.);
#17444=ADVANCED_FACE('',(#846),#16703,.F.);
#17445=ADVANCED_FACE('',(#847),#16704,.F.);
#17446=ADVANCED_FACE('',(#848),#16705,.F.);
#17447=ADVANCED_FACE('',(#849),#16706,.F.);
#17448=ADVANCED_FACE('',(#850),#16707,.F.);
#17449=ADVANCED_FACE('',(#851),#16708,.F.);
#17450=ADVANCED_FACE('',(#852),#16709,.F.);
#17451=ADVANCED_FACE('',(#853),#16710,.F.);
#17452=ADVANCED_FACE('',(#854),#16711,.F.);
#17453=ADVANCED_FACE('',(#855),#16712,.F.);
#17454=ADVANCED_FACE('',(#856),#16713,.F.);
#17455=ADVANCED_FACE('',(#857),#16714,.F.);
#17456=ADVANCED_FACE('',(#858),#16715,.F.);
#17457=ADVANCED_FACE('',(#859),#16716,.F.);
#17458=ADVANCED_FACE('',(#860),#16717,.F.);
#17459=ADVANCED_FACE('',(#861),#16718,.F.);
#17460=ADVANCED_FACE('',(#862),#16719,.F.);
#17461=ADVANCED_FACE('',(#863),#16720,.F.);
#17462=ADVANCED_FACE('',(#864),#16721,.F.);
#17463=ADVANCED_FACE('',(#865),#16722,.F.);
#17464=ADVANCED_FACE('',(#866),#16723,.F.);
#17465=ADVANCED_FACE('',(#867),#16724,.F.);
#17466=ADVANCED_FACE('',(#868),#16725,.F.);
#17467=ADVANCED_FACE('',(#869),#16726,.F.);
#17468=ADVANCED_FACE('',(#870),#16727,.F.);
#17469=ADVANCED_FACE('',(#871),#16728,.F.);
#17470=ADVANCED_FACE('',(#872),#16729,.F.);
#17471=ADVANCED_FACE('',(#873),#16730,.F.);
#17472=ADVANCED_FACE('',(#874),#16731,.F.);
#17473=ADVANCED_FACE('',(#875),#16732,.F.);
#17474=ADVANCED_FACE('',(#876),#16733,.F.);
#17475=ADVANCED_FACE('',(#877),#16734,.F.);
#17476=ADVANCED_FACE('',(#878),#16735,.F.);
#17477=ADVANCED_FACE('',(#879),#16736,.F.);
#17478=ADVANCED_FACE('',(#880),#16737,.F.);
#17479=ADVANCED_FACE('',(#881),#16738,.F.);
#17480=ADVANCED_FACE('',(#882),#16739,.F.);
#17481=ADVANCED_FACE('',(#883),#16740,.F.);
#17482=ADVANCED_FACE('',(#884),#16741,.F.);
#17483=ADVANCED_FACE('',(#885),#16742,.F.);
#17484=ADVANCED_FACE('',(#886),#16743,.F.);
#17485=ADVANCED_FACE('',(#887),#16744,.F.);
#17486=ADVANCED_FACE('',(#888),#16745,.F.);
#17487=ADVANCED_FACE('',(#889),#16746,.F.);
#17488=ADVANCED_FACE('',(#890),#16747,.F.);
#17489=ADVANCED_FACE('',(#891),#16748,.F.);
#17490=ADVANCED_FACE('',(#892),#16749,.F.);
#17491=ADVANCED_FACE('',(#893),#16750,.F.);
#17492=ADVANCED_FACE('',(#894),#16751,.F.);
#17493=ADVANCED_FACE('',(#895),#16752,.F.);
#17494=ADVANCED_FACE('',(#896),#16753,.F.);
#17495=ADVANCED_FACE('',(#897),#16754,.F.);
#17496=ADVANCED_FACE('',(#898),#16755,.F.);
#17497=ADVANCED_FACE('',(#899),#16756,.F.);
#17498=ADVANCED_FACE('',(#900),#16757,.F.);
#17499=ADVANCED_FACE('',(#901),#16758,.F.);
#17500=ADVANCED_FACE('',(#902),#16759,.F.);
#17501=ADVANCED_FACE('',(#903),#16760,.F.);
#17502=ADVANCED_FACE('',(#904),#16761,.F.);
#17503=ADVANCED_FACE('',(#905),#16762,.F.);
#17504=ADVANCED_FACE('',(#906),#16763,.F.);
#17505=ADVANCED_FACE('',(#907),#16764,.F.);
#17506=ADVANCED_FACE('',(#908),#16765,.F.);
#17507=ADVANCED_FACE('',(#909),#16766,.F.);
#17508=ADVANCED_FACE('',(#910),#16767,.F.);
#17509=ADVANCED_FACE('',(#911),#16768,.F.);
#17510=ADVANCED_FACE('',(#912),#16769,.F.);
#17511=ADVANCED_FACE('',(#913),#16770,.F.);
#17512=ADVANCED_FACE('',(#914),#16771,.F.);
#17513=ADVANCED_FACE('',(#915),#16772,.F.);
#17514=ADVANCED_FACE('',(#916),#16773,.F.);
#17515=ADVANCED_FACE('',(#917),#16774,.F.);
#17516=ADVANCED_FACE('',(#918),#16775,.F.);
#17517=ADVANCED_FACE('',(#919),#16776,.F.);
#17518=ADVANCED_FACE('',(#920),#16777,.F.);
#17519=ADVANCED_FACE('',(#921),#16778,.F.);
#17520=ADVANCED_FACE('',(#922),#16779,.F.);
#17521=ADVANCED_FACE('',(#923),#16780,.F.);
#17522=ADVANCED_FACE('',(#924),#16781,.F.);
#17523=ADVANCED_FACE('',(#925),#16782,.F.);
#17524=ADVANCED_FACE('',(#926),#16783,.F.);
#17525=ADVANCED_FACE('',(#927),#16784,.F.);
#17526=ADVANCED_FACE('',(#928),#16785,.F.);
#17527=ADVANCED_FACE('',(#929),#16786,.F.);
#17528=ADVANCED_FACE('',(#930),#16787,.F.);
#17529=ADVANCED_FACE('',(#931),#16788,.F.);
#17530=ADVANCED_FACE('',(#932),#16789,.F.);
#17531=ADVANCED_FACE('',(#933),#16790,.F.);
#17532=ADVANCED_FACE('',(#934),#16791,.F.);
#17533=ADVANCED_FACE('',(#935),#16792,.F.);
#17534=ADVANCED_FACE('',(#936),#16793,.F.);
#17535=ADVANCED_FACE('',(#937),#16794,.F.);
#17536=ADVANCED_FACE('',(#938),#16795,.F.);
#17537=ADVANCED_FACE('',(#939),#16796,.F.);
#17538=ADVANCED_FACE('',(#940),#16797,.F.);
#17539=ADVANCED_FACE('',(#941),#16798,.F.);
#17540=ADVANCED_FACE('',(#942),#16799,.F.);
#17541=ADVANCED_FACE('',(#943),#16800,.F.);
#17542=ADVANCED_FACE('',(#944),#16801,.F.);
#17543=ADVANCED_FACE('',(#945),#16802,.F.);
#17544=ADVANCED_FACE('',(#946),#16803,.F.);
#17545=ADVANCED_FACE('',(#947),#16804,.F.);
#17546=ADVANCED_FACE('',(#948),#16805,.F.);
#17547=ADVANCED_FACE('',(#949),#16806,.F.);
#17548=ADVANCED_FACE('',(#950),#16807,.F.);
#17549=ADVANCED_FACE('',(#951),#16808,.F.);
#17550=ADVANCED_FACE('',(#952),#16809,.F.);
#17551=ADVANCED_FACE('',(#953),#16810,.F.);
#17552=ADVANCED_FACE('',(#954),#16811,.F.);
#17553=ADVANCED_FACE('',(#955),#16812,.F.);
#17554=ADVANCED_FACE('',(#956),#16813,.F.);
#17555=ADVANCED_FACE('',(#957),#16814,.F.);
#17556=ADVANCED_FACE('',(#958),#16815,.F.);
#17557=ADVANCED_FACE('',(#959),#16816,.F.);
#17558=ADVANCED_FACE('',(#960),#16817,.F.);
#17559=ADVANCED_FACE('',(#961),#16818,.F.);
#17560=ADVANCED_FACE('',(#962),#16819,.F.);
#17561=ADVANCED_FACE('',(#963),#16820,.F.);
#17562=ADVANCED_FACE('',(#964),#16821,.F.);
#17563=ADVANCED_FACE('',(#965),#16822,.F.);
#17564=ADVANCED_FACE('',(#966),#16823,.F.);
#17565=ADVANCED_FACE('',(#967),#16824,.F.);
#17566=ADVANCED_FACE('',(#968),#16825,.F.);
#17567=ADVANCED_FACE('',(#969),#16826,.F.);
#17568=ADVANCED_FACE('',(#970),#16827,.F.);
#17569=ADVANCED_FACE('',(#971),#16828,.F.);
#17570=ADVANCED_FACE('',(#972),#16829,.F.);
#17571=ADVANCED_FACE('',(#973),#16830,.F.);
#17572=ADVANCED_FACE('',(#974),#16831,.F.);
#17573=ADVANCED_FACE('',(#975),#16832,.F.);
#17574=ADVANCED_FACE('',(#976),#16833,.F.);
#17575=ADVANCED_FACE('',(#977),#16834,.F.);
#17576=ADVANCED_FACE('',(#978),#16835,.F.);
#17577=ADVANCED_FACE('',(#979),#16836,.F.);
#17578=ADVANCED_FACE('',(#980),#16837,.F.);
#17579=ADVANCED_FACE('',(#981),#16838,.F.);
#17580=ADVANCED_FACE('',(#982),#16839,.F.);
#17581=ADVANCED_FACE('',(#983),#16840,.F.);
#17582=ADVANCED_FACE('',(#984),#16841,.F.);
#17583=ADVANCED_FACE('',(#985),#16842,.F.);
#17584=ADVANCED_FACE('',(#986),#16843,.F.);
#17585=ADVANCED_FACE('',(#987),#16844,.F.);
#17586=ADVANCED_FACE('',(#988),#16845,.F.);
#17587=ADVANCED_FACE('',(#989),#16846,.F.);
#17588=ADVANCED_FACE('',(#990),#16847,.F.);
#17589=ADVANCED_FACE('',(#991),#16848,.F.);
#17590=ADVANCED_FACE('',(#992),#16849,.F.);
#17591=ADVANCED_FACE('',(#993),#16850,.F.);
#17592=ADVANCED_FACE('',(#994),#16851,.F.);
#17593=ADVANCED_FACE('',(#995),#16852,.F.);
#17594=ADVANCED_FACE('',(#996),#16853,.F.);
#17595=ADVANCED_FACE('',(#997),#16854,.F.);
#17596=ADVANCED_FACE('',(#998),#16855,.F.);
#17597=ADVANCED_FACE('',(#999),#16856,.F.);
#17598=ADVANCED_FACE('',(#1000),#16857,.F.);
#17599=ADVANCED_FACE('',(#1001),#16858,.F.);
#17600=ADVANCED_FACE('',(#1002),#16859,.F.);
#17601=ADVANCED_FACE('',(#1003),#16860,.F.);
#17602=ADVANCED_FACE('',(#1004),#16861,.F.);
#17603=ADVANCED_FACE('',(#1005),#16862,.F.);
#17604=ADVANCED_FACE('',(#1006),#16863,.F.);
#17605=ADVANCED_FACE('',(#1007),#16864,.F.);
#17606=ADVANCED_FACE('',(#1008),#16865,.F.);
#17607=ADVANCED_FACE('',(#1009),#16866,.F.);
#17608=ADVANCED_FACE('',(#1010),#16867,.F.);
#17609=ADVANCED_FACE('',(#1011),#16868,.F.);
#17610=ADVANCED_FACE('',(#1012),#16869,.F.);
#17611=ADVANCED_FACE('',(#1013),#16870,.F.);
#17612=ADVANCED_FACE('',(#1014),#16871,.F.);
#17613=ADVANCED_FACE('',(#1015),#16872,.F.);
#17614=ADVANCED_FACE('',(#1016),#16873,.F.);
#17615=ADVANCED_FACE('',(#1017),#16874,.F.);
#17616=ADVANCED_FACE('',(#1018),#16875,.F.);
#17617=ADVANCED_FACE('',(#1019),#16876,.F.);
#17618=ADVANCED_FACE('',(#1020),#16877,.F.);
#17619=ADVANCED_FACE('',(#1021),#16878,.F.);
#17620=ADVANCED_FACE('',(#1022),#16879,.F.);
#17621=ADVANCED_FACE('',(#1023),#16880,.F.);
#17622=ADVANCED_FACE('',(#1024),#16881,.F.);
#17623=ADVANCED_FACE('',(#1025),#16882,.F.);
#17624=ADVANCED_FACE('',(#1026),#16883,.F.);
#17625=ADVANCED_FACE('',(#1027),#16884,.F.);
#17626=ADVANCED_FACE('',(#1028),#16885,.F.);
#17627=ADVANCED_FACE('',(#1029),#16886,.F.);
#17628=ADVANCED_FACE('',(#1030),#16887,.F.);
#17629=ADVANCED_FACE('',(#1031),#16888,.F.);
#17630=ADVANCED_FACE('',(#1032),#16889,.F.);
#17631=ADVANCED_FACE('',(#1033),#16890,.F.);
#17632=ADVANCED_FACE('',(#1034),#16891,.F.);
#17633=ADVANCED_FACE('',(#1035),#16892,.F.);
#17634=ADVANCED_FACE('',(#1036),#16893,.F.);
#17635=ADVANCED_FACE('',(#1037),#16894,.F.);
#17636=ADVANCED_FACE('',(#1038),#16895,.F.);
#17637=ADVANCED_FACE('',(#1039),#614,.F.);
#17638=ADVANCED_FACE('',(#1040),#16896,.F.);
#17639=ADVANCED_FACE('',(#1041),#615,.F.);
#17640=ADVANCED_FACE('',(#1042),#616,.F.);
#17641=ADVANCED_FACE('',(#1043),#16897,.F.);
#17642=ADVANCED_FACE('',(#1044),#617,.F.);
#17643=ADVANCED_FACE('',(#1045),#618,.F.);
#17644=ADVANCED_FACE('',(#1046),#16898,.F.);
#17645=ADVANCED_FACE('',(#1047),#619,.F.);
#17646=ADVANCED_FACE('',(#1048),#16899,.F.);
#17647=ADVANCED_FACE('',(#1049),#440,.F.);
#17648=ADVANCED_FACE('',(#1050),#16900,.F.);
#17649=ADVANCED_FACE('',(#1051),#441,.F.);
#17650=ADVANCED_FACE('',(#1052),#16901,.F.);
#17651=ADVANCED_FACE('',(#1053),#442,.F.);
#17652=ADVANCED_FACE('',(#1054),#620,.F.);
#17653=ADVANCED_FACE('',(#1055),#16902,.F.);
#17654=ADVANCED_FACE('',(#1056),#621,.F.);
#17655=ADVANCED_FACE('',(#1057),#16903,.F.);
#17656=ADVANCED_FACE('',(#1058),#443,.F.);
#17657=ADVANCED_FACE('',(#1059),#444,.F.);
#17658=ADVANCED_FACE('',(#1060),#16904,.F.);
#17659=ADVANCED_FACE('',(#1061),#622,.F.);
#17660=ADVANCED_FACE('',(#1062),#623,.F.);
#17661=ADVANCED_FACE('',(#1063),#16905,.F.);
#17662=ADVANCED_FACE('',(#1064),#445,.F.);
#17663=ADVANCED_FACE('',(#1065),#16906,.F.);
#17664=ADVANCED_FACE('',(#1066),#624,.F.);
#17665=ADVANCED_FACE('',(#1067),#625,.F.);
#17666=ADVANCED_FACE('',(#1068),#16907,.F.);
#17667=ADVANCED_FACE('',(#1069),#446,.F.);
#17668=ADVANCED_FACE('',(#1070),#16908,.F.);
#17669=ADVANCED_FACE('',(#1071),#626,.F.);
#17670=ADVANCED_FACE('',(#1072),#627,.F.);
#17671=ADVANCED_FACE('',(#1073),#16909,.F.);
#17672=ADVANCED_FACE('',(#1074),#447,.F.);
#17673=ADVANCED_FACE('',(#1075),#16910,.F.);
#17674=ADVANCED_FACE('',(#1076),#628,.F.);
#17675=ADVANCED_FACE('',(#1077),#629,.F.);
#17676=ADVANCED_FACE('',(#1078),#16911,.F.);
#17677=ADVANCED_FACE('',(#1079),#448,.F.);
#17678=ADVANCED_FACE('',(#1080),#16912,.F.);
#17679=ADVANCED_FACE('',(#1081),#630,.F.);
#17680=ADVANCED_FACE('',(#1082),#631,.F.);
#17681=ADVANCED_FACE('',(#1083),#16913,.F.);
#17682=ADVANCED_FACE('',(#1084),#449,.F.);
#17683=ADVANCED_FACE('',(#1085),#450,.F.);
#17684=ADVANCED_FACE('',(#1086),#451,.F.);
#17685=ADVANCED_FACE('',(#1087),#452,.F.);
#17686=ADVANCED_FACE('',(#1088),#453,.F.);
#17687=ADVANCED_FACE('',(#1089),#454,.T.);
#17688=ADVANCED_FACE('',(#1090),#16914,.F.);
#17689=ADVANCED_FACE('',(#1091),#632,.F.);
#17690=ADVANCED_FACE('',(#1092),#633,.F.);
#17691=ADVANCED_FACE('',(#1093),#16915,.F.);
#17692=ADVANCED_FACE('',(#1094),#455,.T.);
#17693=ADVANCED_FACE('',(#1095),#16916,.F.);
#17694=ADVANCED_FACE('',(#1096),#634,.F.);
#17695=ADVANCED_FACE('',(#1097),#635,.F.);
#17696=ADVANCED_FACE('',(#1098),#16917,.F.);
#17697=ADVANCED_FACE('',(#1099),#456,.T.);
#17698=ADVANCED_FACE('',(#1100),#16918,.F.);
#17699=ADVANCED_FACE('',(#1101),#636,.F.);
#17700=ADVANCED_FACE('',(#1102),#637,.F.);
#17701=ADVANCED_FACE('',(#1103),#16919,.F.);
#17702=ADVANCED_FACE('',(#1104),#457,.T.);
#17703=ADVANCED_FACE('',(#1105),#16920,.F.);
#17704=ADVANCED_FACE('',(#1106),#638,.F.);
#17705=ADVANCED_FACE('',(#1107),#639,.F.);
#17706=ADVANCED_FACE('',(#1108),#16921,.F.);
#17707=ADVANCED_FACE('',(#1109),#458,.T.);
#17708=ADVANCED_FACE('',(#1110),#16922,.F.);
#17709=ADVANCED_FACE('',(#1111),#640,.F.);
#17710=ADVANCED_FACE('',(#1112),#641,.F.);
#17711=ADVANCED_FACE('',(#1113),#16923,.F.);
#17712=ADVANCED_FACE('',(#1114),#459,.F.);
#17713=ADVANCED_FACE('',(#1115),#460,.F.);
#17714=ADVANCED_FACE('',(#1116),#461,.F.);
#17715=ADVANCED_FACE('',(#1117),#462,.F.);
#17716=ADVANCED_FACE('',(#1118),#463,.F.);
#17717=ADVANCED_FACE('',(#1119),#464,.F.);
#17718=ADVANCED_FACE('',(#1120),#16924,.F.);
#17719=ADVANCED_FACE('',(#1121),#642,.F.);
#17720=ADVANCED_FACE('',(#1122),#643,.F.);
#17721=ADVANCED_FACE('',(#1123),#16925,.F.);
#17722=ADVANCED_FACE('',(#1124),#465,.F.);
#17723=ADVANCED_FACE('',(#1125),#466,.T.);
#17724=ADVANCED_FACE('',(#1126),#16926,.F.);
#17725=ADVANCED_FACE('',(#1127),#644,.F.);
#17726=ADVANCED_FACE('',(#1128),#645,.F.);
#17727=ADVANCED_FACE('',(#1129),#16927,.F.);
#17728=ADVANCED_FACE('',(#1130),#467,.F.);
#17729=ADVANCED_FACE('',(#1131),#16928,.F.);
#17730=ADVANCED_FACE('',(#1132,#332,#333,#334,#335),#16929,.T.);
#17731=ADVANCED_FACE('',(#1133,#336,#337,#338,#339,#340,#341,#342),#468,
 .T.);
#17732=ADVANCED_FACE('',(#1134,#343,#344,#345,#346,#347,#348,#349),#469,
 .F.);
#18270=CLOSED_SHELL('',(#17273,#17274,#17275,#17276,#17277,#17278,#17279,
#17280,#17281,#17282,#17283,#17284,#17285,#17286,#17287,#17288,#17289,#17290,
#17291,#17292,#17293,#17294,#17295,#17296,#17297,#17298,#17299,#17300,#17301,
#17302,#17303,#17304,#17305,#17306,#17307,#17308,#17309,#17310,#17311,#17312,
#17313,#17314,#17315,#17316,#17317,#17318,#17319,#17320,#17321,#17322,#17323,
#17324,#17325,#17326,#17327,#17328,#17329,#17330,#17331,#17332,#17333,#17334,
#17335,#17336,#17337,#17338,#17339,#17340,#17341,#17342,#17343,#17344,#17345,
#17346,#17347,#17348,#17349,#17350,#17351,#17352,#17353,#17354,#17355,#17356,
#17357,#17358,#17359,#17360,#17361,#17362,#17363,#17364,#17365,#17366,#17367,
#17368,#17369,#17370,#17371,#17372,#17373,#17374,#17375,#17376,#17377,#17378,
#17379,#17380,#17381,#17382,#17383,#17384,#17385,#17386,#17387,#17388,#17389,
#17390,#17391,#17392,#17393,#17394,#17395,#17396,#17397,#17398,#17399,#17400,
#17401,#17402,#17403,#17404,#17405,#17406,#17407,#17408,#17409,#17410,#17411,
#17412,#17413,#17414,#17415,#17416,#17417,#17418,#17419,#17420,#17421,#17422,
#17423,#17424,#17425,#17426,#17427,#17428,#17429,#17430,#17431,#17432,#17433,
#17434,#17435,#17436,#17437,#17438,#17439,#17440,#17441,#17442,#17443,#17444,
#17445,#17446,#17447,#17448,#17449,#17450,#17451,#17452,#17453,#17454,#17455,
#17456,#17457,#17458,#17459,#17460,#17461,#17462,#17463,#17464,#17465,#17466,
#17467,#17468,#17469,#17470,#17471,#17472,#17473,#17474,#17475,#17476,#17477,
#17478,#17479,#17480,#17481,#17482,#17483,#17484,#17485,#17486,#17487,#17488,
#17489,#17490,#17491,#17492,#17493,#17494,#17495,#17496,#17497,#17498,#17499,
#17500,#17501,#17502,#17503,#17504,#17505,#17506,#17507,#17508,#17509,#17510,
#17511,#17512,#17513,#17514,#17515,#17516,#17517,#17518,#17519,#17520,#17521,
#17522,#17523,#17524,#17525,#17526,#17527,#17528,#17529,#17530,#17531,#17532,
#17533,#17534,#17535,#17536,#17537,#17538,#17539,#17540,#17541,#17542,#17543,
#17544,#17545,#17546,#17547,#17548,#17549,#17550,#17551,#17552,#17553,#17554,
#17555,#17556,#17557,#17558,#17559,#17560,#17561,#17562,#17563,#17564,#17565,
#17566,#17567,#17568,#17569,#17570,#17571,#17572,#17573,#17574,#17575,#17576,
#17577,#17578,#17579,#17580,#17581,#17582,#17583,#17584,#17585,#17586,#17587,
#17588,#17589,#17590,#17591,#17592,#17593,#17594,#17595,#17596,#17597,#17598,
#17599,#17600,#17601,#17602,#17603,#17604,#17605,#17606,#17607,#17608,#17609,
#17610,#17611,#17612,#17613,#17614,#17615,#17616,#17617,#17618,#17619,#17620,
#17621,#17622,#17623,#17624,#17625,#17626,#17627,#17628,#17629,#17630,#17631,
#17632,#17633,#17634,#17635,#17636,#17637,#17638,#17639,#17640,#17641,#17642,
#17643,#17644,#17645,#17646,#17647,#17648,#17649,#17650,#17651,#17652,#17653,
#17654,#17655,#17656,#17657,#17658,#17659,#17660,#17661,#17662,#17663,#17664,
#17665,#17666,#17667,#17668,#17669,#17670,#17671,#17672,#17673,#17674,#17675,
#17676,#17677,#17678,#17679,#17680,#17681,#17682,#17683,#17684,#17685,#17686,
#17687,#17688,#17689,#17690,#17691,#17692,#17693,#17694,#17695,#17696,#17697,
#17698,#17699,#17700,#17701,#17702,#17703,#17704,#17705,#17706,#17707,#17708,
#17709,#17710,#17711,#17712,#17713,#17714,#17715,#17716,#17717,#17718,#17719,
#17720,#17721,#17722,#17723,#17724,#17725,#17726,#17727,#17728,#17729,#17730,
#17731,#17732));
#18464=AXIS2_PLACEMENT_3D('',#23376,#19801,#19802);
#18465=AXIS2_PLACEMENT_3D('',#23377,#19803,#19804);
#18466=AXIS2_PLACEMENT_3D('',#23405,#19806,#19807);
#18467=AXIS2_PLACEMENT_3D('',#23416,#19809,#19810);
#18468=AXIS2_PLACEMENT_3D('',#23439,#19811,#19812);
#18469=AXIS2_PLACEMENT_3D('',#23490,#19814,#19815);
#18470=AXIS2_PLACEMENT_3D('',#23538,#19817,#19818);
#18471=AXIS2_PLACEMENT_3D('',#23586,#19820,#19821);
#18472=AXIS2_PLACEMENT_3D('',#23637,#19823,#19824);
#18473=AXIS2_PLACEMENT_3D('',#23685,#19826,#19827);
#18474=AXIS2_PLACEMENT_3D('',#23733,#19829,#19830);
#18475=AXIS2_PLACEMENT_3D('',#23784,#19832,#19833);
#18476=AXIS2_PLACEMENT_3D('',#23835,#19835,#19836);
#18477=AXIS2_PLACEMENT_3D('',#23883,#19838,#19839);
#18478=AXIS2_PLACEMENT_3D('',#23934,#19841,#19842);
#18479=AXIS2_PLACEMENT_3D('',#23953,#19844,#19845);
#18480=AXIS2_PLACEMENT_3D('',#23973,#19846,#19847);
#18481=AXIS2_PLACEMENT_3D('',#23986,#19849,#19850);
#18482=AXIS2_PLACEMENT_3D('',#23995,#19851,#19852);
#18483=AXIS2_PLACEMENT_3D('',#24019,#19854,#19855);
#18484=AXIS2_PLACEMENT_3D('',#24044,#19857,#19858);
#18485=AXIS2_PLACEMENT_3D('',#24069,#19860,#19861);
#18486=AXIS2_PLACEMENT_3D('',#24093,#19863,#19864);
#18487=AXIS2_PLACEMENT_3D('',#24118,#19866,#19867);
#18488=AXIS2_PLACEMENT_3D('',#24142,#19869,#19870);
#18489=AXIS2_PLACEMENT_3D('',#24167,#19872,#19873);
#18490=AXIS2_PLACEMENT_3D('',#24191,#19875,#19876);
#18491=AXIS2_PLACEMENT_3D('',#24216,#19878,#19879);
#18492=AXIS2_PLACEMENT_3D('',#24241,#19881,#19882);
#18493=AXIS2_PLACEMENT_3D('',#24265,#19884,#19885);
#18494=AXIS2_PLACEMENT_3D('',#24276,#19887,#19888);
#18495=AXIS2_PLACEMENT_3D('',#24282,#19889,#19890);
#18496=AXIS2_PLACEMENT_3D('',#24310,#19892,#19893);
#18497=AXIS2_PLACEMENT_3D('',#24321,#19895,#19896);
#18498=AXIS2_PLACEMENT_3D('',#24344,#19897,#19898);
#18499=AXIS2_PLACEMENT_3D('',#24395,#19900,#19901);
#18500=AXIS2_PLACEMENT_3D('',#24443,#19903,#19904);
#18501=AXIS2_PLACEMENT_3D('',#24491,#19906,#19907);
#18502=AXIS2_PLACEMENT_3D('',#24542,#19909,#19910);
#18503=AXIS2_PLACEMENT_3D('',#24590,#19912,#19913);
#18504=AXIS2_PLACEMENT_3D('',#24638,#19915,#19916);
#18505=AXIS2_PLACEMENT_3D('',#24689,#19918,#19919);
#18506=AXIS2_PLACEMENT_3D('',#24740,#19921,#19922);
#18507=AXIS2_PLACEMENT_3D('',#24788,#19924,#19925);
#18508=AXIS2_PLACEMENT_3D('',#24839,#19927,#19928);
#18509=AXIS2_PLACEMENT_3D('',#24858,#19930,#19931);
#18510=AXIS2_PLACEMENT_3D('',#24878,#19932,#19933);
#18511=AXIS2_PLACEMENT_3D('',#24891,#19935,#19936);
#18512=AXIS2_PLACEMENT_3D('',#24900,#19937,#19938);
#18513=AXIS2_PLACEMENT_3D('',#24924,#19940,#19941);
#18514=AXIS2_PLACEMENT_3D('',#24949,#19943,#19944);
#18515=AXIS2_PLACEMENT_3D('',#24974,#19946,#19947);
#18516=AXIS2_PLACEMENT_3D('',#24998,#19949,#19950);
#18517=AXIS2_PLACEMENT_3D('',#25023,#19952,#19953);
#18518=AXIS2_PLACEMENT_3D('',#25047,#19955,#19956);
#18519=AXIS2_PLACEMENT_3D('',#25072,#19958,#19959);
#18520=AXIS2_PLACEMENT_3D('',#25096,#19961,#19962);
#18521=AXIS2_PLACEMENT_3D('',#25121,#19964,#19965);
#18522=AXIS2_PLACEMENT_3D('',#25146,#19967,#19968);
#18523=AXIS2_PLACEMENT_3D('',#25170,#19970,#19971);
#18524=AXIS2_PLACEMENT_3D('',#25181,#19973,#19974);
#18525=AXIS2_PLACEMENT_3D('',#25187,#19975,#19976);
#18526=AXIS2_PLACEMENT_3D('',#25215,#19978,#19979);
#18527=AXIS2_PLACEMENT_3D('',#25226,#19981,#19982);
#18528=AXIS2_PLACEMENT_3D('',#25249,#19983,#19984);
#18529=AXIS2_PLACEMENT_3D('',#25300,#19986,#19987);
#18530=AXIS2_PLACEMENT_3D('',#25348,#19989,#19990);
#18531=AXIS2_PLACEMENT_3D('',#25396,#19992,#19993);
#18532=AXIS2_PLACEMENT_3D('',#25447,#19995,#19996);
#18533=AXIS2_PLACEMENT_3D('',#25495,#19998,#19999);
#18534=AXIS2_PLACEMENT_3D('',#25543,#20001,#20002);
#18535=AXIS2_PLACEMENT_3D('',#25594,#20004,#20005);
#18536=AXIS2_PLACEMENT_3D('',#25645,#20007,#20008);
#18537=AXIS2_PLACEMENT_3D('',#25693,#20010,#20011);
#18538=AXIS2_PLACEMENT_3D('',#25744,#20013,#20014);
#18539=AXIS2_PLACEMENT_3D('',#25763,#20016,#20017);
#18540=AXIS2_PLACEMENT_3D('',#25783,#20018,#20019);
#18541=AXIS2_PLACEMENT_3D('',#25796,#20021,#20022);
#18542=AXIS2_PLACEMENT_3D('',#25805,#20023,#20024);
#18543=AXIS2_PLACEMENT_3D('',#25829,#20026,#20027);
#18544=AXIS2_PLACEMENT_3D('',#25854,#20029,#20030);
#18545=AXIS2_PLACEMENT_3D('',#25879,#20032,#20033);
#18546=AXIS2_PLACEMENT_3D('',#25903,#20035,#20036);
#18547=AXIS2_PLACEMENT_3D('',#25928,#20038,#20039);
#18548=AXIS2_PLACEMENT_3D('',#25952,#20041,#20042);
#18549=AXIS2_PLACEMENT_3D('',#25977,#20044,#20045);
#18550=AXIS2_PLACEMENT_3D('',#26001,#20047,#20048);
#18551=AXIS2_PLACEMENT_3D('',#26026,#20050,#20051);
#18552=AXIS2_PLACEMENT_3D('',#26051,#20053,#20054);
#18553=AXIS2_PLACEMENT_3D('',#26075,#20056,#20057);
#18554=AXIS2_PLACEMENT_3D('',#26086,#20059,#20060);
#18555=AXIS2_PLACEMENT_3D('',#26092,#20061,#20062);
#18556=AXIS2_PLACEMENT_3D('',#26120,#20064,#20065);
#18557=AXIS2_PLACEMENT_3D('',#26131,#20067,#20068);
#18558=AXIS2_PLACEMENT_3D('',#26154,#20069,#20070);
#18559=AXIS2_PLACEMENT_3D('',#26205,#20072,#20073);
#18560=AXIS2_PLACEMENT_3D('',#26253,#20075,#20076);
#18561=AXIS2_PLACEMENT_3D('',#26301,#20078,#20079);
#18562=AXIS2_PLACEMENT_3D('',#26352,#20081,#20082);
#18563=AXIS2_PLACEMENT_3D('',#26400,#20084,#20085);
#18564=AXIS2_PLACEMENT_3D('',#26448,#20087,#20088);
#18565=AXIS2_PLACEMENT_3D('',#26499,#20090,#20091);
#18566=AXIS2_PLACEMENT_3D('',#26550,#20093,#20094);
#18567=AXIS2_PLACEMENT_3D('',#26598,#20096,#20097);
#18568=AXIS2_PLACEMENT_3D('',#26649,#20099,#20100);
#18569=AXIS2_PLACEMENT_3D('',#26668,#20102,#20103);
#18570=AXIS2_PLACEMENT_3D('',#26688,#20104,#20105);
#18571=AXIS2_PLACEMENT_3D('',#26701,#20107,#20108);
#18572=AXIS2_PLACEMENT_3D('',#26710,#20109,#20110);
#18573=AXIS2_PLACEMENT_3D('',#26734,#20112,#20113);
#18574=AXIS2_PLACEMENT_3D('',#26759,#20115,#20116);
#18575=AXIS2_PLACEMENT_3D('',#26784,#20118,#20119);
#18576=AXIS2_PLACEMENT_3D('',#26808,#20121,#20122);
#18577=AXIS2_PLACEMENT_3D('',#26833,#20124,#20125);
#18578=AXIS2_PLACEMENT_3D('',#26857,#20127,#20128);
#18579=AXIS2_PLACEMENT_3D('',#26882,#20130,#20131);
#18580=AXIS2_PLACEMENT_3D('',#26906,#20133,#20134);
#18581=AXIS2_PLACEMENT_3D('',#26931,#20136,#20137);
#18582=AXIS2_PLACEMENT_3D('',#26956,#20139,#20140);
#18583=AXIS2_PLACEMENT_3D('',#26980,#20142,#20143);
#18584=AXIS2_PLACEMENT_3D('',#26991,#20145,#20146);
#18585=AXIS2_PLACEMENT_3D('',#26997,#20147,#20148);
#18586=AXIS2_PLACEMENT_3D('',#27025,#20150,#20151);
#18587=AXIS2_PLACEMENT_3D('',#27036,#20153,#20154);
#18588=AXIS2_PLACEMENT_3D('',#27059,#20155,#20156);
#18589=AXIS2_PLACEMENT_3D('',#27110,#20158,#20159);
#18590=AXIS2_PLACEMENT_3D('',#27158,#20161,#20162);
#18591=AXIS2_PLACEMENT_3D('',#27206,#20164,#20165);
#18592=AXIS2_PLACEMENT_3D('',#27257,#20167,#20168);
#18593=AXIS2_PLACEMENT_3D('',#27305,#20170,#20171);
#18594=AXIS2_PLACEMENT_3D('',#27353,#20173,#20174);
#18595=AXIS2_PLACEMENT_3D('',#27404,#20176,#20177);
#18596=AXIS2_PLACEMENT_3D('',#27455,#20179,#20180);
#18597=AXIS2_PLACEMENT_3D('',#27503,#20182,#20183);
#18598=AXIS2_PLACEMENT_3D('',#27554,#20185,#20186);
#18599=AXIS2_PLACEMENT_3D('',#27573,#20188,#20189);
#18600=AXIS2_PLACEMENT_3D('',#27593,#20190,#20191);
#18601=AXIS2_PLACEMENT_3D('',#27606,#20193,#20194);
#18602=AXIS2_PLACEMENT_3D('',#27615,#20195,#20196);
#18603=AXIS2_PLACEMENT_3D('',#27639,#20198,#20199);
#18604=AXIS2_PLACEMENT_3D('',#27664,#20201,#20202);
#18605=AXIS2_PLACEMENT_3D('',#27689,#20204,#20205);
#18606=AXIS2_PLACEMENT_3D('',#27713,#20207,#20208);
#18607=AXIS2_PLACEMENT_3D('',#27738,#20210,#20211);
#18608=AXIS2_PLACEMENT_3D('',#27762,#20213,#20214);
#18609=AXIS2_PLACEMENT_3D('',#27787,#20216,#20217);
#18610=AXIS2_PLACEMENT_3D('',#27811,#20219,#20220);
#18611=AXIS2_PLACEMENT_3D('',#27836,#20222,#20223);
#18612=AXIS2_PLACEMENT_3D('',#27861,#20225,#20226);
#18613=AXIS2_PLACEMENT_3D('',#27885,#20228,#20229);
#18614=AXIS2_PLACEMENT_3D('',#27896,#20231,#20232);
#18615=AXIS2_PLACEMENT_3D('',#27902,#20233,#20234);
#18616=AXIS2_PLACEMENT_3D('',#27930,#20236,#20237);
#18617=AXIS2_PLACEMENT_3D('',#27941,#20239,#20240);
#18618=AXIS2_PLACEMENT_3D('',#27964,#20241,#20242);
#18619=AXIS2_PLACEMENT_3D('',#28015,#20244,#20245);
#18620=AXIS2_PLACEMENT_3D('',#28063,#20247,#20248);
#18621=AXIS2_PLACEMENT_3D('',#28111,#20250,#20251);
#18622=AXIS2_PLACEMENT_3D('',#28162,#20253,#20254);
#18623=AXIS2_PLACEMENT_3D('',#28210,#20256,#20257);
#18624=AXIS2_PLACEMENT_3D('',#28258,#20259,#20260);
#18625=AXIS2_PLACEMENT_3D('',#28309,#20262,#20263);
#18626=AXIS2_PLACEMENT_3D('',#28360,#20265,#20266);
#18627=AXIS2_PLACEMENT_3D('',#28408,#20268,#20269);
#18628=AXIS2_PLACEMENT_3D('',#28459,#20271,#20272);
#18629=AXIS2_PLACEMENT_3D('',#28478,#20274,#20275);
#18630=AXIS2_PLACEMENT_3D('',#28498,#20276,#20277);
#18631=AXIS2_PLACEMENT_3D('',#28511,#20279,#20280);
#18632=AXIS2_PLACEMENT_3D('',#28520,#20281,#20282);
#18633=AXIS2_PLACEMENT_3D('',#28544,#20284,#20285);
#18634=AXIS2_PLACEMENT_3D('',#28569,#20287,#20288);
#18635=AXIS2_PLACEMENT_3D('',#28594,#20290,#20291);
#18636=AXIS2_PLACEMENT_3D('',#28618,#20293,#20294);
#18637=AXIS2_PLACEMENT_3D('',#28643,#20296,#20297);
#18638=AXIS2_PLACEMENT_3D('',#28667,#20299,#20300);
#18639=AXIS2_PLACEMENT_3D('',#28692,#20302,#20303);
#18640=AXIS2_PLACEMENT_3D('',#28716,#20305,#20306);
#18641=AXIS2_PLACEMENT_3D('',#28741,#20308,#20309);
#18642=AXIS2_PLACEMENT_3D('',#28766,#20311,#20312);
#18643=AXIS2_PLACEMENT_3D('',#28790,#20314,#20315);
#18644=AXIS2_PLACEMENT_3D('',#28801,#20317,#20318);
#18645=AXIS2_PLACEMENT_3D('',#28807,#20319,#20320);
#18646=AXIS2_PLACEMENT_3D('',#28835,#20322,#20323);
#18647=AXIS2_PLACEMENT_3D('',#28846,#20325,#20326);
#18648=AXIS2_PLACEMENT_3D('',#28869,#20327,#20328);
#18649=AXIS2_PLACEMENT_3D('',#28920,#20330,#20331);
#18650=AXIS2_PLACEMENT_3D('',#28968,#20333,#20334);
#18651=AXIS2_PLACEMENT_3D('',#29016,#20336,#20337);
#18652=AXIS2_PLACEMENT_3D('',#29067,#20339,#20340);
#18653=AXIS2_PLACEMENT_3D('',#29115,#20342,#20343);
#18654=AXIS2_PLACEMENT_3D('',#29163,#20345,#20346);
#18655=AXIS2_PLACEMENT_3D('',#29214,#20348,#20349);
#18656=AXIS2_PLACEMENT_3D('',#29265,#20351,#20352);
#18657=AXIS2_PLACEMENT_3D('',#29313,#20354,#20355);
#18658=AXIS2_PLACEMENT_3D('',#29364,#20357,#20358);
#18659=AXIS2_PLACEMENT_3D('',#29383,#20360,#20361);
#18660=AXIS2_PLACEMENT_3D('',#29403,#20362,#20363);
#18661=AXIS2_PLACEMENT_3D('',#29416,#20365,#20366);
#18662=AXIS2_PLACEMENT_3D('',#29425,#20367,#20368);
#18663=AXIS2_PLACEMENT_3D('',#29449,#20370,#20371);
#18664=AXIS2_PLACEMENT_3D('',#29474,#20373,#20374);
#18665=AXIS2_PLACEMENT_3D('',#29499,#20376,#20377);
#18666=AXIS2_PLACEMENT_3D('',#29523,#20379,#20380);
#18667=AXIS2_PLACEMENT_3D('',#29548,#20382,#20383);
#18668=AXIS2_PLACEMENT_3D('',#29572,#20385,#20386);
#18669=AXIS2_PLACEMENT_3D('',#29597,#20388,#20389);
#18670=AXIS2_PLACEMENT_3D('',#29621,#20391,#20392);
#18671=AXIS2_PLACEMENT_3D('',#29646,#20394,#20395);
#18672=AXIS2_PLACEMENT_3D('',#29671,#20397,#20398);
#18673=AXIS2_PLACEMENT_3D('',#29695,#20400,#20401);
#18674=AXIS2_PLACEMENT_3D('',#29706,#20403,#20404);
#18675=AXIS2_PLACEMENT_3D('',#29712,#20405,#20406);
#18676=AXIS2_PLACEMENT_3D('',#29740,#20408,#20409);
#18677=AXIS2_PLACEMENT_3D('',#29751,#20411,#20412);
#18678=AXIS2_PLACEMENT_3D('',#29774,#20413,#20414);
#18679=AXIS2_PLACEMENT_3D('',#29825,#20416,#20417);
#18680=AXIS2_PLACEMENT_3D('',#29873,#20419,#20420);
#18681=AXIS2_PLACEMENT_3D('',#29921,#20422,#20423);
#18682=AXIS2_PLACEMENT_3D('',#29972,#20425,#20426);
#18683=AXIS2_PLACEMENT_3D('',#30020,#20428,#20429);
#18684=AXIS2_PLACEMENT_3D('',#30068,#20431,#20432);
#18685=AXIS2_PLACEMENT_3D('',#30119,#20434,#20435);
#18686=AXIS2_PLACEMENT_3D('',#30170,#20437,#20438);
#18687=AXIS2_PLACEMENT_3D('',#30218,#20440,#20441);
#18688=AXIS2_PLACEMENT_3D('',#30269,#20443,#20444);
#18689=AXIS2_PLACEMENT_3D('',#30288,#20446,#20447);
#18690=AXIS2_PLACEMENT_3D('',#30308,#20448,#20449);
#18691=AXIS2_PLACEMENT_3D('',#30321,#20451,#20452);
#18692=AXIS2_PLACEMENT_3D('',#30330,#20453,#20454);
#18693=AXIS2_PLACEMENT_3D('',#30354,#20456,#20457);
#18694=AXIS2_PLACEMENT_3D('',#30379,#20459,#20460);
#18695=AXIS2_PLACEMENT_3D('',#30404,#20462,#20463);
#18696=AXIS2_PLACEMENT_3D('',#30428,#20465,#20466);
#18697=AXIS2_PLACEMENT_3D('',#30453,#20468,#20469);
#18698=AXIS2_PLACEMENT_3D('',#30477,#20471,#20472);
#18699=AXIS2_PLACEMENT_3D('',#30502,#20474,#20475);
#18700=AXIS2_PLACEMENT_3D('',#30526,#20477,#20478);
#18701=AXIS2_PLACEMENT_3D('',#30551,#20480,#20481);
#18702=AXIS2_PLACEMENT_3D('',#30576,#20483,#20484);
#18703=AXIS2_PLACEMENT_3D('',#30600,#20486,#20487);
#18704=AXIS2_PLACEMENT_3D('',#30611,#20489,#20490);
#18705=AXIS2_PLACEMENT_3D('',#30617,#20491,#20492);
#18706=AXIS2_PLACEMENT_3D('',#30645,#20494,#20495);
#18707=AXIS2_PLACEMENT_3D('',#30656,#20497,#20498);
#18708=AXIS2_PLACEMENT_3D('',#30679,#20499,#20500);
#18709=AXIS2_PLACEMENT_3D('',#30730,#20502,#20503);
#18710=AXIS2_PLACEMENT_3D('',#30778,#20505,#20506);
#18711=AXIS2_PLACEMENT_3D('',#30826,#20508,#20509);
#18712=AXIS2_PLACEMENT_3D('',#30877,#20511,#20512);
#18713=AXIS2_PLACEMENT_3D('',#30925,#20514,#20515);
#18714=AXIS2_PLACEMENT_3D('',#30973,#20517,#20518);
#18715=AXIS2_PLACEMENT_3D('',#31024,#20520,#20521);
#18716=AXIS2_PLACEMENT_3D('',#31075,#20523,#20524);
#18717=AXIS2_PLACEMENT_3D('',#31123,#20526,#20527);
#18718=AXIS2_PLACEMENT_3D('',#31174,#20529,#20530);
#18719=AXIS2_PLACEMENT_3D('',#31193,#20532,#20533);
#18720=AXIS2_PLACEMENT_3D('',#31213,#20534,#20535);
#18721=AXIS2_PLACEMENT_3D('',#31226,#20537,#20538);
#18722=AXIS2_PLACEMENT_3D('',#31235,#20539,#20540);
#18723=AXIS2_PLACEMENT_3D('',#31259,#20542,#20543);
#18724=AXIS2_PLACEMENT_3D('',#31284,#20545,#20546);
#18725=AXIS2_PLACEMENT_3D('',#31309,#20548,#20549);
#18726=AXIS2_PLACEMENT_3D('',#31333,#20551,#20552);
#18727=AXIS2_PLACEMENT_3D('',#31358,#20554,#20555);
#18728=AXIS2_PLACEMENT_3D('',#31382,#20557,#20558);
#18729=AXIS2_PLACEMENT_3D('',#31407,#20560,#20561);
#18730=AXIS2_PLACEMENT_3D('',#31431,#20563,#20564);
#18731=AXIS2_PLACEMENT_3D('',#31456,#20566,#20567);
#18732=AXIS2_PLACEMENT_3D('',#31481,#20569,#20570);
#18733=AXIS2_PLACEMENT_3D('',#31505,#20572,#20573);
#18734=AXIS2_PLACEMENT_3D('',#31516,#20575,#20576);
#18735=AXIS2_PLACEMENT_3D('',#31522,#20577,#20578);
#18736=AXIS2_PLACEMENT_3D('',#31550,#20580,#20581);
#18737=AXIS2_PLACEMENT_3D('',#31561,#20583,#20584);
#18738=AXIS2_PLACEMENT_3D('',#31584,#20585,#20586);
#18739=AXIS2_PLACEMENT_3D('',#31635,#20588,#20589);
#18740=AXIS2_PLACEMENT_3D('',#31683,#20591,#20592);
#18741=AXIS2_PLACEMENT_3D('',#31731,#20594,#20595);
#18742=AXIS2_PLACEMENT_3D('',#31782,#20597,#20598);
#18743=AXIS2_PLACEMENT_3D('',#31830,#20600,#20601);
#18744=AXIS2_PLACEMENT_3D('',#31878,#20603,#20604);
#18745=AXIS2_PLACEMENT_3D('',#31929,#20606,#20607);
#18746=AXIS2_PLACEMENT_3D('',#31980,#20609,#20610);
#18747=AXIS2_PLACEMENT_3D('',#32028,#20612,#20613);
#18748=AXIS2_PLACEMENT_3D('',#32079,#20615,#20616);
#18749=AXIS2_PLACEMENT_3D('',#32098,#20618,#20619);
#18750=AXIS2_PLACEMENT_3D('',#32118,#20620,#20621);
#18751=AXIS2_PLACEMENT_3D('',#32131,#20623,#20624);
#18752=AXIS2_PLACEMENT_3D('',#32140,#20625,#20626);
#18753=AXIS2_PLACEMENT_3D('',#32164,#20628,#20629);
#18754=AXIS2_PLACEMENT_3D('',#32189,#20631,#20632);
#18755=AXIS2_PLACEMENT_3D('',#32214,#20634,#20635);
#18756=AXIS2_PLACEMENT_3D('',#32238,#20637,#20638);
#18757=AXIS2_PLACEMENT_3D('',#32263,#20640,#20641);
#18758=AXIS2_PLACEMENT_3D('',#32287,#20643,#20644);
#18759=AXIS2_PLACEMENT_3D('',#32312,#20646,#20647);
#18760=AXIS2_PLACEMENT_3D('',#32336,#20649,#20650);
#18761=AXIS2_PLACEMENT_3D('',#32361,#20652,#20653);
#18762=AXIS2_PLACEMENT_3D('',#32386,#20655,#20656);
#18763=AXIS2_PLACEMENT_3D('',#32410,#20658,#20659);
#18764=AXIS2_PLACEMENT_3D('',#32421,#20661,#20662);
#18765=AXIS2_PLACEMENT_3D('',#32427,#20663,#20664);
#18766=AXIS2_PLACEMENT_3D('',#32455,#20666,#20667);
#18767=AXIS2_PLACEMENT_3D('',#32466,#20669,#20670);
#18768=AXIS2_PLACEMENT_3D('',#32489,#20671,#20672);
#18769=AXIS2_PLACEMENT_3D('',#32540,#20674,#20675);
#18770=AXIS2_PLACEMENT_3D('',#32588,#20677,#20678);
#18771=AXIS2_PLACEMENT_3D('',#32636,#20680,#20681);
#18772=AXIS2_PLACEMENT_3D('',#32687,#20683,#20684);
#18773=AXIS2_PLACEMENT_3D('',#32735,#20686,#20687);
#18774=AXIS2_PLACEMENT_3D('',#32783,#20689,#20690);
#18775=AXIS2_PLACEMENT_3D('',#32834,#20692,#20693);
#18776=AXIS2_PLACEMENT_3D('',#32885,#20695,#20696);
#18777=AXIS2_PLACEMENT_3D('',#32933,#20698,#20699);
#18778=AXIS2_PLACEMENT_3D('',#32984,#20701,#20702);
#18779=AXIS2_PLACEMENT_3D('',#33003,#20704,#20705);
#18780=AXIS2_PLACEMENT_3D('',#33023,#20706,#20707);
#18781=AXIS2_PLACEMENT_3D('',#33036,#20709,#20710);
#18782=AXIS2_PLACEMENT_3D('',#33045,#20711,#20712);
#18783=AXIS2_PLACEMENT_3D('',#33069,#20714,#20715);
#18784=AXIS2_PLACEMENT_3D('',#33094,#20717,#20718);
#18785=AXIS2_PLACEMENT_3D('',#33119,#20720,#20721);
#18786=AXIS2_PLACEMENT_3D('',#33143,#20723,#20724);
#18787=AXIS2_PLACEMENT_3D('',#33168,#20726,#20727);
#18788=AXIS2_PLACEMENT_3D('',#33192,#20729,#20730);
#18789=AXIS2_PLACEMENT_3D('',#33217,#20732,#20733);
#18790=AXIS2_PLACEMENT_3D('',#33241,#20735,#20736);
#18791=AXIS2_PLACEMENT_3D('',#33266,#20738,#20739);
#18792=AXIS2_PLACEMENT_3D('',#33291,#20741,#20742);
#18793=AXIS2_PLACEMENT_3D('',#33315,#20744,#20745);
#18794=AXIS2_PLACEMENT_3D('',#33326,#20747,#20748);
#18795=AXIS2_PLACEMENT_3D('',#33332,#20749,#20750);
#18796=AXIS2_PLACEMENT_3D('',#33360,#20752,#20753);
#18797=AXIS2_PLACEMENT_3D('',#33371,#20755,#20756);
#18798=AXIS2_PLACEMENT_3D('',#33394,#20757,#20758);
#18799=AXIS2_PLACEMENT_3D('',#33445,#20760,#20761);
#18800=AXIS2_PLACEMENT_3D('',#33493,#20763,#20764);
#18801=AXIS2_PLACEMENT_3D('',#33541,#20766,#20767);
#18802=AXIS2_PLACEMENT_3D('',#33592,#20769,#20770);
#18803=AXIS2_PLACEMENT_3D('',#33640,#20772,#20773);
#18804=AXIS2_PLACEMENT_3D('',#33688,#20775,#20776);
#18805=AXIS2_PLACEMENT_3D('',#33739,#20778,#20779);
#18806=AXIS2_PLACEMENT_3D('',#33790,#20781,#20782);
#18807=AXIS2_PLACEMENT_3D('',#33838,#20784,#20785);
#18808=AXIS2_PLACEMENT_3D('',#33889,#20787,#20788);
#18809=AXIS2_PLACEMENT_3D('',#33908,#20790,#20791);
#18810=AXIS2_PLACEMENT_3D('',#33928,#20792,#20793);
#18811=AXIS2_PLACEMENT_3D('',#33941,#20795,#20796);
#18812=AXIS2_PLACEMENT_3D('',#33950,#20797,#20798);
#18813=AXIS2_PLACEMENT_3D('',#33974,#20800,#20801);
#18814=AXIS2_PLACEMENT_3D('',#33999,#20803,#20804);
#18815=AXIS2_PLACEMENT_3D('',#34024,#20806,#20807);
#18816=AXIS2_PLACEMENT_3D('',#34048,#20809,#20810);
#18817=AXIS2_PLACEMENT_3D('',#34073,#20812,#20813);
#18818=AXIS2_PLACEMENT_3D('',#34097,#20815,#20816);
#18819=AXIS2_PLACEMENT_3D('',#34122,#20818,#20819);
#18820=AXIS2_PLACEMENT_3D('',#34146,#20821,#20822);
#18821=AXIS2_PLACEMENT_3D('',#34171,#20824,#20825);
#18822=AXIS2_PLACEMENT_3D('',#34196,#20827,#20828);
#18823=AXIS2_PLACEMENT_3D('',#34220,#20830,#20831);
#18824=AXIS2_PLACEMENT_3D('',#34231,#20833,#20834);
#18825=AXIS2_PLACEMENT_3D('',#34237,#20835,#20836);
#18826=AXIS2_PLACEMENT_3D('',#34247,#20838,#20839);
#18827=AXIS2_PLACEMENT_3D('',#34258,#20840,#20841);
#18828=AXIS2_PLACEMENT_3D('',#34309,#20843,#20844);
#18829=AXIS2_PLACEMENT_3D('',#34360,#20846,#20847);
#18830=AXIS2_PLACEMENT_3D('',#34408,#20849,#20850);
#18831=AXIS2_PLACEMENT_3D('',#34462,#20852,#20853);
#18832=AXIS2_PLACEMENT_3D('',#34510,#20855,#20856);
#18833=AXIS2_PLACEMENT_3D('',#34558,#20858,#20859);
#18834=AXIS2_PLACEMENT_3D('',#34608,#20861,#20862);
#18835=AXIS2_PLACEMENT_3D('',#34622,#20864,#20865);
#18836=AXIS2_PLACEMENT_3D('',#34632,#20866,#20867);
#18837=AXIS2_PLACEMENT_3D('',#34656,#20869,#20870);
#18838=AXIS2_PLACEMENT_3D('',#34681,#20872,#20873);
#18839=AXIS2_PLACEMENT_3D('',#34706,#20875,#20876);
#18840=AXIS2_PLACEMENT_3D('',#34731,#20878,#20879);
#18841=AXIS2_PLACEMENT_3D('',#34755,#20881,#20882);
#18842=AXIS2_PLACEMENT_3D('',#34780,#20884,#20885);
#18843=AXIS2_PLACEMENT_3D('',#34806,#20887,#20888);
#18844=AXIS2_PLACEMENT_3D('',#34816,#20890,#20891);
#18845=AXIS2_PLACEMENT_3D('',#34827,#20892,#20893);
#18846=AXIS2_PLACEMENT_3D('',#34878,#20895,#20896);
#18847=AXIS2_PLACEMENT_3D('',#34929,#20898,#20899);
#18848=AXIS2_PLACEMENT_3D('',#34977,#20901,#20902);
#18849=AXIS2_PLACEMENT_3D('',#35031,#20904,#20905);
#18850=AXIS2_PLACEMENT_3D('',#35079,#20907,#20908);
#18851=AXIS2_PLACEMENT_3D('',#35127,#20910,#20911);
#18852=AXIS2_PLACEMENT_3D('',#35177,#20913,#20914);
#18853=AXIS2_PLACEMENT_3D('',#35187,#20916,#20917);
#18854=AXIS2_PLACEMENT_3D('',#35198,#20918,#20919);
#18855=AXIS2_PLACEMENT_3D('',#35249,#20921,#20922);
#18856=AXIS2_PLACEMENT_3D('',#35300,#20924,#20925);
#18857=AXIS2_PLACEMENT_3D('',#35348,#20927,#20928);
#18858=AXIS2_PLACEMENT_3D('',#35402,#20930,#20931);
#18859=AXIS2_PLACEMENT_3D('',#35450,#20933,#20934);
#18860=AXIS2_PLACEMENT_3D('',#35498,#20936,#20937);
#18861=AXIS2_PLACEMENT_3D('',#35548,#20939,#20940);
#18862=AXIS2_PLACEMENT_3D('',#35558,#20942,#20943);
#18863=AXIS2_PLACEMENT_3D('',#35569,#20944,#20945);
#18864=AXIS2_PLACEMENT_3D('',#35620,#20947,#20948);
#18865=AXIS2_PLACEMENT_3D('',#35671,#20950,#20951);
#18866=AXIS2_PLACEMENT_3D('',#35719,#20953,#20954);
#18867=AXIS2_PLACEMENT_3D('',#35773,#20956,#20957);
#18868=AXIS2_PLACEMENT_3D('',#35821,#20959,#20960);
#18869=AXIS2_PLACEMENT_3D('',#35869,#20962,#20963);
#18870=AXIS2_PLACEMENT_3D('',#35919,#20965,#20966);
#18871=AXIS2_PLACEMENT_3D('',#35933,#20968,#20969);
#18872=AXIS2_PLACEMENT_3D('',#35943,#20970,#20971);
#18873=AXIS2_PLACEMENT_3D('',#35967,#20973,#20974);
#18874=AXIS2_PLACEMENT_3D('',#35992,#20976,#20977);
#18875=AXIS2_PLACEMENT_3D('',#36017,#20979,#20980);
#18876=AXIS2_PLACEMENT_3D('',#36042,#20982,#20983);
#18877=AXIS2_PLACEMENT_3D('',#36066,#20985,#20986);
#18878=AXIS2_PLACEMENT_3D('',#36091,#20988,#20989);
#18879=AXIS2_PLACEMENT_3D('',#36117,#20991,#20992);
#18880=AXIS2_PLACEMENT_3D('',#36131,#20994,#20995);
#18881=AXIS2_PLACEMENT_3D('',#36141,#20996,#20997);
#18882=AXIS2_PLACEMENT_3D('',#36165,#20999,#21000);
#18883=AXIS2_PLACEMENT_3D('',#36190,#21002,#21003);
#18884=AXIS2_PLACEMENT_3D('',#36215,#21005,#21006);
#18885=AXIS2_PLACEMENT_3D('',#36240,#21008,#21009);
#18886=AXIS2_PLACEMENT_3D('',#36264,#21011,#21012);
#18887=AXIS2_PLACEMENT_3D('',#36289,#21014,#21015);
#18888=AXIS2_PLACEMENT_3D('',#36315,#21017,#21018);
#18889=AXIS2_PLACEMENT_3D('',#36329,#21020,#21021);
#18890=AXIS2_PLACEMENT_3D('',#36339,#21022,#21023);
#18891=AXIS2_PLACEMENT_3D('',#36363,#21025,#21026);
#18892=AXIS2_PLACEMENT_3D('',#36388,#21028,#21029);
#18893=AXIS2_PLACEMENT_3D('',#36413,#21031,#21032);
#18894=AXIS2_PLACEMENT_3D('',#36438,#21034,#21035);
#18895=AXIS2_PLACEMENT_3D('',#36462,#21037,#21038);
#18896=AXIS2_PLACEMENT_3D('',#36487,#21040,#21041);
#18897=AXIS2_PLACEMENT_3D('',#36879,#21043,#21044);
#18898=AXIS2_PLACEMENT_3D('',#37613,#21045,#21046);
#18899=AXIS2_PLACEMENT_3D('',#38347,#21047,#21048);
#18900=AXIS2_PLACEMENT_3D('',#38715,#21049,#21050);
#18901=AXIS2_PLACEMENT_3D('',#38716,#21051,#21052);
#18902=AXIS2_PLACEMENT_3D('',#38717,#21053,#21054);
#18903=AXIS2_PLACEMENT_3D('',#38718,#21055,#21056);
#18904=AXIS2_PLACEMENT_3D('',#38719,#21057,#21058);
#18905=AXIS2_PLACEMENT_3D('',#38720,#21059,#21060);
#18906=AXIS2_PLACEMENT_3D('',#39087,#21061,#21062);
#18907=AXIS2_PLACEMENT_3D('',#39455,#21063,#21064);
#18908=AXIS2_PLACEMENT_3D('',#39456,#21065,#21066);
#18909=AXIS2_PLACEMENT_3D('',#39457,#21067,#21068);
#18910=AXIS2_PLACEMENT_3D('',#39631,#21069,#21070);
#18911=AXIS2_PLACEMENT_3D('',#40555,#21071,#21072);
#18912=AXIS2_PLACEMENT_3D('',#40556,#21073,#21074);
#18913=AXIS2_PLACEMENT_3D('',#40730,#21075,#21076);
#18914=AXIS2_PLACEMENT_3D('',#41654,#21077,#21078);
#18915=AXIS2_PLACEMENT_3D('',#41655,#21079,#21080);
#18916=AXIS2_PLACEMENT_3D('',#41829,#21081,#21082);
#18917=AXIS2_PLACEMENT_3D('',#42753,#21083,#21084);
#18918=AXIS2_PLACEMENT_3D('',#42754,#21085,#21086);
#18919=AXIS2_PLACEMENT_3D('',#42928,#21087,#21088);
#18920=AXIS2_PLACEMENT_3D('',#43852,#21089,#21090);
#18921=AXIS2_PLACEMENT_3D('',#43853,#21091,#21092);
#18922=AXIS2_PLACEMENT_3D('',#44027,#21093,#21094);
#18923=AXIS2_PLACEMENT_3D('',#44951,#21095,#21096);
#18924=AXIS2_PLACEMENT_3D('',#44952,#21097,#21098);
#18925=AXIS2_PLACEMENT_3D('',#44953,#21099,#21100);
#18926=AXIS2_PLACEMENT_3D('',#44954,#21101,#21102);
#18927=AXIS2_PLACEMENT_3D('',#44955,#21103,#21104);
#18928=AXIS2_PLACEMENT_3D('',#44956,#21105,#21106);
#18929=AXIS2_PLACEMENT_3D('',#44957,#21107,#21108);
#18930=AXIS2_PLACEMENT_3D('',#45131,#21109,#21110);
#18931=AXIS2_PLACEMENT_3D('',#46055,#21111,#21112);
#18932=AXIS2_PLACEMENT_3D('',#46056,#21113,#21114);
#18933=AXIS2_PLACEMENT_3D('',#46230,#21115,#21116);
#18934=AXIS2_PLACEMENT_3D('',#47154,#21117,#21118);
#18935=AXIS2_PLACEMENT_3D('',#47155,#21119,#21120);
#18936=AXIS2_PLACEMENT_3D('',#47329,#21121,#21122);
#18937=AXIS2_PLACEMENT_3D('',#48253,#21123,#21124);
#18938=AXIS2_PLACEMENT_3D('',#48254,#21125,#21126);
#18939=AXIS2_PLACEMENT_3D('',#48428,#21127,#21128);
#18940=AXIS2_PLACEMENT_3D('',#49352,#21129,#21130);
#18941=AXIS2_PLACEMENT_3D('',#49353,#21131,#21132);
#18942=AXIS2_PLACEMENT_3D('',#49527,#21133,#21134);
#18943=AXIS2_PLACEMENT_3D('',#50451,#21135,#21136);
#18944=AXIS2_PLACEMENT_3D('',#50452,#21137,#21138);
#18945=AXIS2_PLACEMENT_3D('',#50453,#21139,#21140);
#18946=AXIS2_PLACEMENT_3D('',#50454,#21141,#21142);
#18947=AXIS2_PLACEMENT_3D('',#50455,#21143,#21144);
#18948=AXIS2_PLACEMENT_3D('',#50456,#21145,#21146);
#18949=AXIS2_PLACEMENT_3D('',#50457,#21147,#21148);
#18950=AXIS2_PLACEMENT_3D('',#50631,#21149,#21150);
#18951=AXIS2_PLACEMENT_3D('',#51555,#21151,#21152);
#18952=AXIS2_PLACEMENT_3D('',#51556,#21153,#21154);
#18953=AXIS2_PLACEMENT_3D('',#51557,#21155,#21156);
#18954=AXIS2_PLACEMENT_3D('',#51731,#21157,#21158);
#18955=AXIS2_PLACEMENT_3D('',#52655,#21159,#21160);
#18956=AXIS2_PLACEMENT_3D('',#52656,#21161,#21162);
#18957=AXIS2_PLACEMENT_3D('',#52657,#21163,#21164);
#18958=AXIS2_PLACEMENT_3D('',#52659,#21165,#21166);
#18959=AXIS2_PLACEMENT_3D('',#52662,#21168,#21169);
#18960=AXIS2_PLACEMENT_3D('',#52663,#21170,#21171);
#18961=AXIS2_PLACEMENT_3D('',#52665,#21172,#21173);
#18962=AXIS2_PLACEMENT_3D('',#52668,#21175,#21176);
#18963=AXIS2_PLACEMENT_3D('',#52669,#21177,#21178);
#18964=AXIS2_PLACEMENT_3D('',#52670,#21179,#21180);
#19801=DIRECTION('axis',(0.,0.,1.));
#19802=DIRECTION('refdir',(1.,0.,0.));
#19803=DIRECTION('center_axis',(0.,0.,-1.));
#19804=DIRECTION('ref_axis',(1.,0.,0.));
#19805=DIRECTION('',(0.,0.,-1.));
#19806=DIRECTION('center_axis',(0.,0.,1.));
#19807=DIRECTION('ref_axis',(1.,0.,0.));
#19808=DIRECTION('',(0.,0.,-1.));
#19809=DIRECTION('center_axis',(0.,0.,1.));
#19810=DIRECTION('ref_axis',(1.,0.,0.));
#19811=DIRECTION('center_axis',(0.,0.,-1.));
#19812=DIRECTION('ref_axis',(1.,0.,0.));
#19813=DIRECTION('',(0.,0.,-1.));
#19814=DIRECTION('center_axis',(0.,0.,-1.));
#19815=DIRECTION('ref_axis',(1.,0.,0.));
#19816=DIRECTION('',(0.,0.,-1.));
#19817=DIRECTION('center_axis',(0.,0.,-1.));
#19818=DIRECTION('ref_axis',(1.,0.,0.));
#19819=DIRECTION('',(0.,0.,-1.));
#19820=DIRECTION('center_axis',(0.,0.,-1.));
#19821=DIRECTION('ref_axis',(1.,0.,0.));
#19822=DIRECTION('',(0.,0.,-1.));
#19823=DIRECTION('center_axis',(0.,0.,-1.));
#19824=DIRECTION('ref_axis',(1.,0.,0.));
#19825=DIRECTION('',(0.,0.,-1.));
#19826=DIRECTION('center_axis',(0.,0.,-1.));
#19827=DIRECTION('ref_axis',(1.,0.,0.));
#19828=DIRECTION('',(0.,0.,-1.));
#19829=DIRECTION('center_axis',(0.,0.,-1.));
#19830=DIRECTION('ref_axis',(1.,0.,0.));
#19831=DIRECTION('',(0.,0.,-1.));
#19832=DIRECTION('center_axis',(0.,0.,-1.));
#19833=DIRECTION('ref_axis',(1.,0.,0.));
#19834=DIRECTION('',(0.,0.,-1.));
#19835=DIRECTION('center_axis',(0.,0.,-1.));
#19836=DIRECTION('ref_axis',(1.,0.,0.));
#19837=DIRECTION('',(0.,0.,-1.));
#19838=DIRECTION('center_axis',(0.,0.,-1.));
#19839=DIRECTION('ref_axis',(1.,0.,0.));
#19840=DIRECTION('',(0.,0.,-1.));
#19841=DIRECTION('center_axis',(0.,0.,-1.));
#19842=DIRECTION('ref_axis',(0.938437885424521,-0.345448020981382,0.));
#19843=DIRECTION('',(0.,0.,-1.));
#19844=DIRECTION('center_axis',(0.,0.,-1.));
#19845=DIRECTION('ref_axis',(1.,0.,0.));
#19846=DIRECTION('center_axis',(0.,0.,-1.));
#19847=DIRECTION('ref_axis',(0.450150052286485,0.892952927329585,0.));
#19848=DIRECTION('',(1.22464679914735E-16,-7.67327966807698E-30,-1.));
#19849=DIRECTION('center_axis',(0.,0.,1.));
#19850=DIRECTION('ref_axis',(1.,-6.25346187617716E-14,0.));
#19851=DIRECTION('center_axis',(0.,0.,-1.));
#19852=DIRECTION('ref_axis',(1.,-6.25346187617716E-14,0.));
#19853=DIRECTION('',(1.22464679914735E-16,-7.67327966807698E-30,-1.));
#19854=DIRECTION('center_axis',(0.,0.,-1.));
#19855=DIRECTION('ref_axis',(1.,-6.25346187617716E-14,0.));
#19856=DIRECTION('',(1.22464679914735E-16,-7.67327966807698E-30,-1.));
#19857=DIRECTION('center_axis',(0.,0.,-1.));
#19858=DIRECTION('ref_axis',(1.,-6.25346187617716E-14,0.));
#19859=DIRECTION('',(1.22464679914735E-16,-7.67327966807698E-30,-1.));
#19860=DIRECTION('center_axis',(0.,0.,-1.));
#19861=DIRECTION('ref_axis',(1.,-6.25346187617716E-14,0.));
#19862=DIRECTION('',(1.22464679914735E-16,-7.67327966807698E-30,-1.));
#19863=DIRECTION('center_axis',(0.,0.,-1.));
#19864=DIRECTION('ref_axis',(1.,-6.25346187617716E-14,0.));
#19865=DIRECTION('',(1.22464679914735E-16,-7.67327966807698E-30,-1.));
#19866=DIRECTION('center_axis',(0.,0.,-1.));
#19867=DIRECTION('ref_axis',(1.,-6.25346187617716E-14,0.));
#19868=DIRECTION('',(1.22464679914735E-16,-7.67327966807698E-30,-1.));
#19869=DIRECTION('center_axis',(0.,0.,-1.));
#19870=DIRECTION('ref_axis',(1.,-6.25346187617716E-14,0.));
#19871=DIRECTION('',(1.22464679914735E-16,-7.67327966807698E-30,-1.));
#19872=DIRECTION('center_axis',(0.,0.,-1.));
#19873=DIRECTION('ref_axis',(1.,-6.25346187617716E-14,0.));
#19874=DIRECTION('',(1.22464679914735E-16,-7.67327966807698E-30,-1.));
#19875=DIRECTION('center_axis',(0.,0.,-1.));
#19876=DIRECTION('ref_axis',(1.,-6.25346187617716E-14,0.));
#19877=DIRECTION('',(1.22464679914735E-16,-7.67327966807698E-30,-1.));
#19878=DIRECTION('center_axis',(0.,0.,-1.));
#19879=DIRECTION('ref_axis',(1.,-6.25346187617716E-14,0.));
#19880=DIRECTION('',(1.22464679914735E-16,-7.67327966807698E-30,-1.));
#19881=DIRECTION('center_axis',(0.,0.,-1.));
#19882=DIRECTION('ref_axis',(1.,-6.25346187617716E-14,0.));
#19883=DIRECTION('',(1.22464679914735E-16,-7.67327966807698E-30,-1.));
#19884=DIRECTION('center_axis',(0.,0.,-1.));
#19885=DIRECTION('ref_axis',(-0.609343127961874,-0.792906647976696,0.));
#19886=DIRECTION('',(1.22464679914735E-16,-7.67327966807698E-30,-1.));
#19887=DIRECTION('center_axis',(0.,0.,-1.));
#19888=DIRECTION('ref_axis',(1.,-6.25346187617716E-14,0.));
#19889=DIRECTION('center_axis',(0.,0.,1.));
#19890=DIRECTION('ref_axis',(-1.,0.,0.));
#19891=DIRECTION('',(0.,0.,1.));
#19892=DIRECTION('center_axis',(0.,0.,-1.));
#19893=DIRECTION('ref_axis',(-1.,0.,0.));
#19894=DIRECTION('',(0.,0.,1.));
#19895=DIRECTION('center_axis',(0.,0.,-1.));
#19896=DIRECTION('ref_axis',(-1.,0.,0.));
#19897=DIRECTION('center_axis',(0.,0.,1.));
#19898=DIRECTION('ref_axis',(-1.,0.,0.));
#19899=DIRECTION('',(0.,0.,1.));
#19900=DIRECTION('center_axis',(0.,0.,1.));
#19901=DIRECTION('ref_axis',(-1.,0.,0.));
#19902=DIRECTION('',(0.,0.,1.));
#19903=DIRECTION('center_axis',(0.,0.,1.));
#19904=DIRECTION('ref_axis',(-1.,0.,0.));
#19905=DIRECTION('',(0.,0.,1.));
#19906=DIRECTION('center_axis',(0.,0.,1.));
#19907=DIRECTION('ref_axis',(-1.,0.,0.));
#19908=DIRECTION('',(0.,0.,1.));
#19909=DIRECTION('center_axis',(0.,0.,1.));
#19910=DIRECTION('ref_axis',(-1.,0.,0.));
#19911=DIRECTION('',(0.,0.,1.));
#19912=DIRECTION('center_axis',(0.,0.,1.));
#19913=DIRECTION('ref_axis',(-1.,0.,0.));
#19914=DIRECTION('',(0.,0.,1.));
#19915=DIRECTION('center_axis',(0.,0.,1.));
#19916=DIRECTION('ref_axis',(-1.,0.,0.));
#19917=DIRECTION('',(0.,0.,1.));
#19918=DIRECTION('center_axis',(0.,0.,1.));
#19919=DIRECTION('ref_axis',(-1.,0.,0.));
#19920=DIRECTION('',(0.,0.,1.));
#19921=DIRECTION('center_axis',(0.,0.,1.));
#19922=DIRECTION('ref_axis',(-1.,0.,0.));
#19923=DIRECTION('',(0.,0.,1.));
#19924=DIRECTION('center_axis',(0.,0.,1.));
#19925=DIRECTION('ref_axis',(-1.,0.,0.));
#19926=DIRECTION('',(0.,0.,1.));
#19927=DIRECTION('center_axis',(0.,0.,1.));
#19928=DIRECTION('ref_axis',(-0.938437365767004,-0.345449432670379,0.));
#19929=DIRECTION('',(0.,0.,1.));
#19930=DIRECTION('center_axis',(0.,0.,-1.));
#19931=DIRECTION('ref_axis',(-1.,0.,0.));
#19932=DIRECTION('center_axis',(0.,0.,1.));
#19933=DIRECTION('ref_axis',(-0.450147885469881,0.892954019648825,0.));
#19934=DIRECTION('',(-1.22464679914735E-16,-6.15178233488065E-30,1.));
#19935=DIRECTION('center_axis',(0.,0.,-1.));
#19936=DIRECTION('ref_axis',(-1.,-5.01106501999328E-14,0.));
#19937=DIRECTION('center_axis',(0.,0.,1.));
#19938=DIRECTION('ref_axis',(-1.,-5.01106501999328E-14,0.));
#19939=DIRECTION('',(-1.22464679914735E-16,-6.15178233488065E-30,1.));
#19940=DIRECTION('center_axis',(0.,0.,1.));
#19941=DIRECTION('ref_axis',(-1.,-5.01106501999328E-14,0.));
#19942=DIRECTION('',(-1.22464679914735E-16,-6.15178233488065E-30,1.));
#19943=DIRECTION('center_axis',(0.,0.,1.));
#19944=DIRECTION('ref_axis',(-1.,-5.01106501999328E-14,0.));
#19945=DIRECTION('',(-1.22464679914735E-16,-6.15178233488065E-30,1.));
#19946=DIRECTION('center_axis',(0.,0.,1.));
#19947=DIRECTION('ref_axis',(-1.,-5.01106501999328E-14,0.));
#19948=DIRECTION('',(-1.22464679914735E-16,-6.15178233488065E-30,1.));
#19949=DIRECTION('center_axis',(0.,0.,1.));
#19950=DIRECTION('ref_axis',(-1.,-5.01106501999328E-14,0.));
#19951=DIRECTION('',(-1.22464679914735E-16,-6.15178233488065E-30,1.));
#19952=DIRECTION('center_axis',(0.,0.,1.));
#19953=DIRECTION('ref_axis',(-1.,-5.01106501999328E-14,0.));
#19954=DIRECTION('',(-1.22464679914735E-16,-6.15178233488065E-30,1.));
#19955=DIRECTION('center_axis',(0.,0.,1.));
#19956=DIRECTION('ref_axis',(-1.,-5.01106501999328E-14,0.));
#19957=DIRECTION('',(-1.22464679914735E-16,-6.15178233488065E-30,1.));
#19958=DIRECTION('center_axis',(0.,0.,1.));
#19959=DIRECTION('ref_axis',(-1.,-5.01106501999328E-14,0.));
#19960=DIRECTION('',(-1.22464679914735E-16,-6.15178233488065E-30,1.));
#19961=DIRECTION('center_axis',(0.,0.,1.));
#19962=DIRECTION('ref_axis',(-1.,-5.01106501999328E-14,0.));
#19963=DIRECTION('',(-1.22464679914735E-16,-6.15178233488065E-30,1.));
#19964=DIRECTION('center_axis',(0.,0.,1.));
#19965=DIRECTION('ref_axis',(-1.,-5.01106501999328E-14,0.));
#19966=DIRECTION('',(-1.22464679914735E-16,-6.15178233488065E-30,1.));
#19967=DIRECTION('center_axis',(0.,0.,1.));
#19968=DIRECTION('ref_axis',(-1.,-5.01106501999328E-14,0.));
#19969=DIRECTION('',(-1.22464679914735E-16,-6.15178233488065E-30,1.));
#19970=DIRECTION('center_axis',(0.,0.,1.));
#19971=DIRECTION('ref_axis',(0.609344456561462,-0.792905626955577,0.));
#19972=DIRECTION('',(-1.22464679914735E-16,-6.15178233488065E-30,1.));
#19973=DIRECTION('center_axis',(0.,0.,1.));
#19974=DIRECTION('ref_axis',(-1.,-5.01106501999328E-14,0.));
#19975=DIRECTION('center_axis',(0.,0.,-1.));
#19976=DIRECTION('ref_axis',(0.5,0.866025403784439,0.));
#19977=DIRECTION('',(0.,0.,-1.));
#19978=DIRECTION('center_axis',(0.,0.,1.));
#19979=DIRECTION('ref_axis',(0.5,0.866025403784439,0.));
#19980=DIRECTION('',(0.,0.,-1.));
#19981=DIRECTION('center_axis',(0.,0.,1.));
#19982=DIRECTION('ref_axis',(0.5,0.866025403784439,0.));
#19983=DIRECTION('center_axis',(0.,0.,-1.));
#19984=DIRECTION('ref_axis',(0.5,0.866025403784439,0.));
#19985=DIRECTION('',(0.,0.,-1.));
#19986=DIRECTION('center_axis',(0.,0.,-1.));
#19987=DIRECTION('ref_axis',(0.5,0.866025403784439,0.));
#19988=DIRECTION('',(0.,0.,-1.));
#19989=DIRECTION('center_axis',(0.,0.,-1.));
#19990=DIRECTION('ref_axis',(0.5,0.866025403784439,0.));
#19991=DIRECTION('',(0.,0.,-1.));
#19992=DIRECTION('center_axis',(0.,0.,-1.));
#19993=DIRECTION('ref_axis',(0.5,0.866025403784439,0.));
#19994=DIRECTION('',(0.,0.,-1.));
#19995=DIRECTION('center_axis',(0.,0.,-1.));
#19996=DIRECTION('ref_axis',(0.5,0.866025403784439,0.));
#19997=DIRECTION('',(0.,0.,-1.));
#19998=DIRECTION('center_axis',(0.,0.,-1.));
#19999=DIRECTION('ref_axis',(0.5,0.866025403784439,0.));
#20000=DIRECTION('',(0.,0.,-1.));
#20001=DIRECTION('center_axis',(0.,0.,-1.));
#20002=DIRECTION('ref_axis',(0.5,0.866025403784439,0.));
#20003=DIRECTION('',(0.,0.,-1.));
#20004=DIRECTION('center_axis',(0.,0.,-1.));
#20005=DIRECTION('ref_axis',(0.5,0.866025403784439,0.));
#20006=DIRECTION('',(0.,0.,-1.));
#20007=DIRECTION('center_axis',(0.,0.,-1.));
#20008=DIRECTION('ref_axis',(0.5,0.866025403784439,0.));
#20009=DIRECTION('',(0.,0.,-1.));
#20010=DIRECTION('center_axis',(0.,0.,-1.));
#20011=DIRECTION('ref_axis',(0.5,0.866025403784439,0.));
#20012=DIRECTION('',(0.,0.,-1.));
#20013=DIRECTION('center_axis',(0.,0.,-1.));
#20014=DIRECTION('ref_axis',(0.76838443895182,0.639988557692008,0.));
#20015=DIRECTION('',(0.,0.,-1.));
#20016=DIRECTION('center_axis',(0.,0.,-1.));
#20017=DIRECTION('ref_axis',(0.5,0.866025403784439,0.));
#20018=DIRECTION('center_axis',(0.,0.,-1.));
#20019=DIRECTION('ref_axis',(-0.548242225181982,0.836319593533183,0.));
#20020=DIRECTION('',(6.12323399573741E-17,1.06057523872487E-16,-1.));
#20021=DIRECTION('center_axis',(0.,0.,1.));
#20022=DIRECTION('ref_axis',(0.500000000000052,0.866025403784409,0.));
#20023=DIRECTION('center_axis',(0.,0.,-1.));
#20024=DIRECTION('ref_axis',(0.500000000000052,0.866025403784408,0.));
#20025=DIRECTION('',(6.12323399573741E-17,1.06057523872487E-16,-1.));
#20026=DIRECTION('center_axis',(0.,0.,-1.));
#20027=DIRECTION('ref_axis',(0.500000000000052,0.866025403784408,0.));
#20028=DIRECTION('',(6.12323399573741E-17,1.06057523872487E-16,-1.));
#20029=DIRECTION('center_axis',(0.,0.,-1.));
#20030=DIRECTION('ref_axis',(0.500000000000052,0.866025403784408,0.));
#20031=DIRECTION('',(6.12323399573741E-17,1.06057523872487E-16,-1.));
#20032=DIRECTION('center_axis',(0.,0.,-1.));
#20033=DIRECTION('ref_axis',(0.500000000000052,0.866025403784408,0.));
#20034=DIRECTION('',(6.12323399573741E-17,1.06057523872487E-16,-1.));
#20035=DIRECTION('center_axis',(0.,0.,-1.));
#20036=DIRECTION('ref_axis',(0.500000000000052,0.866025403784408,0.));
#20037=DIRECTION('',(6.12323399573741E-17,1.06057523872487E-16,-1.));
#20038=DIRECTION('center_axis',(0.,0.,-1.));
#20039=DIRECTION('ref_axis',(0.500000000000052,0.866025403784408,0.));
#20040=DIRECTION('',(6.12323399573741E-17,1.06057523872487E-16,-1.));
#20041=DIRECTION('center_axis',(0.,0.,-1.));
#20042=DIRECTION('ref_axis',(0.500000000000052,0.866025403784408,0.));
#20043=DIRECTION('',(6.12323399573741E-17,1.06057523872487E-16,-1.));
#20044=DIRECTION('center_axis',(0.,0.,-1.));
#20045=DIRECTION('ref_axis',(0.500000000000052,0.866025403784408,0.));
#20046=DIRECTION('',(6.12323399573741E-17,1.06057523872487E-16,-1.));
#20047=DIRECTION('center_axis',(0.,0.,-1.));
#20048=DIRECTION('ref_axis',(0.500000000000052,0.866025403784408,0.));
#20049=DIRECTION('',(6.12323399573741E-17,1.06057523872487E-16,-1.));
#20050=DIRECTION('center_axis',(0.,0.,-1.));
#20051=DIRECTION('ref_axis',(0.500000000000052,0.866025403784408,0.));
#20052=DIRECTION('',(6.12323399573741E-17,1.06057523872487E-16,-1.));
#20053=DIRECTION('center_axis',(0.,0.,-1.));
#20054=DIRECTION('ref_axis',(0.500000000000052,0.866025403784408,0.));
#20055=DIRECTION('',(6.12323399573741E-17,1.06057523872487E-16,-1.));
#20056=DIRECTION('center_axis',(0.,0.,-1.));
#20057=DIRECTION('ref_axis',(0.382007546651495,-0.924159203980194,0.));
#20058=DIRECTION('',(6.12323399573741E-17,1.06057523872487E-16,-1.));
#20059=DIRECTION('center_axis',(0.,0.,-1.));
#20060=DIRECTION('ref_axis',(0.500000000000052,0.866025403784409,0.));
#20061=DIRECTION('center_axis',(0.,0.,-1.));
#20062=DIRECTION('ref_axis',(-0.5,0.866025403784439,0.));
#20063=DIRECTION('',(0.,0.,-1.));
#20064=DIRECTION('center_axis',(0.,0.,1.));
#20065=DIRECTION('ref_axis',(-0.5,0.866025403784439,0.));
#20066=DIRECTION('',(0.,0.,-1.));
#20067=DIRECTION('center_axis',(0.,0.,1.));
#20068=DIRECTION('ref_axis',(-0.5,0.866025403784439,0.));
#20069=DIRECTION('center_axis',(0.,0.,-1.));
#20070=DIRECTION('ref_axis',(-0.5,0.866025403784439,0.));
#20071=DIRECTION('',(0.,0.,-1.));
#20072=DIRECTION('center_axis',(0.,0.,-1.));
#20073=DIRECTION('ref_axis',(-0.5,0.866025403784439,0.));
#20074=DIRECTION('',(0.,0.,-1.));
#20075=DIRECTION('center_axis',(0.,0.,-1.));
#20076=DIRECTION('ref_axis',(-0.5,0.866025403784439,0.));
#20077=DIRECTION('',(0.,0.,-1.));
#20078=DIRECTION('center_axis',(0.,0.,-1.));
#20079=DIRECTION('ref_axis',(-0.5,0.866025403784439,0.));
#20080=DIRECTION('',(0.,0.,-1.));
#20081=DIRECTION('center_axis',(0.,0.,-1.));
#20082=DIRECTION('ref_axis',(-0.5,0.866025403784439,0.));
#20083=DIRECTION('',(0.,0.,-1.));
#20084=DIRECTION('center_axis',(0.,0.,-1.));
#20085=DIRECTION('ref_axis',(-0.5,0.866025403784439,0.));
#20086=DIRECTION('',(0.,0.,-1.));
#20087=DIRECTION('center_axis',(0.,0.,-1.));
#20088=DIRECTION('ref_axis',(-0.5,0.866025403784439,0.));
#20089=DIRECTION('',(0.,0.,-1.));
#20090=DIRECTION('center_axis',(0.,0.,-1.));
#20091=DIRECTION('ref_axis',(-0.5,0.866025403784439,0.));
#20092=DIRECTION('',(0.,0.,-1.));
#20093=DIRECTION('center_axis',(0.,0.,-1.));
#20094=DIRECTION('ref_axis',(-0.5,0.866025403784439,0.));
#20095=DIRECTION('',(0.,0.,-1.));
#20096=DIRECTION('center_axis',(0.,0.,-1.));
#20097=DIRECTION('ref_axis',(-0.5,0.866025403784439,0.));
#20098=DIRECTION('',(0.,0.,-1.));
#20099=DIRECTION('center_axis',(0.,0.,-1.));
#20100=DIRECTION('ref_axis',(-0.170054135023851,0.98543472191784,0.));
#20101=DIRECTION('',(0.,0.,-1.));
#20102=DIRECTION('center_axis',(0.,0.,-1.));
#20103=DIRECTION('ref_axis',(-0.5,0.866025403784439,0.));
#20104=DIRECTION('center_axis',(0.,0.,-1.));
#20105=DIRECTION('ref_axis',(-0.998395126723898,-0.0566318897262918,0.));
#20106=DIRECTION('',(-6.12323399573607E-17,1.06057523872495E-16,-1.));
#20107=DIRECTION('center_axis',(0.,0.,1.));
#20108=DIRECTION('ref_axis',(-0.499999999999944,0.866025403784471,0.));
#20109=DIRECTION('center_axis',(0.,0.,-1.));
#20110=DIRECTION('ref_axis',(-0.499999999999944,0.866025403784471,0.));
#20111=DIRECTION('',(-6.12323399573607E-17,1.06057523872495E-16,-1.));
#20112=DIRECTION('center_axis',(0.,0.,-1.));
#20113=DIRECTION('ref_axis',(-0.499999999999944,0.866025403784471,0.));
#20114=DIRECTION('',(-6.12323399573607E-17,1.06057523872495E-16,-1.));
#20115=DIRECTION('center_axis',(0.,0.,-1.));
#20116=DIRECTION('ref_axis',(-0.499999999999944,0.866025403784471,0.));
#20117=DIRECTION('',(-6.12323399573607E-17,1.06057523872495E-16,-1.));
#20118=DIRECTION('center_axis',(0.,0.,-1.));
#20119=DIRECTION('ref_axis',(-0.499999999999944,0.866025403784471,0.));
#20120=DIRECTION('',(-6.12323399573607E-17,1.06057523872495E-16,-1.));
#20121=DIRECTION('center_axis',(0.,0.,-1.));
#20122=DIRECTION('ref_axis',(-0.499999999999944,0.866025403784471,0.));
#20123=DIRECTION('',(-6.12323399573607E-17,1.06057523872495E-16,-1.));
#20124=DIRECTION('center_axis',(0.,0.,-1.));
#20125=DIRECTION('ref_axis',(-0.499999999999944,0.866025403784471,0.));
#20126=DIRECTION('',(-6.12323399573607E-17,1.06057523872495E-16,-1.));
#20127=DIRECTION('center_axis',(0.,0.,-1.));
#20128=DIRECTION('ref_axis',(-0.499999999999944,0.866025403784471,0.));
#20129=DIRECTION('',(-6.12323399573607E-17,1.06057523872495E-16,-1.));
#20130=DIRECTION('center_axis',(0.,0.,-1.));
#20131=DIRECTION('ref_axis',(-0.499999999999944,0.866025403784471,0.));
#20132=DIRECTION('',(-6.12323399573607E-17,1.06057523872495E-16,-1.));
#20133=DIRECTION('center_axis',(0.,0.,-1.));
#20134=DIRECTION('ref_axis',(-0.499999999999944,0.866025403784471,0.));
#20135=DIRECTION('',(-6.12323399573607E-17,1.06057523872495E-16,-1.));
#20136=DIRECTION('center_axis',(0.,0.,-1.));
#20137=DIRECTION('ref_axis',(-0.499999999999944,0.866025403784471,0.));
#20138=DIRECTION('',(-6.12323399573607E-17,1.06057523872495E-16,-1.));
#20139=DIRECTION('center_axis',(0.,0.,-1.));
#20140=DIRECTION('ref_axis',(-0.499999999999944,0.866025403784471,0.));
#20141=DIRECTION('',(-6.12323399573607E-17,1.06057523872495E-16,-1.));
#20142=DIRECTION('center_axis',(0.,0.,-1.));
#20143=DIRECTION('ref_axis',(0.991349121590847,-0.131251358549376,0.));
#20144=DIRECTION('',(-6.12323399573607E-17,1.06057523872495E-16,-1.));
#20145=DIRECTION('center_axis',(0.,0.,-1.));
#20146=DIRECTION('ref_axis',(-0.499999999999944,0.866025403784471,0.));
#20147=DIRECTION('center_axis',(0.,0.,-1.));
#20148=DIRECTION('ref_axis',(-1.,1.38777878078145E-16,0.));
#20149=DIRECTION('',(0.,0.,-1.));
#20150=DIRECTION('center_axis',(0.,0.,1.));
#20151=DIRECTION('ref_axis',(-1.,1.38777878078145E-16,0.));
#20152=DIRECTION('',(0.,0.,-1.));
#20153=DIRECTION('center_axis',(0.,0.,1.));
#20154=DIRECTION('ref_axis',(-1.,1.38777878078145E-16,0.));
#20155=DIRECTION('center_axis',(0.,0.,-1.));
#20156=DIRECTION('ref_axis',(-1.,1.38777878078145E-16,0.));
#20157=DIRECTION('',(0.,0.,-1.));
#20158=DIRECTION('center_axis',(0.,0.,-1.));
#20159=DIRECTION('ref_axis',(-1.,1.38777878078145E-16,0.));
#20160=DIRECTION('',(0.,0.,-1.));
#20161=DIRECTION('center_axis',(0.,0.,-1.));
#20162=DIRECTION('ref_axis',(-1.,1.38777878078145E-16,0.));
#20163=DIRECTION('',(0.,0.,-1.));
#20164=DIRECTION('center_axis',(0.,0.,-1.));
#20165=DIRECTION('ref_axis',(-1.,1.38777878078145E-16,0.));
#20166=DIRECTION('',(0.,0.,-1.));
#20167=DIRECTION('center_axis',(0.,0.,-1.));
#20168=DIRECTION('ref_axis',(-1.,1.38777878078145E-16,0.));
#20169=DIRECTION('',(0.,0.,-1.));
#20170=DIRECTION('center_axis',(0.,0.,-1.));
#20171=DIRECTION('ref_axis',(-1.,1.38777878078145E-16,0.));
#20172=DIRECTION('',(0.,0.,-1.));
#20173=DIRECTION('center_axis',(0.,0.,-1.));
#20174=DIRECTION('ref_axis',(-1.,1.38777878078145E-16,0.));
#20175=DIRECTION('',(0.,0.,-1.));
#20176=DIRECTION('center_axis',(0.,0.,-1.));
#20177=DIRECTION('ref_axis',(-1.,1.38777878078145E-16,0.));
#20178=DIRECTION('',(0.,0.,-1.));
#20179=DIRECTION('center_axis',(0.,0.,-1.));
#20180=DIRECTION('ref_axis',(-1.,1.38777878078145E-16,0.));
#20181=DIRECTION('',(0.,0.,-1.));
#20182=DIRECTION('center_axis',(0.,0.,-1.));
#20183=DIRECTION('ref_axis',(-1.,1.38777878078145E-16,0.));
#20184=DIRECTION('',(0.,0.,-1.));
#20185=DIRECTION('center_axis',(0.,0.,-1.));
#20186=DIRECTION('ref_axis',(-0.938437885424518,0.34544802098139,0.));
#20187=DIRECTION('',(0.,0.,-1.));
#20188=DIRECTION('center_axis',(0.,0.,-1.));
#20189=DIRECTION('ref_axis',(-1.,1.38777878078145E-16,0.));
#20190=DIRECTION('center_axis',(0.,0.,-1.));
#20191=DIRECTION('ref_axis',(-0.450150052286485,-0.892952927329585,0.));
#20192=DIRECTION('',(-1.22464679914735E-16,7.70405498938443E-30,-1.));
#20193=DIRECTION('center_axis',(0.,0.,1.));
#20194=DIRECTION('ref_axis',(-1.,6.27859183309933E-14,0.));
#20195=DIRECTION('center_axis',(0.,0.,-1.));
#20196=DIRECTION('ref_axis',(-1.,6.27859183309933E-14,0.));
#20197=DIRECTION('',(-1.22464679914735E-16,7.70405498938443E-30,-1.));
#20198=DIRECTION('center_axis',(0.,0.,-1.));
#20199=DIRECTION('ref_axis',(-1.,6.27859183309933E-14,0.));
#20200=DIRECTION('',(-1.22464679914735E-16,7.70405498938443E-30,-1.));
#20201=DIRECTION('center_axis',(0.,0.,-1.));
#20202=DIRECTION('ref_axis',(-1.,6.27859183309933E-14,0.));
#20203=DIRECTION('',(-1.22464679914735E-16,7.70405498938443E-30,-1.));
#20204=DIRECTION('center_axis',(0.,0.,-1.));
#20205=DIRECTION('ref_axis',(-1.,6.27859183309933E-14,0.));
#20206=DIRECTION('',(-1.22464679914735E-16,7.70405498938443E-30,-1.));
#20207=DIRECTION('center_axis',(0.,0.,-1.));
#20208=DIRECTION('ref_axis',(-1.,6.27859183309933E-14,0.));
#20209=DIRECTION('',(-1.22464679914735E-16,7.70405498938443E-30,-1.));
#20210=DIRECTION('center_axis',(0.,0.,-1.));
#20211=DIRECTION('ref_axis',(-1.,6.27859183309933E-14,0.));
#20212=DIRECTION('',(-1.22464679914735E-16,7.70405498938443E-30,-1.));
#20213=DIRECTION('center_axis',(0.,0.,-1.));
#20214=DIRECTION('ref_axis',(-1.,6.27859183309933E-14,0.));
#20215=DIRECTION('',(-1.22464679914735E-16,7.70405498938443E-30,-1.));
#20216=DIRECTION('center_axis',(0.,0.,-1.));
#20217=DIRECTION('ref_axis',(-1.,6.27859183309933E-14,0.));
#20218=DIRECTION('',(-1.22464679914735E-16,7.70405498938443E-30,-1.));
#20219=DIRECTION('center_axis',(0.,0.,-1.));
#20220=DIRECTION('ref_axis',(-1.,6.27859183309933E-14,0.));
#20221=DIRECTION('',(-1.22464679914735E-16,7.70405498938443E-30,-1.));
#20222=DIRECTION('center_axis',(0.,0.,-1.));
#20223=DIRECTION('ref_axis',(-1.,6.27859183309933E-14,0.));
#20224=DIRECTION('',(-1.22464679914735E-16,7.70405498938443E-30,-1.));
#20225=DIRECTION('center_axis',(0.,0.,-1.));
#20226=DIRECTION('ref_axis',(-1.,6.27859183309933E-14,0.));
#20227=DIRECTION('',(-1.22464679914735E-16,7.70405498938443E-30,-1.));
#20228=DIRECTION('center_axis',(0.,0.,-1.));
#20229=DIRECTION('ref_axis',(0.609343127961874,0.792906647976696,0.));
#20230=DIRECTION('',(-1.22464679914735E-16,7.70405498938443E-30,-1.));
#20231=DIRECTION('center_axis',(0.,0.,-1.));
#20232=DIRECTION('ref_axis',(-1.,6.27859183309933E-14,0.));
#20233=DIRECTION('center_axis',(0.,0.,-1.));
#20234=DIRECTION('ref_axis',(-0.5,-0.866025403784438,0.));
#20235=DIRECTION('',(0.,0.,-1.));
#20236=DIRECTION('center_axis',(0.,0.,1.));
#20237=DIRECTION('ref_axis',(-0.5,-0.866025403784438,0.));
#20238=DIRECTION('',(0.,0.,-1.));
#20239=DIRECTION('center_axis',(0.,0.,1.));
#20240=DIRECTION('ref_axis',(-0.5,-0.866025403784438,0.));
#20241=DIRECTION('center_axis',(0.,0.,-1.));
#20242=DIRECTION('ref_axis',(-0.5,-0.866025403784438,0.));
#20243=DIRECTION('',(0.,0.,-1.));
#20244=DIRECTION('center_axis',(0.,0.,-1.));
#20245=DIRECTION('ref_axis',(-0.5,-0.866025403784438,0.));
#20246=DIRECTION('',(0.,0.,-1.));
#20247=DIRECTION('center_axis',(0.,0.,-1.));
#20248=DIRECTION('ref_axis',(-0.5,-0.866025403784438,0.));
#20249=DIRECTION('',(0.,0.,-1.));
#20250=DIRECTION('center_axis',(0.,0.,-1.));
#20251=DIRECTION('ref_axis',(-0.5,-0.866025403784438,0.));
#20252=DIRECTION('',(0.,0.,-1.));
#20253=DIRECTION('center_axis',(0.,0.,-1.));
#20254=DIRECTION('ref_axis',(-0.5,-0.866025403784438,0.));
#20255=DIRECTION('',(0.,0.,-1.));
#20256=DIRECTION('center_axis',(0.,0.,-1.));
#20257=DIRECTION('ref_axis',(-0.5,-0.866025403784438,0.));
#20258=DIRECTION('',(0.,0.,-1.));
#20259=DIRECTION('center_axis',(0.,0.,-1.));
#20260=DIRECTION('ref_axis',(-0.5,-0.866025403784438,0.));
#20261=DIRECTION('',(0.,0.,-1.));
#20262=DIRECTION('center_axis',(0.,0.,-1.));
#20263=DIRECTION('ref_axis',(-0.5,-0.866025403784438,0.));
#20264=DIRECTION('',(0.,0.,-1.));
#20265=DIRECTION('center_axis',(0.,0.,-1.));
#20266=DIRECTION('ref_axis',(-0.5,-0.866025403784438,0.));
#20267=DIRECTION('',(0.,0.,-1.));
#20268=DIRECTION('center_axis',(0.,0.,-1.));
#20269=DIRECTION('ref_axis',(-0.5,-0.866025403784438,0.));
#20270=DIRECTION('',(0.,0.,-1.));
#20271=DIRECTION('center_axis',(0.,0.,-1.));
#20272=DIRECTION('ref_axis',(-0.768384438951799,-0.639988557692033,0.));
#20273=DIRECTION('',(0.,0.,-1.));
#20274=DIRECTION('center_axis',(0.,0.,-1.));
#20275=DIRECTION('ref_axis',(-0.5,-0.866025403784438,0.));
#20276=DIRECTION('center_axis',(0.,0.,-1.));
#20277=DIRECTION('ref_axis',(0.548242225181956,-0.8363195935332,0.));
#20278=DIRECTION('',(-6.12323399573746E-17,-1.06057523872487E-16,-1.));
#20279=DIRECTION('center_axis',(0.,0.,1.));
#20280=DIRECTION('ref_axis',(-0.500000000000056,-0.866025403784406,0.));
#20281=DIRECTION('center_axis',(0.,0.,-1.));
#20282=DIRECTION('ref_axis',(-0.500000000000056,-0.866025403784406,0.));
#20283=DIRECTION('',(-6.12323399573746E-17,-1.06057523872487E-16,-1.));
#20284=DIRECTION('center_axis',(0.,0.,-1.));
#20285=DIRECTION('ref_axis',(-0.500000000000056,-0.866025403784406,0.));
#20286=DIRECTION('',(-6.12323399573746E-17,-1.06057523872487E-16,-1.));
#20287=DIRECTION('center_axis',(0.,0.,-1.));
#20288=DIRECTION('ref_axis',(-0.500000000000056,-0.866025403784406,0.));
#20289=DIRECTION('',(-6.12323399573746E-17,-1.06057523872487E-16,-1.));
#20290=DIRECTION('center_axis',(0.,0.,-1.));
#20291=DIRECTION('ref_axis',(-0.500000000000056,-0.866025403784406,0.));
#20292=DIRECTION('',(-6.12323399573746E-17,-1.06057523872487E-16,-1.));
#20293=DIRECTION('center_axis',(0.,0.,-1.));
#20294=DIRECTION('ref_axis',(-0.500000000000056,-0.866025403784406,0.));
#20295=DIRECTION('',(-6.12323399573746E-17,-1.06057523872487E-16,-1.));
#20296=DIRECTION('center_axis',(0.,0.,-1.));
#20297=DIRECTION('ref_axis',(-0.500000000000056,-0.866025403784406,0.));
#20298=DIRECTION('',(-6.12323399573746E-17,-1.06057523872487E-16,-1.));
#20299=DIRECTION('center_axis',(0.,0.,-1.));
#20300=DIRECTION('ref_axis',(-0.500000000000056,-0.866025403784406,0.));
#20301=DIRECTION('',(-6.12323399573746E-17,-1.06057523872487E-16,-1.));
#20302=DIRECTION('center_axis',(0.,0.,-1.));
#20303=DIRECTION('ref_axis',(-0.500000000000056,-0.866025403784406,0.));
#20304=DIRECTION('',(-6.12323399573746E-17,-1.06057523872487E-16,-1.));
#20305=DIRECTION('center_axis',(0.,0.,-1.));
#20306=DIRECTION('ref_axis',(-0.500000000000056,-0.866025403784406,0.));
#20307=DIRECTION('',(-6.12323399573746E-17,-1.06057523872487E-16,-1.));
#20308=DIRECTION('center_axis',(0.,0.,-1.));
#20309=DIRECTION('ref_axis',(-0.500000000000056,-0.866025403784406,0.));
#20310=DIRECTION('',(-6.12323399573746E-17,-1.06057523872487E-16,-1.));
#20311=DIRECTION('center_axis',(0.,0.,-1.));
#20312=DIRECTION('ref_axis',(-0.500000000000056,-0.866025403784406,0.));
#20313=DIRECTION('',(-6.12323399573746E-17,-1.06057523872487E-16,-1.));
#20314=DIRECTION('center_axis',(0.,0.,-1.));
#20315=DIRECTION('ref_axis',(-0.382007546651474,0.924159203980203,0.));
#20316=DIRECTION('',(-6.12323399573746E-17,-1.06057523872487E-16,-1.));
#20317=DIRECTION('center_axis',(0.,0.,-1.));
#20318=DIRECTION('ref_axis',(-0.500000000000056,-0.866025403784406,0.));
#20319=DIRECTION('center_axis',(0.,0.,-1.));
#20320=DIRECTION('ref_axis',(0.499999999999999,-0.866025403784439,0.));
#20321=DIRECTION('',(0.,0.,-1.));
#20322=DIRECTION('center_axis',(0.,0.,1.));
#20323=DIRECTION('ref_axis',(0.499999999999999,-0.866025403784439,0.));
#20324=DIRECTION('',(0.,0.,-1.));
#20325=DIRECTION('center_axis',(0.,0.,1.));
#20326=DIRECTION('ref_axis',(0.499999999999999,-0.866025403784439,0.));
#20327=DIRECTION('center_axis',(0.,0.,-1.));
#20328=DIRECTION('ref_axis',(0.499999999999999,-0.866025403784439,0.));
#20329=DIRECTION('',(0.,0.,-1.));
#20330=DIRECTION('center_axis',(0.,0.,-1.));
#20331=DIRECTION('ref_axis',(0.499999999999999,-0.866025403784439,0.));
#20332=DIRECTION('',(0.,0.,-1.));
#20333=DIRECTION('center_axis',(0.,0.,-1.));
#20334=DIRECTION('ref_axis',(0.499999999999999,-0.866025403784439,0.));
#20335=DIRECTION('',(0.,0.,-1.));
#20336=DIRECTION('center_axis',(0.,0.,-1.));
#20337=DIRECTION('ref_axis',(0.499999999999999,-0.866025403784439,0.));
#20338=DIRECTION('',(0.,0.,-1.));
#20339=DIRECTION('center_axis',(0.,0.,-1.));
#20340=DIRECTION('ref_axis',(0.499999999999999,-0.866025403784439,0.));
#20341=DIRECTION('',(0.,0.,-1.));
#20342=DIRECTION('center_axis',(0.,0.,-1.));
#20343=DIRECTION('ref_axis',(0.499999999999999,-0.866025403784439,0.));
#20344=DIRECTION('',(0.,0.,-1.));
#20345=DIRECTION('center_axis',(0.,0.,-1.));
#20346=DIRECTION('ref_axis',(0.499999999999999,-0.866025403784439,0.));
#20347=DIRECTION('',(0.,0.,-1.));
#20348=DIRECTION('center_axis',(0.,0.,-1.));
#20349=DIRECTION('ref_axis',(0.499999999999999,-0.866025403784439,0.));
#20350=DIRECTION('',(0.,0.,-1.));
#20351=DIRECTION('center_axis',(0.,0.,-1.));
#20352=DIRECTION('ref_axis',(0.499999999999999,-0.866025403784439,0.));
#20353=DIRECTION('',(0.,0.,-1.));
#20354=DIRECTION('center_axis',(0.,0.,-1.));
#20355=DIRECTION('ref_axis',(0.499999999999999,-0.866025403784439,0.));
#20356=DIRECTION('',(0.,0.,-1.));
#20357=DIRECTION('center_axis',(0.,0.,-1.));
#20358=DIRECTION('ref_axis',(0.170054135023835,-0.985434721917842,0.));
#20359=DIRECTION('',(0.,0.,-1.));
#20360=DIRECTION('center_axis',(0.,0.,-1.));
#20361=DIRECTION('ref_axis',(0.499999999999999,-0.866025403784439,0.));
#20362=DIRECTION('center_axis',(0.,0.,-1.));
#20363=DIRECTION('ref_axis',(0.998395126723898,0.0566318897262945,0.));
#20364=DIRECTION('',(6.12323399573609E-17,-1.06057523872495E-16,-1.));
#20365=DIRECTION('center_axis',(0.,0.,1.));
#20366=DIRECTION('ref_axis',(0.499999999999945,-0.86602540378447,0.));
#20367=DIRECTION('center_axis',(0.,0.,-1.));
#20368=DIRECTION('ref_axis',(0.499999999999945,-0.86602540378447,0.));
#20369=DIRECTION('',(6.12323399573609E-17,-1.06057523872495E-16,-1.));
#20370=DIRECTION('center_axis',(0.,0.,-1.));
#20371=DIRECTION('ref_axis',(0.499999999999945,-0.86602540378447,0.));
#20372=DIRECTION('',(6.12323399573609E-17,-1.06057523872495E-16,-1.));
#20373=DIRECTION('center_axis',(0.,0.,-1.));
#20374=DIRECTION('ref_axis',(0.499999999999945,-0.86602540378447,0.));
#20375=DIRECTION('',(6.12323399573609E-17,-1.06057523872495E-16,-1.));
#20376=DIRECTION('center_axis',(0.,0.,-1.));
#20377=DIRECTION('ref_axis',(0.499999999999945,-0.86602540378447,0.));
#20378=DIRECTION('',(6.12323399573609E-17,-1.06057523872495E-16,-1.));
#20379=DIRECTION('center_axis',(0.,0.,-1.));
#20380=DIRECTION('ref_axis',(0.499999999999945,-0.86602540378447,0.));
#20381=DIRECTION('',(6.12323399573609E-17,-1.06057523872495E-16,-1.));
#20382=DIRECTION('center_axis',(0.,0.,-1.));
#20383=DIRECTION('ref_axis',(0.499999999999945,-0.86602540378447,0.));
#20384=DIRECTION('',(6.12323399573609E-17,-1.06057523872495E-16,-1.));
#20385=DIRECTION('center_axis',(0.,0.,-1.));
#20386=DIRECTION('ref_axis',(0.499999999999945,-0.86602540378447,0.));
#20387=DIRECTION('',(6.12323399573609E-17,-1.06057523872495E-16,-1.));
#20388=DIRECTION('center_axis',(0.,0.,-1.));
#20389=DIRECTION('ref_axis',(0.499999999999945,-0.86602540378447,0.));
#20390=DIRECTION('',(6.12323399573609E-17,-1.06057523872495E-16,-1.));
#20391=DIRECTION('center_axis',(0.,0.,-1.));
#20392=DIRECTION('ref_axis',(0.499999999999945,-0.86602540378447,0.));
#20393=DIRECTION('',(6.12323399573609E-17,-1.06057523872495E-16,-1.));
#20394=DIRECTION('center_axis',(0.,0.,-1.));
#20395=DIRECTION('ref_axis',(0.499999999999945,-0.86602540378447,0.));
#20396=DIRECTION('',(6.12323399573609E-17,-1.06057523872495E-16,-1.));
#20397=DIRECTION('center_axis',(0.,0.,-1.));
#20398=DIRECTION('ref_axis',(0.499999999999945,-0.86602540378447,0.));
#20399=DIRECTION('',(6.12323399573609E-17,-1.06057523872495E-16,-1.));
#20400=DIRECTION('center_axis',(0.,0.,-1.));
#20401=DIRECTION('ref_axis',(-0.991349121590847,0.13125135854937,0.));
#20402=DIRECTION('',(6.12323399573609E-17,-1.06057523872495E-16,-1.));
#20403=DIRECTION('center_axis',(0.,0.,-1.));
#20404=DIRECTION('ref_axis',(0.499999999999945,-0.86602540378447,0.));
#20405=DIRECTION('center_axis',(0.,0.,1.));
#20406=DIRECTION('ref_axis',(-0.5,-0.866025403784439,0.));
#20407=DIRECTION('',(0.,0.,1.));
#20408=DIRECTION('center_axis',(0.,0.,-1.));
#20409=DIRECTION('ref_axis',(-0.5,-0.866025403784439,0.));
#20410=DIRECTION('',(0.,0.,1.));
#20411=DIRECTION('center_axis',(0.,0.,-1.));
#20412=DIRECTION('ref_axis',(-0.5,-0.866025403784439,0.));
#20413=DIRECTION('center_axis',(0.,0.,1.));
#20414=DIRECTION('ref_axis',(-0.5,-0.866025403784439,0.));
#20415=DIRECTION('',(0.,0.,1.));
#20416=DIRECTION('center_axis',(0.,0.,1.));
#20417=DIRECTION('ref_axis',(-0.5,-0.866025403784439,0.));
#20418=DIRECTION('',(0.,0.,1.));
#20419=DIRECTION('center_axis',(0.,0.,1.));
#20420=DIRECTION('ref_axis',(-0.5,-0.866025403784439,0.));
#20421=DIRECTION('',(0.,0.,1.));
#20422=DIRECTION('center_axis',(0.,0.,1.));
#20423=DIRECTION('ref_axis',(-0.5,-0.866025403784439,0.));
#20424=DIRECTION('',(0.,0.,1.));
#20425=DIRECTION('center_axis',(0.,0.,1.));
#20426=DIRECTION('ref_axis',(-0.5,-0.866025403784439,0.));
#20427=DIRECTION('',(0.,0.,1.));
#20428=DIRECTION('center_axis',(0.,0.,1.));
#20429=DIRECTION('ref_axis',(-0.5,-0.866025403784439,0.));
#20430=DIRECTION('',(0.,0.,1.));
#20431=DIRECTION('center_axis',(0.,0.,1.));
#20432=DIRECTION('ref_axis',(-0.5,-0.866025403784439,0.));
#20433=DIRECTION('',(0.,0.,1.));
#20434=DIRECTION('center_axis',(0.,0.,1.));
#20435=DIRECTION('ref_axis',(-0.5,-0.866025403784439,0.));
#20436=DIRECTION('',(0.,0.,1.));
#20437=DIRECTION('center_axis',(0.,0.,1.));
#20438=DIRECTION('ref_axis',(-0.5,-0.866025403784439,0.));
#20439=DIRECTION('',(0.,0.,1.));
#20440=DIRECTION('center_axis',(0.,0.,1.));
#20441=DIRECTION('ref_axis',(-0.5,-0.866025403784439,0.));
#20442=DIRECTION('',(0.,0.,1.));
#20443=DIRECTION('center_axis',(0.,0.,1.));
#20444=DIRECTION('ref_axis',(-0.170053080456876,-0.985434903901383,0.));
#20445=DIRECTION('',(0.,0.,1.));
#20446=DIRECTION('center_axis',(0.,0.,-1.));
#20447=DIRECTION('ref_axis',(-0.5,-0.866025403784439,0.));
#20448=DIRECTION('center_axis',(0.,0.,1.));
#20449=DIRECTION('ref_axis',(-0.998395022062647,0.0566337348276312,0.));
#20450=DIRECTION('',(-6.12323399573623E-17,-1.06057523872494E-16,1.));
#20451=DIRECTION('center_axis',(0.,0.,-1.));
#20452=DIRECTION('ref_axis',(-0.499999999999956,-0.866025403784464,0.));
#20453=DIRECTION('center_axis',(0.,0.,1.));
#20454=DIRECTION('ref_axis',(-0.499999999999956,-0.866025403784464,0.));
#20455=DIRECTION('',(-6.12323399573623E-17,-1.06057523872494E-16,1.));
#20456=DIRECTION('center_axis',(0.,0.,1.));
#20457=DIRECTION('ref_axis',(-0.499999999999956,-0.866025403784464,0.));
#20458=DIRECTION('',(-6.12323399573623E-17,-1.06057523872494E-16,1.));
#20459=DIRECTION('center_axis',(0.,0.,1.));
#20460=DIRECTION('ref_axis',(-0.499999999999956,-0.866025403784464,0.));
#20461=DIRECTION('',(-6.12323399573623E-17,-1.06057523872494E-16,1.));
#20462=DIRECTION('center_axis',(0.,0.,1.));
#20463=DIRECTION('ref_axis',(-0.499999999999956,-0.866025403784464,0.));
#20464=DIRECTION('',(-6.12323399573623E-17,-1.06057523872494E-16,1.));
#20465=DIRECTION('center_axis',(0.,0.,1.));
#20466=DIRECTION('ref_axis',(-0.499999999999956,-0.866025403784464,0.));
#20467=DIRECTION('',(-6.12323399573623E-17,-1.06057523872494E-16,1.));
#20468=DIRECTION('center_axis',(0.,0.,1.));
#20469=DIRECTION('ref_axis',(-0.499999999999956,-0.866025403784464,0.));
#20470=DIRECTION('',(-6.12323399573623E-17,-1.06057523872494E-16,1.));
#20471=DIRECTION('center_axis',(0.,0.,1.));
#20472=DIRECTION('ref_axis',(-0.499999999999956,-0.866025403784464,0.));
#20473=DIRECTION('',(-6.12323399573623E-17,-1.06057523872494E-16,1.));
#20474=DIRECTION('center_axis',(0.,0.,1.));
#20475=DIRECTION('ref_axis',(-0.499999999999956,-0.866025403784464,0.));
#20476=DIRECTION('',(-6.12323399573623E-17,-1.06057523872494E-16,1.));
#20477=DIRECTION('center_axis',(0.,0.,1.));
#20478=DIRECTION('ref_axis',(-0.499999999999956,-0.866025403784464,0.));
#20479=DIRECTION('',(-6.12323399573623E-17,-1.06057523872494E-16,1.));
#20480=DIRECTION('center_axis',(0.,0.,1.));
#20481=DIRECTION('ref_axis',(-0.499999999999956,-0.866025403784464,0.));
#20482=DIRECTION('',(-6.12323399573623E-17,-1.06057523872494E-16,1.));
#20483=DIRECTION('center_axis',(0.,0.,1.));
#20484=DIRECTION('ref_axis',(-0.499999999999956,-0.866025403784464,0.));
#20485=DIRECTION('',(-6.12323399573623E-17,-1.06057523872494E-16,1.));
#20486=DIRECTION('center_axis',(0.,0.,1.));
#20487=DIRECTION('ref_axis',(0.991348961503156,0.131252567695316,0.));
#20488=DIRECTION('',(-6.12323399573623E-17,-1.06057523872494E-16,1.));
#20489=DIRECTION('center_axis',(0.,0.,1.));
#20490=DIRECTION('ref_axis',(-0.499999999999956,-0.866025403784464,0.));
#20491=DIRECTION('center_axis',(0.,0.,1.));
#20492=DIRECTION('ref_axis',(0.5,-0.866025403784439,0.));
#20493=DIRECTION('',(0.,0.,1.));
#20494=DIRECTION('center_axis',(0.,0.,-1.));
#20495=DIRECTION('ref_axis',(0.5,-0.866025403784439,0.));
#20496=DIRECTION('',(0.,0.,1.));
#20497=DIRECTION('center_axis',(0.,0.,-1.));
#20498=DIRECTION('ref_axis',(0.5,-0.866025403784439,0.));
#20499=DIRECTION('center_axis',(0.,0.,1.));
#20500=DIRECTION('ref_axis',(0.5,-0.866025403784439,0.));
#20501=DIRECTION('',(0.,0.,1.));
#20502=DIRECTION('center_axis',(0.,0.,1.));
#20503=DIRECTION('ref_axis',(0.5,-0.866025403784439,0.));
#20504=DIRECTION('',(0.,0.,1.));
#20505=DIRECTION('center_axis',(0.,0.,1.));
#20506=DIRECTION('ref_axis',(0.5,-0.866025403784439,0.));
#20507=DIRECTION('',(0.,0.,1.));
#20508=DIRECTION('center_axis',(0.,0.,1.));
#20509=DIRECTION('ref_axis',(0.5,-0.866025403784439,0.));
#20510=DIRECTION('',(0.,0.,1.));
#20511=DIRECTION('center_axis',(0.,0.,1.));
#20512=DIRECTION('ref_axis',(0.5,-0.866025403784439,0.));
#20513=DIRECTION('',(0.,0.,1.));
#20514=DIRECTION('center_axis',(0.,0.,1.));
#20515=DIRECTION('ref_axis',(0.5,-0.866025403784439,0.));
#20516=DIRECTION('',(0.,0.,1.));
#20517=DIRECTION('center_axis',(0.,0.,1.));
#20518=DIRECTION('ref_axis',(0.5,-0.866025403784439,0.));
#20519=DIRECTION('',(0.,0.,1.));
#20520=DIRECTION('center_axis',(0.,0.,1.));
#20521=DIRECTION('ref_axis',(0.5,-0.866025403784439,0.));
#20522=DIRECTION('',(0.,0.,1.));
#20523=DIRECTION('center_axis',(0.,0.,1.));
#20524=DIRECTION('ref_axis',(0.5,-0.866025403784439,0.));
#20525=DIRECTION('',(0.,0.,1.));
#20526=DIRECTION('center_axis',(0.,0.,1.));
#20527=DIRECTION('ref_axis',(0.5,-0.866025403784439,0.));
#20528=DIRECTION('',(0.,0.,1.));
#20529=DIRECTION('center_axis',(0.,0.,1.));
#20530=DIRECTION('ref_axis',(0.768385143082245,-0.639987712296477,0.));
#20531=DIRECTION('',(0.,0.,1.));
#20532=DIRECTION('center_axis',(0.,0.,-1.));
#20533=DIRECTION('ref_axis',(0.5,-0.866025403784439,0.));
#20534=DIRECTION('center_axis',(0.,0.,1.));
#20535=DIRECTION('ref_axis',(-0.548243791989891,-0.836318566423432,0.));
#20536=DIRECTION('',(6.12323399573727E-17,-1.06057523872488E-16,1.));
#20537=DIRECTION('center_axis',(0.,0.,-1.));
#20538=DIRECTION('ref_axis',(0.500000000000041,-0.866025403784415,0.));
#20539=DIRECTION('center_axis',(0.,0.,1.));
#20540=DIRECTION('ref_axis',(0.500000000000041,-0.866025403784415,0.));
#20541=DIRECTION('',(6.12323399573727E-17,-1.06057523872488E-16,1.));
#20542=DIRECTION('center_axis',(0.,0.,1.));
#20543=DIRECTION('ref_axis',(0.500000000000041,-0.866025403784415,0.));
#20544=DIRECTION('',(6.12323399573727E-17,-1.06057523872488E-16,1.));
#20545=DIRECTION('center_axis',(0.,0.,1.));
#20546=DIRECTION('ref_axis',(0.500000000000041,-0.866025403784415,0.));
#20547=DIRECTION('',(6.12323399573727E-17,-1.06057523872488E-16,1.));
#20548=DIRECTION('center_axis',(0.,0.,1.));
#20549=DIRECTION('ref_axis',(0.500000000000041,-0.866025403784415,0.));
#20550=DIRECTION('',(6.12323399573727E-17,-1.06057523872488E-16,1.));
#20551=DIRECTION('center_axis',(0.,0.,1.));
#20552=DIRECTION('ref_axis',(0.500000000000041,-0.866025403784415,0.));
#20553=DIRECTION('',(6.12323399573727E-17,-1.06057523872488E-16,1.));
#20554=DIRECTION('center_axis',(0.,0.,1.));
#20555=DIRECTION('ref_axis',(0.500000000000041,-0.866025403784415,0.));
#20556=DIRECTION('',(6.12323399573727E-17,-1.06057523872488E-16,1.));
#20557=DIRECTION('center_axis',(0.,0.,1.));
#20558=DIRECTION('ref_axis',(0.500000000000041,-0.866025403784415,0.));
#20559=DIRECTION('',(6.12323399573727E-17,-1.06057523872488E-16,1.));
#20560=DIRECTION('center_axis',(0.,0.,1.));
#20561=DIRECTION('ref_axis',(0.500000000000041,-0.866025403784415,0.));
#20562=DIRECTION('',(6.12323399573727E-17,-1.06057523872488E-16,1.));
#20563=DIRECTION('center_axis',(0.,0.,1.));
#20564=DIRECTION('ref_axis',(0.500000000000041,-0.866025403784415,0.));
#20565=DIRECTION('',(6.12323399573727E-17,-1.06057523872488E-16,1.));
#20566=DIRECTION('center_axis',(0.,0.,1.));
#20567=DIRECTION('ref_axis',(0.500000000000041,-0.866025403784415,0.));
#20568=DIRECTION('',(6.12323399573727E-17,-1.06057523872488E-16,1.));
#20569=DIRECTION('center_axis',(0.,0.,1.));
#20570=DIRECTION('ref_axis',(0.500000000000041,-0.866025403784415,0.));
#20571=DIRECTION('',(6.12323399573727E-17,-1.06057523872488E-16,1.));
#20572=DIRECTION('center_axis',(0.,0.,1.));
#20573=DIRECTION('ref_axis',(0.382006426201404,0.92415966712513,0.));
#20574=DIRECTION('',(6.12323399573727E-17,-1.06057523872488E-16,1.));
#20575=DIRECTION('center_axis',(0.,0.,1.));
#20576=DIRECTION('ref_axis',(0.500000000000041,-0.866025403784415,0.));
#20577=DIRECTION('center_axis',(0.,0.,1.));
#20578=DIRECTION('ref_axis',(1.,-1.38777878078145E-16,0.));
#20579=DIRECTION('',(0.,0.,1.));
#20580=DIRECTION('center_axis',(0.,0.,-1.));
#20581=DIRECTION('ref_axis',(1.,-1.38777878078145E-16,0.));
#20582=DIRECTION('',(0.,0.,1.));
#20583=DIRECTION('center_axis',(0.,0.,-1.));
#20584=DIRECTION('ref_axis',(1.,-1.38777878078145E-16,0.));
#20585=DIRECTION('center_axis',(0.,0.,1.));
#20586=DIRECTION('ref_axis',(1.,-1.38777878078145E-16,0.));
#20587=DIRECTION('',(0.,0.,1.));
#20588=DIRECTION('center_axis',(0.,0.,1.));
#20589=DIRECTION('ref_axis',(1.,-1.38777878078145E-16,0.));
#20590=DIRECTION('',(0.,0.,1.));
#20591=DIRECTION('center_axis',(0.,0.,1.));
#20592=DIRECTION('ref_axis',(1.,-1.38777878078145E-16,0.));
#20593=DIRECTION('',(0.,0.,1.));
#20594=DIRECTION('center_axis',(0.,0.,1.));
#20595=DIRECTION('ref_axis',(1.,-1.38777878078145E-16,0.));
#20596=DIRECTION('',(0.,0.,1.));
#20597=DIRECTION('center_axis',(0.,0.,1.));
#20598=DIRECTION('ref_axis',(1.,-1.38777878078145E-16,0.));
#20599=DIRECTION('',(0.,0.,1.));
#20600=DIRECTION('center_axis',(0.,0.,1.));
#20601=DIRECTION('ref_axis',(1.,-1.38777878078145E-16,0.));
#20602=DIRECTION('',(0.,0.,1.));
#20603=DIRECTION('center_axis',(0.,0.,1.));
#20604=DIRECTION('ref_axis',(1.,-1.38777878078145E-16,0.));
#20605=DIRECTION('',(0.,0.,1.));
#20606=DIRECTION('center_axis',(0.,0.,1.));
#20607=DIRECTION('ref_axis',(1.,-1.38777878078145E-16,0.));
#20608=DIRECTION('',(0.,0.,1.));
#20609=DIRECTION('center_axis',(0.,0.,1.));
#20610=DIRECTION('ref_axis',(1.,-1.38777878078145E-16,0.));
#20611=DIRECTION('',(0.,0.,1.));
#20612=DIRECTION('center_axis',(0.,0.,1.));
#20613=DIRECTION('ref_axis',(1.,-1.38777878078145E-16,0.));
#20614=DIRECTION('',(0.,0.,1.));
#20615=DIRECTION('center_axis',(0.,0.,1.));
#20616=DIRECTION('ref_axis',(0.938437365767004,0.345449432670379,0.));
#20617=DIRECTION('',(0.,0.,1.));
#20618=DIRECTION('center_axis',(0.,0.,-1.));
#20619=DIRECTION('ref_axis',(1.,-1.38777878078145E-16,0.));
#20620=DIRECTION('center_axis',(0.,0.,1.));
#20621=DIRECTION('ref_axis',(0.450147885469881,-0.892954019648825,0.));
#20622=DIRECTION('',(1.22464679914735E-16,6.13548173299478E-30,1.));
#20623=DIRECTION('center_axis',(0.,0.,-1.));
#20624=DIRECTION('ref_axis',(1.,4.99775456844331E-14,0.));
#20625=DIRECTION('center_axis',(0.,0.,1.));
#20626=DIRECTION('ref_axis',(1.,4.99775456844331E-14,0.));
#20627=DIRECTION('',(1.22464679914735E-16,6.13548173299478E-30,1.));
#20628=DIRECTION('center_axis',(0.,0.,1.));
#20629=DIRECTION('ref_axis',(1.,4.99775456844331E-14,0.));
#20630=DIRECTION('',(1.22464679914735E-16,6.13548173299478E-30,1.));
#20631=DIRECTION('center_axis',(0.,0.,1.));
#20632=DIRECTION('ref_axis',(1.,4.99775456844331E-14,0.));
#20633=DIRECTION('',(1.22464679914735E-16,6.13548173299478E-30,1.));
#20634=DIRECTION('center_axis',(0.,0.,1.));
#20635=DIRECTION('ref_axis',(1.,4.99775456844331E-14,0.));
#20636=DIRECTION('',(1.22464679914735E-16,6.13548173299478E-30,1.));
#20637=DIRECTION('center_axis',(0.,0.,1.));
#20638=DIRECTION('ref_axis',(1.,4.99775456844331E-14,0.));
#20639=DIRECTION('',(1.22464679914735E-16,6.13548173299478E-30,1.));
#20640=DIRECTION('center_axis',(0.,0.,1.));
#20641=DIRECTION('ref_axis',(1.,4.99775456844331E-14,0.));
#20642=DIRECTION('',(1.22464679914735E-16,6.13548173299478E-30,1.));
#20643=DIRECTION('center_axis',(0.,0.,1.));
#20644=DIRECTION('ref_axis',(1.,4.99775456844331E-14,0.));
#20645=DIRECTION('',(1.22464679914735E-16,6.13548173299478E-30,1.));
#20646=DIRECTION('center_axis',(0.,0.,1.));
#20647=DIRECTION('ref_axis',(1.,4.99775456844331E-14,0.));
#20648=DIRECTION('',(1.22464679914735E-16,6.13548173299478E-30,1.));
#20649=DIRECTION('center_axis',(0.,0.,1.));
#20650=DIRECTION('ref_axis',(1.,4.99775456844331E-14,0.));
#20651=DIRECTION('',(1.22464679914735E-16,6.13548173299478E-30,1.));
#20652=DIRECTION('center_axis',(0.,0.,1.));
#20653=DIRECTION('ref_axis',(1.,4.99775456844331E-14,0.));
#20654=DIRECTION('',(1.22464679914735E-16,6.13548173299478E-30,1.));
#20655=DIRECTION('center_axis',(0.,0.,1.));
#20656=DIRECTION('ref_axis',(1.,4.99775456844331E-14,0.));
#20657=DIRECTION('',(1.22464679914735E-16,6.13548173299478E-30,1.));
#20658=DIRECTION('center_axis',(0.,0.,1.));
#20659=DIRECTION('ref_axis',(-0.609344456561461,0.792905626955577,0.));
#20660=DIRECTION('',(1.22464679914735E-16,6.13548173299478E-30,1.));
#20661=DIRECTION('center_axis',(0.,0.,1.));
#20662=DIRECTION('ref_axis',(1.,4.99775456844331E-14,0.));
#20663=DIRECTION('center_axis',(0.,0.,1.));
#20664=DIRECTION('ref_axis',(0.5,0.866025403784438,0.));
#20665=DIRECTION('',(0.,0.,1.));
#20666=DIRECTION('center_axis',(0.,0.,-1.));
#20667=DIRECTION('ref_axis',(0.5,0.866025403784438,0.));
#20668=DIRECTION('',(0.,0.,1.));
#20669=DIRECTION('center_axis',(0.,0.,-1.));
#20670=DIRECTION('ref_axis',(0.5,0.866025403784438,0.));
#20671=DIRECTION('center_axis',(0.,0.,1.));
#20672=DIRECTION('ref_axis',(0.5,0.866025403784438,0.));
#20673=DIRECTION('',(0.,0.,1.));
#20674=DIRECTION('center_axis',(0.,0.,1.));
#20675=DIRECTION('ref_axis',(0.5,0.866025403784438,0.));
#20676=DIRECTION('',(0.,0.,1.));
#20677=DIRECTION('center_axis',(0.,0.,1.));
#20678=DIRECTION('ref_axis',(0.5,0.866025403784438,0.));
#20679=DIRECTION('',(0.,0.,1.));
#20680=DIRECTION('center_axis',(0.,0.,1.));
#20681=DIRECTION('ref_axis',(0.5,0.866025403784438,0.));
#20682=DIRECTION('',(0.,0.,1.));
#20683=DIRECTION('center_axis',(0.,0.,1.));
#20684=DIRECTION('ref_axis',(0.5,0.866025403784438,0.));
#20685=DIRECTION('',(0.,0.,1.));
#20686=DIRECTION('center_axis',(0.,0.,1.));
#20687=DIRECTION('ref_axis',(0.5,0.866025403784438,0.));
#20688=DIRECTION('',(0.,0.,1.));
#20689=DIRECTION('center_axis',(0.,0.,1.));
#20690=DIRECTION('ref_axis',(0.5,0.866025403784438,0.));
#20691=DIRECTION('',(0.,0.,1.));
#20692=DIRECTION('center_axis',(0.,0.,1.));
#20693=DIRECTION('ref_axis',(0.5,0.866025403784438,0.));
#20694=DIRECTION('',(0.,0.,1.));
#20695=DIRECTION('center_axis',(0.,0.,1.));
#20696=DIRECTION('ref_axis',(0.5,0.866025403784438,0.));
#20697=DIRECTION('',(0.,0.,1.));
#20698=DIRECTION('center_axis',(0.,0.,1.));
#20699=DIRECTION('ref_axis',(0.5,0.866025403784438,0.));
#20700=DIRECTION('',(0.,0.,1.));
#20701=DIRECTION('center_axis',(0.,0.,1.));
#20702=DIRECTION('ref_axis',(0.170053080456934,0.985434903901373,0.));
#20703=DIRECTION('',(0.,0.,1.));
#20704=DIRECTION('center_axis',(0.,0.,-1.));
#20705=DIRECTION('ref_axis',(0.5,0.866025403784438,0.));
#20706=DIRECTION('center_axis',(0.,0.,1.));
#20707=DIRECTION('ref_axis',(0.998395022062648,-0.0566337348276226,0.));
#20708=DIRECTION('',(6.12323399573605E-17,1.06057523872495E-16,1.));
#20709=DIRECTION('center_axis',(0.,0.,-1.));
#20710=DIRECTION('ref_axis',(0.499999999999942,0.866025403784472,0.));
#20711=DIRECTION('center_axis',(0.,0.,1.));
#20712=DIRECTION('ref_axis',(0.499999999999942,0.866025403784472,0.));
#20713=DIRECTION('',(6.12323399573605E-17,1.06057523872495E-16,1.));
#20714=DIRECTION('center_axis',(0.,0.,1.));
#20715=DIRECTION('ref_axis',(0.499999999999942,0.866025403784472,0.));
#20716=DIRECTION('',(6.12323399573605E-17,1.06057523872495E-16,1.));
#20717=DIRECTION('center_axis',(0.,0.,1.));
#20718=DIRECTION('ref_axis',(0.499999999999942,0.866025403784472,0.));
#20719=DIRECTION('',(6.12323399573605E-17,1.06057523872495E-16,1.));
#20720=DIRECTION('center_axis',(0.,0.,1.));
#20721=DIRECTION('ref_axis',(0.499999999999942,0.866025403784472,0.));
#20722=DIRECTION('',(6.12323399573605E-17,1.06057523872495E-16,1.));
#20723=DIRECTION('center_axis',(0.,0.,1.));
#20724=DIRECTION('ref_axis',(0.499999999999942,0.866025403784472,0.));
#20725=DIRECTION('',(6.12323399573605E-17,1.06057523872495E-16,1.));
#20726=DIRECTION('center_axis',(0.,0.,1.));
#20727=DIRECTION('ref_axis',(0.499999999999942,0.866025403784472,0.));
#20728=DIRECTION('',(6.12323399573605E-17,1.06057523872495E-16,1.));
#20729=DIRECTION('center_axis',(0.,0.,1.));
#20730=DIRECTION('ref_axis',(0.499999999999942,0.866025403784472,0.));
#20731=DIRECTION('',(6.12323399573605E-17,1.06057523872495E-16,1.));
#20732=DIRECTION('center_axis',(0.,0.,1.));
#20733=DIRECTION('ref_axis',(0.499999999999942,0.866025403784472,0.));
#20734=DIRECTION('',(6.12323399573605E-17,1.06057523872495E-16,1.));
#20735=DIRECTION('center_axis',(0.,0.,1.));
#20736=DIRECTION('ref_axis',(0.499999999999942,0.866025403784472,0.));
#20737=DIRECTION('',(6.12323399573605E-17,1.06057523872495E-16,1.));
#20738=DIRECTION('center_axis',(0.,0.,1.));
#20739=DIRECTION('ref_axis',(0.499999999999942,0.866025403784472,0.));
#20740=DIRECTION('',(6.12323399573605E-17,1.06057523872495E-16,1.));
#20741=DIRECTION('center_axis',(0.,0.,1.));
#20742=DIRECTION('ref_axis',(0.499999999999942,0.866025403784472,0.));
#20743=DIRECTION('',(6.12323399573605E-17,1.06057523872495E-16,1.));
#20744=DIRECTION('center_axis',(0.,0.,1.));
#20745=DIRECTION('ref_axis',(-0.991348961503154,-0.131252567695333,0.));
#20746=DIRECTION('',(6.12323399573605E-17,1.06057523872495E-16,1.));
#20747=DIRECTION('center_axis',(0.,0.,1.));
#20748=DIRECTION('ref_axis',(0.499999999999942,0.866025403784472,0.));
#20749=DIRECTION('center_axis',(0.,0.,1.));
#20750=DIRECTION('ref_axis',(-0.499999999999999,0.866025403784439,0.));
#20751=DIRECTION('',(0.,0.,1.));
#20752=DIRECTION('center_axis',(0.,0.,-1.));
#20753=DIRECTION('ref_axis',(-0.499999999999999,0.866025403784439,0.));
#20754=DIRECTION('',(0.,0.,1.));
#20755=DIRECTION('center_axis',(0.,0.,-1.));
#20756=DIRECTION('ref_axis',(-0.499999999999999,0.866025403784439,0.));
#20757=DIRECTION('center_axis',(0.,0.,1.));
#20758=DIRECTION('ref_axis',(-0.499999999999999,0.866025403784439,0.));
#20759=DIRECTION('',(0.,0.,1.));
#20760=DIRECTION('center_axis',(0.,0.,1.));
#20761=DIRECTION('ref_axis',(-0.499999999999999,0.866025403784439,0.));
#20762=DIRECTION('',(0.,0.,1.));
#20763=DIRECTION('center_axis',(0.,0.,1.));
#20764=DIRECTION('ref_axis',(-0.499999999999999,0.866025403784439,0.));
#20765=DIRECTION('',(0.,0.,1.));
#20766=DIRECTION('center_axis',(0.,0.,1.));
#20767=DIRECTION('ref_axis',(-0.499999999999999,0.866025403784439,0.));
#20768=DIRECTION('',(0.,0.,1.));
#20769=DIRECTION('center_axis',(0.,0.,1.));
#20770=DIRECTION('ref_axis',(-0.499999999999999,0.866025403784439,0.));
#20771=DIRECTION('',(0.,0.,1.));
#20772=DIRECTION('center_axis',(0.,0.,1.));
#20773=DIRECTION('ref_axis',(-0.499999999999999,0.866025403784439,0.));
#20774=DIRECTION('',(0.,0.,1.));
#20775=DIRECTION('center_axis',(0.,0.,1.));
#20776=DIRECTION('ref_axis',(-0.499999999999999,0.866025403784439,0.));
#20777=DIRECTION('',(0.,0.,1.));
#20778=DIRECTION('center_axis',(0.,0.,1.));
#20779=DIRECTION('ref_axis',(-0.499999999999999,0.866025403784439,0.));
#20780=DIRECTION('',(0.,0.,1.));
#20781=DIRECTION('center_axis',(0.,0.,1.));
#20782=DIRECTION('ref_axis',(-0.499999999999999,0.866025403784439,0.));
#20783=DIRECTION('',(0.,0.,1.));
#20784=DIRECTION('center_axis',(0.,0.,1.));
#20785=DIRECTION('ref_axis',(-0.499999999999999,0.866025403784439,0.));
#20786=DIRECTION('',(0.,0.,1.));
#20787=DIRECTION('center_axis',(0.,0.,1.));
#20788=DIRECTION('ref_axis',(-0.768385143082287,0.639987712296426,0.));
#20789=DIRECTION('',(0.,0.,1.));
#20790=DIRECTION('center_axis',(0.,0.,-1.));
#20791=DIRECTION('ref_axis',(-0.499999999999999,0.866025403784439,0.));
#20792=DIRECTION('center_axis',(0.,0.,1.));
#20793=DIRECTION('ref_axis',(0.548243791989886,0.836318566423436,0.));
#20794=DIRECTION('',(-6.12323399573743E-17,1.06057523872487E-16,1.));
#20795=DIRECTION('center_axis',(0.,0.,-1.));
#20796=DIRECTION('ref_axis',(-0.500000000000054,0.866025403784408,0.));
#20797=DIRECTION('center_axis',(0.,0.,1.));
#20798=DIRECTION('ref_axis',(-0.500000000000054,0.866025403784408,0.));
#20799=DIRECTION('',(-6.12323399573743E-17,1.06057523872487E-16,1.));
#20800=DIRECTION('center_axis',(0.,0.,1.));
#20801=DIRECTION('ref_axis',(-0.500000000000054,0.866025403784408,0.));
#20802=DIRECTION('',(-6.12323399573743E-17,1.06057523872487E-16,1.));
#20803=DIRECTION('center_axis',(0.,0.,1.));
#20804=DIRECTION('ref_axis',(-0.500000000000054,0.866025403784408,0.));
#20805=DIRECTION('',(-6.12323399573743E-17,1.06057523872487E-16,1.));
#20806=DIRECTION('center_axis',(0.,0.,1.));
#20807=DIRECTION('ref_axis',(-0.500000000000054,0.866025403784408,0.));
#20808=DIRECTION('',(-6.12323399573743E-17,1.06057523872487E-16,1.));
#20809=DIRECTION('center_axis',(0.,0.,1.));
#20810=DIRECTION('ref_axis',(-0.500000000000054,0.866025403784408,0.));
#20811=DIRECTION('',(-6.12323399573743E-17,1.06057523872487E-16,1.));
#20812=DIRECTION('center_axis',(0.,0.,1.));
#20813=DIRECTION('ref_axis',(-0.500000000000054,0.866025403784408,0.));
#20814=DIRECTION('',(-6.12323399573743E-17,1.06057523872487E-16,1.));
#20815=DIRECTION('center_axis',(0.,0.,1.));
#20816=DIRECTION('ref_axis',(-0.500000000000054,0.866025403784408,0.));
#20817=DIRECTION('',(-6.12323399573743E-17,1.06057523872487E-16,1.));
#20818=DIRECTION('center_axis',(0.,0.,1.));
#20819=DIRECTION('ref_axis',(-0.500000000000054,0.866025403784408,0.));
#20820=DIRECTION('',(-6.12323399573743E-17,1.06057523872487E-16,1.));
#20821=DIRECTION('center_axis',(0.,0.,1.));
#20822=DIRECTION('ref_axis',(-0.500000000000054,0.866025403784408,0.));
#20823=DIRECTION('',(-6.12323399573743E-17,1.06057523872487E-16,1.));
#20824=DIRECTION('center_axis',(0.,0.,1.));
#20825=DIRECTION('ref_axis',(-0.500000000000054,0.866025403784408,0.));
#20826=DIRECTION('',(-6.12323399573743E-17,1.06057523872487E-16,1.));
#20827=DIRECTION('center_axis',(0.,0.,1.));
#20828=DIRECTION('ref_axis',(-0.500000000000054,0.866025403784408,0.));
#20829=DIRECTION('',(-6.12323399573743E-17,1.06057523872487E-16,1.));
#20830=DIRECTION('center_axis',(0.,0.,1.));
#20831=DIRECTION('ref_axis',(-0.382006426201385,-0.924159667125138,0.));
#20832=DIRECTION('',(-6.12323399573743E-17,1.06057523872487E-16,1.));
#20833=DIRECTION('center_axis',(0.,0.,1.));
#20834=DIRECTION('ref_axis',(-0.500000000000054,0.866025403784407,0.));
#20835=DIRECTION('center_axis',(-0.965925826289068,-0.258819045102521,3.59183578855394E-17));
#20836=DIRECTION('ref_axis',(0.0897739762313162,-0.335041040492753,0.937916912299353));
#20837=DIRECTION('',(-0.965925826289068,-0.258819045102521,3.59183578855394E-17));
#20838=DIRECTION('center_axis',(0.965925826289068,0.258819045102521,-3.59183578855394E-17));
#20839=DIRECTION('ref_axis',(-0.258819045102521,0.965925826289068,0.));
#20840=DIRECTION('center_axis',(-0.965925826289068,-0.258819045102521,3.59183578855394E-17));
#20841=DIRECTION('ref_axis',(-0.258819045102521,0.965925826289068,0.));
#20842=DIRECTION('',(-0.965925826289068,-0.258819045102521,3.59183578855394E-17));
#20843=DIRECTION('center_axis',(-0.965925826289068,-0.258819045102521,3.59183578855394E-17));
#20844=DIRECTION('ref_axis',(-0.258819045102521,0.965925826289068,0.));
#20845=DIRECTION('',(-0.965925826289068,-0.258819045102521,3.59183578855394E-17));
#20846=DIRECTION('center_axis',(-0.965925826289068,-0.258819045102521,3.59183578855394E-17));
#20847=DIRECTION('ref_axis',(-0.258819045102521,0.965925826289068,0.));
#20848=DIRECTION('',(-0.965925826289068,-0.258819045102521,3.59183578855394E-17));
#20849=DIRECTION('center_axis',(-0.965925826289068,-0.258819045102521,3.59183578855394E-17));
#20850=DIRECTION('ref_axis',(-0.258819045102521,0.965925826289068,0.));
#20851=DIRECTION('',(-0.965925826289068,-0.258819045102521,3.59183578855394E-17));
#20852=DIRECTION('center_axis',(-0.965925826289068,-0.258819045102521,3.59183578855394E-17));
#20853=DIRECTION('ref_axis',(-0.258819045102521,0.965925826289068,0.));
#20854=DIRECTION('',(-0.965925826289068,-0.258819045102521,3.59183578855394E-17));
#20855=DIRECTION('center_axis',(-0.965925826289068,-0.258819045102521,3.59183578855394E-17));
#20856=DIRECTION('ref_axis',(-0.258819045102521,0.965925826289068,0.));
#20857=DIRECTION('',(-0.965925826289068,-0.258819045102521,3.59183578855394E-17));
#20858=DIRECTION('center_axis',(-0.965925826289068,-0.258819045102521,3.59183578855394E-17));
#20859=DIRECTION('ref_axis',(-0.236559838638084,0.882853336827626,-0.405720874981618));
#20860=DIRECTION('',(-0.965925826289068,-0.258819045102521,3.59183578855394E-17));
#20861=DIRECTION('center_axis',(-0.965925826289068,-0.258819045102521,3.59183578855394E-17));
#20862=DIRECTION('ref_axis',(-0.205298336336054,0.766183821915523,0.608945764524699));
#20863=DIRECTION('',(-0.965925826289067,-0.258819045102527,3.59183578857433E-17));
#20864=DIRECTION('center_axis',(0.965925826289068,0.258819045102521,0.));
#20865=DIRECTION('ref_axis',(-0.25881904510252,0.965925826289069,-3.10652936774893E-14));
#20866=DIRECTION('center_axis',(-0.965925826289068,-0.258819045102521,3.59183578855394E-17));
#20867=DIRECTION('ref_axis',(-0.25881904510252,0.965925826289069,-3.10652936774893E-14));
#20868=DIRECTION('',(-0.965925826289067,-0.258819045102527,3.59183578857433E-17));
#20869=DIRECTION('center_axis',(-0.965925826289068,-0.258819045102521,3.59183578855394E-17));
#20870=DIRECTION('ref_axis',(-0.25881904510252,0.965925826289069,-3.10652936774893E-14));
#20871=DIRECTION('',(-0.965925826289067,-0.258819045102527,3.59183578857433E-17));
#20872=DIRECTION('center_axis',(-0.965925826289068,-0.258819045102521,3.59183578855394E-17));
#20873=DIRECTION('ref_axis',(-0.25881904510252,0.965925826289069,-3.10652936774893E-14));
#20874=DIRECTION('',(-0.965925826289067,-0.258819045102527,3.59183578857433E-17));
#20875=DIRECTION('center_axis',(-0.965925826289068,-0.258819045102521,3.59183578855394E-17));
#20876=DIRECTION('ref_axis',(-0.25881904510252,0.965925826289069,-3.10652936774893E-14));
#20877=DIRECTION('',(-0.965925826289067,-0.258819045102527,3.59183578857433E-17));
#20878=DIRECTION('center_axis',(-0.965925826289068,-0.258819045102521,3.59183578855394E-17));
#20879=DIRECTION('ref_axis',(-0.25881904510252,0.965925826289069,-3.10652936774893E-14));
#20880=DIRECTION('',(-0.965925826289067,-0.258819045102527,3.59183578857433E-17));
#20881=DIRECTION('center_axis',(-0.965925826289068,-0.258819045102521,3.59183578855394E-17));
#20882=DIRECTION('ref_axis',(-0.25881904510252,0.965925826289069,-3.10652936774893E-14));
#20883=DIRECTION('',(-0.965925826289067,-0.258819045102527,3.59183578857433E-17));
#20884=DIRECTION('center_axis',(-0.965925826289068,-0.258819045102521,3.59183578855394E-17));
#20885=DIRECTION('ref_axis',(0.16010022241081,-0.597502164340218,-0.785722013432718));
#20886=DIRECTION('',(-0.965925826289067,-0.258819045102527,3.59183578857433E-17));
#20887=DIRECTION('center_axis',(0.258819045102521,-0.965925826289068,3.59183578855394E-17));
#20888=DIRECTION('ref_axis',(0.335041040492769,0.0897739762313205,0.937916912299347));
#20889=DIRECTION('',(0.258819045102521,-0.965925826289068,3.59183578855394E-17));
#20890=DIRECTION('center_axis',(-0.258819045102521,0.965925826289068,-3.59183578855394E-17));
#20891=DIRECTION('ref_axis',(-0.965925826289068,-0.258819045102521,0.));
#20892=DIRECTION('center_axis',(0.258819045102521,-0.965925826289068,3.59183578855394E-17));
#20893=DIRECTION('ref_axis',(-0.965925826289068,-0.258819045102521,0.));
#20894=DIRECTION('',(0.258819045102521,-0.965925826289068,3.59183578855394E-17));
#20895=DIRECTION('center_axis',(0.258819045102521,-0.965925826289068,3.59183578855394E-17));
#20896=DIRECTION('ref_axis',(-0.965925826289068,-0.258819045102521,0.));
#20897=DIRECTION('',(0.258819045102521,-0.965925826289068,3.59183578855394E-17));
#20898=DIRECTION('center_axis',(0.258819045102521,-0.965925826289068,3.59183578855394E-17));
#20899=DIRECTION('ref_axis',(-0.965925826289068,-0.258819045102521,0.));
#20900=DIRECTION('',(0.258819045102521,-0.965925826289068,3.59183578855394E-17));
#20901=DIRECTION('center_axis',(0.258819045102521,-0.965925826289068,3.59183578855394E-17));
#20902=DIRECTION('ref_axis',(-0.965925826289068,-0.258819045102521,0.));
#20903=DIRECTION('',(0.258819045102521,-0.965925826289068,3.59183578855394E-17));
#20904=DIRECTION('center_axis',(0.258819045102521,-0.965925826289068,3.59183578855394E-17));
#20905=DIRECTION('ref_axis',(-0.965925826289068,-0.258819045102521,0.));
#20906=DIRECTION('',(0.258819045102521,-0.965925826289068,3.59183578855394E-17));
#20907=DIRECTION('center_axis',(0.258819045102521,-0.965925826289068,3.59183578855394E-17));
#20908=DIRECTION('ref_axis',(-0.965925826289068,-0.258819045102521,0.));
#20909=DIRECTION('',(0.258819045102521,-0.965925826289068,3.59183578855394E-17));
#20910=DIRECTION('center_axis',(0.258819045102521,-0.965925826289068,3.59183578855394E-17));
#20911=DIRECTION('ref_axis',(-0.882853336827661,-0.236559838638094,-0.405720874981536));
#20912=DIRECTION('',(0.258819045102521,-0.965925826289068,3.59183578855394E-17));
#20913=DIRECTION('center_axis',(0.965925826289068,0.258819045102521,3.59183578855394E-17));
#20914=DIRECTION('ref_axis',(-0.0897739762312974,0.335041040492683,0.93791691229938));
#20915=DIRECTION('',(0.965925826289068,0.258819045102521,3.59183578855394E-17));
#20916=DIRECTION('center_axis',(-0.965925826289068,-0.258819045102521,-3.59183578855394E-17));
#20917=DIRECTION('ref_axis',(0.258819045102521,-0.965925826289068,0.));
#20918=DIRECTION('center_axis',(0.965925826289068,0.258819045102521,3.59183578855394E-17));
#20919=DIRECTION('ref_axis',(0.258819045102521,-0.965925826289068,0.));
#20920=DIRECTION('',(0.965925826289068,0.258819045102521,3.59183578855394E-17));
#20921=DIRECTION('center_axis',(0.965925826289068,0.258819045102521,3.59183578855394E-17));
#20922=DIRECTION('ref_axis',(0.258819045102521,-0.965925826289068,0.));
#20923=DIRECTION('',(0.965925826289068,0.258819045102521,3.59183578855394E-17));
#20924=DIRECTION('center_axis',(0.965925826289068,0.258819045102521,3.59183578855394E-17));
#20925=DIRECTION('ref_axis',(0.258819045102521,-0.965925826289068,0.));
#20926=DIRECTION('',(0.965925826289068,0.258819045102521,3.59183578855394E-17));
#20927=DIRECTION('center_axis',(0.965925826289068,0.258819045102521,3.59183578855394E-17));
#20928=DIRECTION('ref_axis',(0.258819045102521,-0.965925826289068,0.));
#20929=DIRECTION('',(0.965925826289068,0.258819045102521,3.59183578855394E-17));
#20930=DIRECTION('center_axis',(0.965925826289068,0.258819045102521,3.59183578855394E-17));
#20931=DIRECTION('ref_axis',(0.258819045102521,-0.965925826289068,0.));
#20932=DIRECTION('',(0.965925826289068,0.258819045102521,3.59183578855394E-17));
#20933=DIRECTION('center_axis',(0.965925826289068,0.258819045102521,3.59183578855394E-17));
#20934=DIRECTION('ref_axis',(0.258819045102521,-0.965925826289068,0.));
#20935=DIRECTION('',(0.965925826289068,0.258819045102521,3.59183578855394E-17));
#20936=DIRECTION('center_axis',(0.965925826289068,0.258819045102521,3.59183578855394E-17));
#20937=DIRECTION('ref_axis',(0.236559838638087,-0.882853336827637,-0.405720874981593));
#20938=DIRECTION('',(0.965925826289068,0.258819045102521,3.59183578855394E-17));
#20939=DIRECTION('center_axis',(-0.258819045102521,0.965925826289068,3.59183578855394E-17));
#20940=DIRECTION('ref_axis',(-0.335041040492721,-0.0897739762313076,0.937916912299365));
#20941=DIRECTION('',(-0.258819045102521,0.965925826289068,3.59183578855394E-17));
#20942=DIRECTION('center_axis',(0.258819045102521,-0.965925826289068,-3.59183578855394E-17));
#20943=DIRECTION('ref_axis',(0.965925826289068,0.25881904510252,0.));
#20944=DIRECTION('center_axis',(-0.258819045102521,0.965925826289068,3.59183578855394E-17));
#20945=DIRECTION('ref_axis',(0.965925826289068,0.25881904510252,0.));
#20946=DIRECTION('',(-0.258819045102521,0.965925826289068,3.59183578855394E-17));
#20947=DIRECTION('center_axis',(-0.258819045102521,0.965925826289068,3.59183578855394E-17));
#20948=DIRECTION('ref_axis',(0.965925826289068,0.25881904510252,0.));
#20949=DIRECTION('',(-0.258819045102521,0.965925826289068,3.59183578855394E-17));
#20950=DIRECTION('center_axis',(-0.258819045102521,0.965925826289068,3.59183578855394E-17));
#20951=DIRECTION('ref_axis',(0.965925826289068,0.25881904510252,0.));
#20952=DIRECTION('',(-0.258819045102521,0.965925826289068,3.59183578855394E-17));
#20953=DIRECTION('center_axis',(-0.258819045102521,0.965925826289068,3.59183578855394E-17));
#20954=DIRECTION('ref_axis',(0.965925826289068,0.25881904510252,0.));
#20955=DIRECTION('',(-0.258819045102521,0.965925826289068,3.59183578855394E-17));
#20956=DIRECTION('center_axis',(-0.258819045102521,0.965925826289068,3.59183578855394E-17));
#20957=DIRECTION('ref_axis',(0.965925826289068,0.25881904510252,0.));
#20958=DIRECTION('',(-0.258819045102521,0.965925826289068,3.59183578855394E-17));
#20959=DIRECTION('center_axis',(-0.258819045102521,0.965925826289068,3.59183578855394E-17));
#20960=DIRECTION('ref_axis',(0.965925826289068,0.25881904510252,0.));
#20961=DIRECTION('',(-0.258819045102521,0.965925826289068,3.59183578855394E-17));
#20962=DIRECTION('center_axis',(-0.258819045102521,0.965925826289068,3.59183578855394E-17));
#20963=DIRECTION('ref_axis',(0.882853336827629,0.236559838638085,-0.40572087498161));
#20964=DIRECTION('',(-0.258819045102521,0.965925826289068,3.59183578855394E-17));
#20965=DIRECTION('center_axis',(0.258819045102521,-0.965925826289068,3.59183578855394E-17));
#20966=DIRECTION('ref_axis',(-0.766183821915484,-0.205298336336044,0.608945764524752));
#20967=DIRECTION('',(0.258819045102527,-0.965925826289067,3.59183578856725E-17));
#20968=DIRECTION('center_axis',(-0.258819045102521,0.965925826289068,0.));
#20969=DIRECTION('ref_axis',(-0.965925826289069,-0.25881904510252,-2.02285633248767E-14));
#20970=DIRECTION('center_axis',(0.258819045102521,-0.965925826289068,3.59183578855394E-17));
#20971=DIRECTION('ref_axis',(-0.965925826289069,-0.25881904510252,-2.02285633248767E-14));
#20972=DIRECTION('',(0.258819045102527,-0.965925826289067,3.59183578856725E-17));
#20973=DIRECTION('center_axis',(0.258819045102521,-0.965925826289068,3.59183578855394E-17));
#20974=DIRECTION('ref_axis',(-0.965925826289069,-0.25881904510252,-2.02285633248767E-14));
#20975=DIRECTION('',(0.258819045102527,-0.965925826289067,3.59183578856725E-17));
#20976=DIRECTION('center_axis',(0.258819045102521,-0.965925826289068,3.59183578855394E-17));
#20977=DIRECTION('ref_axis',(-0.965925826289069,-0.25881904510252,-2.02285633248767E-14));
#20978=DIRECTION('',(0.258819045102527,-0.965925826289067,3.59183578856725E-17));
#20979=DIRECTION('center_axis',(0.258819045102521,-0.965925826289068,3.59183578855394E-17));
#20980=DIRECTION('ref_axis',(-0.965925826289069,-0.25881904510252,-2.02285633248767E-14));
#20981=DIRECTION('',(0.258819045102527,-0.965925826289067,3.59183578856725E-17));
#20982=DIRECTION('center_axis',(0.258819045102521,-0.965925826289068,3.59183578855394E-17));
#20983=DIRECTION('ref_axis',(-0.965925826289069,-0.25881904510252,-2.02285633248767E-14));
#20984=DIRECTION('',(0.258819045102527,-0.965925826289067,3.59183578856725E-17));
#20985=DIRECTION('center_axis',(0.258819045102521,-0.965925826289068,3.59183578855394E-17));
#20986=DIRECTION('ref_axis',(-0.965925826289069,-0.25881904510252,-2.02285633248767E-14));
#20987=DIRECTION('',(0.258819045102527,-0.965925826289067,3.59183578856725E-17));
#20988=DIRECTION('center_axis',(0.258819045102521,-0.965925826289068,3.59183578855394E-17));
#20989=DIRECTION('ref_axis',(0.597502164340198,0.160100222410805,-0.785722013432735));
#20990=DIRECTION('',(0.258819045102527,-0.965925826289067,3.59183578856725E-17));
#20991=DIRECTION('center_axis',(0.965925826289068,0.258819045102521,3.59183578855394E-17));
#20992=DIRECTION('ref_axis',(0.205298336336062,-0.766183821915549,0.608945764524665));
#20993=DIRECTION('',(0.965925826289067,0.258819045102527,3.59183578857386E-17));
#20994=DIRECTION('center_axis',(-0.965925826289068,-0.258819045102521,0.));
#20995=DIRECTION('ref_axis',(0.25881904510252,-0.965925826289069,-3.03428449873152E-14));
#20996=DIRECTION('center_axis',(0.965925826289068,0.258819045102521,3.59183578855394E-17));
#20997=DIRECTION('ref_axis',(0.25881904510252,-0.965925826289069,-3.03428449873152E-14));
#20998=DIRECTION('',(0.965925826289067,0.258819045102527,3.59183578857386E-17));
#20999=DIRECTION('center_axis',(0.965925826289068,0.258819045102521,3.59183578855394E-17));
#21000=DIRECTION('ref_axis',(0.25881904510252,-0.965925826289069,-3.03428449873152E-14));
#21001=DIRECTION('',(0.965925826289067,0.258819045102527,3.59183578857386E-17));
#21002=DIRECTION('center_axis',(0.965925826289068,0.258819045102521,3.59183578855394E-17));
#21003=DIRECTION('ref_axis',(0.25881904510252,-0.965925826289069,-3.03428449873152E-14));
#21004=DIRECTION('',(0.965925826289067,0.258819045102527,3.59183578857386E-17));
#21005=DIRECTION('center_axis',(0.965925826289068,0.258819045102521,3.59183578855394E-17));
#21006=DIRECTION('ref_axis',(0.25881904510252,-0.965925826289069,-3.03428449873152E-14));
#21007=DIRECTION('',(0.965925826289067,0.258819045102527,3.59183578857386E-17));
#21008=DIRECTION('center_axis',(0.965925826289068,0.258819045102521,3.59183578855394E-17));
#21009=DIRECTION('ref_axis',(0.25881904510252,-0.965925826289069,-3.03428449873152E-14));
#21010=DIRECTION('',(0.965925826289067,0.258819045102527,3.59183578857386E-17));
#21011=DIRECTION('center_axis',(0.965925826289068,0.258819045102521,3.59183578855394E-17));
#21012=DIRECTION('ref_axis',(0.25881904510252,-0.965925826289069,-3.03428449873152E-14));
#21013=DIRECTION('',(0.965925826289067,0.258819045102527,3.59183578857386E-17));
#21014=DIRECTION('center_axis',(0.965925826289068,0.258819045102521,3.59183578855394E-17));
#21015=DIRECTION('ref_axis',(-0.16010022241082,0.597502164340256,-0.785722013432687));
#21016=DIRECTION('',(0.965925826289067,0.258819045102527,3.59183578857386E-17));
#21017=DIRECTION('center_axis',(-0.258819045102521,0.965925826289068,3.59183578855394E-17));
#21018=DIRECTION('ref_axis',(0.766183821915516,0.205298336336053,0.608945764524709));
#21019=DIRECTION('',(-0.258819045102527,0.965925826289067,3.59183578856961E-17));
#21020=DIRECTION('center_axis',(0.258819045102521,-0.965925826289068,0.));
#21021=DIRECTION('ref_axis',(0.965925826289069,0.25881904510252,-2.38408067757476E-14));
#21022=DIRECTION('center_axis',(-0.258819045102521,0.965925826289068,3.59183578855394E-17));
#21023=DIRECTION('ref_axis',(0.965925826289069,0.25881904510252,-2.38408067757476E-14));
#21024=DIRECTION('',(-0.258819045102527,0.965925826289067,3.59183578856961E-17));
#21025=DIRECTION('center_axis',(-0.258819045102521,0.965925826289068,3.59183578855394E-17));
#21026=DIRECTION('ref_axis',(0.965925826289069,0.25881904510252,-2.38408067757476E-14));
#21027=DIRECTION('',(-0.258819045102527,0.965925826289067,3.59183578856961E-17));
#21028=DIRECTION('center_axis',(-0.258819045102521,0.965925826289068,3.59183578855394E-17));
#21029=DIRECTION('ref_axis',(0.965925826289069,0.25881904510252,-2.38408067757476E-14));
#21030=DIRECTION('',(-0.258819045102527,0.965925826289067,3.59183578856961E-17));
#21031=DIRECTION('center_axis',(-0.258819045102521,0.965925826289068,3.59183578855394E-17));
#21032=DIRECTION('ref_axis',(0.965925826289069,0.25881904510252,-2.38408067757476E-14));
#21033=DIRECTION('',(-0.258819045102527,0.965925826289067,3.59183578856961E-17));
#21034=DIRECTION('center_axis',(-0.258819045102521,0.965925826289068,3.59183578855394E-17));
#21035=DIRECTION('ref_axis',(0.965925826289069,0.25881904510252,-2.38408067757476E-14));
#21036=DIRECTION('',(-0.258819045102527,0.965925826289067,3.59183578856961E-17));
#21037=DIRECTION('center_axis',(-0.258819045102521,0.965925826289068,3.59183578855394E-17));
#21038=DIRECTION('ref_axis',(0.965925826289069,0.25881904510252,-2.38408067757476E-14));
#21039=DIRECTION('',(-0.258819045102527,0.965925826289067,3.59183578856961E-17));
#21040=DIRECTION('center_axis',(-0.258819045102521,0.965925826289068,3.59183578855394E-17));
#21041=DIRECTION('ref_axis',(-0.597502164340203,-0.160100222410806,-0.78572201343273));
#21042=DIRECTION('',(-0.258819045102527,0.965925826289067,3.59183578856961E-17));
#21043=DIRECTION('center_axis',(-0.258819045102521,0.965925826289068,3.59183578855394E-17));
#21044=DIRECTION('ref_axis',(0.965925826289069,0.25881904510252,-2.38408067757476E-14));
#21045=DIRECTION('center_axis',(0.965925826289068,0.258819045102521,3.59183578855394E-17));
#21046=DIRECTION('ref_axis',(0.25881904510252,-0.965925826289069,-3.03428449873152E-14));
#21047=DIRECTION('center_axis',(0.258819045102521,-0.965925826289068,3.59183578855394E-17));
#21048=DIRECTION('ref_axis',(-0.965925826289069,-0.25881904510252,-2.02285633248767E-14));
#21049=DIRECTION('center_axis',(-0.258819045102521,0.965925826289068,3.59183578855394E-17));
#21050=DIRECTION('ref_axis',(0.965925826289068,0.25881904510252,0.));
#21051=DIRECTION('center_axis',(-0.258819045102521,0.965925826289068,3.59183578855394E-17));
#21052=DIRECTION('ref_axis',(0.965925826289068,0.25881904510252,0.));
#21053=DIRECTION('center_axis',(0.965925826289068,0.258819045102521,3.59183578855394E-17));
#21054=DIRECTION('ref_axis',(0.258819045102521,-0.965925826289068,0.));
#21055=DIRECTION('center_axis',(0.965925826289068,0.258819045102521,3.59183578855394E-17));
#21056=DIRECTION('ref_axis',(0.258819045102521,-0.965925826289068,0.));
#21057=DIRECTION('center_axis',(0.258819045102521,-0.965925826289068,3.59183578855394E-17));
#21058=DIRECTION('ref_axis',(-0.965925826289068,-0.258819045102521,0.));
#21059=DIRECTION('center_axis',(0.258819045102521,-0.965925826289068,3.59183578855394E-17));
#21060=DIRECTION('ref_axis',(-0.965925826289068,-0.258819045102521,0.));
#21061=DIRECTION('center_axis',(-0.965925826289068,-0.258819045102521,3.59183578855394E-17));
#21062=DIRECTION('ref_axis',(-0.25881904510252,0.965925826289069,-3.10652936774893E-14));
#21063=DIRECTION('center_axis',(-0.965925826289068,-0.258819045102521,3.59183578855394E-17));
#21064=DIRECTION('ref_axis',(-0.258819045102521,0.965925826289068,0.));
#21065=DIRECTION('center_axis',(-0.965925826289068,-0.258819045102521,3.59183578855394E-17));
#21066=DIRECTION('ref_axis',(-0.258819045102521,0.965925826289068,0.));
#21067=DIRECTION('center_axis',(0.,0.,1.));
#21068=DIRECTION('ref_axis',(1.,0.,0.));
#21069=DIRECTION('center_axis',(0.,0.,1.));
#21070=DIRECTION('ref_axis',(-0.500000000000054,0.866025403784408,0.));
#21071=DIRECTION('center_axis',(0.,0.,1.));
#21072=DIRECTION('ref_axis',(-0.499999999999999,0.866025403784439,0.));
#21073=DIRECTION('center_axis',(0.,0.,1.));
#21074=DIRECTION('ref_axis',(1.,0.,0.));
#21075=DIRECTION('center_axis',(0.,0.,1.));
#21076=DIRECTION('ref_axis',(0.499999999999942,0.866025403784472,0.));
#21077=DIRECTION('center_axis',(0.,0.,1.));
#21078=DIRECTION('ref_axis',(0.5,0.866025403784438,0.));
#21079=DIRECTION('center_axis',(0.,0.,1.));
#21080=DIRECTION('ref_axis',(1.,0.,0.));
#21081=DIRECTION('center_axis',(0.,0.,1.));
#21082=DIRECTION('ref_axis',(1.,4.99775456844331E-14,0.));
#21083=DIRECTION('center_axis',(0.,0.,1.));
#21084=DIRECTION('ref_axis',(1.,-1.38777878078145E-16,0.));
#21085=DIRECTION('center_axis',(0.,0.,1.));
#21086=DIRECTION('ref_axis',(1.,0.,0.));
#21087=DIRECTION('center_axis',(0.,0.,1.));
#21088=DIRECTION('ref_axis',(0.500000000000041,-0.866025403784415,0.));
#21089=DIRECTION('center_axis',(0.,0.,1.));
#21090=DIRECTION('ref_axis',(0.5,-0.866025403784439,0.));
#21091=DIRECTION('center_axis',(0.,0.,1.));
#21092=DIRECTION('ref_axis',(1.,0.,0.));
#21093=DIRECTION('center_axis',(0.,0.,1.));
#21094=DIRECTION('ref_axis',(-0.499999999999956,-0.866025403784464,0.));
#21095=DIRECTION('center_axis',(0.,0.,1.));
#21096=DIRECTION('ref_axis',(-0.5,-0.866025403784439,0.));
#21097=DIRECTION('center_axis',(0.,0.,1.));
#21098=DIRECTION('ref_axis',(-0.499999999999999,0.866025403784439,0.));
#21099=DIRECTION('center_axis',(0.,0.,1.));
#21100=DIRECTION('ref_axis',(0.5,0.866025403784438,0.));
#21101=DIRECTION('center_axis',(0.,0.,1.));
#21102=DIRECTION('ref_axis',(1.,-1.66533453693773E-16,0.));
#21103=DIRECTION('center_axis',(0.,0.,1.));
#21104=DIRECTION('ref_axis',(0.5,-0.866025403784439,0.));
#21105=DIRECTION('center_axis',(0.,0.,1.));
#21106=DIRECTION('ref_axis',(-0.5,-0.866025403784439,0.));
#21107=DIRECTION('center_axis',(0.,0.,1.));
#21108=DIRECTION('ref_axis',(1.,0.,0.));
#21109=DIRECTION('center_axis',(0.,0.,-1.));
#21110=DIRECTION('ref_axis',(0.499999999999945,-0.86602540378447,0.));
#21111=DIRECTION('center_axis',(0.,0.,-1.));
#21112=DIRECTION('ref_axis',(0.499999999999999,-0.866025403784439,0.));
#21113=DIRECTION('center_axis',(0.,0.,1.));
#21114=DIRECTION('ref_axis',(1.,0.,0.));
#21115=DIRECTION('center_axis',(0.,0.,-1.));
#21116=DIRECTION('ref_axis',(-0.500000000000056,-0.866025403784406,0.));
#21117=DIRECTION('center_axis',(0.,0.,-1.));
#21118=DIRECTION('ref_axis',(-0.5,-0.866025403784438,0.));
#21119=DIRECTION('center_axis',(0.,0.,1.));
#21120=DIRECTION('ref_axis',(1.,0.,0.));
#21121=DIRECTION('center_axis',(0.,0.,-1.));
#21122=DIRECTION('ref_axis',(-1.,6.27859183309933E-14,0.));
#21123=DIRECTION('center_axis',(0.,0.,-1.));
#21124=DIRECTION('ref_axis',(-1.,1.38777878078145E-16,0.));
#21125=DIRECTION('center_axis',(0.,0.,1.));
#21126=DIRECTION('ref_axis',(1.,0.,0.));
#21127=DIRECTION('center_axis',(0.,0.,-1.));
#21128=DIRECTION('ref_axis',(-0.499999999999944,0.866025403784471,0.));
#21129=DIRECTION('center_axis',(0.,0.,-1.));
#21130=DIRECTION('ref_axis',(-0.5,0.866025403784439,0.));
#21131=DIRECTION('center_axis',(0.,0.,1.));
#21132=DIRECTION('ref_axis',(1.,0.,0.));
#21133=DIRECTION('center_axis',(0.,0.,-1.));
#21134=DIRECTION('ref_axis',(0.500000000000052,0.866025403784408,0.));
#21135=DIRECTION('center_axis',(0.,0.,-1.));
#21136=DIRECTION('ref_axis',(0.5,0.866025403784439,0.));
#21137=DIRECTION('center_axis',(0.,0.,-1.));
#21138=DIRECTION('ref_axis',(0.499999999999999,-0.866025403784439,0.));
#21139=DIRECTION('center_axis',(0.,0.,-1.));
#21140=DIRECTION('ref_axis',(-0.5,-0.866025403784438,0.));
#21141=DIRECTION('center_axis',(0.,0.,-1.));
#21142=DIRECTION('ref_axis',(-1.,1.66533453693773E-16,0.));
#21143=DIRECTION('center_axis',(0.,0.,-1.));
#21144=DIRECTION('ref_axis',(-0.5,0.866025403784439,0.));
#21145=DIRECTION('center_axis',(0.,0.,-1.));
#21146=DIRECTION('ref_axis',(0.5,0.866025403784439,0.));
#21147=DIRECTION('center_axis',(0.,0.,1.));
#21148=DIRECTION('ref_axis',(1.,0.,0.));
#21149=DIRECTION('center_axis',(0.,0.,1.));
#21150=DIRECTION('ref_axis',(-1.,-5.01106501999328E-14,0.));
#21151=DIRECTION('center_axis',(0.,0.,1.));
#21152=DIRECTION('ref_axis',(-1.,0.,0.));
#21153=DIRECTION('center_axis',(0.,0.,1.));
#21154=DIRECTION('ref_axis',(-1.,0.,0.));
#21155=DIRECTION('center_axis',(0.,0.,1.));
#21156=DIRECTION('ref_axis',(1.,0.,0.));
#21157=DIRECTION('center_axis',(0.,0.,-1.));
#21158=DIRECTION('ref_axis',(1.,-6.25346187617716E-14,0.));
#21159=DIRECTION('center_axis',(0.,0.,-1.));
#21160=DIRECTION('ref_axis',(1.,0.,0.));
#21161=DIRECTION('center_axis',(0.,0.,-1.));
#21162=DIRECTION('ref_axis',(1.,0.,0.));
#21163=DIRECTION('center_axis',(0.,0.,1.));
#21164=DIRECTION('ref_axis',(1.,0.,0.));
#21165=DIRECTION('center_axis',(0.,0.,-1.));
#21166=DIRECTION('ref_axis',(1.,0.,0.));
#21167=DIRECTION('',(0.,0.,-1.));
#21168=DIRECTION('center_axis',(0.,0.,-1.));
#21169=DIRECTION('ref_axis',(1.,0.,0.));
#21170=DIRECTION('center_axis',(0.,0.,1.));
#21171=DIRECTION('ref_axis',(1.,0.,0.));
#21172=DIRECTION('center_axis',(0.,0.,1.));
#21173=DIRECTION('ref_axis',(1.,0.,0.));
#21174=DIRECTION('',(0.,0.,-1.));
#21175=DIRECTION('center_axis',(0.,0.,1.));
#21176=DIRECTION('ref_axis',(1.,0.,0.));
#21177=DIRECTION('center_axis',(0.,0.,1.));
#21178=DIRECTION('ref_axis',(1.,0.,0.));
#21179=DIRECTION('center_axis',(0.,0.,1.));
#21180=DIRECTION('ref_axis',(1.,0.,0.));
#23376=CARTESIAN_POINT('',(0.,0.,0.));
#23377=CARTESIAN_POINT('Origin',(65.,0.,17.));
#23378=CARTESIAN_POINT('',(63.3324486297716,-0.00121435961605691,13.8714803633902));
#23379=CARTESIAN_POINT('',(63.3320009243657,0.000968828099764776,13.6785196366098));
#23380=CARTESIAN_POINT('',(63.334,2.04026156737949E-16,17.));
#23381=CARTESIAN_POINT('',(63.3648706727485,-0.3192304546283,13.));
#23382=CARTESIAN_POINT('Ctrl Pts',(63.3320009243657,0.000968828099764776,
13.6785196366098));
#23383=CARTESIAN_POINT('Ctrl Pts',(63.3315933114009,0.059054876303456,13.6746222055426));
#23384=CARTESIAN_POINT('Ctrl Pts',(63.3343634348107,0.117102016123704,13.6707247744754));
#23385=CARTESIAN_POINT('Ctrl Pts',(63.3404396356832,0.174801282227228,13.6668273434083));
#23386=CARTESIAN_POINT('Ctrl Pts',(63.3981952988365,0.723245852641101,13.6297813798856));
#23387=CARTESIAN_POINT('Ctrl Pts',(63.7546528235523,1.24026026815388,13.5927354163629));
#23388=CARTESIAN_POINT('Ctrl Pts',(64.2467810781753,1.48913792445445,13.5556894528402));
#23389=CARTESIAN_POINT('Ctrl Pts',(64.7389093327983,1.73801558075501,13.5186434893175));
#23390=CARTESIAN_POINT('Ctrl Pts',(65.3667083173286,1.71875647784335,13.4815975257948));
#23391=CARTESIAN_POINT('Ctrl Pts',(65.8426564295865,1.44035726535855,13.4445515622722));
#23392=CARTESIAN_POINT('Ctrl Pts',(66.3186045418444,1.16195805287375,13.4075055987495));
#23393=CARTESIAN_POINT('Ctrl Pts',(66.6427017818299,0.624418730815826,13.3704596352268));
#23394=CARTESIAN_POINT('Ctrl Pts',(66.6670336186705,0.0733842827933222,
13.3334136717041));
#23395=CARTESIAN_POINT('Ctrl Pts',(66.691365455511,-0.477650165229181,13.2963677081814));
#23396=CARTESIAN_POINT('Ctrl Pts',(66.4159318892067,-1.04217973921626,13.2593217446588));
#23397=CARTESIAN_POINT('Ctrl Pts',(65.9659478490025,-1.36111593499208,13.2222757811361));
#23398=CARTESIAN_POINT('Ctrl Pts',(65.5159638087983,-1.6800521307679,13.1852298176134));
#23399=CARTESIAN_POINT('Ctrl Pts',(64.8914292946943,-1.75339494833247,13.1481838540907));
#23400=CARTESIAN_POINT('Ctrl Pts',(64.3801939409253,-1.54911937996348,13.111137890568));
#23401=CARTESIAN_POINT('Ctrl Pts',(63.8689585871564,-1.34484381159449,13.0740919270454));
#23402=CARTESIAN_POINT('Ctrl Pts',(63.4710223937224,-0.862949857291961,
13.0370459635227));
#23403=CARTESIAN_POINT('Ctrl Pts',(63.3648706727485,-0.319230454628348,
13.));
#23404=CARTESIAN_POINT('',(64.9474239245698,1.66819769235427,13.));
#23405=CARTESIAN_POINT('Origin',(65.,0.,13.));
#23406=CARTESIAN_POINT('',(63.3365558121435,-0.000651319618122093,13.1714803633902));
#23407=CARTESIAN_POINT('Ctrl Pts',(64.9474239513002,1.66819938802347,13.));
#23408=CARTESIAN_POINT('Ctrl Pts',(64.4069183000551,1.6504713908779,13.0363229181856));
#23409=CARTESIAN_POINT('Ctrl Pts',(63.874833765777,1.34577267304803,13.0726458363711));
#23410=CARTESIAN_POINT('Ctrl Pts',(63.5871509129382,0.887831743084597,13.1089687545567));
#23411=CARTESIAN_POINT('Ctrl Pts',(63.42211720178,0.625126856723245,13.1298059575012));
#23412=CARTESIAN_POINT('Ctrl Pts',(63.3375141386089,0.311991178117364,13.1506431604457));
#23413=CARTESIAN_POINT('Ctrl Pts',(63.3365558121435,-0.000651319618122093,
13.1714803633902));
#23414=CARTESIAN_POINT('',(63.334,-2.04026156737949E-16,12.));
#23415=CARTESIAN_POINT('',(63.334,2.04026156737949E-16,17.));
#23416=CARTESIAN_POINT('Origin',(65.,0.,12.));
#23417=CARTESIAN_POINT('Ctrl Pts',(63.3365558121435,-0.000651319618122093,
13.1714803633902));
#23418=CARTESIAN_POINT('Ctrl Pts',(63.3358103529628,-0.243848422696125,
13.1876891239684));
#23419=CARTESIAN_POINT('Ctrl Pts',(63.385677580256,-0.486747106414449,13.2038978845465));
#23420=CARTESIAN_POINT('Ctrl Pts',(63.4876703201545,-0.7053781763955,13.2201066451247));
#23421=CARTESIAN_POINT('Ctrl Pts',(63.7207800205315,-1.20507083360908,13.2571526086474));
#23422=CARTESIAN_POINT('Ctrl Pts',(64.2261802362228,-1.57799560462435,13.2941985721701));
#23423=CARTESIAN_POINT('Ctrl Pts',(64.7725065735009,-1.65321436231664,13.3312445356927));
#23424=CARTESIAN_POINT('Ctrl Pts',(65.318832910779,-1.72843312000893,13.3682904992154));
#23425=CARTESIAN_POINT('Ctrl Pts',(65.906085369644,-1.50594586437824,13.4053364627381));
#23426=CARTESIAN_POINT('Ctrl Pts',(66.265537296365,-1.08770963232589,13.4423824262608));
#23427=CARTESIAN_POINT('Ctrl Pts',(66.6249892230859,-0.669473400273535,
13.4794283897835));
#23428=CARTESIAN_POINT('Ctrl Pts',(66.7566406176629,-0.0554881917995138,
13.5164743533061));
#23429=CARTESIAN_POINT('Ctrl Pts',(66.6002239654009,0.47331994937011,13.5535203168288));
#23430=CARTESIAN_POINT('Ctrl Pts',(66.4438073131388,1.00212809053973,13.5905662803515));
#23431=CARTESIAN_POINT('Ctrl Pts',(65.9993226140377,1.44575916440496,13.6276122438742));
#23432=CARTESIAN_POINT('Ctrl Pts',(65.470199129815,1.60114874218549,13.6646582073969));
#23433=CARTESIAN_POINT('Ctrl Pts',(64.9410756455923,1.75653831996602,13.7017041709195));
#23434=CARTESIAN_POINT('Ctrl Pts',(64.327313376248,1.62368640166186,13.7387501344422));
#23435=CARTESIAN_POINT('Ctrl Pts',(63.9097999122987,1.26341063241475,13.7757960979649));
#23436=CARTESIAN_POINT('Ctrl Pts',(63.550341325322,0.953230889441892,13.8076908531067));
#23437=CARTESIAN_POINT('Ctrl Pts',(63.3363495020968,0.474476303274697,13.8395856082484));
#23438=CARTESIAN_POINT('Ctrl Pts',(63.3324486297716,-0.00121435961605691,
13.8714803633902));
#23439=CARTESIAN_POINT('Origin',(65.,0.,17.));
#23440=CARTESIAN_POINT('',(63.3327604959513,0.00132477262097364,14.5714803633902));
#23441=CARTESIAN_POINT('',(63.3362968330887,0.000832304224862905,14.3785196366098));
#23442=CARTESIAN_POINT('',(63.334,2.04026156737949E-16,17.));
#23443=CARTESIAN_POINT('Ctrl Pts',(63.3362968330887,0.000832304224862905,
14.3785196366098));
#23444=CARTESIAN_POINT('Ctrl Pts',(63.3352820110227,0.225194784962812,14.3635646533454));
#23445=CARTESIAN_POINT('Ctrl Pts',(63.3774911908197,0.449191325190215,14.3486096700809));
#23446=CARTESIAN_POINT('Ctrl Pts',(63.4647380475121,0.65400242785626,14.3336546868165));
#23447=CARTESIAN_POINT('Ctrl Pts',(63.6808629212981,1.16135335592135,14.2966087232938));
#23448=CARTESIAN_POINT('Ctrl Pts',(64.1733546191173,1.55097577727799,14.2595627597711));
#23449=CARTESIAN_POINT('Ctrl Pts',(64.7168232236993,1.64455527160813,14.2225167962485));
#23450=CARTESIAN_POINT('Ctrl Pts',(65.2602918282814,1.73813476593827,14.1854708327258));
#23451=CARTESIAN_POINT('Ctrl Pts',(65.8547373396264,1.53567133324193,14.1484248692031));
#23452=CARTESIAN_POINT('Ctrl Pts',(66.2281050246363,1.12982650677502,14.1113789056804));
#23453=CARTESIAN_POINT('Ctrl Pts',(66.6014727096463,0.723981680308096,14.0743329421577));
#23454=CARTESIAN_POINT('Ctrl Pts',(66.7537625683213,0.114755460070602,14.0372869786351));
#23455=CARTESIAN_POINT('Ctrl Pts',(66.6152849767096,-0.419042261543969,
14.0002410151124));
#23456=CARTESIAN_POINT('Ctrl Pts',(66.4768073850979,-0.952839983158524,
13.9631950515897));
#23457=CARTESIAN_POINT('Ctrl Pts',(66.0475623431996,-1.41120920615016,13.926149088067));
#23458=CARTESIAN_POINT('Ctrl Pts',(65.5239830002582,-1.58436286925844,13.8891031245443));
#23459=CARTESIAN_POINT('Ctrl Pts',(65.0004036573169,-1.75751653236671,13.8520571610217));
#23460=CARTESIAN_POINT('Ctrl Pts',(64.3824900133324,-1.64545463559162,13.815011197499));
#23461=CARTESIAN_POINT('Ctrl Pts',(63.9530600921357,-1.29948632454661,13.7779652339763));
#23462=CARTESIAN_POINT('Ctrl Pts',(63.5688084672201,-0.989915707487894,
13.7448167015208));
#23463=CARTESIAN_POINT('Ctrl Pts',(63.3354677647952,-0.493066145425912,
13.7116681690653));
#23464=CARTESIAN_POINT('Ctrl Pts',(63.3320009243657,0.000968828099764776,
13.6785196366098));
#23465=CARTESIAN_POINT('Ctrl Pts',(63.3324486297716,-0.00121435961605691,
13.8714803633902));
#23466=CARTESIAN_POINT('Ctrl Pts',(63.3318186137667,-0.0780414654682614,
13.8766315717711));
#23467=CARTESIAN_POINT('Ctrl Pts',(63.3366686795385,-0.154788650933411,
13.881782780152));
#23468=CARTESIAN_POINT('Ctrl Pts',(63.3472710750459,-0.230732838385404,
13.8869339885329));
#23469=CARTESIAN_POINT('Ctrl Pts',(63.4235203602966,-0.776900919748414,
13.9239799520556));
#23470=CARTESIAN_POINT('Ctrl Pts',(63.7972835893523,-1.28153746228441,13.9610259155783));
#23471=CARTESIAN_POINT('Ctrl Pts',(64.2975048362999,-1.51368831950505,13.998071879101));
#23472=CARTESIAN_POINT('Ctrl Pts',(64.7977260832475,-1.7458391767257,14.0351178426237));
#23473=CARTESIAN_POINT('Ctrl Pts',(65.424405348087,-1.70550434863098,14.0721638061464));
#23474=CARTESIAN_POINT('Ctrl Pts',(65.8907398483472,-1.41114550098828,14.109209769669));
#23475=CARTESIAN_POINT('Ctrl Pts',(66.3570743486074,-1.1167866533456,14.1462557331917));
#23476=CARTESIAN_POINT('Ctrl Pts',(66.6630640842882,-0.568403786154937,
14.1833016967144));
#23477=CARTESIAN_POINT('Ctrl Pts',(66.6686708473517,-0.0169663179122549,
14.2203476602371));
#23478=CARTESIAN_POINT('Ctrl Pts',(66.6742776104151,0.534471150330427,14.2573936237598));
#23479=CARTESIAN_POINT('Ctrl Pts',(66.3795014008612,1.08896321962513,14.2944395872824));
#23480=CARTESIAN_POINT('Ctrl Pts',(65.9192483587705,1.39274289076842,14.3314855508051));
#23481=CARTESIAN_POINT('Ctrl Pts',(65.4589953166798,1.69652256191171,14.3685315143278));
#23482=CARTESIAN_POINT('Ctrl Pts',(64.8332654420522,1.74958983490358,14.4055774778505));
#23483=CARTESIAN_POINT('Ctrl Pts',(64.3284274914591,1.52765845331761,14.4426234413732));
#23484=CARTESIAN_POINT('Ctrl Pts',(63.823589540866,1.30572707173164,14.4796694048958));
#23485=CARTESIAN_POINT('Ctrl Pts',(63.4396435143075,0.808797035567841,14.5167153684185));
#23486=CARTESIAN_POINT('Ctrl Pts',(63.352304522573,0.264291051559231,14.5537613319412));
#23487=CARTESIAN_POINT('Ctrl Pts',(63.3383798175659,0.177478906704716,14.5596676757575));
#23488=CARTESIAN_POINT('Ctrl Pts',(63.3319945181308,0.0894574366348187,
14.5655740195739));
#23489=CARTESIAN_POINT('Ctrl Pts',(63.3327604959513,0.00132477262097364,
14.5714803633902));
#23490=CARTESIAN_POINT('Origin',(65.,0.,17.));
#23491=CARTESIAN_POINT('',(63.3366282199437,0.000380246208316198,15.2714803633902));
#23492=CARTESIAN_POINT('',(63.3350218272016,-0.00143128727516526,15.0785196366098));
#23493=CARTESIAN_POINT('',(63.334,2.04026156737949E-16,17.));
#23494=CARTESIAN_POINT('Ctrl Pts',(63.3350218272016,-0.00143128727516526,
15.0785196366098));
#23495=CARTESIAN_POINT('Ctrl Pts',(63.3382129761596,0.388071089145999,15.0525071011481));
#23496=CARTESIAN_POINT('Ctrl Pts',(63.4745702784036,0.77958633576253,15.0264945656864));
#23497=CARTESIAN_POINT('Ctrl Pts',(63.7241632245643,1.07563467970709,15.0004820302248));
#23498=CARTESIAN_POINT('Ctrl Pts',(64.0796230447962,1.49725433177356,14.9634360667021));
#23499=CARTESIAN_POINT('Ctrl Pts',(64.6647503809125,1.72524549701854,14.9263901031794));
#23500=CARTESIAN_POINT('Ctrl Pts',(65.2117584175496,1.65526670109563,14.8893441396567));
#23501=CARTESIAN_POINT('Ctrl Pts',(65.7587664541868,1.58528790517272,14.852298176134));
#23502=CARTESIAN_POINT('Ctrl Pts',(66.2676551913447,1.21733914808192,14.8152522126113));
#23503=CARTESIAN_POINT('Ctrl Pts',(66.5055287575052,0.719814314063385,14.7782062490887));
#23504=CARTESIAN_POINT('Ctrl Pts',(66.7434023236657,0.222289480044847,14.741160285566));
#23505=CARTESIAN_POINT('Ctrl Pts',(66.7102607188288,-0.40481143090143,14.7041143220433));
#23506=CARTESIAN_POINT('Ctrl Pts',(66.4212714962,-0.874492228471354,14.6670683585206));
#23507=CARTESIAN_POINT('Ctrl Pts',(66.1322822735712,-1.34417302604128,14.630022394998));
#23508=CARTESIAN_POINT('Ctrl Pts',(65.5874454331506,-1.65643371023485,14.5929764314753));
#23509=CARTESIAN_POINT('Ctrl Pts',(65.0361084265221,-1.66836621488623,14.5559304679526));
#23510=CARTESIAN_POINT('Ctrl Pts',(64.4847714198936,-1.6802987195376,14.5188845044299));
#23511=CARTESIAN_POINT('Ctrl Pts',(63.9269342470572,-1.39190304464678,14.4818385409072));
#23512=CARTESIAN_POINT('Ctrl Pts',(63.6178946855153,-0.935165489814587,
14.4447925773845));
#23513=CARTESIAN_POINT('Ctrl Pts',(63.4336104557676,-0.662807064022192,
14.4227015971263));
#23514=CARTESIAN_POINT('Ctrl Pts',(63.3377958928888,-0.330588135707226,
14.400610616868));
#23515=CARTESIAN_POINT('Ctrl Pts',(63.3362968330887,0.000832304224862905,
14.3785196366098));
#23516=CARTESIAN_POINT('Ctrl Pts',(63.3327604959513,0.00132477262097364,
14.5714803633902));
#23517=CARTESIAN_POINT('Ctrl Pts',(63.336798909355,-0.463331150982518,14.6026199830965));
#23518=CARTESIAN_POINT('Ctrl Pts',(63.5396173640042,-0.931077870254258,
14.6337596028029));
#23519=CARTESIAN_POINT('Ctrl Pts',(63.8843359278475,-1.24098501894124,14.6648992225092));
#23520=CARTESIAN_POINT('Ctrl Pts',(64.294438281767,-1.60967317357969,14.7019451860319));
#23521=CARTESIAN_POINT('Ctrl Pts',(64.9053749465165,-1.75496755100317,14.7389911495546));
#23522=CARTESIAN_POINT('Ctrl Pts',(65.4375473020178,-1.61037339159949,14.7760371130773));
#23523=CARTESIAN_POINT('Ctrl Pts',(65.9697196575191,-1.46577923219581,14.8130830766));
#23524=CARTESIAN_POINT('Ctrl Pts',(66.4231277037722,-1.03129653596498,14.8501290401226));
#23525=CARTESIAN_POINT('Ctrl Pts',(66.5902666729806,-0.505768754333085,
14.8871750036453));
#23526=CARTESIAN_POINT('Ctrl Pts',(66.757405642189,0.0197590272988233,14.924220967168));
#23527=CARTESIAN_POINT('Ctrl Pts',(66.6382755343526,0.636331894331814,14.9612669306907));
#23528=CARTESIAN_POINT('Ctrl Pts',(66.2873969210692,1.06177176879601,14.9983128942134));
#23529=CARTESIAN_POINT('Ctrl Pts',(65.9365183077858,1.4872116432602,15.0353588577361));
#23530=CARTESIAN_POINT('Ctrl Pts',(65.3538911890554,1.7215185251556,15.0724048212587));
#23531=CARTESIAN_POINT('Ctrl Pts',(64.8061581683602,1.65746054599185,15.1094507847814));
#23532=CARTESIAN_POINT('Ctrl Pts',(64.2584251476649,1.5934025668281,15.1464967483041));
#23533=CARTESIAN_POINT('Ctrl Pts',(63.7455862250048,1.23097972660522,15.1835427118268));
#23534=CARTESIAN_POINT('Ctrl Pts',(63.5023450418969,0.736056890900436,15.2205886753495));
#23535=CARTESIAN_POINT('Ctrl Pts',(63.390961297378,0.509424385728741,15.237552571363));
#23536=CARTESIAN_POINT('Ctrl Pts',(63.336108421692,0.255008487872148,15.2545164673766));
#23537=CARTESIAN_POINT('Ctrl Pts',(63.3366282199437,0.000380246208316198,
15.2714803633902));
#23538=CARTESIAN_POINT('Origin',(65.,0.,17.));
#23539=CARTESIAN_POINT('',(63.3341549687971,-0.00152342623458264,15.9714803633902));
#23540=CARTESIAN_POINT('',(63.3312431600774,6.71117920464596E-6,15.7785196366098));
#23541=CARTESIAN_POINT('',(63.334,2.04026156737949E-16,17.));
#23542=CARTESIAN_POINT('Ctrl Pts',(63.3312431738575,6.7111456588167E-6,
15.7785196366098));
#23543=CARTESIAN_POINT('Ctrl Pts',(63.3312102147262,0.551831913054104,15.7414495489509));
#23544=CARTESIAN_POINT('Ctrl Pts',(63.6320564203023,1.10362622346454,15.7043794612919));
#23545=CARTESIAN_POINT('Ctrl Pts',(64.0958701387024,1.4026042396328,15.667309373633));
#23546=CARTESIAN_POINT('Ctrl Pts',(64.5593820206073,1.70138768959276,15.6302634101103));
#23547=CARTESIAN_POINT('Ctrl Pts',(65.1856492588609,1.74768378931892,15.5932174465876));
#23548=CARTESIAN_POINT('Ctrl Pts',(65.6880571011576,1.52030486584838,15.556171483065));
#23549=CARTESIAN_POINT('Ctrl Pts',(66.1904649434542,1.29292594237784,15.5191255195423));
#23550=CARTESIAN_POINT('Ctrl Pts',(66.569013389794,0.791871995710604,15.4820795560196));
#23551=CARTESIAN_POINT('Ctrl Pts',(66.6504575962853,0.246453206514432,15.4450335924969));
#23552=CARTESIAN_POINT('Ctrl Pts',(66.7319018027767,-0.29896558268174,15.4079876289742));
#23553=CARTESIAN_POINT('Ctrl Pts',(66.5162417694196,-0.888749214406839,
15.3709416654516));
#23554=CARTESIAN_POINT('Ctrl Pts',(66.1021755351577,-1.25297986690093,15.3338957019289));
#23555=CARTESIAN_POINT('Ctrl Pts',(65.6881093008957,-1.61721051939501,15.2968497384062));
#23556=CARTESIAN_POINT('Ctrl Pts',(65.0756368657288,-1.75588819265809,15.2598037748835));
#23557=CARTESIAN_POINT('Ctrl Pts',(64.5450597089912,-1.60554625999198,15.2227578113608));
#23558=CARTESIAN_POINT('Ctrl Pts',(64.0144825522536,-1.45520432732587,15.1857118478382));
#23559=CARTESIAN_POINT('Ctrl Pts',(63.5658006739452,-1.01584278873058,15.1486658843155));
#23560=CARTESIAN_POINT('Ctrl Pts',(63.4043558869649,-0.488537949988941,
15.1116199207928));
#23561=CARTESIAN_POINT('Ctrl Pts',(63.3562726607889,-0.331490340715363,
15.1005864927318));
#23562=CARTESIAN_POINT('Ctrl Pts',(63.3336682754684,-0.166641881842641,
15.0895530646708));
#23563=CARTESIAN_POINT('Ctrl Pts',(63.3350218272016,-0.00143128727516526,
15.0785196366098));
#23564=CARTESIAN_POINT('Ctrl Pts',(63.3366282199437,0.000380246208316198,
15.2714803633902));
#23565=CARTESIAN_POINT('Ctrl Pts',(63.3372435634692,-0.301051779472626,
15.2915624308993));
#23566=CARTESIAN_POINT('Ctrl Pts',(63.4154588028067,-0.602781386183098,
15.3116444984084));
#23567=CARTESIAN_POINT('Ctrl Pts',(63.5693524834351,-0.859067985064377,
15.3317265659175));
#23568=CARTESIAN_POINT('Ctrl Pts',(63.8532445516371,-1.3318471941377,15.3687725294402));
#23569=CARTESIAN_POINT('Ctrl Pts',(64.3946721315968,-1.64998278109766,15.4058184929629));
#23570=CARTESIAN_POINT('Ctrl Pts',(64.9458478213867,-1.66787819121184,15.4428644564855));
#23571=CARTESIAN_POINT('Ctrl Pts',(65.4970235111765,-1.68577360132601,15.4799104200082));
#23572=CARTESIAN_POINT('Ctrl Pts',(66.0579473107965,-1.40342883459439,15.5169563835309));
#23573=CARTESIAN_POINT('Ctrl Pts',(66.3719092626235,-0.950060574217453,
15.5540023470536));
#23574=CARTESIAN_POINT('Ctrl Pts',(66.6858712144506,-0.496692313840509,
15.5910483105763));
#23575=CARTESIAN_POINT('Ctrl Pts',(66.7528713184848,0.127699440181754,15.6280942740989));
#23576=CARTESIAN_POINT('Ctrl Pts',(66.542246597235,0.637358260928835,15.6651402376216));
#23577=CARTESIAN_POINT('Ctrl Pts',(66.3316218759853,1.14701708167591,15.7021862011443));
#23578=CARTESIAN_POINT('Ctrl Pts',(65.8433723294516,1.54194296914781,15.739232164667));
#23579=CARTESIAN_POINT('Ctrl Pts',(65.3009481311498,1.64139585163659,15.7762781281897));
#23580=CARTESIAN_POINT('Ctrl Pts',(64.7585239328481,1.74084873412538,15.8133240917123));
#23581=CARTESIAN_POINT('Ctrl Pts',(64.1619250827784,1.54482861163106,15.850370055235));
#23582=CARTESIAN_POINT('Ctrl Pts',(63.7841884276299,1.14304520468472,15.8874160187577));
#23583=CARTESIAN_POINT('Ctrl Pts',(63.4984696309493,0.839137521926606,15.9154374669685));
#23584=CARTESIAN_POINT('Ctrl Pts',(63.3379698006251,0.417505232584558,15.9434589151794));
#23585=CARTESIAN_POINT('Ctrl Pts',(63.3341549687971,-0.00152342623458264,
15.9714803633902));
#23586=CARTESIAN_POINT('Origin',(65.,0.,17.));
#23587=CARTESIAN_POINT('',(63.3314647116295,0.000550350488423834,16.6714803633902));
#23588=CARTESIAN_POINT('',(63.3350414063796,0.00142706819227928,16.4785196366098));
#23589=CARTESIAN_POINT('',(63.334,2.04026156737949E-16,17.));
#23590=CARTESIAN_POINT('Ctrl Pts',(63.3350414063796,0.00142706819227928,
16.4785196366098));
#23591=CARTESIAN_POINT('Ctrl Pts',(63.3336871074336,0.167365053879281,16.4674379602763));
#23592=CARTESIAN_POINT('Ctrl Pts',(63.3564935743301,0.33293915311042,16.4563562839428));
#23593=CARTESIAN_POINT('Ctrl Pts',(63.4049919569221,0.490610641878083,16.4452746076093));
#23594=CARTESIAN_POINT('Ctrl Pts',(63.5671216977971,1.0177052840304,16.4082286440866));
#23595=CARTESIAN_POINT('Ctrl Pts',(64.0163740234165,1.45648350908886,16.3711826805639));
#23596=CARTESIAN_POINT('Ctrl Pts',(64.5471460595228,1.60613597431706,16.3341367170413));
#23597=CARTESIAN_POINT('Ctrl Pts',(65.0779180956292,1.75578843954526,16.2970907535186));
#23598=CARTESIAN_POINT('Ctrl Pts',(65.6902098422225,1.61631514494319,16.2600447899959));
#23599=CARTESIAN_POINT('Ctrl Pts',(66.1038025095515,1.2515468346462,16.2229988264732));
#23600=CARTESIAN_POINT('Ctrl Pts',(66.5173951768805,0.886778524349212,16.1859528629505));
#23601=CARTESIAN_POINT('Ctrl Pts',(66.7322887649452,0.296715198357295,16.1489068994279));
#23602=CARTESIAN_POINT('Ctrl Pts',(66.6501360046234,-0.248597316289489,
16.1118609359052));
#23603=CARTESIAN_POINT('Ctrl Pts',(66.5679832443015,-0.793909830936272,
16.0748149723825));
#23604=CARTESIAN_POINT('Ctrl Pts',(66.1887841355932,-1.29447153423793,16.0377690088598));
#23605=CARTESIAN_POINT('Ctrl Pts',(65.6860813008334,-1.52119752432679,16.0007230453371));
#23606=CARTESIAN_POINT('Ctrl Pts',(65.1833784660736,-1.74792351441565,15.9636770818144));
#23607=CARTESIAN_POINT('Ctrl Pts',(64.5571719052625,-1.70081379129173,15.9266311182918));
#23608=CARTESIAN_POINT('Ctrl Pts',(64.0940486017292,-1.40142838682091,15.8895851547691));
#23609=CARTESIAN_POINT('Ctrl Pts',(63.6312268816509,-1.10223794054801,15.8525633153827));
#23610=CARTESIAN_POINT('Ctrl Pts',(63.3312760900911,-0.551100267138433,
15.8155414759962));
#23611=CARTESIAN_POINT('Ctrl Pts',(63.3312431738575,6.7111456588167E-6,
15.7785196366098));
#23612=CARTESIAN_POINT('Ctrl Pts',(63.3341549687971,-0.00152342623458264,
15.9714803633902));
#23613=CARTESIAN_POINT('Ctrl Pts',(63.3329263739013,-0.136474714946136,
15.980504878702));
#23614=CARTESIAN_POINT('Ctrl Pts',(63.3479493008663,-0.271155952543882,
15.9895293940139));
#23615=CARTESIAN_POINT('Ctrl Pts',(63.3802748445461,-0.401547681148703,
15.9985539093257));
#23616=CARTESIAN_POINT('Ctrl Pts',(63.5129723768379,-0.936810468637373,
16.0355998728484));
#23617=CARTESIAN_POINT('Ctrl Pts',(63.9372419016487,-1.39978935221634,16.0726458363711));
#23618=CARTESIAN_POINT('Ctrl Pts',(64.4589140651794,-1.57859942055654,16.1096917998938));
#23619=CARTESIAN_POINT('Ctrl Pts',(64.9805862287101,-1.75740948889674,16.1467377634165));
#23620=CARTESIAN_POINT('Ctrl Pts',(65.5996610309607,-1.65205074199818,16.1837837269391));
#23621=CARTESIAN_POINT('Ctrl Pts',(66.0328153782871,-1.31074120779883,16.2208296904618));
#23622=CARTESIAN_POINT('Ctrl Pts',(66.4659697256135,-0.969431673599482,
16.2578756539845));
#23623=CARTESIAN_POINT('Ctrl Pts',(66.7132036180157,-0.392171352099344,
16.2949216175072));
#23624=CARTESIAN_POINT('Ctrl Pts',(66.661369062725,0.156853297275929,16.3319675810299));
#23625=CARTESIAN_POINT('Ctrl Pts',(66.6095345074342,0.705877946651205,16.3690135445526));
#23626=CARTESIAN_POINT('Ctrl Pts',(66.2586315044505,1.22666692390161,16.4060595080752));
#23627=CARTESIAN_POINT('Ctrl Pts',(65.7692528028443,1.48087820051541,16.4431054715979));
#23628=CARTESIAN_POINT('Ctrl Pts',(65.2798741012382,1.73508947712919,16.4801514351206));
#23629=CARTESIAN_POINT('Ctrl Pts',(64.6520197010096,1.72272305310636,16.5171973986433));
#23630=CARTESIAN_POINT('Ctrl Pts',(64.1730307286,1.44943849252272,16.5542433621659));
#23631=CARTESIAN_POINT('Ctrl Pts',(63.6940417561904,1.17615393193908,16.5912893256886));
#23632=CARTESIAN_POINT('Ctrl Pts',(63.3639182115997,0.641951234794639,16.6283352892113));
#23633=CARTESIAN_POINT('Ctrl Pts',(63.3337430069376,0.0913112945731737,
16.665381252734));
#23634=CARTESIAN_POINT('Ctrl Pts',(63.3320870288426,0.0610928523301667,
16.6674142896194));
#23635=CARTESIAN_POINT('Ctrl Pts',(63.3313343989597,0.0308249063821219,
16.6694473265048));
#23636=CARTESIAN_POINT('Ctrl Pts',(63.3314647116295,0.000550350488423834,
16.6714803633902));
#23637=CARTESIAN_POINT('Origin',(65.,0.,17.));
#23638=CARTESIAN_POINT('',(63.3357797744869,0.00117646094453,17.3714803633902));
#23639=CARTESIAN_POINT('',(63.3362856132907,-0.000842509924175838,17.1785196366098));
#23640=CARTESIAN_POINT('',(63.334,2.04026156737949E-16,17.));
#23641=CARTESIAN_POINT('Ctrl Pts',(63.3362856132907,-0.000842509924175838,
17.1785196366098));
#23642=CARTESIAN_POINT('Ctrl Pts',(63.3378066597351,0.331296382409458,17.156380408079));
#23643=CARTESIAN_POINT('Ctrl Pts',(63.4340697022003,0.664247316775266,17.1342411795483));
#23644=CARTESIAN_POINT('Ctrl Pts',(63.6191109651628,0.936960475618686,17.1121019510176));
#23645=CARTESIAN_POINT('Ctrl Pts',(63.9287437903708,1.39329623820574,17.0750559874949));
#23646=CARTESIAN_POINT('Ctrl Pts',(64.4869549413411,1.68096669861507,17.0380100239722));
#23647=CARTESIAN_POINT('Ctrl Pts',(65.0382759195595,1.66831783943796,17.0009640604495));
#23648=CARTESIAN_POINT('Ctrl Pts',(65.5895968977779,1.65566898026085,16.9639180969268));
#23649=CARTESIAN_POINT('Ctrl Pts',(66.1340277032444,1.34270080149729,16.9268721334041));
#23650=CARTESIAN_POINT('Ctrl Pts',(66.4224064907048,0.872644964808594,16.8898261698815));
#23651=CARTESIAN_POINT('Ctrl Pts',(66.7107852781652,0.402589128119899,16.8527802063588));
#23652=CARTESIAN_POINT('Ctrl Pts',(66.7431120476195,-0.224554366493935,
16.8157342428361));
#23653=CARTESIAN_POINT('Ctrl Pts',(66.5045922697214,-0.721769742577186,
16.7786882793134));
#23654=CARTESIAN_POINT('Ctrl Pts',(66.2660724918233,-1.21898511866044,16.7416423157907));
#23655=CARTESIAN_POINT('Ctrl Pts',(65.7567061665729,-1.58627237621311,16.7045963522681));
#23656=CARTESIAN_POINT('Ctrl Pts',(65.2096076810249,-1.65554041915625,16.6675503887454));
#23657=CARTESIAN_POINT('Ctrl Pts',(64.6625091954769,-1.72480846209938,16.6305044252227));
#23658=CARTESIAN_POINT('Ctrl Pts',(64.0776785496314,-1.49605729043299,16.5934584617));
#23659=CARTESIAN_POINT('Ctrl Pts',(63.7227668047739,-1.07397617497671,16.5564124981773));
#23660=CARTESIAN_POINT('Ctrl Pts',(63.4740209335901,-0.778153519638626,
16.5304482109881));
#23661=CARTESIAN_POINT('Ctrl Pts',(63.338214518977,-0.38736442745422,16.504483923799));
#23662=CARTESIAN_POINT('Ctrl Pts',(63.3350414063796,0.00142706819227928,
16.4785196366098));
#23663=CARTESIAN_POINT('Ctrl Pts',(63.3314647116295,0.000550350488423834,
16.6714803633902));
#23664=CARTESIAN_POINT('Ctrl Pts',(63.3337089542098,-0.520837535827165,
16.7064932900275));
#23665=CARTESIAN_POINT('Ctrl Pts',(63.5978310421932,-1.04418591019567,16.7415062166648));
#23666=CARTESIAN_POINT('Ctrl Pts',(64.0195992076647,-1.35039416683956,16.776519143302));
#23667=CARTESIAN_POINT('Ctrl Pts',(64.4658574777874,-1.67438250473233,16.8135651068247));
#23668=CARTESIAN_POINT('Ctrl Pts',(65.0886008827663,-1.7552819972194,16.8506110703474));
#23669=CARTESIAN_POINT('Ctrl Pts',(65.6028273721175,-1.55606853283267,16.8876570338701));
#23670=CARTESIAN_POINT('Ctrl Pts',(66.1170538614687,-1.35685506844592,16.9247029973928));
#23671=CARTESIAN_POINT('Ctrl Pts',(66.5227634351922,-0.877528647185354,
16.9617489609154));
#23672=CARTESIAN_POINT('Ctrl Pts',(66.6342808063438,-0.337455723706574,
16.9987949244381));
#23673=CARTESIAN_POINT('Ctrl Pts',(66.7457981774953,0.202617199772198,17.0358408879608));
#23674=CARTESIAN_POINT('Ctrl Pts',(66.5631233460748,0.803436625469181,17.0728868514835));
#23675=CARTESIAN_POINT('Ctrl Pts',(66.1698584845187,1.19003413633631,17.1099328150062));
#23676=CARTESIAN_POINT('Ctrl Pts',(65.7765936229625,1.57663164720344,17.1469787785288));
#23677=CARTESIAN_POINT('Ctrl Pts',(65.1727387312707,1.74900724324072,17.1840247420515));
#23678=CARTESIAN_POINT('Ctrl Pts',(64.6346514247161,1.62827225548557,17.2210707055742));
#23679=CARTESIAN_POINT('Ctrl Pts',(64.0965641181614,1.50753726773042,17.2581166690969));
#23680=CARTESIAN_POINT('Ctrl Pts',(63.624244396744,1.09369169618284,17.2951626326196));
#23681=CARTESIAN_POINT('Ctrl Pts',(63.4338520592054,0.576134313325577,17.3322085961422));
#23682=CARTESIAN_POINT('Ctrl Pts',(63.3665748819314,0.393249853550898,17.3452991852249));
#23683=CARTESIAN_POINT('Ctrl Pts',(63.334500232668,0.197415541610634,17.3583897743076));
#23684=CARTESIAN_POINT('Ctrl Pts',(63.3357797744869,0.00117646094453,17.3714803633902));
#23685=CARTESIAN_POINT('Origin',(65.,0.,17.));
#23686=CARTESIAN_POINT('',(63.3357162681914,-0.00120644382256618,18.0714803633902));
#23687=CARTESIAN_POINT('',(63.331966723543,-0.000974733628950259,17.8785196366098));
#23688=CARTESIAN_POINT('',(63.334,2.04026156737949E-16,17.));
#23689=CARTESIAN_POINT('Ctrl Pts',(63.331966723543,-0.000974733628950259,
17.8785196366098));
#23690=CARTESIAN_POINT('Ctrl Pts',(63.3354056721751,0.493761861582914,17.8453228558818));
#23691=CARTESIAN_POINT('Ctrl Pts',(63.569536843221,0.991325263991038,17.8121260751538));
#23692=CARTESIAN_POINT('Ctrl Pts',(63.9547567233169,1.30085201001267,17.7789292944258));
#23693=CARTESIAN_POINT('Ctrl Pts',(64.3846430349799,1.64626853206536,17.7418833309031));
#23694=CARTESIAN_POINT('Ctrl Pts',(65.002686987972,1.75751445347199,17.7048373673804));
#23695=CARTESIAN_POINT('Ctrl Pts',(65.5260372626587,1.58367744749354,17.6677914038578));
#23696=CARTESIAN_POINT('Ctrl Pts',(66.0493875373455,1.4098404415151,17.6307454403351));
#23697=CARTESIAN_POINT('Ctrl Pts',(66.4780441337267,0.950920508151569,17.5936994768124));
#23698=CARTESIAN_POINT('Ctrl Pts',(66.6158299298206,0.41694495715979,17.5566535132897));
#23699=CARTESIAN_POINT('Ctrl Pts',(66.7536157259145,-0.117030593831986,
17.519607549767));
#23700=CARTESIAN_POINT('Ctrl Pts',(66.6005307217209,-0.726061762452014,
17.4825615862444));
#23701=CARTESIAN_POINT('Ctrl Pts',(66.22663513746,-1.13142198093973,17.4455156227217));
#23702=CARTESIAN_POINT('Ctrl Pts',(65.8527395531992,-1.53678219942745,17.408469659199));
#23703=CARTESIAN_POINT('Ctrl Pts',(65.258033388871,-1.73847146778285,17.3714236956763));
#23704=CARTESIAN_POINT('Ctrl Pts',(64.7146872927936,-1.64418554868716,17.3343777321536));
#23705=CARTESIAN_POINT('Ctrl Pts',(64.1713411967163,-1.54989962959146,17.2973317686309));
#23706=CARTESIAN_POINT('Ctrl Pts',(63.6793551688898,-1.15963852304467,17.2602858051083));
#23707=CARTESIAN_POINT('Ctrl Pts',(63.4638894046994,-0.652007437388898,
17.2232398415856));
#23708=CARTESIAN_POINT('Ctrl Pts',(63.37718924249,-0.447744372051043,17.2083331065937));
#23709=CARTESIAN_POINT('Ctrl Pts',(63.3352614657588,-0.224477513359574,
17.1934263716017));
#23710=CARTESIAN_POINT('Ctrl Pts',(63.3362856132907,-0.000842509924175838,
17.1785196366098));
#23711=CARTESIAN_POINT('Ctrl Pts',(63.3357797744869,0.00117646094453,17.3714803633902));
#23712=CARTESIAN_POINT('Ctrl Pts',(63.3381212965673,-0.357935006648061,
17.3954357378302));
#23713=CARTESIAN_POINT('Ctrl Pts',(63.4521589055967,-0.71840195855398,17.4193911122702));
#23714=CARTESIAN_POINT('Ctrl Pts',(63.6665656652298,-1.00334589962881,17.4433464867103));
#23715=CARTESIAN_POINT('Ctrl Pts',(63.9981365624523,-1.443999535559,17.480392450233));
#23716=CARTESIAN_POINT('Ctrl Pts',(64.569743310557,-1.70403761325245,17.5174384137557));
#23717=CARTESIAN_POINT('Ctrl Pts',(65.1197868400431,-1.66445223193655,17.5544843772783));
#23718=CARTESIAN_POINT('Ctrl Pts',(65.6698303695292,-1.62486685062064,17.591530340801));
#23719=CARTESIAN_POINT('Ctrl Pts',(66.1983106803967,-1.28565801029538,17.6285763043237));
#23720=CARTESIAN_POINT('Ctrl Pts',(66.4633657616898,-0.802066560180589,
17.6656222678464));
#23721=CARTESIAN_POINT('Ctrl Pts',(66.728420842983,-0.318475110065801,17.702668231369));
#23722=CARTESIAN_POINT('Ctrl Pts',(66.7300506947019,0.309498949838513,17.7397141948917));
#23723=CARTESIAN_POINT('Ctrl Pts',(66.4675094059654,0.794459730162078,17.7767601584144));
#23724=CARTESIAN_POINT('Ctrl Pts',(66.2049681172289,1.27942051048565,17.8138061219371));
#23725=CARTESIAN_POINT('Ctrl Pts',(65.6782556880371,1.62136801122845,17.8508520854598));
#23726=CARTESIAN_POINT('Ctrl Pts',(65.1284250482722,1.66380801970131,17.8878980489824));
#23727=CARTESIAN_POINT('Ctrl Pts',(64.5785944085073,1.70624802817416,17.9249440125051));
#23728=CARTESIAN_POINT('Ctrl Pts',(64.0056455581693,1.44918054437705,17.9619899760278));
#23729=CARTESIAN_POINT('Ctrl Pts',(63.6717917874564,1.01025395994159,17.9990359395505));
#23730=CARTESIAN_POINT('Ctrl Pts',(63.4541716406064,0.724142865382969,18.0231840808304));
#23731=CARTESIAN_POINT('Ctrl Pts',(63.3381427347181,0.36076003548376,18.0473322221103));
#23732=CARTESIAN_POINT('Ctrl Pts',(63.3357162681914,-0.00120644382256618,
18.0714803633902));
#23733=CARTESIAN_POINT('Origin',(65.,0.,17.));
#23734=CARTESIAN_POINT('',(63.3314263973441,-0.000500571934790497,18.7714803633902));
#23735=CARTESIAN_POINT('',(63.3333325352018,0.00145874397800797,18.5785196366098));
#23736=CARTESIAN_POINT('',(63.334,2.04026156737949E-16,17.));
#23737=CARTESIAN_POINT('Ctrl Pts',(63.3333325352018,0.00145874397800797,
18.5785196366098));
#23738=CARTESIAN_POINT('Ctrl Pts',(63.3323458932764,0.109115274956356,18.5713112672072));
#23739=CARTESIAN_POINT('Ctrl Pts',(63.3418839056658,0.216597722493275,18.5641028978047));
#23740=CARTESIAN_POINT('Ctrl Pts',(63.3625817175621,0.321886358429003,18.5568945284021));
#23741=CARTESIAN_POINT('Ctrl Pts',(63.4689539553991,0.862996108553322,18.5198485648794));
#23742=CARTESIAN_POINT('Ctrl Pts',(63.8700831830826,1.34616204853444,18.4828026013567));
#23743=CARTESIAN_POINT('Ctrl Pts',(64.382390335006,1.55026054620228,18.445756637834));
#23744=CARTESIAN_POINT('Ctrl Pts',(64.8946974869294,1.75435904387011,18.4087106743114));
#23745=CARTESIAN_POINT('Ctrl Pts',(65.5181825630929,1.67939009922466,18.3716647107887));
#23746=CARTESIAN_POINT('Ctrl Pts',(65.9675040829891,1.359663674886,18.334618747266));
#23747=CARTESIAN_POINT('Ctrl Pts',(66.4168256028854,1.03993725054733,18.2975727837433));
#23748=CARTESIAN_POINT('Ctrl Pts',(66.6919835665143,0.475453346515458,18.2605268202206));
#23749=CARTESIAN_POINT('Ctrl Pts',(66.6670503715696,-0.0754487776881312,
18.223480856698));
#23750=CARTESIAN_POINT('Ctrl Pts',(66.6421171766249,-0.626350901891724,
18.1864348931753));
#23751=CARTESIAN_POINT('Ctrl Pts',(66.3170928231065,-1.16367124626703,18.1493889296526));
#23752=CARTESIAN_POINT('Ctrl Pts',(65.8407265494155,-1.44150210839705,18.1123429661299));
#23753=CARTESIAN_POINT('Ctrl Pts',(65.3643602757244,-1.71933297052706,18.0752970026072));
#23754=CARTESIAN_POINT('Ctrl Pts',(64.7366520818608,-1.73767435041179,18.0382510390846));
#23755=CARTESIAN_POINT('Ctrl Pts',(64.2448761820938,-1.48813221154433,18.0012050755619));
#23756=CARTESIAN_POINT('Ctrl Pts',(63.7531002823268,-1.23859007267686,17.9641591120392));
#23757=CARTESIAN_POINT('Ctrl Pts',(63.3972566766564,-0.721164415057194,
17.9271131485165));
#23758=CARTESIAN_POINT('Ctrl Pts',(63.3401992089882,-0.172658024897985,
17.8900671849938));
#23759=CARTESIAN_POINT('Ctrl Pts',(63.3342707730138,-0.115666623972996,
17.8862180021992));
#23760=CARTESIAN_POINT('Ctrl Pts',(63.3315679757844,-0.0583396813265016,
17.8823688194045));
#23761=CARTESIAN_POINT('Ctrl Pts',(63.331966723543,-0.000974733628950259,
17.8785196366098));
#23762=CARTESIAN_POINT('Ctrl Pts',(63.3357162681914,-0.00120644382256618,
18.0714803633902));
#23763=CARTESIAN_POINT('Ctrl Pts',(63.3344202622762,-0.194537237022046,
18.084378185633));
#23764=CARTESIAN_POINT('Ctrl Pts',(63.3655323149503,-0.387463979276361,
18.0972760078758));
#23765=CARTESIAN_POINT('Ctrl Pts',(63.4308825664874,-0.567997006411725,
18.1101738301185));
#23766=CARTESIAN_POINT('Ctrl Pts',(63.6185858073192,-1.08653570325577,18.1472197936412));
#23767=CARTESIAN_POINT('Ctrl Pts',(64.0887509800707,-1.50282741187005,18.1842657571639));
#23768=CARTESIAN_POINT('Ctrl Pts',(64.6262043274144,-1.62635387127239,18.2213117206866));
#23769=CARTESIAN_POINT('Ctrl Pts',(65.1636576747581,-1.74988033067472,18.2583576842093));
#23770=CARTESIAN_POINT('Ctrl Pts',(65.768399196694,-1.5806415408651,18.2954036477319));
#23771=CARTESIAN_POINT('Ctrl Pts',(66.1636655065904,-1.19609059364975,18.3324496112546));
#23772=CARTESIAN_POINT('Ctrl Pts',(66.5589318164868,-0.811539646434406,
18.3694955747773));
#23773=CARTESIAN_POINT('Ctrl Pts',(66.7447229143437,-0.21167654181333,18.4065415383));
#23774=CARTESIAN_POINT('Ctrl Pts',(66.6360104507197,0.328967968929765,18.4435875018227));
#23775=CARTESIAN_POINT('Ctrl Pts',(66.5272979870957,0.869612479672864,18.4806334653453));
#23776=CARTESIAN_POINT('Ctrl Pts',(66.1240819619909,1.35103839653798,18.517679428868));
#23777=CARTESIAN_POINT('Ctrl Pts',(65.6108964756848,1.55291841879865,18.5547253923907));
#23778=CARTESIAN_POINT('Ctrl Pts',(65.0977109893788,1.75479844105931,18.5917713559134));
#23779=CARTESIAN_POINT('Ctrl Pts',(64.4745560418716,1.67713256871553,18.6288173194361));
#23780=CARTESIAN_POINT('Ctrl Pts',(64.0266220284185,1.3554650286459,18.6658632829587));
#23781=CARTESIAN_POINT('Ctrl Pts',(63.6009392798522,1.04977642615326,18.7010689764359));
#23782=CARTESIAN_POINT('Ctrl Pts',(63.3335015355576,0.523725769548793,18.7362746699131));
#23783=CARTESIAN_POINT('Ctrl Pts',(63.3314263973441,-0.000500571934790497,
18.7714803633902));
#23784=CARTESIAN_POINT('Origin',(65.,0.,17.));
#23785=CARTESIAN_POINT('',(63.3342413915565,0.00152189757970267,19.4714803633902));
#23786=CARTESIAN_POINT('',(63.3367061905351,6.33250723265802E-5,19.2785196366098));
#23787=CARTESIAN_POINT('',(63.334,2.04026156737949E-16,17.));
#23788=CARTESIAN_POINT('Ctrl Pts',(63.3367061905351,6.33250723265801E-5,
19.2785196366098));
#23789=CARTESIAN_POINT('Ctrl Pts',(63.336613224224,0.274266937448926,19.26025371501));
#23790=CARTESIAN_POINT('Ctrl Pts',(63.4006540507369,0.548429669491752,19.2419877934101));
#23791=CARTESIAN_POINT('Ctrl Pts',(63.5290671316579,0.788102757387651,19.2237218718103));
#23792=CARTESIAN_POINT('Ctrl Pts',(63.7895076621637,1.27419487286283,19.1866759082877));
#23793=CARTESIAN_POINT('Ctrl Pts',(64.3147356017013,1.61841804812355,19.149629944765));
#23794=CARTESIAN_POINT('Ctrl Pts',(64.8643774055205,1.66323659510229,19.1125839812423));
#23795=CARTESIAN_POINT('Ctrl Pts',(65.4140192093397,1.70805514208103,19.0755380177196));
#23796=CARTESIAN_POINT('Ctrl Pts',(65.9880748774405,1.4534690607778,19.0384920541969));
#23797=CARTESIAN_POINT('Ctrl Pts',(66.3238245781873,1.01599111491805,19.0014460906742));
#23798=CARTESIAN_POINT('Ctrl Pts',(66.6595742789341,0.578513169058305,18.9644001271516));
#23799=CARTESIAN_POINT('Ctrl Pts',(66.757018012327,-0.0418566413579579,
18.9273541636289));
#23800=CARTESIAN_POINT('Ctrl Pts',(66.5715601012413,-0.561202554865601,
18.8903082001062));
#23801=CARTESIAN_POINT('Ctrl Pts',(66.3861021901555,-1.08054846837324,18.8532622365835));
#23802=CARTESIAN_POINT('Ctrl Pts',(65.9177426345912,-1.49887048497226,18.8162162730609));
#23803=CARTESIAN_POINT('Ctrl Pts',(65.3808288409285,-1.62472116171495,18.7791703095382));
#23804=CARTESIAN_POINT('Ctrl Pts',(64.8439150472658,-1.75057183845763,18.7421243460155));
#23805=CARTESIAN_POINT('Ctrl Pts',(64.2384470155047,-1.58395117534399,18.7050783824928));
#23806=CARTESIAN_POINT('Ctrl Pts',(63.8415206236195,-1.20111406365341,18.6680324189701));
#23807=CARTESIAN_POINT('Ctrl Pts',(63.5218278028516,-0.892769043939022,
18.63819482485));
#23808=CARTESIAN_POINT('Ctrl Pts',(63.3374165408442,-0.444163795089777,
18.6083572307299));
#23809=CARTESIAN_POINT('Ctrl Pts',(63.3333325352018,0.00145874397800797,
18.5785196366098));
#23810=CARTESIAN_POINT('Ctrl Pts',(63.3314263973441,-0.000500571934790497,
18.7714803633902));
#23811=CARTESIAN_POINT('Ctrl Pts',(63.3313179258352,-0.0279029020134356,
18.7733206334357));
#23812=CARTESIAN_POINT('Ctrl Pts',(63.3319345194755,-0.0553002474134368,
18.7751609034813));
#23813=CARTESIAN_POINT('Ctrl Pts',(63.3332914773975,-0.0826608742403259,
18.7770011735268));
#23814=CARTESIAN_POINT('Ctrl Pts',(63.3606080192284,-0.633450029261446,
18.8140471370495));
#23815=CARTESIAN_POINT('Ctrl Pts',(63.6879541822893,-1.16935913150821,18.8510931005721));
#23816=CARTESIAN_POINT('Ctrl Pts',(64.1655181388753,-1.44512634150632,18.8881390640948));
#23817=CARTESIAN_POINT('Ctrl Pts',(64.6430820954612,-1.72089355150444,18.9251850276175));
#23818=CARTESIAN_POINT('Ctrl Pts',(65.2708638455722,-1.73651886925392,18.9622309911402));
#23819=CARTESIAN_POINT('Ctrl Pts',(65.7615555115074,-1.48485127952433,18.9992769546629));
#23820=CARTESIAN_POINT('Ctrl Pts',(66.2522471774427,-1.23318368979475,19.0363229181856));
#23821=CARTESIAN_POINT('Ctrl Pts',(66.6058487592021,-0.714223192586113,
19.0733688817082));
#23822=CARTESIAN_POINT('Ctrl Pts',(66.6605324878321,-0.165475002074327,
19.1104148452309));
#23823=CARTESIAN_POINT('Ctrl Pts',(66.715216216462,0.383273188437468,19.1474608087536));
#23824=CARTESIAN_POINT('Ctrl Pts',(66.4709820919624,0.961809072252411,19.1845067722763));
#23825=CARTESIAN_POINT('Ctrl Pts',(66.0396052463205,1.30536242146667,19.221552735799));
#23826=CARTESIAN_POINT('Ctrl Pts',(65.6082284006786,1.64891577068093,19.2585986993216));
#23827=CARTESIAN_POINT('Ctrl Pts',(64.9897088338945,1.7574865852945,19.2956446628443));
#23828=CARTESIAN_POINT('Ctrl Pts',(64.4671155329348,1.58138681666735,19.332690626367));
#23829=CARTESIAN_POINT('Ctrl Pts',(63.9445222319752,1.4052870480402,19.3697365898897));
#23830=CARTESIAN_POINT('Ctrl Pts',(63.5178551968399,0.94451669617232,19.4067825534124));
#23831=CARTESIAN_POINT('Ctrl Pts',(63.3823810155581,0.409949924733969,19.443828516935));
#23832=CARTESIAN_POINT('Ctrl Pts',(63.34867413809,0.27694615609758,19.4530457990868));
#23833=CARTESIAN_POINT('Ctrl Pts',(63.3329934814549,0.139374038553371,19.4622630812385));
#23834=CARTESIAN_POINT('Ctrl Pts',(63.3342413915565,0.00152189757970267,
19.4714803633902));
#23835=CARTESIAN_POINT('Origin',(65.,0.,17.));
#23836=CARTESIAN_POINT('',(63.33660733148,-0.000426122236795029,20.1714803633902));
#23837=CARTESIAN_POINT('',(63.3335649842428,-0.00149162251194977,19.9785196366098));
#23838=CARTESIAN_POINT('',(63.334,2.04026156737949E-16,17.));
#23839=CARTESIAN_POINT('Ctrl Pts',(63.3335649842428,-0.00149162251194977,
19.9785196366098));
#23840=CARTESIAN_POINT('Ctrl Pts',(63.3376081205507,0.436609739463929,19.9491961628127));
#23841=CARTESIAN_POINT('Ctrl Pts',(63.5150446040949,0.877608758866625,19.9198726890157));
#23842=CARTESIAN_POINT('Ctrl Pts',(63.8250037086467,1.18496125357119,19.8905492152186));
#23843=CARTESIAN_POINT('Ctrl Pts',(64.2165921595995,1.57325663038185,19.8535032516959));
#23844=CARTESIAN_POINT('Ctrl Pts',(64.8196955128484,1.748243279982,19.8164572881732));
#23845=CARTESIAN_POINT('Ctrl Pts',(65.3583001004237,1.62983756803352,19.7794113246505));
#23846=CARTESIAN_POINT('Ctrl Pts',(65.896904687999,1.51143185608505,19.7423653611279));
#23847=CARTESIAN_POINT('Ctrl Pts',(66.3710105099008,1.09963378258794,19.7053193976052));
#23848=CARTESIAN_POINT('Ctrl Pts',(66.5636403476301,0.582905071893254,19.6682734340825));
#23849=CARTESIAN_POINT('Ctrl Pts',(66.7562701853594,0.0661763611985695,
19.6312274705598));
#23850=CARTESIAN_POINT('Ctrl Pts',(66.6674240389162,-0.55548298669369,19.5941815070372));
#23851=CARTESIAN_POINT('Ctrl Pts',(66.3377628513866,-0.997567046656913,
19.5571355435145));
#23852=CARTESIAN_POINT('Ctrl Pts',(66.008101663857,-1.43965110662013,19.5200895799918));
#23853=CARTESIAN_POINT('Ctrl Pts',(65.437625435241,-1.70215987865432,19.4830436164691));
#23854=CARTESIAN_POINT('Ctrl Pts',(64.8874158461961,-1.6649547344678,19.4459976529464));
#23855=CARTESIAN_POINT('Ctrl Pts',(64.3372062571513,-1.62774959028127,19.4089516894237));
#23856=CARTESIAN_POINT('Ctrl Pts',(63.8072633076776,-1.29083052987404,19.3719057259011));
#23857=CARTESIAN_POINT('Ctrl Pts',(63.5401183936778,-0.808390471825603,
19.3348597623784));
#23858=CARTESIAN_POINT('Ctrl Pts',(63.404692230951,-0.563822814410766,19.3160797204555));
#23859=CARTESIAN_POINT('Ctrl Pts',(63.3368017735151,-0.28185813767411,19.2972996785327));
#23860=CARTESIAN_POINT('Ctrl Pts',(63.3367061905351,6.33250723265801E-5,
19.2785196366098));
#23861=CARTESIAN_POINT('Ctrl Pts',(63.3342413915565,0.00152189757970267,
19.4714803633902));
#23862=CARTESIAN_POINT('Ctrl Pts',(63.3380090632001,-0.414679238971563,
19.4993090447612));
#23863=CARTESIAN_POINT('Ctrl Pts',(63.496088728647,-0.833432923200605,19.5271377261321));
#23864=CARTESIAN_POINT('Ctrl Pts',(63.778271499721,-1.1367187830676,19.5549664075031));
#23865=CARTESIAN_POINT('Ctrl Pts',(64.1539174925939,-1.54045752842199,19.5920123710258));
#23866=CARTESIAN_POINT('Ctrl Pts',(64.7494908057681,-1.73957182812194,19.6290583345484));
#23867=CARTESIAN_POINT('Ctrl Pts',(65.2924239354676,-1.64293589624755,19.6661042980711));
#23868=CARTESIAN_POINT('Ctrl Pts',(65.835357065167,-1.54629996437316,19.7031502615938));
#23869=CARTESIAN_POINT('Ctrl Pts',(66.3256500113918,-1.15391380092443,19.7401962251165));
#23870=CARTESIAN_POINT('Ctrl Pts',(66.5389174268969,-0.645355153836869,
19.7772421886392));
#23871=CARTESIAN_POINT('Ctrl Pts',(66.7521848424021,-0.136796506749309,
19.8142881521618));
#23872=CARTESIAN_POINT('Ctrl Pts',(66.6884267271877,0.487934623977085,19.8513341156845));
#23873=CARTESIAN_POINT('Ctrl Pts',(66.3768223447206,0.942926484478224,19.8883800792072));
#23874=CARTESIAN_POINT('Ctrl Pts',(66.0652179622535,1.39791834497936,19.9254260427299));
#23875=CARTESIAN_POINT('Ctrl Pts',(65.5057673125336,1.68317093525526,19.9624720062526));
#23876=CARTESIAN_POINT('Ctrl Pts',(64.9545061567026,1.6681368085672,19.9995179697752));
#23877=CARTESIAN_POINT('Ctrl Pts',(64.4032450008716,1.65310268187915,20.0365639332979));
#23878=CARTESIAN_POINT('Ctrl Pts',(63.8601733389293,1.33778183822715,20.0736098968206));
#23879=CARTESIAN_POINT('Ctrl Pts',(63.5738309983811,0.866482612606734,20.1106558603433));
#23880=CARTESIAN_POINT('Ctrl Pts',(63.4171190932323,0.608545908587611,20.1309306946923));
#23881=CARTESIAN_POINT('Ctrl Pts',(63.3373039960783,0.303889805224319,20.1512055290412));
#23882=CARTESIAN_POINT('Ctrl Pts',(63.33660733148,-0.000426122236795029,
20.1714803633902));
#23883=CARTESIAN_POINT('Origin',(65.,0.,17.));
#23884=CARTESIAN_POINT('',(63.3326792503596,-0.00130047270866476,20.8714803633902));
#23885=CARTESIAN_POINT('',(63.3318013787731,0.000864016794202189,20.6785196366098));
#23886=CARTESIAN_POINT('',(63.334,2.04026156737949E-16,17.));
#23887=CARTESIAN_POINT('Ctrl Pts',(63.3318013787731,0.000864016794202189,
20.6785196366098));
#23888=CARTESIAN_POINT('Ctrl Pts',(63.3314877360124,0.050553985174294,20.6751845741382));
#23889=CARTESIAN_POINT('Ctrl Pts',(63.3335154742976,0.100217999006552,20.6718495116665));
#23890=CARTESIAN_POINT('Ctrl Pts',(63.3379679807618,0.149663664483466,20.6685144491949));
#23891=CARTESIAN_POINT('Ctrl Pts',(63.3874265421712,0.698907444829377,20.6314684856722));
#23892=CARTESIAN_POINT('Ctrl Pts',(63.7360730319708,1.22120960136622,20.5944225221495));
#23893=CARTESIAN_POINT('Ctrl Pts',(64.2243472290266,1.47753582103746,20.5573765586268));
#23894=CARTESIAN_POINT('Ctrl Pts',(64.7126214260825,1.73386204070869,20.5203305951042));
#23895=CARTESIAN_POINT('Ctrl Pts',(65.3405233303947,1.72421232351432,20.4832846315815));
#23896=CARTESIAN_POINT('Ctrl Pts',(65.8206901647961,1.453002801034,20.4462386680588));
#23897=CARTESIAN_POINT('Ctrl Pts',(66.3008569991975,1.18179327855368,20.4091927045361));
#23898=CARTESIAN_POINT('Ctrl Pts',(66.6332887636883,0.649023950787429,20.3721467410134));
#23899=CARTESIAN_POINT('Ctrl Pts',(66.6658461309716,0.0985197801765333,
20.3351007774908));
#23900=CARTESIAN_POINT('Ctrl Pts',(66.698403498255,-0.451984390434366,20.2980548139681));
#23901=CARTESIAN_POINT('Ctrl Pts',(66.431086468331,-1.02022340388991,20.2610088504454));
#23902=CARTESIAN_POINT('Ctrl Pts',(65.9862342185508,-1.34613948307828,20.2239628869227));
#23903=CARTESIAN_POINT('Ctrl Pts',(65.5413819687707,-1.67205556226665,20.1869169234));
#23904=CARTESIAN_POINT('Ctrl Pts',(64.9189944991343,-1.75564870718784,20.1498709598773));
#23905=CARTESIAN_POINT('Ctrl Pts',(64.4039109527966,-1.55866202617724,20.1128249963547));
#23906=CARTESIAN_POINT('Ctrl Pts',(63.8888274064588,-1.36167534516664,20.075779032832));
#23907=CARTESIAN_POINT('Ctrl Pts',(63.4810477834196,-0.884108838224231,
20.0387330693093));
#23908=CARTESIAN_POINT('Ctrl Pts',(63.3671947462284,-0.344523532742441,
20.0016871057866));
#23909=CARTESIAN_POINT('Ctrl Pts',(63.3434612857827,-0.232043208803138,
19.993964616061));
#23910=CARTESIAN_POINT('Ctrl Pts',(63.332500203214,-0.116867900576725,19.9862421263354));
#23911=CARTESIAN_POINT('Ctrl Pts',(63.3335649842428,-0.00149162251194977,
19.9785196366098));
#23912=CARTESIAN_POINT('Ctrl Pts',(63.33660733148,-0.000426122236795029,
20.1714803633902));
#23913=CARTESIAN_POINT('Ctrl Pts',(63.3360310578707,-0.252153048396656,
20.1882514925639));
#23914=CARTESIAN_POINT('Ctrl Pts',(63.3895909699888,-0.503647211782716,
20.2050226217376));
#23915=CARTESIAN_POINT('Ctrl Pts',(63.4985445030998,-0.728272982538809,
20.2217937509113));
#23916=CARTESIAN_POINT('Ctrl Pts',(63.7392133675209,-1.2244517444751,20.258839714434));
#23917=CARTESIAN_POINT('Ctrl Pts',(64.2501641155174,-1.58953166075886,20.2958856779567));
#23918=CARTESIAN_POINT('Ctrl Pts',(64.7975572478223,-1.65643198360555,20.3329316414794));
#23919=CARTESIAN_POINT('Ctrl Pts',(65.3449503801273,-1.72333230645224,20.369977605002));
#23920=CARTESIAN_POINT('Ctrl Pts',(65.9287858967409,-1.49205303586186,20.4070235685247));
#23921=CARTESIAN_POINT('Ctrl Pts',(66.2818681473523,-1.06844015166583,20.4440695320474));
#23922=CARTESIAN_POINT('Ctrl Pts',(66.6349503979637,-0.644827267469802,
20.4811154955701));
#23923=CARTESIAN_POINT('Ctrl Pts',(66.757279382573,-0.0288807696681307,
20.5181614590928));
#23924=CARTESIAN_POINT('Ctrl Pts',(66.5928705785965,0.497507359328871,20.5552074226155));
#23925=CARTESIAN_POINT('Ctrl Pts',(66.42846177462,1.02389548832587,20.5922533861381));
#23926=CARTESIAN_POINT('Ctrl Pts',(65.9773151820577,1.4607252485182,20.6292993496608));
#23927=CARTESIAN_POINT('Ctrl Pts',(65.4459005359057,1.60808016419334,20.6663453131835));
#23928=CARTESIAN_POINT('Ctrl Pts',(64.9144858897538,1.75543507986848,20.7033912767062));
#23929=CARTESIAN_POINT('Ctrl Pts',(64.3028031900122,1.61331515102643,20.7404372402289));
#23930=CARTESIAN_POINT('Ctrl Pts',(63.8907926142615,1.24676010485229,20.7774832037515));
#23931=CARTESIAN_POINT('Ctrl Pts',(63.5423261851822,0.936738625989566,20.8088155902978));
#23932=CARTESIAN_POINT('Ctrl Pts',(63.3366907965296,0.466172446764657,20.840147976844));
#23933=CARTESIAN_POINT('Ctrl Pts',(63.3326792503596,-0.00130047270866476,
20.8714803633902));
#23934=CARTESIAN_POINT('Origin',(65.,0.,17.));
#23935=CARTESIAN_POINT('',(63.3325282901756,0.00121307831918299,21.5714803633902));
#23936=CARTESIAN_POINT('',(63.3361634080255,0.000941845566869666,21.3785196366098));
#23937=CARTESIAN_POINT('',(63.334,2.04026156737949E-16,17.));
#23938=CARTESIAN_POINT('',(66.2690708798524,1.07935865304853,22.));
#23939=CARTESIAN_POINT('Ctrl Pts',(63.3325282901756,0.00121307831918299,
21.5714803633902));
#23940=CARTESIAN_POINT('Ctrl Pts',(63.3364666394986,-0.471552579298224,
21.6031823516921));
#23941=CARTESIAN_POINT('Ctrl Pts',(63.5475594887738,-0.947301871471163,
21.634884339994));
#23942=CARTESIAN_POINT('Ctrl Pts',(63.9032471486994,-1.25758535694561,21.6665863282959));
#23943=CARTESIAN_POINT('Ctrl Pts',(64.3188927526783,-1.62017304624496,21.7036322918186));
#23944=CARTESIAN_POINT('Ctrl Pts',(64.9319903369097,-1.75680828918912,21.7406782553412));
#23945=CARTESIAN_POINT('Ctrl Pts',(65.4619049207954,-1.60385028487085,21.7777242188639));
#23946=CARTESIAN_POINT('Ctrl Pts',(65.991819504681,-1.45089228055259,21.8147701823866));
#23947=CARTESIAN_POINT('Ctrl Pts',(66.4385510882208,-1.0083410289719,21.8518161459093));
#23948=CARTESIAN_POINT('Ctrl Pts',(66.5975920398022,-0.481277360573865,
21.8888621094319));
#23949=CARTESIAN_POINT('Ctrl Pts',(66.7566329913836,0.0457863078241707,
21.9259080729546));
#23950=CARTESIAN_POINT('Ctrl Pts',(66.6279833110066,0.657362393039556,21.9629540364773));
#23951=CARTESIAN_POINT('Ctrl Pts',(66.2690708798524,1.07935865304855,22.));
#23952=CARTESIAN_POINT('',(63.7285313545748,1.08121009939331,22.));
#23953=CARTESIAN_POINT('Origin',(65.,0.,22.));
#23954=CARTESIAN_POINT('Ctrl Pts',(63.7285300176229,1.0812111317272,22.));
#23955=CARTESIAN_POINT('Ctrl Pts',(64.0793901440196,1.49274250755582,21.9636770818144));
#23956=CARTESIAN_POINT('Ctrl Pts',(64.6493623256457,1.71876565001736,21.9273541636289));
#23957=CARTESIAN_POINT('Ctrl Pts',(65.1867621807782,1.65816351020322,21.8910312454434));
#23958=CARTESIAN_POINT('Ctrl Pts',(65.7348595370708,1.59635502197871,21.8539852819207));
#23959=CARTESIAN_POINT('Ctrl Pts',(66.2490748882323,1.23639652943471,21.816939318398));
#23960=CARTESIAN_POINT('Ctrl Pts',(66.4944088007071,0.742590901212614,21.7798933548753));
#23961=CARTESIAN_POINT('Ctrl Pts',(66.7397427131819,0.248785272990521,21.7428473913526));
#23962=CARTESIAN_POINT('Ctrl Pts',(66.7161951869699,-0.378867490909659,
21.7058014278299));
#23963=CARTESIAN_POINT('Ctrl Pts',(66.4343747134738,-0.852900746623158,
21.6687554643073));
#23964=CARTESIAN_POINT('Ctrl Pts',(66.1525542399776,-1.32693400233666,21.6317095007846));
#23965=CARTESIAN_POINT('Ctrl Pts',(65.6124608191971,-1.64734774986348,21.5946635372619));
#23966=CARTESIAN_POINT('Ctrl Pts',(65.061356017574,-1.66761252399562,21.5576175737392));
#23967=CARTESIAN_POINT('Ctrl Pts',(64.5102512159508,-1.68787729812775,21.5205716102165));
#23968=CARTESIAN_POINT('Ctrl Pts',(63.9481350334849,-1.40799309886521,21.4835256466939));
#23969=CARTESIAN_POINT('Ctrl Pts',(63.6322204085561,-0.95599522362411,21.4464796831712));
#23970=CARTESIAN_POINT('Ctrl Pts',(63.4390408141815,-0.679601668824516,
21.4238263343174));
#23971=CARTESIAN_POINT('Ctrl Pts',(63.3379218264913,-0.338850724949921,
21.4011729854636));
#23972=CARTESIAN_POINT('Ctrl Pts',(63.3361634080255,0.000941845566869666,
21.3785196366098));
#23973=CARTESIAN_POINT('Origin',(65.,0.,23.5459252805377));
#23974=CARTESIAN_POINT('',(62.9427844533856,0.00119489768198394,13.4540747194623));
#23975=CARTESIAN_POINT('',(62.9484021938786,-0.000803300711486093,13.3959252805377));
#23976=CARTESIAN_POINT('',(62.94525,1.28744642201805E-13,23.5459252805377));
#23977=CARTESIAN_POINT('',(66.8826275096638,-0.823232180103057,13.));
#23978=CARTESIAN_POINT('Ctrl Pts',(62.9484021938786,-0.000803300711485905,
13.3959252805377));
#23979=CARTESIAN_POINT('Ctrl Pts',(62.9495841394398,0.384792240838318,13.3750880775932));
#23980=CARTESIAN_POINT('Ctrl Pts',(63.239440569463,1.45761852527274,13.3172049111259));
#23981=CARTESIAN_POINT('Ctrl Pts',(64.970198323091,2.42992595215152,13.2222757811361));
#23982=CARTESIAN_POINT('Ctrl Pts',(67.0251392906009,1.33877286094185,13.111137890568));
#23983=CARTESIAN_POINT('Ctrl Pts',(67.1563717950601,-0.197213743559485,
13.0370459635227));
#23984=CARTESIAN_POINT('Ctrl Pts',(66.8826275096638,-0.823232180103057,
13.));
#23985=CARTESIAN_POINT('',(66.2235927967208,-1.65534565011393,13.));
#23986=CARTESIAN_POINT('Origin',(65.,0.,13.));
#23987=CARTESIAN_POINT('Ctrl Pts',(62.9427844533856,0.00119489768198401,
13.4540747194623));
#23988=CARTESIAN_POINT('Ctrl Pts',(62.9422817266512,0.0728349382260934,
13.4501772883951));
#23989=CARTESIAN_POINT('Ctrl Pts',(62.9781729708452,0.824925643882596,13.4092338938053));
#23990=CARTESIAN_POINT('Ctrl Pts',(63.9036938704104,2.16732302296764,13.3312445356927));
#23991=CARTESIAN_POINT('Ctrl Pts',(66.2265689546786,2.09606376419022,13.2201066451247));
#23992=CARTESIAN_POINT('Ctrl Pts',(67.4179368644029,0.120091680801066,13.1096917998938));
#23993=CARTESIAN_POINT('Ctrl Pts',(66.7594496906129,-1.25819328818366,13.0363229181856));
#23994=CARTESIAN_POINT('Ctrl Pts',(66.2235939546714,-1.65534738192936,13.));
#23995=CARTESIAN_POINT('Origin',(65.,0.,23.5459252805377));
#23996=CARTESIAN_POINT('',(62.9480827837869,0.00102651687048705,14.1540747194623));
#23997=CARTESIAN_POINT('',(62.9433366278651,-0.0014977223415923,14.0959252805377));
#23998=CARTESIAN_POINT('',(62.94525,1.28744642201805E-13,23.5459252805377));
#23999=CARTESIAN_POINT('Ctrl Pts',(62.9433366278651,-0.00149772234159223,
14.0959252805377));
#24000=CARTESIAN_POINT('Ctrl Pts',(62.9481477427571,0.585192187367158,14.0640305253959));
#24001=CARTESIAN_POINT('Ctrl Pts',(63.5186241718586,1.86149425637258,13.9950898067315));
#24002=CARTESIAN_POINT('Ctrl Pts',(65.684305645688,2.3302668619962,13.8891031245443));
#24003=CARTESIAN_POINT('Ctrl Pts',(67.3289123722387,0.688818574436941,13.7779652339763));
#24004=CARTESIAN_POINT('Ctrl Pts',(66.8417982611818,-1.58294512384396,13.6668273434083));
#24005=CARTESIAN_POINT('Ctrl Pts',(64.6689465387577,-2.4061546469661,13.5556894528402));
#24006=CARTESIAN_POINT('Ctrl Pts',(63.14955544062,-1.28502616351135,13.4653887652167));
#24007=CARTESIAN_POINT('Ctrl Pts',(62.9474827867649,-0.300748827451898,
13.4121340411158));
#24008=CARTESIAN_POINT('Ctrl Pts',(62.9484021938786,-0.000803300711485905,
13.3959252805377));
#24009=CARTESIAN_POINT('Ctrl Pts',(62.9480827837869,0.00102651687048705,
14.1540747194623));
#24010=CARTESIAN_POINT('Ctrl Pts',(62.9468311597533,0.277742487636534,14.1391197361979));
#24011=CARTESIAN_POINT('Ctrl Pts',(63.1278468516848,1.23836027065323,14.0871187894108));
#24012=CARTESIAN_POINT('Ctrl Pts',(64.5878737813476,2.39342385873018,13.998071879101));
#24013=CARTESIAN_POINT('Ctrl Pts',(66.7873400138256,1.64430308142019,13.8869339885329));
#24014=CARTESIAN_POINT('Ctrl Pts',(67.3508170614469,-0.609852217558742,
13.7757960979649));
#24015=CARTESIAN_POINT('Ctrl Pts',(65.7625975239189,-2.30583209920716,13.6646582073969));
#24016=CARTESIAN_POINT('Ctrl Pts',(63.5564754082319,-1.90574022357351,13.557417747896));
#24017=CARTESIAN_POINT('Ctrl Pts',(62.9470602579309,-0.608119845326389,
13.4872232519178));
#24018=CARTESIAN_POINT('Ctrl Pts',(62.9427844533856,0.00119489768198401,
13.4540747194623));
#24019=CARTESIAN_POINT('Origin',(65.,0.,23.5459252805377));
#24020=CARTESIAN_POINT('',(62.9465102637711,-0.00176526862452037,14.8540747194623));
#24021=CARTESIAN_POINT('',(62.94372126594,0.00163389948556141,14.7959252805377));
#24022=CARTESIAN_POINT('',(62.94525,1.28744642201805E-13,23.5459252805377));
#24023=CARTESIAN_POINT('Ctrl Pts',(62.94372126594,0.00163389948556124,14.7959252805377));
#24024=CARTESIAN_POINT('Ctrl Pts',(62.9427765522985,0.110331733448615,14.7900189367213));
#24025=CARTESIAN_POINT('Ctrl Pts',(63.0000473239053,0.899810372641752,14.7470666293823));
#24026=CARTESIAN_POINT('Ctrl Pts',(64.0226192720082,2.22329513352231,14.6670683585206));
#24027=CARTESIAN_POINT('Ctrl Pts',(66.3378385875382,2.02694463079714,14.5559304679526));
#24028=CARTESIAN_POINT('Ctrl Pts',(67.4285194097127,-0.0246926670119161,
14.4447925773845));
#24029=CARTESIAN_POINT('Ctrl Pts',(66.2963482043283,-2.05372573368659,14.3336546868165));
#24030=CARTESIAN_POINT('Ctrl Pts',(63.9776161165208,-2.20296580816612,14.2225167962485));
#24031=CARTESIAN_POINT('Ctrl Pts',(62.9915607037629,-0.871642779145011,
14.1432736608222));
#24032=CARTESIAN_POINT('Ctrl Pts',(62.942559601823,-0.0962519214711344,
14.1010764889186));
#24033=CARTESIAN_POINT('Ctrl Pts',(62.9433366278651,-0.00149772234159223,
14.0959252805377));
#24034=CARTESIAN_POINT('Ctrl Pts',(62.946510263771,-0.00176526862452042,
14.8540747194623));
#24035=CARTESIAN_POINT('Ctrl Pts',(62.9504460460768,0.478624892210608,14.8280621840006));
#24036=CARTESIAN_POINT('Ctrl Pts',(63.3581297348817,1.64918471803046,14.7650036850163));
#24037=CARTESIAN_POINT('Ctrl Pts',(65.308185017446,2.40901142364104,14.6648992225093));
#24038=CARTESIAN_POINT('Ctrl Pts',(67.1910886177016,1.04758997952522,14.5537613319412));
#24039=CARTESIAN_POINT('Ctrl Pts',(67.068463685159,-1.27270221153156,14.4426234413732));
#24040=CARTESIAN_POINT('Ctrl Pts',(65.0525510239567,-2.42807611461693,14.3314855508051));
#24041=CARTESIAN_POINT('Ctrl Pts',(63.2662754947239,-1.50459133827137,14.2353026435015));
#24042=CARTESIAN_POINT('Ctrl Pts',(62.9499316392037,-0.407728674576407,
14.1761656997206));
#24043=CARTESIAN_POINT('Ctrl Pts',(62.9480827837869,0.00102651687048705,
14.1540747194623));
#24044=CARTESIAN_POINT('Origin',(65.,0.,23.5459252805377));
#24045=CARTESIAN_POINT('',(62.9418498698494,8.27718827440684E-6,15.5540747194623));
#24046=CARTESIAN_POINT('',(62.9484914975566,0.000468974127544061,15.4959252805377));
#24047=CARTESIAN_POINT('',(62.94525,1.28744642201805E-13,23.5459252805377));
#24048=CARTESIAN_POINT('Ctrl Pts',(62.9484914975566,0.000468974127544111,
15.4959252805377));
#24049=CARTESIAN_POINT('Ctrl Pts',(62.9478504078462,0.31451301948094,15.4789613845241));
#24050=CARTESIAN_POINT('Ctrl Pts',(63.1632430376845,1.31353647315873,15.4249515249878));
#24051=CARTESIAN_POINT('Ctrl Pts',(64.7178900651262,2.41220423477674,15.3338957019289));
#24052=CARTESIAN_POINT('Ctrl Pts',(66.8736278902366,1.54526173974448,15.2227578113608));
#24053=CARTESIAN_POINT('Ctrl Pts',(67.3144128645646,-0.736076372865367,
15.1116199207928));
#24054=CARTESIAN_POINT('Ctrl Pts',(65.6367894857436,-2.34367538861624,15.0004820302248));
#24055=CARTESIAN_POINT('Ctrl Pts',(63.4964372981478,-1.83465185719793,14.895250483473));
#24056=CARTESIAN_POINT('Ctrl Pts',(62.9487020162047,-0.571446388044015,
14.827064900244));
#24057=CARTESIAN_POINT('Ctrl Pts',(62.94372126594,0.00163389948556124,14.7959252805377));
#24058=CARTESIAN_POINT('Ctrl Pts',(62.9418498868449,8.27714690067514E-6,
15.5540747194623));
#24059=CARTESIAN_POINT('Ctrl Pts',(62.9418498603911,0.000451185307771551,
15.5540505953261));
#24060=CARTESIAN_POINT('Ctrl Pts',(62.9420505595996,0.681041096754115,15.5169805076671));
#24061=CARTESIAN_POINT('Ctrl Pts',(63.6841642251148,2.04129618504104,15.4428644564855));
#24062=CARTESIAN_POINT('Ctrl Pts',(66.0013718021885,2.21259314346663,15.3317265659175));
#24063=CARTESIAN_POINT('Ctrl Pts',(67.4020124146433,0.358678503164372,15.2205886753494));
#24064=CARTESIAN_POINT('Ctrl Pts',(66.6040638188323,-1.82353863480769,15.1094507847814));
#24065=CARTESIAN_POINT('Ctrl Pts',(64.3378974271891,-2.33665018787605,14.9983128942134));
#24066=CARTESIAN_POINT('Ctrl Pts',(63.0663265778663,-1.09149331437408,14.913187539107));
#24067=CARTESIAN_POINT('Ctrl Pts',(62.9448408697591,-0.205526654691508,
14.8651081475233));
#24068=CARTESIAN_POINT('Ctrl Pts',(62.946510263771,-0.00176526862452042,
14.8540747194623));
#24069=CARTESIAN_POINT('Origin',(65.,0.,23.5459252805377));
#24070=CARTESIAN_POINT('',(62.9465344116198,0.00176006504695819,16.2540747194623));
#24071=CARTESIAN_POINT('',(62.9454411297334,-0.00187890759640223,16.1959252805377));
#24072=CARTESIAN_POINT('',(62.94525,1.28744642201805E-13,23.5459252805377));
#24073=CARTESIAN_POINT('Ctrl Pts',(62.9454411297334,-0.0018789075964022,
16.1959252805377));
#24074=CARTESIAN_POINT('Ctrl Pts',(62.9501461271515,0.514927296910589,16.1679038323268));
#24075=CARTESIAN_POINT('Ctrl Pts',(63.4098006358751,1.7224375006787,16.1028364205933));
#24076=CARTESIAN_POINT('Ctrl Pts',(65.4379883182475,2.38882429960344,16.0007230453371));
#24077=CARTESIAN_POINT('Ctrl Pts',(67.24452629377,0.927586663439804,15.8895851547691));
#24078=CARTESIAN_POINT('Ctrl Pts',(66.996623898036,-1.3826815656909,15.7784472642011));
#24079=CARTESIAN_POINT('Ctrl Pts',(64.9211890049946,-2.42736567633038,15.667309373633));
#24080=CARTESIAN_POINT('Ctrl Pts',(63.223670707888,-1.42992668390708,15.5731353790785));
#24081=CARTESIAN_POINT('Ctrl Pts',(62.9492504273939,-0.37130020640541,15.5160073480468));
#24082=CARTESIAN_POINT('Ctrl Pts',(62.9484914975566,0.000468974127544111,
15.4959252805377));
#24083=CARTESIAN_POINT('Ctrl Pts',(62.9465344116198,0.00176006504695823,
16.2540747194623));
#24084=CARTESIAN_POINT('Ctrl Pts',(62.944864096038,0.206418574104773,16.2429930431288));
#24085=CARTESIAN_POINT('Ctrl Pts',(63.0670246817589,1.09329987115452,16.1948654032727));
#24086=CARTESIAN_POINT('Ctrl Pts',(64.3409338179361,2.33750843231645,16.1096917998938));
#24087=CARTESIAN_POINT('Ctrl Pts',(66.6064316564341,1.82145305641563,15.9985539093258));
#24088=CARTESIAN_POINT('Ctrl Pts',(67.401544381661,-0.361798958737837,15.8874160187577));
#24089=CARTESIAN_POINT('Ctrl Pts',(65.9984962989145,-2.2138922838142,15.7762781281897));
#24090=CARTESIAN_POINT('Ctrl Pts',(63.6820161659208,-2.03962273041628,15.6651643617579));
#24091=CARTESIAN_POINT('Ctrl Pts',(62.9418904838623,-0.679695842678602,
15.5910965588488));
#24092=CARTESIAN_POINT('Ctrl Pts',(62.9418498868449,8.27714690067514E-6,
15.5540747194623));
#24093=CARTESIAN_POINT('Origin',(65.,0.,23.5459252805377));
#24094=CARTESIAN_POINT('',(62.9480689459238,-0.00103910400150425,16.9540747194623));
#24095=CARTESIAN_POINT('',(62.9421231189799,0.000678771108096866,16.8959252805377));
#24096=CARTESIAN_POINT('',(62.94525,1.28744642201805E-13,23.5459252805377));
#24097=CARTESIAN_POINT('Ctrl Pts',(62.9421231189799,0.000678771108097069,
16.8959252805377));
#24098=CARTESIAN_POINT('Ctrl Pts',(62.9419623987169,0.0380176929103635,
16.8938922436523));
#24099=CARTESIAN_POINT('Ctrl Pts',(62.9598052246296,0.755589108274135,16.8548132432442));
#24100=CARTESIAN_POINT('Ctrl Pts',(63.7964607753782,2.1094569529468,16.7786882793134));
#24101=CARTESIAN_POINT('Ctrl Pts',(66.119540899393,2.15521309297247,16.6675503887454));
#24102=CARTESIAN_POINT('Ctrl Pts',(67.4178925417354,0.228278247224652,16.5564124981773));
#24103=CARTESIAN_POINT('Ctrl Pts',(66.5031197198625,-1.90760226706539,16.4452746076093));
#24104=CARTESIAN_POINT('Ctrl Pts',(64.2125243718594,-2.29743279261728,16.3341367170413));
#24105=CARTESIAN_POINT('Ctrl Pts',(63.0385141433925,-1.01630861777053,16.251020274684));
#24106=CARTESIAN_POINT('Ctrl Pts',(62.9439258504044,-0.168320180393539,
16.2049497958495));
#24107=CARTESIAN_POINT('Ctrl Pts',(62.9454411297334,-0.0018789075964022,
16.1959252805377));
#24108=CARTESIAN_POINT('Ctrl Pts',(62.9480689459238,-0.00103910400150412,
16.9540747194623));
#24109=CARTESIAN_POINT('Ctrl Pts',(62.9499449184218,0.408602185927949,16.9319354909316));
#24110=CARTESIAN_POINT('Ctrl Pts',(63.2673355867028,1.50638090616108,16.8727502988781));
#24111=CARTESIAN_POINT('Ctrl Pts',(65.0557052990257,2.42800552371272,16.776519143302));
#24112=CARTESIAN_POINT('Ctrl Pts',(67.0701156187118,1.27001386948508,16.665381252734));
#24113=CARTESIAN_POINT('Ctrl Pts',(67.1897256358837,-1.05043588241968,16.5542433621659));
#24114=CARTESIAN_POINT('Ctrl Pts',(65.3050549453524,-2.40940975839149,16.4431054715979));
#24115=CARTESIAN_POINT('Ctrl Pts',(63.3569278527547,-1.64741761903889,16.3430492573633));
#24116=CARTESIAN_POINT('Ctrl Pts',(62.9504479489003,-0.477753335721165,
16.2800390066515));
#24117=CARTESIAN_POINT('Ctrl Pts',(62.9465344116198,0.00176006504695823,
16.2540747194623));
#24118=CARTESIAN_POINT('Origin',(65.,0.,23.5459252805377));
#24119=CARTESIAN_POINT('',(62.9427422720288,-0.00120218122682567,17.6540747194623));
#24120=CARTESIAN_POINT('',(62.9474450730054,0.00145098026757097,17.5959252805377));
#24121=CARTESIAN_POINT('',(62.94525,1.28744642201805E-13,23.5459252805377));
#24122=CARTESIAN_POINT('Ctrl Pts',(62.9474450730054,0.00145098026757093,
17.5959252805377));
#24123=CARTESIAN_POINT('Ctrl Pts',(62.9458669586282,0.243481142931844,17.582834691455));
#24124=CARTESIAN_POINT('Ctrl Pts',(63.0973769195488,1.16853721152032,17.5326981388497));
#24125=CARTESIAN_POINT('Ctrl Pts',(64.4682857559272,2.3697247232932,17.4455156227217));
#24126=CARTESIAN_POINT('Ctrl Pts',(66.7025669780829,1.73192984461804,17.3343777321536));
#24127=CARTESIAN_POINT('Ctrl Pts',(67.3784693367765,-0.491120062256288,
17.2232398415856));
#24128=CARTESIAN_POINT('Ctrl Pts',(65.8773317378418,-2.26464220646722,17.1121019510175));
#24129=CARTESIAN_POINT('Ctrl Pts',(63.6153124412349,-1.97078728704393,17.0029970973349));
#24130=CARTESIAN_POINT('Ctrl Pts',(62.9448910406138,-0.642371504646379,
16.930938207175));
#24131=CARTESIAN_POINT('Ctrl Pts',(62.9421231189799,0.000678771108097069,
16.8959252805377));
#24132=CARTESIAN_POINT('Ctrl Pts',(62.9427422720288,-0.00120218122682566,
17.6540747194623));
#24133=CARTESIAN_POINT('Ctrl Pts',(62.9469836764117,0.60897790221346,17.6208779387343));
#24134=CARTESIAN_POINT('Ctrl Pts',(63.5579942556341,1.90746584530599,17.5506351944836));
#24135=CARTESIAN_POINT('Ctrl Pts',(65.7655743703156,2.30482315743208,17.4433464867103));
#24136=CARTESIAN_POINT('Ctrl Pts',(67.3516166417705,0.606805630879791,17.3322085961422));
#24137=CARTESIAN_POINT('Ctrl Pts',(66.7851975318663,-1.64662797126069,17.2210707055742));
#24138=CARTESIAN_POINT('Ctrl Pts',(64.5847668755277,-2.39288431727495,17.1099328150062));
#24139=CARTESIAN_POINT('Ctrl Pts',(63.1270293146865,-1.23655417501041,17.0209341529689));
#24140=CARTESIAN_POINT('Ctrl Pts',(62.9468058203889,-0.276857845483467,
16.9689814544543));
#24141=CARTESIAN_POINT('Ctrl Pts',(62.9480689459238,-0.00103910400150412,
16.9540747194623));
#24142=CARTESIAN_POINT('Origin',(65.,0.,23.5459252805377));
#24143=CARTESIAN_POINT('',(62.9444267867382,0.0017991321662697,18.3540747194623));
#24144=CARTESIAN_POINT('',(62.9473667479389,-0.00148795945043145,18.2959252805377));
#24145=CARTESIAN_POINT('',(62.94525,1.28744642201805E-13,23.5459252805377));
#24146=CARTESIAN_POINT('Ctrl Pts',(62.9473667479389,-0.00148795945043152,
18.2959252805377));
#24147=CARTESIAN_POINT('Ctrl Pts',(62.9503594142629,0.444940986140609,18.2717771392578));
#24148=CARTESIAN_POINT('Ctrl Pts',(63.3129997156342,1.58066882860309,18.2105830344552));
#24149=CARTESIAN_POINT('Ctrl Pts',(65.1869048686148,2.42144210577608,18.1123429661299));
#24150=CARTESIAN_POINT('Ctrl Pts',(67.1357566643205,1.15622609049767,18.0012050755618));
#24151=CARTESIAN_POINT('Ctrl Pts',(67.1297261640456,-1.16729677790885,17.8900671849939));
#24152=CARTESIAN_POINT('Ctrl Pts',(65.1743331530824,-2.42237966744962,17.7789292944258));
#24153=CARTESIAN_POINT('Ctrl Pts',(63.3084858902886,-1.57355950027139,17.6808819929404));
#24154=CARTESIAN_POINT('Ctrl Pts',(62.9503329736625,-0.441456755648323,
17.6198806549777));
#24155=CARTESIAN_POINT('Ctrl Pts',(62.9474450730054,0.00145098026757093,
17.5959252805377));
#24156=CARTESIAN_POINT('Ctrl Pts',(62.9444267867382,0.00179913216626967,
18.3540747194623));
#24157=CARTESIAN_POINT('Ctrl Pts',(62.9432099184932,0.134576597368968,18.3468663500598));
#24158=CARTESIAN_POINT('Ctrl Pts',(63.0154304430432,0.94841898130449,18.3026120171345));
#24159=CARTESIAN_POINT('Ctrl Pts',(64.1011546824859,2.25618948643599,18.2213117206866));
#24160=CARTESIAN_POINT('Ctrl Pts',(66.4080681763277,1.97880214127948,18.1101738301185));
#24161=CARTESIAN_POINT('Ctrl Pts',(67.4261608997972,-0.109805244932086,
17.9990359395505));
#24162=CARTESIAN_POINT('Ctrl Pts',(66.2235610371465,-2.09790664518147,17.8878980489825));
#24163=CARTESIAN_POINT('Ctrl Pts',(63.9010218810697,-2.16577030121656,17.7767601584144));
#24164=CARTESIAN_POINT('Ctrl Pts',(62.9776665752518,-0.823136293702506,
17.6988190485744));
#24165=CARTESIAN_POINT('Ctrl Pts',(62.9422504791375,-0.0719528572662064,
17.657923902257));
#24166=CARTESIAN_POINT('Ctrl Pts',(62.9427422720288,-0.00120218122682566,
17.6540747194623));
#24167=CARTESIAN_POINT('Origin',(65.,0.,23.5459252805377));
#24168=CARTESIAN_POINT('',(62.948587662066,7.8101556172383E-5,19.0540747194623));
#24169=CARTESIAN_POINT('',(62.9420758643114,-0.000617377060631522,18.9959252805377));
#24170=CARTESIAN_POINT('',(62.94525,1.28744642201805E-13,23.5459252805377));
#24171=CARTESIAN_POINT('Ctrl Pts',(62.9420758643114,-0.000617377060631477,
18.9959252805377));
#24172=CARTESIAN_POINT('Ctrl Pts',(62.9446352222011,0.645933688463614,18.9607195870605));
#24173=CARTESIAN_POINT('Ctrl Pts',(63.621561854257,1.97744992677629,18.8884679300607));
#24174=CARTESIAN_POINT('Ctrl Pts',(65.88907520037,2.26005765183973,18.7791703095382));
#24175=CARTESIAN_POINT('Ctrl Pts',(67.3809865945794,0.478767310881884,18.6680324189701));
#24176=CARTESIAN_POINT('Ctrl Pts',(66.6935539565454,-1.74074417931048,18.5568945284021));
#24177=CARTESIAN_POINT('Ctrl Pts',(64.4559921758773,-2.36693278080144,18.445756637834));
#24178=CARTESIAN_POINT('Ctrl Pts',(63.0943542721865,-1.16131696258989,18.3587668885459));
#24179=CARTESIAN_POINT('Ctrl Pts',(62.9457683276783,-0.239931205144687,
18.3088231027804));
#24180=CARTESIAN_POINT('Ctrl Pts',(62.9473667479389,-0.00148795945043152,
18.2959252805377));
#24181=CARTESIAN_POINT('Ctrl Pts',(62.948587662066,7.81015561724177E-5,
19.0540747194623));
#24182=CARTESIAN_POINT('Ctrl Pts',(62.9484730026856,0.338265299953978,19.0358087978625));
#24183=CARTESIAN_POINT('Ctrl Pts',(63.1876491089047,1.36219297688967,18.98049691274));
#24184=CARTESIAN_POINT('Ctrl Pts',(64.8026200998564,2.42061047643986,18.8881390640948));
#24185=CARTESIAN_POINT('Ctrl Pts',(66.9266433003906,1.47863433497921,18.7770011735268));
#24186=CARTESIAN_POINT('Ctrl Pts',(67.2871880384261,-0.816752582102671,
18.6658632829587));
#24187=CARTESIAN_POINT('Ctrl Pts',(65.5542436264288,-2.36455659820143,18.5547253923907));
#24188=CARTESIAN_POINT('Ctrl Pts',(63.4592956564195,-1.78804123877568,18.4507958712252));
#24189=CARTESIAN_POINT('Ctrl Pts',(62.9494637678869,-0.547806457359297,
18.3839123135824));
#24190=CARTESIAN_POINT('Ctrl Pts',(62.9444267867382,0.00179913216626967,
18.3540747194623));
#24191=CARTESIAN_POINT('Origin',(65.,0.,23.5459252805377));
#24192=CARTESIAN_POINT('',(62.9447134762142,-0.00183968268685886,19.7540747194623));
#24193=CARTESIAN_POINT('',(62.9455477186679,0.0018770222400039,19.6959252805377));
#24194=CARTESIAN_POINT('',(62.94525,1.28744642201805E-13,23.5459252805377));
#24195=CARTESIAN_POINT('Ctrl Pts',(62.9455477186679,0.00187702224000372,
19.6959252805377));
#24196=CARTESIAN_POINT('Ctrl Pts',(62.9440086170586,0.171896041847239,19.6867079983859));
#24197=CARTESIAN_POINT('Ctrl Pts',(63.0410778177033,1.02351952878433,19.6404447527115));
#24198=CARTESIAN_POINT('Ctrl Pts',(64.2244604721458,2.30148946126118,19.5571355435145));
#24199=CARTESIAN_POINT('Ctrl Pts',(66.5130014322595,1.89977418876314,19.4459976529464));
#24200=CARTESIAN_POINT('Ctrl Pts',(67.4166750228635,-0.240825944373849,
19.3348597623784));
#24201=CARTESIAN_POINT('Ctrl Pts',(66.1083385580613,-2.16099535909078,19.2237218718103));
#24202=CARTESIAN_POINT('Ctrl Pts',(63.7855272416616,-2.10318121447058,19.1125839812423));
#24203=CARTESIAN_POINT('Ctrl Pts',(62.9580113964128,-0.748427978399199,
19.0366517841514));
#24204=CARTESIAN_POINT('Ctrl Pts',(62.9419420816986,-0.0344138582905811,
18.9977655505832));
#24205=CARTESIAN_POINT('Ctrl Pts',(62.9420758643114,-0.000617377060631477,
18.9959252805377));
#24206=CARTESIAN_POINT('Ctrl Pts',(62.9447134762142,-0.00183968268685889,
19.7540747194623));
#24207=CARTESIAN_POINT('Ctrl Pts',(62.9497000514415,0.538489713183427,19.7247512456653));
#24208=CARTESIAN_POINT('Ctrl Pts',(63.44501294369,1.7695358622959,19.6583818083455));
#24209=CARTESIAN_POINT('Ctrl Pts',(65.5214561645339,2.37200281981328,19.5549664075031));
#24210=CARTESIAN_POINT('Ctrl Pts',(67.2756619344365,0.848337588988218,19.443828516935));
#24211=CARTESIAN_POINT('Ctrl Pts',(66.9469285261459,-1.45182065545646,19.332690626367));
#24212=CARTESIAN_POINT('Ctrl Pts',(64.8361493591312,-2.42311099039749,19.221552735799));
#24213=CARTESIAN_POINT('Ctrl Pts',(63.1976100342287,-1.38138540402114,19.1286807668307));
#24214=CARTESIAN_POINT('Ctrl Pts',(62.9487055486976,-0.347627856173908,
19.0728547613852));
#24215=CARTESIAN_POINT('Ctrl Pts',(62.948587662066,7.81015561724177E-5,
19.0540747194623));
#24216=CARTESIAN_POINT('Origin',(65.,0.,23.5459252805377));
#24217=CARTESIAN_POINT('',(62.9425383451584,0.00106562935659804,20.4540747194623));
#24218=CARTESIAN_POINT('',(62.9484657349091,-0.000525555021677807,20.3959252805377));
#24219=CARTESIAN_POINT('',(62.94525,1.28744642201805E-13,23.5459252805377));
#24220=CARTESIAN_POINT('Ctrl Pts',(62.9484657349091,-0.000525555021677684,
20.3959252805377));
#24221=CARTESIAN_POINT('Ctrl Pts',(62.9493249615497,0.3748004665574,20.3756504461887));
#24222=CARTESIAN_POINT('Ctrl Pts',(63.2276318468978,1.43710439466948,20.318329648317));
#24223=CARTESIAN_POINT('Ctrl Pts',(64.9337900137556,2.42774204026718,20.2239628869227));
#24224=CARTESIAN_POINT('Ctrl Pts',(67.0037742079544,1.37229889524427,20.1128249963547));
#24225=CARTESIAN_POINT('Ctrl Pts',(67.2396811477566,-0.939225037877053,
20.0016871057866));
#24226=CARTESIAN_POINT('Ctrl Pts',(65.4255825320509,-2.39106561893279,19.8905492152186));
#24227=CARTESIAN_POINT('Ctrl Pts',(63.4047034238819,-1.71543774995268,19.7886286068023));
#24228=CARTESIAN_POINT('Ctrl Pts',(62.9501945513868,-0.511441876516717,
19.7237539619086));
#24229=CARTESIAN_POINT('Ctrl Pts',(62.9455477186679,0.00187702224000372,
19.6959252805377));
#24230=CARTESIAN_POINT('Ctrl Pts',(62.9425383451584,0.00106562935659771,
20.4540747194623));
#24231=CARTESIAN_POINT('Ctrl Pts',(62.9421515159492,0.0623504207905263,
20.4507396569907));
#24232=CARTESIAN_POINT('Ctrl Pts',(62.9724324501069,0.804000733271032,20.4103586309964));
#24233=CARTESIAN_POINT('Ctrl Pts',(63.8711449203827,2.15034861017487,20.3329316414794));
#24234=CARTESIAN_POINT('Ctrl Pts',(66.1944008109328,2.11464436694832,20.2217937509113));
#24235=CARTESIAN_POINT('Ctrl Pts',(67.4244083164919,0.143381864737545,20.1106558603433));
#24236=CARTESIAN_POINT('Ctrl Pts',(66.4353272830534,-1.95911953903995,19.9995179697752));
#24237=CARTESIAN_POINT('Ctrl Pts',(64.132474966303,-2.26841668404625,19.8883800792072));
#24238=CARTESIAN_POINT('Ctrl Pts',(63.0217706588138,-0.967627859876295,
19.8065656624362));
#24239=CARTESIAN_POINT('Ctrl Pts',(62.9434002356266,-0.144138246524576,
19.7617972091879));
#24240=CARTESIAN_POINT('Ctrl Pts',(62.9447134762142,-0.00183968268685889,
19.7540747194623));
#24241=CARTESIAN_POINT('Origin',(65.,0.,23.5459252805377));
#24242=CARTESIAN_POINT('',(62.9479182248742,0.00116161895481429,21.1540747194623));
#24243=CARTESIAN_POINT('',(62.9436210622307,-0.00160392935065391,21.0959252805377));
#24244=CARTESIAN_POINT('',(62.94525,1.28744642201805E-13,23.5459252805377));
#24245=CARTESIAN_POINT('Ctrl Pts',(62.9436210622307,-0.00160392935065416,
21.0959252805377));
#24246=CARTESIAN_POINT('Ctrl Pts',(62.9485686759719,0.574950681266289,21.0645928939915));
#24247=CARTESIAN_POINT('Ctrl Pts',(63.5020551216143,1.84152256699688,20.9962145439225));
#24248=CARTESIAN_POINT('Ctrl Pts',(65.6489465241691,2.34033682721966,20.8907902303309));
#24249=CARTESIAN_POINT('Ctrl Pts',(67.3182024564633,0.724053604371175,20.7796523397629));
#24250=CARTESIAN_POINT('Ctrl Pts',(66.865581542071,-1.55496692328425,20.6685144491949));
#24251=CARTESIAN_POINT('Ctrl Pts',(64.7053726085262,-2.41070716562325,20.5573765586268));
#24252=CARTESIAN_POINT('Ctrl Pts',(63.1597285921146,-1.30632755500751,20.4665135024078));
#24253=CARTESIAN_POINT('Ctrl Pts',(62.9477549916925,-0.310991282228732,
20.4126964097114));
#24254=CARTESIAN_POINT('Ctrl Pts',(62.9484657349091,-0.000525555021677684,
20.3959252805377));
#24255=CARTESIAN_POINT('Ctrl Pts',(62.9479182248742,0.00116161895481415,
21.1540747194623));
#24256=CARTESIAN_POINT('Ctrl Pts',(62.9465403381585,0.26742114595832,21.1396821047934));
#24257=CARTESIAN_POINT('Ctrl Pts',(63.1184075387479,1.2173158745075,21.0882435266019));
#24258=CARTESIAN_POINT('Ctrl Pts',(64.5516876929394,2.3868968681091,20.9997589848876));
#24259=CARTESIAN_POINT('Ctrl Pts',(66.7622271403759,1.67118893435552,20.8886210943196));
#24260=CARTESIAN_POINT('Ctrl Pts',(67.3597936726881,-0.574194749175797,
20.7774832037516));
#24261=CARTESIAN_POINT('Ctrl Pts',(65.7974074532359,-2.2940026123021,20.6663453131835));
#24262=CARTESIAN_POINT('Ctrl Pts',(63.573935456952,-1.92548892520573,20.5585424850871));
#24263=CARTESIAN_POINT('Ctrl Pts',(62.9464484251963,-0.618402688713485,
20.4877856205134));
#24264=CARTESIAN_POINT('Ctrl Pts',(62.9425383451584,0.00106562935659771,
20.4540747194623));
#24265=CARTESIAN_POINT('Origin',(65.,0.,23.5459252805377));
#24266=CARTESIAN_POINT('',(62.9473239618077,-0.00235074752840472,21.8540747194623));
#24267=CARTESIAN_POINT('',(62.9434348764936,0.00149614206266628,21.7959252805377));
#24268=CARTESIAN_POINT('',(62.94525,1.28744642201805E-13,23.5459252805377));
#24269=CARTESIAN_POINT('',(64.4698297828114,-1.98517432567172,22.));
#24270=CARTESIAN_POINT('Ctrl Pts',(64.4698297828114,-1.98517432567172,22.));
#24271=CARTESIAN_POINT('Ctrl Pts',(63.8097120902545,-1.80888011517989,21.9629540364773));
#24272=CARTESIAN_POINT('Ctrl Pts',(63.0750422655367,-1.11280694816751,21.9143122762981));
#24273=CARTESIAN_POINT('Ctrl Pts',(62.9457054195483,-0.216594706141779,
21.8656705161189));
#24274=CARTESIAN_POINT('Ctrl Pts',(62.9473239618077,-0.00235074752840471,
21.8540747194623));
#24275=CARTESIAN_POINT('',(65.5313040526013,-1.98873440678485,22.));
#24276=CARTESIAN_POINT('Origin',(65.,0.,22.));
#24277=CARTESIAN_POINT('Ctrl Pts',(65.5313046873329,-1.98873639975131,22.));
#24278=CARTESIAN_POINT('Ctrl Pts',(64.8866967734446,-2.16006352763733,21.9636770818144));
#24279=CARTESIAN_POINT('Ctrl Pts',(63.5069411366323,-1.84063802220702,21.895652175327));
#24280=CARTESIAN_POINT('Ctrl Pts',(62.9482922133912,-0.581586231880544,
21.8276272688395));
#24281=CARTESIAN_POINT('Ctrl Pts',(62.9434348764936,0.0014961420626663,
21.7959252805377));
#24282=CARTESIAN_POINT('Origin',(65.,0.,3.));
#24283=CARTESIAN_POINT('',(66.6675465985015,-0.0012143044629161,6.12851963660979));
#24284=CARTESIAN_POINT('',(66.6679935094968,0.00096847687651065,6.32148036339021));
#24285=CARTESIAN_POINT('',(66.666,2.04026156737949E-16,3.));
#24286=CARTESIAN_POINT('',(66.6351293272515,-0.319230454628274,7.));
#24287=CARTESIAN_POINT('Ctrl Pts',(66.6679935094968,0.00096847687651065,
6.32148036339021));
#24288=CARTESIAN_POINT('Ctrl Pts',(66.6684011451999,0.0590543694261956,
6.32537779445739));
#24289=CARTESIAN_POINT('Ctrl Pts',(66.6656310767024,0.117101359876407,6.32927522552457));
#24290=CARTESIAN_POINT('Ctrl Pts',(66.6595549679121,0.174800485042606,6.33317265659175));
#24291=CARTESIAN_POINT('Ctrl Pts',(66.6018001800214,0.723243715815273,6.37021862011443));
#24292=CARTESIAN_POINT('Ctrl Pts',(66.2453468888446,1.24025755357674,6.40726458363711));
#24293=CARTESIAN_POINT('Ctrl Pts',(65.7532186868383,1.48913446656882,6.44431054715979));
#24294=CARTESIAN_POINT('Ctrl Pts',(65.261090484832,1.73801137956089,6.48135651068247));
#24295=CARTESIAN_POINT('Ctrl Pts',(64.6332873719962,1.71875136778355,6.51840247420515));
#24296=CARTESIAN_POINT('Ctrl Pts',(64.1573426907198,1.44035276658659,6.55544843772783));
#24297=CARTESIAN_POINT('Ctrl Pts',(63.6813980094435,1.16195416538963,6.59249440125051));
#24298=CARTESIAN_POINT('Ctrl Pts',(63.3573117597265,0.624416974773041,6.6295403647732));
#24299=CARTESIAN_POINT('Ctrl Pts',(63.3329761432024,0.0733847413024343,
6.66658632829588));
#24300=CARTESIAN_POINT('Ctrl Pts',(63.3086405266783,-0.477647492168164,
6.70363229181856));
#24301=CARTESIAN_POINT('Ctrl Pts',(63.5840555433469,-1.04217476849279,6.74067825534123));
#24302=CARTESIAN_POINT('Ctrl Pts',(64.0340468080883,-1.36111204342973,6.77772421886391));
#24303=CARTESIAN_POINT('Ctrl Pts',(64.4840380728297,-1.68004931836668,6.81477018238659));
#24304=CARTESIAN_POINT('Ctrl Pts',(65.1086055856438,-1.75339659191593,6.85181614590928));
#24305=CARTESIAN_POINT('Ctrl Pts',(65.6198404690058,-1.54912172664724,6.88886210943196));
#24306=CARTESIAN_POINT('Ctrl Pts',(66.1310753523678,-1.34484686137855,6.92590807295464));
#24307=CARTESIAN_POINT('Ctrl Pts',(66.5289776062776,-0.862949857291923,
6.96295403647732));
#24308=CARTESIAN_POINT('Ctrl Pts',(66.6351293272514,-0.319230454628298,
7.));
#24309=CARTESIAN_POINT('',(65.0525836066607,1.66819787866867,7.));
#24310=CARTESIAN_POINT('Origin',(65.,0.,7.));
#24311=CARTESIAN_POINT('',(66.6634369488939,-0.000652451249335551,6.82851963660979));
#24312=CARTESIAN_POINT('Ctrl Pts',(65.0525835864496,1.66819940096574,7.));
#24313=CARTESIAN_POINT('Ctrl Pts',(65.5930952523355,1.65047433913271,6.96367708181444));
#24314=CARTESIAN_POINT('Ctrl Pts',(66.1251624614536,1.34576660284025,6.92735416362889));
#24315=CARTESIAN_POINT('Ctrl Pts',(66.412840678391,0.887825324655541,6.89103124544334));
#24316=CARTESIAN_POINT('Ctrl Pts',(66.5778717300928,0.625120238531672,6.87019404249883));
#24317=CARTESIAN_POINT('Ctrl Pts',(66.6624763097416,0.311987213470675,6.84935683955431));
#24318=CARTESIAN_POINT('Ctrl Pts',(66.6634369488939,-0.000652451249335551,
6.82851963660979));
#24319=CARTESIAN_POINT('',(66.666,-2.04026156737949E-16,8.));
#24320=CARTESIAN_POINT('',(66.666,2.04026156737949E-16,3.));
#24321=CARTESIAN_POINT('Origin',(65.,0.,8.));
#24322=CARTESIAN_POINT('Ctrl Pts',(66.6634369488939,-0.000652451249335551,
6.82851963660979));
#24323=CARTESIAN_POINT('Ctrl Pts',(66.6641842070583,-0.243847350592474,
6.81231087603163));
#24324=CARTESIAN_POINT('Ctrl Pts',(66.614319260528,-0.486743721979875,6.79610211545346));
#24325=CARTESIAN_POINT('Ctrl Pts',(66.5123276923829,-0.705373629571154,
6.7798933548753));
#24326=CARTESIAN_POINT('Ctrl Pts',(66.2792206701092,-1.20506363008265,6.74284739135262));
#24327=CARTESIAN_POINT('Ctrl Pts',(65.7738173393357,-1.57799175139799,6.70580142782994));
#24328=CARTESIAN_POINT('Ctrl Pts',(65.2274915068526,-1.65321113835932,6.66875546430726));
#24329=CARTESIAN_POINT('Ctrl Pts',(64.6811656743696,-1.72843052532064,6.63170950078458));
#24330=CARTESIAN_POINT('Ctrl Pts',(64.0939173401772,-1.50594117792796,6.5946635372619));
#24331=CARTESIAN_POINT('Ctrl Pts',(63.734467017542,-1.08770559986528,6.55761757373921));
#24332=CARTESIAN_POINT('Ctrl Pts',(63.3750166949069,-0.669470021802595,
6.52057161021653));
#24333=CARTESIAN_POINT('Ctrl Pts',(63.2433643838291,-0.0554882130699084,
6.48352564669385));
#24334=CARTESIAN_POINT('Ctrl Pts',(63.3997802821251,0.473318066669373,6.44647968317117));
#24335=CARTESIAN_POINT('Ctrl Pts',(63.556196180421,1.00212434640864,6.40943371964849));
#24336=CARTESIAN_POINT('Ctrl Pts',(64.0006802880906,1.44575509715451,6.37238775612581));
#24337=CARTESIAN_POINT('Ctrl Pts',(64.5298024116317,1.6011444312508,6.33534179260313));
#24338=CARTESIAN_POINT('Ctrl Pts',(65.0589245351728,1.7565337653471,6.29829582908045));
#24339=CARTESIAN_POINT('Ctrl Pts',(65.6726846745854,1.62368168279382,6.26124986555777));
#24340=CARTESIAN_POINT('Ctrl Pts',(66.0901968514498,1.26340683134223,6.22420390203509));
#24341=CARTESIAN_POINT('Ctrl Pts',(66.4496543303097,0.953227878546208,6.19230914689332));
#24342=CARTESIAN_POINT('Ctrl Pts',(66.6636456701669,0.474474884606731,6.16041439175156));
#24343=CARTESIAN_POINT('Ctrl Pts',(66.6675465985015,-0.0012143044629161,
6.12851963660979));
#24344=CARTESIAN_POINT('Origin',(65.,0.,3.));
#24345=CARTESIAN_POINT('',(66.6672347084384,0.00132477166025269,5.42851963660979));
#24346=CARTESIAN_POINT('',(66.6636987213601,0.0008322902000487,5.62148036339021));
#24347=CARTESIAN_POINT('',(66.666,2.04026156737949E-16,3.));
#24348=CARTESIAN_POINT('Ctrl Pts',(66.6636987213601,0.0008322902000487,
5.62148036339021));
#24349=CARTESIAN_POINT('Ctrl Pts',(66.6647135334695,0.225194170777295,5.63643534665464));
#24350=CARTESIAN_POINT('Ctrl Pts',(66.6225044629126,0.449190113916435,5.65139032991907));
#24351=CARTESIAN_POINT('Ctrl Pts',(66.5352578465541,0.65400067617093,5.6663453131835));
#24352=CARTESIAN_POINT('Ctrl Pts',(66.3191335681149,1.16135026554737,5.70339127670618));
#24353=CARTESIAN_POINT('Ctrl Pts',(65.8266432700797,1.55097169600335,5.74043724022886));
#24354=CARTESIAN_POINT('Ctrl Pts',(65.2831760713863,1.64455092497836,5.77748320375154));
#24355=CARTESIAN_POINT('Ctrl Pts',(64.739708872693,1.73813015395337,5.81452916727422));
#24356=CARTESIAN_POINT('Ctrl Pts',(64.1452647733414,1.53566718144742,5.8515751307969));
#24357=CARTESIAN_POINT('Ctrl Pts',(63.771898150977,1.12982346148107,5.88862109431958));
#24358=CARTESIAN_POINT('Ctrl Pts',(63.3985315286127,0.72397974151472,5.92566705784226));
#24359=CARTESIAN_POINT('Ctrl Pts',(63.2462423832356,0.114755274087973,5.96271302136494));
#24360=CARTESIAN_POINT('Ctrl Pts',(63.3847194791661,-0.419041074004903,
5.99975898488762));
#24361=CARTESIAN_POINT('Ctrl Pts',(63.5231965750967,-0.952837422097788,
6.0368049484103));
#24362=CARTESIAN_POINT('Ctrl Pts',(63.952439912335,-1.41120565085679,6.07385091193298));
#24363=CARTESIAN_POINT('Ctrl Pts',(64.4760180935273,-1.58435878418327,6.11089687545566));
#24364=CARTESIAN_POINT('Ctrl Pts',(64.9995962747196,-1.75751191750976,6.14794283897834));
#24365=CARTESIAN_POINT('Ctrl Pts',(65.6175092998659,-1.64544995540374,6.18498880250103));
#24366=CARTESIAN_POINT('Ctrl Pts',(66.0469376701368,-1.29948266245882,6.22203476602371));
#24367=CARTESIAN_POINT('Ctrl Pts',(66.431187907292,-0.989912956390696,6.25518329847921));
#24368=CARTESIAN_POINT('Ctrl Pts',(66.6645264756734,-0.49306517277657,6.28833183093471));
#24369=CARTESIAN_POINT('Ctrl Pts',(66.6679935094968,0.00096847687651065,
6.32148036339021));
#24370=CARTESIAN_POINT('Ctrl Pts',(66.6675465985015,-0.0012143044629161,
6.12851963660979));
#24371=CARTESIAN_POINT('Ctrl Pts',(66.6681766235524,-0.0780411722834827,
6.12336842822888));
#24372=CARTESIAN_POINT('Ctrl Pts',(66.6633265808958,-0.154788122805552,
6.11821721984797));
#24373=CARTESIAN_POINT('Ctrl Pts',(66.6527242222132,-0.230732082280714,
6.11306601146705));
#24374=CARTESIAN_POINT('Ctrl Pts',(66.5764752017958,-0.776898524102169,
6.07602004794437));
#24375=CARTESIAN_POINT('Ctrl Pts',(66.202712946645,-1.2815337873952,6.03897408442169));
#24376=CARTESIAN_POINT('Ctrl Pts',(65.7024931149025,-1.51368401519416,6.00192812089901));
#24377=CARTESIAN_POINT('Ctrl Pts',(65.20227328316,-1.74583424299313,5.96488215737633));
#24378=CARTESIAN_POINT('Ctrl Pts',(64.5755958748258,-1.70549943529801,5.92783619385365));
#24379=CARTESIAN_POINT('Ctrl Pts',(64.1092627289642,-1.41114141304213,5.89079023033097));
#24380=CARTESIAN_POINT('Ctrl Pts',(63.6429295831026,-1.11678339078625,5.85374426680829));
#24381=CARTESIAN_POINT('Ctrl Pts',(63.3369406997136,-0.568402153969608,
5.81669830328561));
#24382=CARTESIAN_POINT('Ctrl Pts',(63.3313339461091,-0.0169662842418651,
5.77965233976292));
#24383=CARTESIAN_POINT('Ctrl Pts',(63.3257271925045,0.534469585485878,5.74260637624024));
#24384=CARTESIAN_POINT('Ctrl Pts',(63.6205025686844,1.08896008812472,5.70556041271756));
#24385=CARTESIAN_POINT('Ctrl Pts',(64.0807542900534,1.39273889179928,5.66851444919488));
#24386=CARTESIAN_POINT('Ctrl Pts',(64.5410060114225,1.69651769547383,5.6314684856722));
#24387=CARTESIAN_POINT('Ctrl Pts',(65.1667340779808,1.7495848001841,5.59442252214952));
#24388=CARTESIAN_POINT('Ctrl Pts',(65.6715705742232,1.52765405355124,5.55737655862684));
#24389=CARTESIAN_POINT('Ctrl Pts',(66.1764070704656,1.30572330691839,5.52033059510416));
#24390=CARTESIAN_POINT('Ctrl Pts',(66.5603519963922,0.80879470894242,5.48328463158148));
#24391=CARTESIAN_POINT('Ctrl Pts',(66.6476907378026,0.264290293520936,5.4462386680588));
#24392=CARTESIAN_POINT('Ctrl Pts',(66.6616154028998,0.177478398750718,5.44033232424247));
#24393=CARTESIAN_POINT('Ctrl Pts',(66.6680006840388,0.0894571820797134,
5.43442598042613));
#24394=CARTESIAN_POINT('Ctrl Pts',(66.6672347084384,0.00132477166025269,
5.42851963660979));
#24395=CARTESIAN_POINT('Origin',(65.,0.,3.));
#24396=CARTESIAN_POINT('',(66.663366994258,0.000380245158983772,4.72851963660979));
#24397=CARTESIAN_POINT('',(66.664973747664,-0.00143128352026757,4.92148036339021));
#24398=CARTESIAN_POINT('',(66.666,2.04026156737949E-16,3.));
#24399=CARTESIAN_POINT('Ctrl Pts',(66.664973747664,-0.00143128352026757,
4.92148036339021));
#24400=CARTESIAN_POINT('Ctrl Pts',(66.6617826067969,0.38807005747555,4.94749289885189));
#24401=CARTESIAN_POINT('Ctrl Pts',(66.5254256665028,0.779584263278044,4.97350543431357));
#24402=CARTESIAN_POINT('Ctrl Pts',(66.27583338404,1.07563182061435,4.99951796977525));
#24403=CARTESIAN_POINT('Ctrl Pts',(65.9203745090186,1.49725035242627,5.03656393329793));
#24404=CARTESIAN_POINT('Ctrl Pts',(65.3352487301258,1.72524091300359,5.07360989682061));
#24405=CARTESIAN_POINT('Ctrl Pts',(64.7882421463444,1.65526230253066,5.11065586034329));
#24406=CARTESIAN_POINT('Ctrl Pts',(64.2412355625629,1.58528369205773,5.14770182386597));
#24407=CARTESIAN_POINT('Ctrl Pts',(63.7323481738928,1.21733591053454,5.18474778738865));
#24408=CARTESIAN_POINT('Ctrl Pts',(63.4944752416899,0.71981239976822,5.22179375091133));
#24409=CARTESIAN_POINT('Ctrl Pts',(63.256602309487,0.222288889001918,5.25883971443401));
#24410=CARTESIAN_POINT('Ctrl Pts',(63.2897438337514,-0.404810351007516,
5.29588567795669));
#24411=CARTESIAN_POINT('Ctrl Pts',(63.5787322850456,-0.874489902053352,
5.33293164147937));
#24412=CARTESIAN_POINT('Ctrl Pts',(63.8677207363397,-1.34416945309919,5.36997760500205));
#24413=CARTESIAN_POINT('Ctrl Pts',(64.4125561146635,-1.65642931518145,5.40702356852474));
#24414=CARTESIAN_POINT('Ctrl Pts',(64.9638916621075,-1.66836178497851,5.44406953204742));
#24415=CARTESIAN_POINT('Ctrl Pts',(65.5152272095514,-1.68029425477557,5.4811154955701));
#24416=CARTESIAN_POINT('Ctrl Pts',(66.0730629261155,-1.39189933228743,5.51816145909277));
#24417=CARTESIAN_POINT('Ctrl Pts',(66.382101654976,-0.935162996894911,5.55520742261545));
#24418=CARTESIAN_POINT('Ctrl Pts',(66.5663853881852,-0.662805298269937,
5.5772984028737));
#24419=CARTESIAN_POINT('Ctrl Pts',(66.6621996762674,-0.330587263195562,
5.59938938313196));
#24420=CARTESIAN_POINT('Ctrl Pts',(66.6636987213601,0.0008322902000487,
5.62148036339021));
#24421=CARTESIAN_POINT('Ctrl Pts',(66.6672347084384,0.00132477166025269,
5.42851963660979));
#24422=CARTESIAN_POINT('Ctrl Pts',(66.6631963067396,-0.463329814934398,
5.39738001690345));
#24423=CARTESIAN_POINT('Ctrl Pts',(66.4603784340712,-0.931075191763351,
5.3662403971971));
#24424=CARTESIAN_POINT('Ctrl Pts',(66.1156608616196,-1.24098144967673,5.33510077749075));
#24425=CARTESIAN_POINT('Ctrl Pts',(65.705559687132,-1.60966854458595,5.29805481396807));
#24426=CARTESIAN_POINT('Ctrl Pts',(65.0946247812625,-1.75496250153736,5.2610088504454));
#24427=CARTESIAN_POINT('Ctrl Pts',(64.5624539571804,-1.61036875759037,5.22396288692272));
#24428=CARTESIAN_POINT('Ctrl Pts',(64.0302831330983,-1.46577501364339,5.18691692340004));
#24429=CARTESIAN_POINT('Ctrl Pts',(63.5768763908035,-1.031293568798,5.14987095987736));
#24430=CARTESIAN_POINT('Ctrl Pts',(63.4097379023455,-0.505767299507011,
5.11282499635467));
#24431=CARTESIAN_POINT('Ctrl Pts',(63.2425994138875,0.019758969783971,5.07577903283199));
#24432=CARTESIAN_POINT('Ctrl Pts',(63.3617291792663,0.636330063520549,5.03873306930931));
#24433=CARTESIAN_POINT('Ctrl Pts',(63.7126067830815,1.06176871408086,5.00168710578663));
#24434=CARTESIAN_POINT('Ctrl Pts',(64.0634843868967,1.48720736464117,4.96464114226395));
#24435=CARTESIAN_POINT('Ctrl Pts',(64.6461098291483,1.72151357202522,4.92759517874127));
#24436=CARTESIAN_POINT('Ctrl Pts',(65.1938412738804,1.65745577708112,4.89054921521859));
#24437=CARTESIAN_POINT('Ctrl Pts',(65.7415727186126,1.59339798213702,4.85350325169591));
#24438=CARTESIAN_POINT('Ctrl Pts',(66.2544101658253,1.23097618486478,4.81645728817322));
#24439=CARTESIAN_POINT('Ctrl Pts',(66.4976506491047,0.73605477318722,4.77941132465054));
#24440=CARTESIAN_POINT('Ctrl Pts',(66.6090340731616,0.509422920098692,4.76244742863696));
#24441=CARTESIAN_POINT('Ctrl Pts',(66.6638867910221,0.255007754231684,4.74548353262337));
#24442=CARTESIAN_POINT('Ctrl Pts',(66.663366994258,0.000380245158983772,
4.72851963660979));
#24443=CARTESIAN_POINT('Origin',(65.,0.,3.));
#24444=CARTESIAN_POINT('',(66.66584023827,-0.00152342185141638,4.02851963660979));
#24445=CARTESIAN_POINT('',(66.668752404953,6.71116607201819E-6,4.22148036339021));
#24446=CARTESIAN_POINT('',(66.666,2.04026156737949E-16,3.));
#24447=CARTESIAN_POINT('Ctrl Pts',(66.6687523910643,6.71113220718263E-6,
4.22148036339021));
#24448=CARTESIAN_POINT('Ctrl Pts',(66.6687853501023,0.551830446441275,4.25855045104914));
#24449=CARTESIAN_POINT('Ctrl Pts',(66.3679399440666,1.10362329032225,4.29562053870807));
#24450=CARTESIAN_POINT('Ctrl Pts',(65.9041274583633,1.40260051189836,4.332690626367));
#24451=CARTESIAN_POINT('Ctrl Pts',(65.440616808353,1.70138316778325,4.36973658988968));
#24452=CARTESIAN_POINT('Ctrl Pts',(64.8143512345865,1.74767914449738,4.40678255341236));
#24453=CARTESIAN_POINT('Ctrl Pts',(64.3119447275275,1.52030082532265,4.44382851693504));
#24454=CARTESIAN_POINT('Ctrl Pts',(63.8095382204685,1.29292250614791,4.48087448045772));
#24455=CARTESIAN_POINT('Ctrl Pts',(63.430990780117,0.79186989108431,4.5179204439804));
#24456=CARTESIAN_POINT('Ctrl Pts',(63.3495467901205,0.246452551482041,4.55496640750308));
#24457=CARTESIAN_POINT('Ctrl Pts',(63.2681028001239,-0.298964788120227,
4.59201237102576));
#24458=CARTESIAN_POINT('Ctrl Pts',(63.4837622604823,-0.888746852261164,
4.62905833454844));
#24459=CARTESIAN_POINT('Ctrl Pts',(63.897827394199,-1.25297653677901,4.66610429807112));
#24460=CARTESIAN_POINT('Ctrl Pts',(64.3118925279157,-1.61720622129685,4.7031502615938));
#24461=CARTESIAN_POINT('Ctrl Pts',(64.9243633349907,-1.75588352619159,4.74019622511648));
#24462=CARTESIAN_POINT('Ctrl Pts',(65.4549390817441,-1.60554199300636,4.77724218863916));
#24463=CARTESIAN_POINT('Ctrl Pts',(65.9855148284976,-1.45520045982112,4.81428815216184));
#24464=CARTESIAN_POINT('Ctrl Pts',(66.4341955149294,-1.0158400885559,4.85133411568453));
#24465=CARTESIAN_POINT('Ctrl Pts',(66.5956398725704,-0.488536651400016,
4.88838007920721));
#24466=CARTESIAN_POINT('Ctrl Pts',(66.6437229708759,-0.331489459561807,
4.89941350726821));
#24467=CARTESIAN_POINT('Ctrl Pts',(66.6663272959654,-0.166641438903674,
4.91044693532921));
#24468=CARTESIAN_POINT('Ctrl Pts',(66.664973747664,-0.00143128352026757,
4.92148036339021));
#24469=CARTESIAN_POINT('Ctrl Pts',(66.663366994258,0.000380245158983772,
4.72851963660979));
#24470=CARTESIAN_POINT('Ctrl Pts',(66.6627516524935,-0.301050913271577,
4.7084375691007));
#24471=CARTESIAN_POINT('Ctrl Pts',(66.5845366381801,-0.602779651888649,
4.6883555015916));
#24472=CARTESIAN_POINT('Ctrl Pts',(66.4306434003258,-0.859065513400935,
4.66827343408251));
#24473=CARTESIAN_POINT('Ctrl Pts',(66.1467521489217,-1.33184336222865,4.63122747055983));
#24474=CARTESIAN_POINT('Ctrl Pts',(65.6053261267676,-1.6499780338012,4.59418150703714));
#24475=CARTESIAN_POINT('Ctrl Pts',(65.0541520228137,-1.66787339241419,4.55713554351446));
#24476=CARTESIAN_POINT('Ctrl Pts',(64.5029779188599,-1.68576875102718,4.52008957999178));
#24477=CARTESIAN_POINT('Ctrl Pts',(63.9420557331062,-1.4034247966806,4.4830436164691));
#24478=CARTESIAN_POINT('Ctrl Pts',(63.6280946846009,-0.950057840731758,
4.44599765294642));
#24479=CARTESIAN_POINT('Ctrl Pts',(63.3141336360955,-0.496690884782916,
4.40895168942374));
#24480=CARTESIAN_POINT('Ctrl Pts',(63.2471337248385,0.127699072768189,4.37190572590106));
#24481=CARTESIAN_POINT('Ctrl Pts',(63.4577578400848,0.637356427139633,4.33485976237838));
#24482=CARTESIAN_POINT('Ctrl Pts',(63.6683819553311,1.14701378151106,4.2978137988557));
#24483=CARTESIAN_POINT('Ctrl Pts',(64.1566300970808,1.54193853270284,4.26076783533302));
#24484=CARTESIAN_POINT('Ctrl Pts',(64.6990527347307,1.64139112904609,4.22372187181034));
#24485=CARTESIAN_POINT('Ctrl Pts',(65.2414753723806,1.74084372538933,4.18667590828766));
#24486=CARTESIAN_POINT('Ctrl Pts',(65.8380725059307,1.54482416688403,4.14962994476498));
#24487=CARTESIAN_POINT('Ctrl Pts',(66.2158080742639,1.14304191594115,4.1125839812423));
#24488=CARTESIAN_POINT('Ctrl Pts',(66.501526048881,0.839135107580338,4.08456253303146));
#24489=CARTESIAN_POINT('Ctrl Pts',(66.6620254174182,0.417504031348421,4.05654108482063));
#24490=CARTESIAN_POINT('Ctrl Pts',(66.66584023827,-0.00152342185141638,
4.02851963660979));
#24491=CARTESIAN_POINT('Origin',(65.,0.,3.));
#24492=CARTESIAN_POINT('',(66.6685304876972,0.000550348904958531,3.32851963660979));
#24493=CARTESIAN_POINT('',(66.6649541686305,0.00142706439964306,3.52148036339021));
#24494=CARTESIAN_POINT('',(66.666,2.04026156737949E-16,3.));
#24495=CARTESIAN_POINT('Ctrl Pts',(66.6649541686305,0.00142706439964306,
3.52148036339021));
#24496=CARTESIAN_POINT('Ctrl Pts',(66.6663084639771,0.16736460907033,3.53256203972371));
#24497=CARTESIAN_POINT('Ctrl Pts',(66.6435020576938,0.332938268252247,3.5436437160572));
#24498=CARTESIAN_POINT('Ctrl Pts',(66.5950038039968,0.490609337973574,3.5547253923907));
#24499=CARTESIAN_POINT('Ctrl Pts',(66.4328744940168,1.01770257925701,3.59177135591338));
#24500=CARTESIAN_POINT('Ctrl Pts',(65.9836233623828,1.45647963816643,3.62881731943606));
#24501=CARTESIAN_POINT('Ctrl Pts',(65.4528527369189,1.60613170566075,3.66586328295875));
#24502=CARTESIAN_POINT('Ctrl Pts',(64.9220821114551,1.75578377315508,3.70290924648143));
#24503=CARTESIAN_POINT('Ctrl Pts',(64.3097919921614,1.6163108492343,3.73995521000411));
#24504=CARTESIAN_POINT('Ctrl Pts',(63.8962004240445,1.25154350838824,3.77700117352679));
#24505=CARTESIAN_POINT('Ctrl Pts',(63.4826088559276,0.886776167542176,3.81404713704947));
#24506=CARTESIAN_POINT('Ctrl Pts',(63.2677158389876,0.29671440977082,3.85109310057215));
#24507=CARTESIAN_POINT('Ctrl Pts',(63.3498683809715,-0.248596655588643,
3.88813906409483));
#24508=CARTESIAN_POINT('Ctrl Pts',(63.4320209229553,-0.793907720948105,
3.92518502761751));
#24509=CARTESIAN_POINT('Ctrl Pts',(63.8112190238629,-1.29446809389567,3.96223099114019));
#24510=CARTESIAN_POINT('Ctrl Pts',(64.3139205225789,-1.52119348141188,3.99927695466287));
#24511=CARTESIAN_POINT('Ctrl Pts',(64.8166220212948,-1.74791886892809,4.03632291818555));
#24512=CARTESIAN_POINT('Ctrl Pts',(65.4428269178191,-1.70080927101294,4.07336888170823));
#24513=CARTESIAN_POINT('Ctrl Pts',(65.9059489905043,-1.40142466222204,4.11041484523092));
#24514=CARTESIAN_POINT('Ctrl Pts',(66.368769480536,-1.10223501111091,4.14743668461735));
#24515=CARTESIAN_POINT('Ctrl Pts',(66.6687194749238,-0.551098802461342,
4.18445852400377));
#24516=CARTESIAN_POINT('Ctrl Pts',(66.6687523910643,6.71113220718263E-6,
4.22148036339021));
#24517=CARTESIAN_POINT('Ctrl Pts',(66.66584023827,-0.00152342185141638,
4.02851963660979));
#24518=CARTESIAN_POINT('Ctrl Pts',(66.6670688296308,-0.136474322284296,
4.01949512129795));
#24519=CARTESIAN_POINT('Ctrl Pts',(66.6520459458893,-0.271155172380326,
4.0104706059861));
#24520=CARTESIAN_POINT('Ctrl Pts',(66.6197204952158,-0.401546525825014,
4.00144609067426));
#24521=CARTESIAN_POINT('Ctrl Pts',(66.4870233447183,-0.936807773267794,
3.96440012715158));
#24522=CARTESIAN_POINT('Ctrl Pts',(66.0627550406069,-1.39978532477287,3.92735416362889));
#24523=CARTESIAN_POINT('Ctrl Pts',(65.5410843780201,-1.57859487864439,3.89030820010621));
#24524=CARTESIAN_POINT('Ctrl Pts',(65.0194137154332,-1.7574044325159,3.85326223658353));
#24525=CARTESIAN_POINT('Ctrl Pts',(64.400340694371,-1.65204598875385,3.81621627306085));
#24526=CARTESIAN_POINT('Ctrl Pts',(63.9671875933068,-1.310737436563,3.77917030953817));
#24527=CARTESIAN_POINT('Ctrl Pts',(63.5340344922426,-0.969428884372161,
3.74212434601549));
#24528=CARTESIAN_POINT('Ctrl Pts',(63.2868013111764,-0.392170223752528,
3.70507838249281));
#24529=CARTESIAN_POINT('Ctrl Pts',(63.3386357173299,0.156852845981076,3.66803241897013));
#24530=CARTESIAN_POINT('Ctrl Pts',(63.3904701234834,0.70587591571468,3.63098645544745));
#24531=CARTESIAN_POINT('Ctrl Pts',(63.7413721168566,1.22666339456225,3.59394049192477));
#24532=CARTESIAN_POINT('Ctrl Pts',(64.230749410433,1.48087393976488,3.55689452840209));
#24533=CARTESIAN_POINT('Ctrl Pts',(64.7201267040094,1.7350844849675,3.51984856487941));
#24534=CARTESIAN_POINT('Ctrl Pts',(65.347979297789,1.72271809652518,3.48280260135673));
#24535=CARTESIAN_POINT('Ctrl Pts',(65.826966892062,1.44943432222995,3.44575663783405));
#24536=CARTESIAN_POINT('Ctrl Pts',(66.305954486335,1.17615054793472,3.40871067431137));
#24537=CARTESIAN_POINT('Ctrl Pts',(66.6360770811014,0.641949387786594,3.37166471078869));
#24538=CARTESIAN_POINT('Ctrl Pts',(66.6662521989441,0.0913110318543479,
3.33461874726601));
#24539=CARTESIAN_POINT('Ctrl Pts',(66.6679081722746,0.0610926765551679,
3.3325857103806));
#24540=CARTESIAN_POINT('Ctrl Pts',(66.668660799992,0.0308248176933807,3.3305526734952));
#24541=CARTESIAN_POINT('Ctrl Pts',(66.6685304876972,0.000550348904958531,
3.32851963660979));
#24542=CARTESIAN_POINT('Origin',(65.,0.,3.));
#24543=CARTESIAN_POINT('',(66.664215437255,0.00117645755965692,2.62851963660979));
#24544=CARTESIAN_POINT('',(66.663709965026,-0.000842507685006553,2.82148036339021));
#24545=CARTESIAN_POINT('',(66.666,2.04026156737949E-16,3.));
#24546=CARTESIAN_POINT('Ctrl Pts',(66.663709965026,-0.000842507685006553,
2.82148036339021));
#24547=CARTESIAN_POINT('Ctrl Pts',(66.6621889226241,0.331295501917188,2.84361959192095));
#24548=CARTESIAN_POINT('Ctrl Pts',(66.565926135999,0.664245551393377,2.8657588204517));
#24549=CARTESIAN_POINT('Ctrl Pts',(66.3808853648239,0.936957985442183,2.88789804898245));
#24550=CARTESIAN_POINT('Ctrl Pts',(66.0712533625325,1.39329253521756,2.92494401250513));
#24551=CARTESIAN_POINT('Ctrl Pts',(65.5130436951299,1.68096223107998,2.96198997602781));
#24552=CARTESIAN_POINT('Ctrl Pts',(64.9617241821671,1.66831340551997,2.9990359395505));
#24553=CARTESIAN_POINT('Ctrl Pts',(64.4104046692042,1.65566457995996,3.03608190307317));
#24554=CARTESIAN_POINT('Ctrl Pts',(63.8659753106812,1.34269723297749,3.07312786659585));
#24555=CARTESIAN_POINT('Ctrl Pts',(63.5775972896502,0.872642645564547,3.11017383011853));
#24556=CARTESIAN_POINT('Ctrl Pts',(63.2892192686192,0.4025880581516,3.14721979364122));
#24557=CARTESIAN_POINT('Ctrl Pts',(63.2568925850803,-0.224553769691831,
3.1842657571639));
#24558=CARTESIAN_POINT('Ctrl Pts',(63.4954117290602,-0.721767824316922,
3.22131172068658));
#24559=CARTESIAN_POINT('Ctrl Pts',(63.73393087304,-1.21898187894202,3.25835768420926));
#24560=CARTESIAN_POINT('Ctrl Pts',(64.2432958445387,-1.58626816034877,3.29540364773194));
#24561=CARTESIAN_POINT('Ctrl Pts',(64.7903928760533,-1.65553601919701,3.33244961125462));
#24562=CARTESIAN_POINT('Ctrl Pts',(65.3374899075679,-1.72480387804526,3.3694955747773));
#24563=CARTESIAN_POINT('Ctrl Pts',(65.9223189990984,-1.49605331433501,3.40654153829998));
#24564=CARTESIAN_POINT('Ctrl Pts',(66.2772298007007,-1.07397332065116,3.44358750182266));
#24565=CARTESIAN_POINT('Ctrl Pts',(66.5259750107882,-0.778151451526181,
3.46955178901184));
#24566=CARTESIAN_POINT('Ctrl Pts',(66.6617810644663,-0.387363397948804,
3.49551607620103));
#24567=CARTESIAN_POINT('Ctrl Pts',(66.6649541686305,0.00142706439964306,
3.52148036339021));
#24568=CARTESIAN_POINT('Ctrl Pts',(66.6685304876972,0.000550348904958531,
3.32851963660979));
#24569=CARTESIAN_POINT('Ctrl Pts',(66.6662862515739,-0.520836037284763,
3.29350670997252));
#24570=CARTESIAN_POINT('Ctrl Pts',(66.4021649235169,-1.0441829058867,3.25849378333524));
#24571=CARTESIAN_POINT('Ctrl Pts',(65.9803979715476,-1.35039028151487,3.22348085669796));
#24572=CARTESIAN_POINT('Ctrl Pts',(65.5341409853895,-1.67437768723548,3.18643489317528));
#24573=CARTESIAN_POINT('Ctrl Pts',(64.9113993721543,-1.75527694696033,3.1493889296526));
#24574=CARTESIAN_POINT('Ctrl Pts',(64.3971743623243,-1.55606405574624,3.11234296612992));
#24575=CARTESIAN_POINT('Ctrl Pts',(63.8829493524943,-1.35685116453215,3.07529700260724));
#24576=CARTESIAN_POINT('Ctrl Pts',(63.4772409460695,-0.877526122379129,
3.03825103908456));
#24577=CARTESIAN_POINT('Ctrl Pts',(63.3657238957733,-0.337454752786397,
3.00120507556188));
#24578=CARTESIAN_POINT('Ctrl Pts',(63.2542068454771,0.202616616806336,2.9641591120392));
#24579=CARTESIAN_POINT('Ctrl Pts',(63.4368811513095,0.803434313838776,2.92711314851652));
#24580=CARTESIAN_POINT('Ctrl Pts',(63.8301448813726,1.190030712396,2.89006718499384));
#24581=CARTESIAN_POINT('Ctrl Pts',(64.2234086114356,1.57662711095322,2.85302122147116));
#24582=CARTESIAN_POINT('Ctrl Pts',(64.8272617657294,1.74900221103522,2.81597525794848));
#24583=CARTESIAN_POINT('Ctrl Pts',(65.3653475241109,1.62826757065616,2.7789292944258));
#24584=CARTESIAN_POINT('Ctrl Pts',(65.9034332824925,1.50753293027711,2.74188333090311));
#24585=CARTESIAN_POINT('Ctrl Pts',(66.3757516449619,1.093688549437,2.70483736738043));
#24586=CARTESIAN_POINT('Ctrl Pts',(66.5661434347078,0.576132655684555,2.66779140385775));
#24587=CARTESIAN_POINT('Ctrl Pts',(66.6334204184134,0.393248722101042,2.6547008147751));
#24588=CARTESIAN_POINT('Ctrl Pts',(66.6654949753924,0.197414973610974,2.64161022569244));
#24589=CARTESIAN_POINT('Ctrl Pts',(66.664215437255,0.00117645755965692,
2.62851963660979));
#24590=CARTESIAN_POINT('Origin',(65.,0.,3.));
#24591=CARTESIAN_POINT('',(66.6642789433678,-0.00120644035140824,1.92851963660979));
#24592=CARTESIAN_POINT('',(66.6680288432953,-0.000974731038369267,2.1214803633902));
#24593=CARTESIAN_POINT('',(66.666,2.04026156737949E-16,3.));
#24594=CARTESIAN_POINT('Ctrl Pts',(66.6680288432953,-0.000974731038369267,
2.1214803633902));
#24595=CARTESIAN_POINT('Ctrl Pts',(66.6645899038029,0.493760549303249,2.1546771441182));
#24596=CARTESIAN_POINT('Ctrl Pts',(66.4304593550116,0.991322629328269,2.1878739248462));
#24597=CARTESIAN_POINT('Ctrl Pts',(66.0452404987214,1.30084855271516,2.2210707055742));
#24598=CARTESIAN_POINT('Ctrl Pts',(65.6153553295749,1.64626415674821,2.25811666909688));
#24599=CARTESIAN_POINT('Ctrl Pts',(64.9973130191693,1.75750978249458,2.29516263261956));
#24600=CARTESIAN_POINT('Ctrl Pts',(64.4739641353999,1.58367323852582,2.33220859614224));
#24601=CARTESIAN_POINT('Ctrl Pts',(63.9506152516305,1.40983669455707,2.36925455966492));
#24602=CARTESIAN_POINT('Ctrl Pts',(63.5219597944974,0.950917980873213,2.40630052318761));
#24603=CARTESIAN_POINT('Ctrl Pts',(63.3841743645993,0.416943849037749,2.44334648671029));
#24604=CARTESIAN_POINT('Ctrl Pts',(63.2463889347012,-0.117030282797714,
2.48039245023297));
#24605=CARTESIAN_POINT('Ctrl Pts',(63.399473532038,-0.72605983278478,2.51743841375565));
#24606=CARTESIAN_POINT('Ctrl Pts',(63.77336812259,-1.13141897393943,2.55448437727833));
#24607=CARTESIAN_POINT('Ctrl Pts',(64.1472627131419,-1.53677811509408,2.59153034080101));
#24608=CARTESIAN_POINT('Ctrl Pts',(64.741967296909,-1.73846684741632,2.62857630432369));
#24609=CARTESIAN_POINT('Ctrl Pts',(65.2853119489257,-1.64418117890598,2.66562226784637));
#24610=CARTESIAN_POINT('Ctrl Pts',(65.8286566009425,-1.54989551039565,2.70266823136905));
#24611=CARTESIAN_POINT('Ctrl Pts',(66.3206413212089,-1.15963544105274,2.73971419489173));
#24612=CARTESIAN_POINT('Ctrl Pts',(66.5361065127521,-0.652005704537125,
2.77676015841441));
#24613=CARTESIAN_POINT('Ctrl Pts',(66.6228064445369,-0.447743182072849,
2.79166689340634));
#24614=CARTESIAN_POINT('Ctrl Pts',(66.664734109836,-0.22447691676168,2.80657362839827));
#24615=CARTESIAN_POINT('Ctrl Pts',(66.663709965026,-0.000842507685006553,
2.82148036339021));
#24616=CARTESIAN_POINT('Ctrl Pts',(66.664215437255,0.00117645755965692,
2.62851963660979));
#24617=CARTESIAN_POINT('Ctrl Pts',(66.6618739219115,-0.357933976805237,
2.60456426216976));
#24618=CARTESIAN_POINT('Ctrl Pts',(66.5478366409886,-0.718399891583488,
2.58060888772974));
#24619=CARTESIAN_POINT('Ctrl Pts',(66.3334304982421,-1.00334301282382,2.55665351328971));
#24620=CARTESIAN_POINT('Ctrl Pts',(66.0018605550081,-1.443995380915,2.51960754976703));
#24621=CARTESIAN_POINT('Ctrl Pts',(65.4302554515179,-1.70403271043258,2.48256158624435));
#24622=CARTESIAN_POINT('Ctrl Pts',(64.880213504605,-1.66444744301089,2.44551562272167));
#24623=CARTESIAN_POINT('Ctrl Pts',(64.3301715576922,-1.6248621755892,2.40846965919899));
#24624=CARTESIAN_POINT('Ctrl Pts',(63.8016927673567,-1.28565431122825,2.37142369567631));
#24625=CARTESIAN_POINT('Ctrl Pts',(63.5366384486743,-0.802064252492239,
2.33437773215363));
#24626=CARTESIAN_POINT('Ctrl Pts',(63.2715841299918,-0.318474193756233,
2.29733176863095));
#24627=CARTESIAN_POINT('Ctrl Pts',(63.2699542829623,0.309498059354825,2.26028580510827));
#24628=CARTESIAN_POINT('Ctrl Pts',(63.5324948163207,0.794457444359823,2.22323984158559));
#24629=CARTESIAN_POINT('Ctrl Pts',(63.795035349679,1.27941682936482,2.18619387806291));
#24630=CARTESIAN_POINT('Ctrl Pts',(64.3217462634253,1.62136334626376,2.14914791454023));
#24631=CARTESIAN_POINT('Ctrl Pts',(64.8715753212295,1.66380323262916,2.11210195101754));
#24632=CARTESIAN_POINT('Ctrl Pts',(65.4214043790337,1.70624311899456,2.07505598749486));
#24633=CARTESIAN_POINT('Ctrl Pts',(65.9943515808958,1.44917637482642,2.03801002397218));
#24634=CARTESIAN_POINT('Ctrl Pts',(66.3282043910519,1.01025105326097,2.0009640604495));
#24635=CARTESIAN_POINT('Ctrl Pts',(66.54582391177,0.724140781894946,1.9768159191696));
#24636=CARTESIAN_POINT('Ctrl Pts',(66.6618524838225,0.360758997512877,1.95266777788969));
#24637=CARTESIAN_POINT('Ctrl Pts',(66.6642789433678,-0.00120644035140824,
1.92851963660979));
#24638=CARTESIAN_POINT('Origin',(65.,0.,3.));
#24639=CARTESIAN_POINT('',(66.6685688018723,-0.000500570493866259,1.22851963660979));
#24640=CARTESIAN_POINT('',(66.6666630352664,0.00145874010108481,1.4214803633902));
#24641=CARTESIAN_POINT('',(66.666,2.04026156737949E-16,3.));
#24642=CARTESIAN_POINT('Ctrl Pts',(66.6666630352664,0.00145874010108481,
1.4214803633902));
#24643=CARTESIAN_POINT('Ctrl Pts',(66.6676496745696,0.109114984958744,1.42868873279277));
#24644=CARTESIAN_POINT('Ctrl Pts',(66.6581116875295,0.216597146837641,1.43589710219534));
#24645=CARTESIAN_POINT('Ctrl Pts',(66.6374139306422,0.321885502945882,1.44310547159791));
#24646=CARTESIAN_POINT('Ctrl Pts',(66.5310419755125,0.862993814953162,1.48015143512059));
#24647=CARTESIAN_POINT('Ctrl Pts',(66.1299138139174,1.34615847081564,1.51719739864327));
#24648=CARTESIAN_POINT('Ctrl Pts',(65.6176080235618,1.55025642604728,1.55424336216595));
#24649=CARTESIAN_POINT('Ctrl Pts',(65.1053022332063,1.75435438127892,1.59128932568863));
#24650=CARTESIAN_POINT('Ctrl Pts',(64.4818188140901,1.67938563587972,1.62833528921131));
#24651=CARTESIAN_POINT('Ctrl Pts',(64.0324984883637,1.35966006128365,1.66538125273399));
#24652=CARTESIAN_POINT('Ctrl Pts',(63.5831781626372,1.03993448668758,1.70242721625667));
#24653=CARTESIAN_POINT('Ctrl Pts',(63.3080209303004,0.475452082894629,1.73947317977936));
#24654=CARTESIAN_POINT('Ctrl Pts',(63.3329540589798,-0.0754485771665831,
1.77651914330204));
#24655=CARTESIAN_POINT('Ctrl Pts',(63.3578871876591,-0.626349237227795,
1.81356510682472));
#24656=CARTESIAN_POINT('Ctrl Pts',(63.6829106773545,-1.16366815355727,1.8506110703474));
#24657=CARTESIAN_POINT('Ctrl Pts',(64.1592756849985,-1.44149827729127,1.88765703387008));
#24658=CARTESIAN_POINT('Ctrl Pts',(64.6356406926424,-1.71932840102526,1.92470299739276));
#24659=CARTESIAN_POINT('Ctrl Pts',(65.2633472182348,-1.73766973216377,1.96174896091544));
#24660=CARTESIAN_POINT('Ctrl Pts',(65.7551218110002,-1.48812825650888,1.99879492443812));
#24661=CARTESIAN_POINT('Ctrl Pts',(66.2468964037657,-1.23858678085398,2.0358408879608));
#24662=CARTESIAN_POINT('Ctrl Pts',(66.6027390637042,-0.72116249840569,2.07288685148348));
#24663=CARTESIAN_POINT('Ctrl Pts',(66.6597963797297,-0.172657566021668,
2.10993281500616));
#24664=CARTESIAN_POINT('Ctrl Pts',(66.6657247999481,-0.115666316563739,
2.11378199780084));
#24665=CARTESIAN_POINT('Ctrl Pts',(66.6684275899941,-0.058339526276079,
2.11763118059552));
#24666=CARTESIAN_POINT('Ctrl Pts',(66.6680288432953,-0.000974731038369267,
2.1214803633902));
#24667=CARTESIAN_POINT('Ctrl Pts',(66.6642789433678,-0.00120644035140824,
1.92851963660979));
#24668=CARTESIAN_POINT('Ctrl Pts',(66.6655749455541,-0.194536677303716,
1.91562181436701));
#24669=CARTESIAN_POINT('Ctrl Pts',(66.634462982395,-0.387462864473387,1.90272399212424));
#24670=CARTESIAN_POINT('Ctrl Pts',(66.5691129188822,-0.567995372183044,
1.88982616988146));
#24671=CARTESIAN_POINT('Ctrl Pts',(66.3814102181061,-1.08653257709889,1.85278020635878));
#24672=CARTESIAN_POINT('Ctrl Pts',(65.9112463981035,-1.50282308796781,1.8157342428361));
#24673=CARTESIAN_POINT('Ctrl Pts',(65.3737945971089,-1.62634919196251,1.77868827931342));
#24674=CARTESIAN_POINT('Ctrl Pts',(64.8363427961142,-1.74987529595721,1.74164231579074));
#24675=CARTESIAN_POINT('Ctrl Pts',(64.2316030141275,-1.58063699307767,1.70459635226806));
#24676=CARTESIAN_POINT('Ctrl Pts',(63.8363378414827,-1.19608715228398,1.66755038874538));
#24677=CARTESIAN_POINT('Ctrl Pts',(63.4410726688379,-0.811537311490284,
1.6305044252227));
#24678=CARTESIAN_POINT('Ctrl Pts',(63.2552821055351,-0.211675932782416,
1.59345846170002));
#24679=CARTESIAN_POINT('Ctrl Pts',(63.3639942563739,0.328967022430173,1.55641249817734));
#24680=CARTESIAN_POINT('Ctrl Pts',(63.4727064072127,0.869609977642756,1.51936653465465));
#24681=CARTESIAN_POINT('Ctrl Pts',(63.8759212721932,1.35103450936006,1.48232057113197));
#24682=CARTESIAN_POINT('Ctrl Pts',(64.3891052819731,1.55291395077579,1.44527460760929));
#24683=CARTESIAN_POINT('Ctrl Pts',(64.9022892917531,1.75479339219152,1.40822864408661));
#24684=CARTESIAN_POINT('Ctrl Pts',(65.5254424463325,1.67712774330567,1.37118268056393));
#24685=CARTESIAN_POINT('Ctrl Pts',(65.9733751709996,1.35546112873118,1.33413671704125));
#24686=CARTESIAN_POINT('Ctrl Pts',(66.3990566948007,1.04977340575941,1.2989310235641));
#24687=CARTESIAN_POINT('Ctrl Pts',(66.6664936696292,0.523724262697509,1.26372533008694));
#24688=CARTESIAN_POINT('Ctrl Pts',(66.6685688018723,-0.000500570493866259,
1.22851963660979));
#24689=CARTESIAN_POINT('Origin',(65.,0.,3.));
#24690=CARTESIAN_POINT('',(66.6657538157597,0.00152189319961124,0.528519636609788));
#24691=CARTESIAN_POINT('',(66.6632893889008,6.33249066023143E-5,0.721480363390204));
#24692=CARTESIAN_POINT('',(66.666,2.04026156737949E-16,3.));
#24693=CARTESIAN_POINT('Ctrl Pts',(66.6632893889008,6.33249066023143E-5,
0.721480363390204));
#24694=CARTESIAN_POINT('Ctrl Pts',(66.663382354964,0.274266208525867,0.739746284990023));
#24695=CARTESIAN_POINT('Ctrl Pts',(66.5993416986523,0.548428211919456,0.758012206589841));
#24696=CARTESIAN_POINT('Ctrl Pts',(66.4709289590166,0.78810066283112,0.77627812818966));
#24697=CARTESIAN_POINT('Ctrl Pts',(66.2104891206872,1.27419148640901,0.81332409171234));
#24698=CARTESIAN_POINT('Ctrl Pts',(65.6852625770594,1.61841374682523,0.850370055235021));
#24699=CARTESIAN_POINT('Ctrl Pts',(65.1356222340335,1.66323217468977,0.887416018757702));
#24700=CARTESIAN_POINT('Ctrl Pts',(64.5859818910076,1.70805060255431,0.924461982280382));
#24701=CARTESIAN_POINT('Ctrl Pts',(64.0119277485837,1.45346519786717,0.961507945803063));
#24702=CARTESIAN_POINT('Ctrl Pts',(63.6761789401645,1.01598841469989,0.998553909325744));
#24703=CARTESIAN_POINT('Ctrl Pts',(63.3404301317454,0.578511631532615,1.03559987284842));
#24704=CARTESIAN_POINT('Ctrl Pts',(63.242986657331,-0.0418565301147992,
1.0726458363711));
#24705=CARTESIAN_POINT('Ctrl Pts',(63.4284440755221,-0.561201063347335,
1.10969179989379));
#24706=CARTESIAN_POINT('Ctrl Pts',(63.6139014937132,-1.08054559657987,1.14673776341647));
#24707=CARTESIAN_POINT('Ctrl Pts',(64.0822598045097,-1.49886650139754,1.18378372693915));
#24708=CARTESIAN_POINT('Ctrl Pts',(64.619172171207,-1.62471684366476,1.22082969046183));
#24709=CARTESIAN_POINT('Ctrl Pts',(65.1560845379043,-1.75056718593198,1.25787565398451));
#24710=CARTESIAN_POINT('Ctrl Pts',(65.7615509605024,-1.58394696564878,1.29492161750719));
#24711=CARTESIAN_POINT('Ctrl Pts',(66.1584762974693,-1.20111087143113,1.33196758102987));
#24712=CARTESIAN_POINT('Ctrl Pts',(66.4781682685839,-0.892766671210736,
1.36180517514998));
#24713=CARTESIAN_POINT('Ctrl Pts',(66.6625790404782,-0.444162614627704,
1.39164276927009));
#24714=CARTESIAN_POINT('Ctrl Pts',(66.6666630352664,0.00145874010108481,
1.4214803633902));
#24715=CARTESIAN_POINT('Ctrl Pts',(66.6685688018723,-0.000500570493866259,
1.22851963660979));
#24716=CARTESIAN_POINT('Ctrl Pts',(66.6686772730691,-0.0279028217311245,
1.22667936656426));
#24717=CARTESIAN_POINT('Ctrl Pts',(66.6680606812028,-0.0553000883040847,
1.22483909651874));
#24718=CARTESIAN_POINT('Ctrl Pts',(66.6667037271851,-0.0826606364095831,
1.22299882647321));
#24719=CARTESIAN_POINT('Ctrl Pts',(66.6393872639487,-0.633448206712713,
1.18595286295053));
#24720=CARTESIAN_POINT('Ctrl Pts',(66.3120420427213,-1.16935576705583,1.14890689942785));
#24721=CARTESIAN_POINT('Ctrl Pts',(65.8344794601719,-1.4451221836215,1.11186093590517));
#24722=CARTESIAN_POINT('Ctrl Pts',(65.3569168776225,-1.72088860018717,1.07481497238249));
#24723=CARTESIAN_POINT('Ctrl Pts',(64.729136933751,-1.73651387297538,1.03776900885981));
#24724=CARTESIAN_POINT('Ctrl Pts',(64.2384466796233,-1.48484700734034,1.00072304533713));
#24725=CARTESIAN_POINT('Ctrl Pts',(63.7477564254956,-1.2331801417053,0.963677081814447));
#24726=CARTESIAN_POINT('Ctrl Pts',(63.3941558611116,-0.714221137647012,
0.926631118291766));
#24727=CARTESIAN_POINT('Ctrl Pts',(63.3394722898162,-0.165474525977688,
0.889585154769085));
#24728=CARTESIAN_POINT('Ctrl Pts',(63.2847887185207,0.383272085691634,0.852539191246405));
#24729=CARTESIAN_POINT('Ctrl Pts',(63.5290221403138,0.961806304971985,0.815493227723724));
#24730=CARTESIAN_POINT('Ctrl Pts',(63.9603977448083,1.30535866571472,0.778447264201044));
#24731=CARTESIAN_POINT('Ctrl Pts',(64.3917733493027,1.64891102645746,0.741401300678363));
#24732=CARTESIAN_POINT('Ctrl Pts',(65.0102911364986,1.75748152866258,0.704355337155683));
#24733=CARTESIAN_POINT('Ctrl Pts',(65.5328829338629,1.58138226671976,0.667309373633002));
#24734=CARTESIAN_POINT('Ctrl Pts',(66.0554747312272,1.40528300477694,0.630263410110321));
#24735=CARTESIAN_POINT('Ctrl Pts',(66.4821405387599,0.944513978686174,0.593217446587641));
#24736=CARTESIAN_POINT('Ctrl Pts',(66.6176143302611,0.409948745265365,0.55617148306496));
#24737=CARTESIAN_POINT('Ctrl Pts',(66.6513211107492,0.276945359297953,0.546954200913236));
#24738=CARTESIAN_POINT('Ctrl Pts',(66.6670017222694,0.13937363756141,0.537736918761512));
#24739=CARTESIAN_POINT('Ctrl Pts',(66.6657538157597,0.00152189319961124,
0.528519636609788));
#24740=CARTESIAN_POINT('Origin',(65.,0.,3.));
#24741=CARTESIAN_POINT('',(66.6633878829795,-0.000426123154284863,-0.171480363390211));
#24742=CARTESIAN_POINT('',(66.6664305869533,-0.00149161834301985,0.0214803633902055));
#24743=CARTESIAN_POINT('',(66.666,2.04026156737949E-16,3.));
#24744=CARTESIAN_POINT('Ctrl Pts',(66.6664305869533,-0.00149161834301985,
0.0214803633902055));
#24745=CARTESIAN_POINT('Ctrl Pts',(66.6623874613811,0.436608579267598,0.0508038371872736));
#24746=CARTESIAN_POINT('Ctrl Pts',(66.484951449296,0.877606426402575,0.0801273109843417));
#24747=CARTESIAN_POINT('Ctrl Pts',(66.1749931684956,1.18495810418996,0.10945078478141));
#24748=CARTESIAN_POINT('Ctrl Pts',(65.7834057582335,1.57325244894404,0.146496748304091));
#24749=CARTESIAN_POINT('Ctrl Pts',(65.1803040079573,1.74823863365067,0.183542711826771));
#24750=CARTESIAN_POINT('Ctrl Pts',(64.641700851863,1.62983323643182,0.220588675349452));
#24751=CARTESIAN_POINT('Ctrl Pts',(64.1030976957686,1.51142783921297,0.257634638872132));
#24752=CARTESIAN_POINT('Ctrl Pts',(63.6289931338561,1.09963086006864,0.294680602394813));
#24753=CARTESIAN_POINT('Ctrl Pts',(63.4363638080708,0.582903522671605,0.331726565917493));
#24754=CARTESIAN_POINT('Ctrl Pts',(63.2437344822855,0.0661761852745729,
0.368772529440174));
#24755=CARTESIAN_POINT('Ctrl Pts',(63.3325803926274,-0.555481510375157,
0.405818492962855));
#24756=CARTESIAN_POINT('Ctrl Pts',(63.6622407040169,-0.997564395392433,
0.442864456485535));
#24757=CARTESIAN_POINT('Ctrl Pts',(63.9919010154063,-1.43964728040971,0.479910420008216));
#24758=CARTESIAN_POINT('Ctrl Pts',(64.5623757278433,-1.70215535479453,0.516956383530896));
#24759=CARTESIAN_POINT('Ctrl Pts',(65.1125838545831,-1.6649503094947,0.554002347053577));
#24760=CARTESIAN_POINT('Ctrl Pts',(65.6627919813228,-1.62774526419487,0.591048310576258));
#24761=CARTESIAN_POINT('Ctrl Pts',(66.1927335223652,-1.29082709921038,0.628094274098938));
#24762=CARTESIAN_POINT('Ctrl Pts',(66.4598777263709,-0.808388323348352,
0.665140237621619));
#24763=CARTESIAN_POINT('Ctrl Pts',(66.5953035291742,-0.563821315923748,
0.683920279544481));
#24764=CARTESIAN_POINT('Ctrl Pts',(66.6631938061757,-0.281857388570597,
0.702700321467342));
#24765=CARTESIAN_POINT('Ctrl Pts',(66.6632893889008,6.33249066023143E-5,
0.721480363390204));
#24766=CARTESIAN_POINT('Ctrl Pts',(66.6657538157597,0.00152189319961124,
0.528519636609788));
#24767=CARTESIAN_POINT('Ctrl Pts',(66.6619861549602,-0.414678045906902,
0.500690955238832));
#24768=CARTESIAN_POINT('Ctrl Pts',(66.5039069443419,-0.833430525360481,
0.472862273867875));
#24769=CARTESIAN_POINT('Ctrl Pts',(66.2217249851539,-1.13671551258266,0.445033592496918));
#24770=CARTESIAN_POINT('Ctrl Pts',(65.8460800730759,-1.54045309625902,0.407987628974238));
#24771=CARTESIAN_POINT('Ctrl Pts',(65.2505084734505,-1.73956682286089,0.370941665451557));
#24772=CARTESIAN_POINT('Ctrl Pts',(64.7075769058774,-1.64293116911907,0.333895701928877));
#24773=CARTESIAN_POINT('Ctrl Pts',(64.1646453383043,-1.54629551537724,0.296849738406196));
#24774=CARTESIAN_POINT('Ctrl Pts',(63.6743538027836,-1.15391048129172,0.259803774883516));
#24775=CARTESIAN_POINT('Ctrl Pts',(63.4610870008646,-0.645353297241682,
0.222757811360835));
#24776=CARTESIAN_POINT('Ctrl Pts',(63.2478201989456,-0.136796113191638,
0.185711847838155));
#24777=CARTESIAN_POINT('Ctrl Pts',(63.3115781306282,0.48793322082293,0.148665884315474));
#24778=CARTESIAN_POINT('Ctrl Pts',(63.6231816165986,0.942923771900633,0.111619920792793));
#24779=CARTESIAN_POINT('Ctrl Pts',(63.9347851025691,1.39791432297834,0.0745739572701125));
#24780=CARTESIAN_POINT('Ctrl Pts',(64.4942341428273,1.68316609111917,0.0375279937474321));
#24781=CARTESIAN_POINT('Ctrl Pts',(65.0454937124919,1.6681320083057,0.000482030224751638));
#24782=CARTESIAN_POINT('Ctrl Pts',(65.5967532821565,1.65309792549222,-0.0365639332979289));
#24783=CARTESIAN_POINT('Ctrl Pts',(66.1398233812275,1.33777799172443,-0.0736098968206095));
#24784=CARTESIAN_POINT('Ctrl Pts',(66.4261648980985,0.866480120962494,-0.11065586034329));
#24785=CARTESIAN_POINT('Ctrl Pts',(66.5828763524582,0.608544158441986,-0.130930694692264));
#24786=CARTESIAN_POINT('Ctrl Pts',(66.6626912202299,0.303888929858147,-0.151205529041237));
#24787=CARTESIAN_POINT('Ctrl Pts',(66.6633878829795,-0.000426123154284863,
-0.171480363390211));
#24788=CARTESIAN_POINT('Origin',(65.,0.,3.));
#24789=CARTESIAN_POINT('',(66.6673159824367,-0.00130059074131283,-0.871480363390211));
#24790=CARTESIAN_POINT('',(66.6681941903091,0.000864019930038266,-0.678519636609795));
#24791=CARTESIAN_POINT('',(66.666,2.04026156737949E-16,3.));
#24792=CARTESIAN_POINT('Ctrl Pts',(66.6681941903091,0.000864019930038266,
-0.678519636609795));
#24793=CARTESIAN_POINT('Ctrl Pts',(66.6685078326159,0.0505538571114843,
-0.675184574138157));
#24794=CARTESIAN_POINT('Ctrl Pts',(66.6664801000417,0.100217739688425,-0.67184951166652));
#24795=CARTESIAN_POINT('Ctrl Pts',(66.6620276056557,0.149663274321063,-0.668514449194882));
#24796=CARTESIAN_POINT('Ctrl Pts',(66.6125691784105,0.698905601245373,-0.631468485672201));
#24797=CARTESIAN_POINT('Ctrl Pts',(66.2639236084022,1.22120635507833,-0.594422522149521));
#24798=CARTESIAN_POINT('Ctrl Pts',(65.7756507075141,1.47753189011202,-0.557376558626841));
#24799=CARTESIAN_POINT('Ctrl Pts',(65.287377806626,1.7338574251457,-0.52033059510416));
#24800=CARTESIAN_POINT('Ctrl Pts',(64.659477574858,1.7242077413801,-0.483284631581479));
#24801=CARTESIAN_POINT('Ctrl Pts',(64.1793120174543,1.4529989415171,-0.446238668058799));
#24802=CARTESIAN_POINT('Ctrl Pts',(63.6991464600505,1.18179014165409,-0.409192704536118));
#24803=CARTESIAN_POINT('Ctrl Pts',(63.3667155770108,0.649022225693674,-0.372146741013438));
#24804=CARTESIAN_POINT('Ctrl Pts',(63.334158295787,0.0985195171959843,-0.335100777490757));
#24805=CARTESIAN_POINT('Ctrl Pts',(63.3016010145631,-0.451983191301702,
-0.298054813968077));
#24806=CARTESIAN_POINT('Ctrl Pts',(63.568917335155,-1.02022069233666,-0.261008850445396));
#24807=CARTESIAN_POINT('Ctrl Pts',(64.0137684029003,-1.34613590481465,-0.223962886922715));
#24808=CARTESIAN_POINT('Ctrl Pts',(64.4586194706456,-1.67205111729263,-0.186916923400034));
#24809=CARTESIAN_POINT('Ctrl Pts',(65.0810052855443,-1.75564404121364,-0.149870959877354));
#24810=CARTESIAN_POINT('Ctrl Pts',(65.5960874627955,-1.5586578840129,-0.112824996354674));
#24811=CARTESIAN_POINT('Ctrl Pts',(66.1111696400466,-1.36167172681217,-0.0757790328319931));
#24812=CARTESIAN_POINT('Ctrl Pts',(66.5189481796502,-0.884106488489677,
-0.0387330693093125));
#24813=CARTESIAN_POINT('Ctrl Pts',(66.632800914328,-0.344522616927666,-0.00168710578663189));
#24814=CARTESIAN_POINT('Ctrl Pts',(66.6565343117127,-0.232042591898955,
0.00603538393898058));
#24815=CARTESIAN_POINT('Ctrl Pts',(66.6674953651548,-0.116867589766127,
0.013757873664593));
#24816=CARTESIAN_POINT('Ctrl Pts',(66.6664305869533,-0.00149161834301985,
0.0214803633902055));
#24817=CARTESIAN_POINT('Ctrl Pts',(66.6633878829795,-0.000426123154284863,
-0.171480363390211));
#24818=CARTESIAN_POINT('Ctrl Pts',(66.6639641550595,-0.252152325979383,
-0.188251492563918));
#24819=CARTESIAN_POINT('Ctrl Pts',(66.6104043971,-0.50364576625701,-0.205022621737625));
#24820=CARTESIAN_POINT('Ctrl Pts',(66.5014511773033,-0.728270889754927,
-0.221793750911332));
#24821=CARTESIAN_POINT('Ctrl Pts',(66.2607830049661,-1.22444822195432,-0.258839714434013));
#24822=CARTESIAN_POINT('Ctrl Pts',(65.7498337256207,-1.58952707859704,-0.295885677956694));
#24823=CARTESIAN_POINT('Ctrl Pts',(65.2024421689935,-1.65642721292161,-0.332931641479375));
#24824=CARTESIAN_POINT('Ctrl Pts',(64.6550506123664,-1.72332734724617,-0.369977605002055));
#24825=CARTESIAN_POINT('Ctrl Pts',(64.0712167784575,-1.49204875925259,-0.407023568524736));
#24826=CARTESIAN_POINT('Ctrl Pts',(63.7181355422591,-1.06843708657372,-0.444069532047416));
#24827=CARTESIAN_POINT('Ctrl Pts',(63.3650543060608,-0.644825413894849,
-0.481115495570097));
#24828=CARTESIAN_POINT('Ctrl Pts',(63.242725667573,-0.028880656530687,-0.518161459092778));
#24829=CARTESIAN_POINT('Ctrl Pts',(63.4071340014642,0.497505944605294,-0.555207422615458));
#24830=CARTESIAN_POINT('Ctrl Pts',(63.5715423353554,1.02389254574128,-0.592253386138139));
#24831=CARTESIAN_POINT('Ctrl Pts',(64.0226876416257,1.46072099064907,-0.629299349660819));
#24832=CARTESIAN_POINT('Ctrl Pts',(64.5541007528815,1.60807550663331,-0.6663453131835));
#24833=CARTESIAN_POINT('Ctrl Pts',(65.0855138641373,1.75543002261754,-0.70339127670618));
#24834=CARTESIAN_POINT('Ctrl Pts',(65.6971947803788,1.61331060967821,-0.740437240228861));
#24835=CARTESIAN_POINT('Ctrl Pts',(66.1092041825925,1.24675657433954,-0.777483203751541));
#24836=CARTESIAN_POINT('Ctrl Pts',(66.4576696191289,0.936735950411711,-0.808815590297765));
#24837=CARTESIAN_POINT('Ctrl Pts',(66.6633044515624,0.466170980160881,-0.840147976843988));
#24838=CARTESIAN_POINT('Ctrl Pts',(66.6673159824367,-0.00130059074131283,
-0.871480363390211));
#24839=CARTESIAN_POINT('Origin',(65.,0.,3.));
#24840=CARTESIAN_POINT('',(66.6674675207825,0.00121113675536799,-1.57148036339021));
#24841=CARTESIAN_POINT('',(66.6638321395092,0.000941642735149761,-1.3785196366098));
#24842=CARTESIAN_POINT('',(66.666,2.04026156737949E-16,3.));
#24843=CARTESIAN_POINT('',(63.7309291201476,1.0793586530485,-2.));
#24844=CARTESIAN_POINT('Ctrl Pts',(66.6674675207825,0.00121113675536799,
-1.57148036339021));
#24845=CARTESIAN_POINT('Ctrl Pts',(66.6635269376583,-0.471550204230264,
-1.6031823516921));
#24846=CARTESIAN_POINT('Ctrl Pts',(66.452430524463,-0.947291842680174,-1.63488433999399));
#24847=CARTESIAN_POINT('Ctrl Pts',(66.0967466510819,-1.25757678610753,-1.66658632829587));
#24848=CARTESIAN_POINT('Ctrl Pts',(65.6811054719418,-1.62016617912558,-1.70363229181856));
#24849=CARTESIAN_POINT('Ctrl Pts',(65.0680223500032,-1.75681556827131,-1.74067825534124));
#24850=CARTESIAN_POINT('Ctrl Pts',(64.5381019768621,-1.60385217794778,-1.77772421886392));
#24851=CARTESIAN_POINT('Ctrl Pts',(64.008181603721,-1.45088878762425,-1.8147701823866));
#24852=CARTESIAN_POINT('Ctrl Pts',(63.5614239793774,-1.00831261783145,-1.85181614590928));
#24853=CARTESIAN_POINT('Ctrl Pts',(63.4023827506955,-0.481249822665511,
-1.88886210943196));
#24854=CARTESIAN_POINT('Ctrl Pts',(63.2433415220136,0.0458129725004276,
-1.92590807295464));
#24855=CARTESIAN_POINT('Ctrl Pts',(63.3720166889934,0.657362393039508,-1.96295403647732));
#24856=CARTESIAN_POINT('Ctrl Pts',(63.7309291201476,1.07935865304851,-2.));
#24857=CARTESIAN_POINT('',(66.2714644419457,1.08121564890977,-2.));
#24858=CARTESIAN_POINT('Origin',(65.,0.,-2.));
#24859=CARTESIAN_POINT('Ctrl Pts',(66.2714656498818,1.0812165860621,-2.));
#24860=CARTESIAN_POINT('Ctrl Pts',(65.9206041791687,1.49275399655515,-1.96367708181445));
#24861=CARTESIAN_POINT('Ctrl Pts',(65.3506354631191,1.71875942899393,-1.92735416362889));
#24862=CARTESIAN_POINT('Ctrl Pts',(64.8132380266977,1.65815373977101,-1.89103124544334));
#24863=CARTESIAN_POINT('Ctrl Pts',(64.2651431372632,1.59634163148308,-1.85398528192066));
#24864=CARTESIAN_POINT('Ctrl Pts',(63.7509291640017,1.23639424886419,-1.81693931839798));
#24865=CARTESIAN_POINT('Ctrl Pts',(63.5055956276972,0.74259208529255,-1.7798933548753));
#24866=CARTESIAN_POINT('Ctrl Pts',(63.2602620913927,0.248789921720905,-1.74284739135262));
#24867=CARTESIAN_POINT('Ctrl Pts',(63.2838089920452,-0.378867022803494,
-1.70580142782994));
#24868=CARTESIAN_POINT('Ctrl Pts',(63.5656287203753,-0.852900276652179,
-1.66875546430726));
#24869=CARTESIAN_POINT('Ctrl Pts',(63.8474484487053,-1.32693353050086,-1.63170950078458));
#24870=CARTESIAN_POINT('Ctrl Pts',(64.387541004713,-1.64734309367383,-1.5946635372619));
#24871=CARTESIAN_POINT('Ctrl Pts',(64.9386444101885,-1.66760708582442,-1.55761757373922));
#24872=CARTESIAN_POINT('Ctrl Pts',(65.4897478156641,-1.68787107797502,-1.52057161021654));
#24873=CARTESIAN_POINT('Ctrl Pts',(66.0518620706076,-1.40798949910323,-1.48352564669385));
#24874=CARTESIAN_POINT('Ctrl Pts',(66.3677757854406,-0.955993240532984,
-1.44647968317117));
#24875=CARTESIAN_POINT('Ctrl Pts',(66.5609548232979,-0.679600674316361,
-1.42382633431738));
#24876=CARTESIAN_POINT('Ctrl Pts',(66.6620736349107,-0.338850343710036,
-1.40117298546359));
#24877=CARTESIAN_POINT('Ctrl Pts',(66.6638321395092,0.000941642735149761,
-1.3785196366098));
#24878=CARTESIAN_POINT('Origin',(65.,0.,-3.54592528053767));
#24879=CARTESIAN_POINT('',(67.0572086816557,0.00119446450309507,6.54592528053768));
#24880=CARTESIAN_POINT('',(67.0515888779951,-0.000804696401304116,6.60407471946233));
#24881=CARTESIAN_POINT('',(67.05475,1.03216492799367E-13,-3.54592528053767));
#24882=CARTESIAN_POINT('',(63.1173724903363,-0.82323218010314,7.));
#24883=CARTESIAN_POINT('Ctrl Pts',(67.0515888779951,-0.000804696401304414,
6.60407471946233));
#24884=CARTESIAN_POINT('Ctrl Pts',(67.0504040800969,0.384787351067748,6.62491192240684));
#24885=CARTESIAN_POINT('Ctrl Pts',(66.7605424545076,1.45760454425864,6.68279508887404));
#24886=CARTESIAN_POINT('Ctrl Pts',(65.029841359516,2.42994159679627,6.77772421886392));
#24887=CARTESIAN_POINT('Ctrl Pts',(62.9747815436376,1.33872801408516,6.88886210943195));
#24888=CARTESIAN_POINT('Ctrl Pts',(62.8436282049399,-0.197213743559581,
6.96295403647732));
#24889=CARTESIAN_POINT('Ctrl Pts',(63.1173724903363,-0.82323218010314,7.));
#24890=CARTESIAN_POINT('',(63.7764000215903,-1.65534094402445,7.));
#24891=CARTESIAN_POINT('Origin',(65.,0.,7.));
#24892=CARTESIAN_POINT('Ctrl Pts',(67.0572086816557,0.00119446450309495,
6.54592528053768));
#24893=CARTESIAN_POINT('Ctrl Pts',(67.0577114364342,0.0728343130723821,
6.54982271160486));
#24894=CARTESIAN_POINT('Ctrl Pts',(67.0218209037147,0.824923083408356,6.59076610619472));
#24895=CARTESIAN_POINT('Ctrl Pts',(66.0963109962835,2.16731896239629,6.66875546430726));
#24896=CARTESIAN_POINT('Ctrl Pts',(63.7734206371606,2.09605634078856,6.77989335487529));
#24897=CARTESIAN_POINT('Ctrl Pts',(62.5820931272045,0.120092092488812,6.89030820010622));
#24898=CARTESIAN_POINT('Ctrl Pts',(63.2405356955179,-1.25818726815371,6.96367708181445));
#24899=CARTESIAN_POINT('Ctrl Pts',(63.7763989699203,-1.65534250909262,7.));
#24900=CARTESIAN_POINT('Origin',(65.,0.,-3.54592528053767));
#24901=CARTESIAN_POINT('',(67.0519117333221,0.00102649957301762,5.84592528053768));
#24902=CARTESIAN_POINT('',(67.0566574869574,-0.00149765431883365,5.90407471946233));
#24903=CARTESIAN_POINT('',(67.05475,1.03216492799367E-13,-3.54592528053767));
#24904=CARTESIAN_POINT('Ctrl Pts',(67.0566574869574,-0.00149765431883376,
5.90407471946233));
#24905=CARTESIAN_POINT('Ctrl Pts',(67.0518463029865,0.585190437662473,5.93596947460409));
#24906=CARTESIAN_POINT('Ctrl Pts',(66.4813711624858,1.86148826198051,6.00491019326854));
#24907=CARTESIAN_POINT('Ctrl Pts',(64.3156972041947,2.33026144716285,6.11089687545566));
#24908=CARTESIAN_POINT('Ctrl Pts',(62.6710926659578,0.688814355154883,6.22203476602371));
#24909=CARTESIAN_POINT('Ctrl Pts',(63.1582101680956,-1.58293676398101,6.33317265659174));
#24910=CARTESIAN_POINT('Ctrl Pts',(65.3310466291073,-2.4061540266853,6.4443105471598));
#24911=CARTESIAN_POINT('Ctrl Pts',(66.8504470921567,-1.28501547118086,6.53461123478332));
#24912=CARTESIAN_POINT('Ctrl Pts',(67.0525105038734,-0.300747505180004,
6.58786595888416));
#24913=CARTESIAN_POINT('Ctrl Pts',(67.0515888779951,-0.000804696401304414,
6.60407471946233));
#24914=CARTESIAN_POINT('Ctrl Pts',(67.0519117333221,0.00102649957301758,
5.84592528053768));
#24915=CARTESIAN_POINT('Ctrl Pts',(67.0531633450758,0.277741730134882,5.86088026380211));
#24916=CARTESIAN_POINT('Ctrl Pts',(66.8721481216246,1.23835695251561,5.91288121058921));
#24917=CARTESIAN_POINT('Ctrl Pts',(65.4121253417219,2.39341760299657,6.001928120899));
#24918=CARTESIAN_POINT('Ctrl Pts',(63.2126643336617,1.64429852840487,6.11306601146706));
#24919=CARTESIAN_POINT('Ctrl Pts',(62.649189925264,-0.609850285121809,6.22420390203508));
#24920=CARTESIAN_POINT('Ctrl Pts',(64.2374031554985,-2.30582648807954,6.33534179260314));
#24921=CARTESIAN_POINT('Ctrl Pts',(66.4435230617629,-1.90573437919648,6.44258225210399));
#24922=CARTESIAN_POINT('Ctrl Pts',(67.0529326385894,-0.608118645715823,
6.51277674808218));
#24923=CARTESIAN_POINT('Ctrl Pts',(67.0572086816557,0.00119446450309495,
6.54592528053768));
#24924=CARTESIAN_POINT('Origin',(65.,0.,-3.54592528053767));
#24925=CARTESIAN_POINT('',(67.0534842785189,-0.00176526399347135,5.14592528053768));
#24926=CARTESIAN_POINT('',(67.0562728194261,0.00163389830066306,5.20407471946232));
#24927=CARTESIAN_POINT('',(67.05475,1.03216492799367E-13,-3.54592528053767));
#24928=CARTESIAN_POINT('Ctrl Pts',(67.0562728194261,0.00163389830066316,
5.20407471946232));
#24929=CARTESIAN_POINT('Ctrl Pts',(67.0572175303294,0.110331419494773,5.20998106327866));
#24930=CARTESIAN_POINT('Ctrl Pts',(66.9999469228229,0.899807785912472,5.25293337061767));
#24931=CARTESIAN_POINT('Ctrl Pts',(65.9773779060574,2.22328871643559,5.33293164147938));
#24932=CARTESIAN_POINT('Ctrl Pts',(63.6621652804381,2.02693883635741,5.44406953204741));
#24933=CARTESIAN_POINT('Ctrl Pts',(62.5714875417724,-0.0246926647779473,
5.55520742261546));
#24934=CARTESIAN_POINT('Ctrl Pts',(63.7036555936518,-2.05371969901983,5.66634531318349));
#24935=CARTESIAN_POINT('Ctrl Pts',(66.0223808123334,-2.20295969802021,5.77748320375154));
#24936=CARTESIAN_POINT('Ctrl Pts',(67.0084336557534,-0.871640043874865,
5.85672633917782));
#24937=CARTESIAN_POINT('Ctrl Pts',(67.0574345241562,-0.0962515598736413,
5.89892351108141));
#24938=CARTESIAN_POINT('Ctrl Pts',(67.0566574869574,-0.00149765431883376,
5.90407471946233));
#24939=CARTESIAN_POINT('Ctrl Pts',(67.0534842785189,-0.00176526399347133,
5.14592528053768));
#24940=CARTESIAN_POINT('Ctrl Pts',(67.049548506192,0.478623619806713,5.17193781599936));
#24941=CARTESIAN_POINT('Ctrl Pts',(66.641865899552,1.64918033378071,5.23499631498372));
#24942=CARTESIAN_POINT('Ctrl Pts',(64.6918158067503,2.4090050242139,5.33510077749075));
#24943=CARTESIAN_POINT('Ctrl Pts',(62.8089171959401,1.04758718972752,5.4462386680588));
#24944=CARTESIAN_POINT('Ctrl Pts',(62.931541830362,-1.27269881881276,5.55737655862684));
#24945=CARTESIAN_POINT('Ctrl Pts',(64.9474490817621,-2.42806968006158,5.66851444919488));
#24946=CARTESIAN_POINT('Ctrl Pts',(66.7337199477999,-1.50458731301855,5.7646973564985));
#24947=CARTESIAN_POINT('Ctrl Pts',(67.0500628960447,-0.407727598469997,
5.82383430027943));
#24948=CARTESIAN_POINT('Ctrl Pts',(67.0519117333221,0.00102649957301758,
5.84592528053768));
#24949=CARTESIAN_POINT('Origin',(65.,0.,-3.54592528053767));
#24950=CARTESIAN_POINT('',(67.0581446603105,8.27717201815131E-6,4.44592528053768));
#24951=CARTESIAN_POINT('',(67.051502599911,0.000468972833328433,4.50407471946232));
#24952=CARTESIAN_POINT('',(67.05475,1.03216492799367E-13,-3.54592528053767));
#24953=CARTESIAN_POINT('Ctrl Pts',(67.051502599911,0.000468972833328023,
4.50407471946232));
#24954=CARTESIAN_POINT('Ctrl Pts',(67.0521436877867,0.314512114650352,4.52103861547591));
#24955=CARTESIAN_POINT('Ctrl Pts',(66.8367516776872,1.31353269400003,4.57504847501217));
#24956=CARTESIAN_POINT('Ctrl Pts',(65.2821091229946,2.41219729396229,4.66610429807113));
#24957=CARTESIAN_POINT('Ctrl Pts',(63.1263775009061,1.54525729464231,4.77724218863916));
#24958=CARTESIAN_POINT('Ctrl Pts',(62.6855937936814,-0.736074256717675,
4.88838007920721));
#24959=CARTESIAN_POINT('Ctrl Pts',(64.3632123478174,-2.3436686423048,4.99951796977525));
#24960=CARTESIAN_POINT('Ctrl Pts',(66.5035583733625,-1.83464658396606,5.10474951652696));
#24961=CARTESIAN_POINT('Ctrl Pts',(67.0512920835974,-0.571444740237977,
5.17293509975598));
#24962=CARTESIAN_POINT('Ctrl Pts',(67.0562728194261,0.00163389830066316,
5.20407471946232));
#24963=CARTESIAN_POINT('Ctrl Pts',(67.0581446431809,8.27713025121955E-6,
4.44592528053768));
#24964=CARTESIAN_POINT('Ctrl Pts',(67.0581446696346,0.000451184114013542,
4.44594940467392));
#24965=CARTESIAN_POINT('Ctrl Pts',(67.0579439709526,0.681039286739863,4.48301949233285));
#24966=CARTESIAN_POINT('Ctrl Pts',(66.3158322777071,2.04129075981349,4.55713554351446));
#24967=CARTESIAN_POINT('Ctrl Pts',(63.9986308592856,2.21258726309085,4.66827343408251));
#24968=CARTESIAN_POINT('Ctrl Pts',(62.5979939690176,0.358677549762036,4.77941132465055));
#24969=CARTESIAN_POINT('Ctrl Pts',(63.3959404447162,-1.82353378810157,4.89054921521859));
#24970=CARTESIAN_POINT('Ctrl Pts',(65.6621008123707,-2.33664397819607,5.00168710578663));
#24971=CARTESIAN_POINT('Ctrl Pts',(66.9336682838985,-1.09149041292419,5.08681246089299));
#24972=CARTESIAN_POINT('Ctrl Pts',(67.0551536682982,-0.205526108395694,
5.13489185247667));
#24973=CARTESIAN_POINT('Ctrl Pts',(67.0534842785189,-0.00176526399347133,
5.14592528053768));
#24974=CARTESIAN_POINT('Origin',(65.,0.,-3.54592528053767));
#24975=CARTESIAN_POINT('',(67.0534601308484,0.00176006036930576,3.74592528053768));
#24976=CARTESIAN_POINT('',(67.0545529589347,-0.00187890219045319,3.80407471946232));
#24977=CARTESIAN_POINT('',(67.05475,1.03216492799367E-13,-3.54592528053767));
#24978=CARTESIAN_POINT('Ctrl Pts',(67.0545529589347,-0.00187890219045316,
3.80407471946232));
#24979=CARTESIAN_POINT('Ctrl Pts',(67.049847975054,0.514925815374004,3.83209616767316));
#24980=CARTESIAN_POINT('Ctrl Pts',(66.5901947888396,1.72243254492319,3.89716357940667));
#24981=CARTESIAN_POINT('Ctrl Pts',(64.5620129419189,2.3888174265201,3.99927695466288));
#24982=CARTESIAN_POINT('Ctrl Pts',(62.7554801641395,0.927583994626953,4.11041484523091));
#24983=CARTESIAN_POINT('Ctrl Pts',(63.0033818465923,-1.38267758750649,4.22155273579896));
#24984=CARTESIAN_POINT('Ctrl Pts',(65.0788107682801,-2.42735869229696,4.33269062636699));
#24985=CARTESIAN_POINT('Ctrl Pts',(66.7763241812549,-1.4299225698547,4.42686462092146));
#24986=CARTESIAN_POINT('Ctrl Pts',(67.0507436722455,-0.371299138082136,
4.48399265195323));
#24987=CARTESIAN_POINT('Ctrl Pts',(67.051502599911,0.000468972833328023,
4.50407471946232));
#24988=CARTESIAN_POINT('Ctrl Pts',(67.0534601308484,0.00176006036930547,
3.74592528053768));
#24989=CARTESIAN_POINT('Ctrl Pts',(67.055130441991,0.206418025502595,3.75700695687117));
#24990=CARTESIAN_POINT('Ctrl Pts',(66.9329701809384,1.09329696547217,3.80513459672735));
#24991=CARTESIAN_POINT('Ctrl Pts',(65.6590644304509,2.33750221987791,3.89030820010621));
#24992=CARTESIAN_POINT('Ctrl Pts',(63.39357261301,1.82144821550899,4.00144609067426));
#24993=CARTESIAN_POINT('Ctrl Pts',(62.5984620009619,-0.361797997181331,
4.1125839812423));
#24994=CARTESIAN_POINT('Ctrl Pts',(64.0015063548152,-2.21388639990766,4.22372187181034));
#24995=CARTESIAN_POINT('Ctrl Pts',(66.3179803312342,-2.0396173096854,4.33483563824213));
#24996=CARTESIAN_POINT('Ctrl Pts',(67.0581040462783,-0.679694036228919,
4.40890344115124));
#24997=CARTESIAN_POINT('Ctrl Pts',(67.0581446431809,8.27713025121955E-6,
4.44592528053768));
#24998=CARTESIAN_POINT('Origin',(65.,0.,-3.54592528053767));
#24999=CARTESIAN_POINT('',(67.0519256006226,-0.00103910123988304,3.04592528053768));
#25000=CARTESIAN_POINT('',(67.0578709601416,0.000678769155110521,3.10407471946232));
#25001=CARTESIAN_POINT('',(67.05475,1.03216492799367E-13,-3.54592528053767));
#25002=CARTESIAN_POINT('Ctrl Pts',(67.0578709601415,0.000678769155110595,
3.10407471946232));
#25003=CARTESIAN_POINT('Ctrl Pts',(67.0580316799421,0.0380175835266752,
3.10610775634773));
#25004=CARTESIAN_POINT('Ctrl Pts',(67.0401889053665,0.755586934309662,3.14518675675581));
#25005=CARTESIAN_POINT('Ctrl Pts',(66.2035357618251,2.10945088366341,3.22131172068658));
#25006=CARTESIAN_POINT('Ctrl Pts',(63.8804623217255,2.15520689204012,3.33244961125462));
#25007=CARTESIAN_POINT('Ctrl Pts',(62.5821144149725,0.228277590427784,3.44358750182266));
#25008=CARTESIAN_POINT('Ctrl Pts',(63.4968846048806,-1.90759677855456,3.55472539239071));
#25009=CARTESIAN_POINT('Ctrl Pts',(65.7874733624335,-2.29742618249227,3.66586328295874));
#25010=CARTESIAN_POINT('Ctrl Pts',(66.9614802130625,-1.01630569367123,3.74897972531595));
#25011=CARTESIAN_POINT('Ctrl Pts',(67.0560682339038,-0.168319696106675,
3.79505020415048));
#25012=CARTESIAN_POINT('Ctrl Pts',(67.0545529589347,-0.00187890219045316,
3.80407471946232));
#25013=CARTESIAN_POINT('Ctrl Pts',(67.0519256006226,-0.00103910123988287,
3.04592528053768));
#25014=CARTESIAN_POINT('Ctrl Pts',(67.0500496331103,0.408601099978646,3.06806450906842));
#25015=CARTESIAN_POINT('Ctrl Pts',(66.7326598083642,1.50637690262578,3.12724970112185));
#25016=CARTESIAN_POINT('Ctrl Pts',(64.9442948490232,2.42799907075925,3.22348085669796));
#25017=CARTESIAN_POINT('Ctrl Pts',(62.9298898830713,1.27001049414665,3.334618747266));
#25018=CARTESIAN_POINT('Ctrl Pts',(62.8102801837889,-1.05043309065764,3.44575663783405));
#25019=CARTESIAN_POINT('Ctrl Pts',(64.6949458653977,-2.40940335486022,3.55689452840209));
#25020=CARTESIAN_POINT('Ctrl Pts',(66.643067780423,-1.64741324066796,3.65695074263663));
#25021=CARTESIAN_POINT('Ctrl Pts',(67.0495466039689,-0.47775206598754,3.71996099334849));
#25022=CARTESIAN_POINT('Ctrl Pts',(67.0534601308484,0.00176006036930547,
3.74592528053768));
#25023=CARTESIAN_POINT('Origin',(65.,0.,-3.54592528053767));
#25024=CARTESIAN_POINT('',(67.0572522603608,-0.00120217803179352,2.34592528053767));
#25025=CARTESIAN_POINT('',(67.0525490214284,0.00145097609281634,2.40407471946232));
#25026=CARTESIAN_POINT('',(67.05475,1.03216492799367E-13,-3.54592528053767));
#25027=CARTESIAN_POINT('Ctrl Pts',(67.0525490214284,0.00145097609281618,
2.40407471946232));
#25028=CARTESIAN_POINT('Ctrl Pts',(67.054127131265,0.243480442393218,2.41716530854498));
#25029=CARTESIAN_POINT('Ctrl Pts',(66.9026176062656,1.16853384943059,2.46730186115031));
#25030=CARTESIAN_POINT('Ctrl Pts',(65.5317127142361,2.36971790517293,2.55448437727833));
#25031=CARTESIAN_POINT('Ctrl Pts',(63.2974379205056,1.7319248615472,2.66562226784637));
#25032=CARTESIAN_POINT('Ctrl Pts',(62.6215375065036,-0.491118649216439,
2.77676015841441));
#25033=CARTESIAN_POINT('Ctrl Pts',(64.122670786398,-2.2646356906881,2.88789804898245));
#25034=CARTESIAN_POINT('Ctrl Pts',(66.3846835747723,-1.97078161673766,2.99700290266509));
#25035=CARTESIAN_POINT('Ctrl Pts',(67.0551030464715,-0.642369656429112,
3.06906179282505));
#25036=CARTESIAN_POINT('Ctrl Pts',(67.0578709601415,0.000678769155110595,
3.10407471946232));
#25037=CARTESIAN_POINT('Ctrl Pts',(67.0572522603608,-0.00120217803179366,
2.34592528053767));
#25038=CARTESIAN_POINT('Ctrl Pts',(67.0530108672503,0.608976283722048,2.37912206126567));
#25039=CARTESIAN_POINT('Ctrl Pts',(66.4420019119215,1.9074607758001,2.44936480551635));
#25040=CARTESIAN_POINT('Ctrl Pts',(64.234427664365,2.30481703186258,2.55665351328971));
#25041=CARTESIAN_POINT('Ctrl Pts',(62.6483896081628,0.606804018161656,2.66779140385776));
#25042=CARTESIAN_POINT('Ctrl Pts',(63.214807212685,-1.64662359498827,2.77892929442579));
#25043=CARTESIAN_POINT('Ctrl Pts',(65.4152320208998,-2.39287795766375,2.89006718499384));
#25044=CARTESIAN_POINT('Ctrl Pts',(66.8729657074861,-1.23655088859839,2.97906584703113));
#25045=CARTESIAN_POINT('Ctrl Pts',(67.0531887228005,-0.276857109673458,
3.03101854554574));
#25046=CARTESIAN_POINT('Ctrl Pts',(67.0519256006226,-0.00103910123988287,
3.04592528053768));
#25047=CARTESIAN_POINT('Origin',(65.,0.,-3.54592528053767));
#25048=CARTESIAN_POINT('',(67.0555677501283,0.00179912738464932,1.64592528053767));
#25049=CARTESIAN_POINT('',(67.0526273462695,-0.00148795516933082,1.70407471946232));
#25050=CARTESIAN_POINT('',(67.05475,1.03216492799367E-13,-3.54592528053767));
#25051=CARTESIAN_POINT('Ctrl Pts',(67.0526273462695,-0.00148795516933075,
1.70407471946232));
#25052=CARTESIAN_POINT('Ctrl Pts',(67.049634688556,0.444939705966117,1.72822286074222));
#25053=CARTESIAN_POINT('Ctrl Pts',(66.6869954305654,1.58066428073723,1.78941696554481));
#25054=CARTESIAN_POINT('Ctrl Pts',(64.8130956691436,2.42143513885567,1.88765703387008));
#25055=CARTESIAN_POINT('Ctrl Pts',(62.864249480632,1.15622276382909,1.99879492443812));
#25056=CARTESIAN_POINT('Ctrl Pts',(62.8702799635561,-1.16729341938809,2.10993281500616));
#25057=CARTESIAN_POINT('Ctrl Pts',(64.8256673485052,-2.42237269783168,2.2210707055742));
#25058=CARTESIAN_POINT('Ctrl Pts',(66.6915092429239,-1.57355497286027,2.31911800705959));
#25059=CARTESIAN_POINT('Ctrl Pts',(67.0496611290802,-0.441455485498565,
2.3801193450223));
#25060=CARTESIAN_POINT('Ctrl Pts',(67.0525490214284,0.00145097609281618,
2.40407471946232));
#25061=CARTESIAN_POINT('Ctrl Pts',(67.0555677501283,0.00179912738464925,
1.64592528053767));
#25062=CARTESIAN_POINT('Ctrl Pts',(67.0567846151392,0.134576239702318,1.65313364994024));
#25063=CARTESIAN_POINT('Ctrl Pts',(66.9845642825309,0.948416460674401,1.69738798286549));
#25064=CARTESIAN_POINT('Ctrl Pts',(65.898842928637,2.25618349012117,1.77868827931342));
#25065=CARTESIAN_POINT('Ctrl Pts',(63.5919355659201,1.97879688218179,1.88982616988146));
#25066=CARTESIAN_POINT('Ctrl Pts',(62.5738455482538,-0.109804953100732,
2.0009640604495));
#25067=CARTESIAN_POINT('Ctrl Pts',(63.7764422147334,-2.09790106953769,2.11210195101754));
#25068=CARTESIAN_POINT('Ctrl Pts',(66.0989751981566,-2.1657645452103,2.22323984158559));
#25069=CARTESIAN_POINT('Ctrl Pts',(67.0223280499568,-0.823134106038537,
2.30118095142563));
#25070=CARTESIAN_POINT('Ctrl Pts',(67.0577440519451,-0.0719526660358301,
2.34207609774299));
#25071=CARTESIAN_POINT('Ctrl Pts',(67.0572522603608,-0.00120217803179366,
2.34592528053767));
#25072=CARTESIAN_POINT('Origin',(65.,0.,-3.54592528053767));
#25073=CARTESIAN_POINT('',(67.0514068858608,7.8101351718568E-5,0.945925280537675));
#25074=CARTESIAN_POINT('',(67.0579182146741,-0.000617375283490038,1.00407471946232));
#25075=CARTESIAN_POINT('',(67.05475,1.03216492799367E-13,-3.54592528053767));
#25076=CARTESIAN_POINT('Ctrl Pts',(67.0579182146741,-0.000617375283489987,
1.00407471946232));
#25077=CARTESIAN_POINT('Ctrl Pts',(67.0553588641481,0.645931829998614,1.03928041293948));
#25078=CARTESIAN_POINT('Ctrl Pts',(66.378434179731,1.97744423729901,1.11153206993931));
#25079=CARTESIAN_POINT('Ctrl Pts',(64.1109273576576,2.26005114925193,1.22082969046183));
#25080=CARTESIAN_POINT('Ctrl Pts',(62.6190202559434,0.478765933382519,1.33196758102987));
#25081=CARTESIAN_POINT('Ctrl Pts',(63.3064509161112,-1.74073917087913,1.44310547159791));
#25082=CARTESIAN_POINT('Ctrl Pts',(65.5440062589152,-2.36692597071416,1.55424336216595));
#25083=CARTESIAN_POINT('Ctrl Pts',(66.9056402449312,-1.16131362127399,1.64123311145409));
#25084=CARTESIAN_POINT('Ctrl Pts',(67.0542257619312,-0.239930514819838,
1.69117689721954));
#25085=CARTESIAN_POINT('Ctrl Pts',(67.0526273462695,-0.00148795516933075,
1.70407471946232));
#25086=CARTESIAN_POINT('Ctrl Pts',(67.0514068858608,7.81013517185333E-5,
0.945925280537675));
#25087=CARTESIAN_POINT('Ctrl Pts',(67.0515215449353,0.33826440094154,0.964191202137492));
#25088=CARTESIAN_POINT('Ctrl Pts',(66.8123460743743,1.36218935655875,1.01950308725999));
#25089=CARTESIAN_POINT('Ctrl Pts',(65.1973793755662,2.42060404314488,1.11186093590517));
#25090=CARTESIAN_POINT('Ctrl Pts',(63.0733618200821,1.47863040518407,1.22299882647321));
#25091=CARTESIAN_POINT('Ctrl Pts',(62.7128180402749,-0.816750411403602,
1.33413671704125));
#25092=CARTESIAN_POINT('Ctrl Pts',(64.4457578465939,-2.36455031387796,1.4452746076093));
#25093=CARTESIAN_POINT('Ctrl Pts',(66.5407002488233,-1.7880364866664,1.54920412877477));
#25094=CARTESIAN_POINT('Ctrl Pts',(67.0505307823665,-0.547805001444293,
1.61608768641756));
#25095=CARTESIAN_POINT('Ctrl Pts',(67.0555677501283,0.00179912738464925,
1.64592528053767));
#25096=CARTESIAN_POINT('Origin',(65.,0.,-3.54592528053767));
#25097=CARTESIAN_POINT('',(67.05528106155,-0.00183967754518108,0.245925280537674));
#25098=CARTESIAN_POINT('',(67.0544463703074,0.00187701683783275,0.304074719462319));
#25099=CARTESIAN_POINT('',(67.05475,1.03216492799367E-13,-3.54592528053767));
#25100=CARTESIAN_POINT('Ctrl Pts',(67.0544463703074,0.00187701683783252,
0.304074719462319));
#25101=CARTESIAN_POINT('Ctrl Pts',(67.0559854674868,0.17189554728647,0.313292001614044));
#25102=CARTESIAN_POINT('Ctrl Pts',(66.9589165461202,1.02351658402418,0.359555247288449));
#25103=CARTESIAN_POINT('Ctrl Pts',(65.7755372964953,2.301482839391,0.442864456485536));
#25104=CARTESIAN_POINT('Ctrl Pts',(63.4870029209119,1.89976872281362,0.554002347053577));
#25105=CARTESIAN_POINT('Ctrl Pts',(62.5833319303427,-0.24082525149545,0.665140237621619));
#25106=CARTESIAN_POINT('Ctrl Pts',(63.8916646308255,-2.16098914151125,0.77627812818966));
#25107=CARTESIAN_POINT('Ctrl Pts',(66.2144692640843,-2.1031751632491,0.887416018757702));
#25108=CARTESIAN_POINT('Ctrl Pts',(67.0419827284221,-0.748425825038277,
0.963348215848589));
#25109=CARTESIAN_POINT('Ctrl Pts',(67.058051996902,-0.0344137592749356,
1.0022344494168));
#25110=CARTESIAN_POINT('Ctrl Pts',(67.0579182146741,-0.000617375283489987,
1.00407471946232));
#25111=CARTESIAN_POINT('Ctrl Pts',(67.05528106155,-0.00183967754518099,
0.245925280537674));
#25112=CARTESIAN_POINT('Ctrl Pts',(67.0502944995635,0.538488282262984,0.275248754334741));
#25113=CARTESIAN_POINT('Ctrl Pts',(66.5549829233901,1.76953115899708,0.341618191654489));
#25114=CARTESIAN_POINT('Ctrl Pts',(64.4785452214709,2.37199651591817,0.445033592496919));
#25115=CARTESIAN_POINT('Ctrl Pts',(62.7243441135659,0.848335334231218,0.55617148306496));
#25116=CARTESIAN_POINT('Ctrl Pts',(63.0530766482751,-1.45181679686653,0.667309373633002));
#25117=CARTESIAN_POINT('Ctrl Pts',(65.1638502053818,-2.42310455048396,0.778447264201043));
#25118=CARTESIAN_POINT('Ctrl Pts',(66.8023851755325,-1.38138173267994,0.871319233169269));
#25119=CARTESIAN_POINT('Ctrl Pts',(67.0512889995436,-0.347626932272121,
0.927145238614812));
#25120=CARTESIAN_POINT('Ctrl Pts',(67.0514068858608,7.81013517185333E-5,
0.945925280537675));
#25121=CARTESIAN_POINT('Origin',(65.,0.,-3.54592528053767));
#25122=CARTESIAN_POINT('',(67.0574561899986,0.00106563322408104,-0.454074719462326));
#25123=CARTESIAN_POINT('',(67.0515283628764,-0.00052555615327251,-0.39592528053768));
#25124=CARTESIAN_POINT('',(67.05475,1.03216492799367E-13,-3.54592528053767));
#25125=CARTESIAN_POINT('Ctrl Pts',(67.0515283628764,-0.000525556153272815,
-0.39592528053768));
#25126=CARTESIAN_POINT('Ctrl Pts',(67.0506691385159,0.374799386930355,-0.375650446188706));
#25127=CARTESIAN_POINT('Ctrl Pts',(66.7723630529996,1.43710026477805,-0.318329648317051));
#25128=CARTESIAN_POINT('Ctrl Pts',(65.0662097961853,2.42773505180943,-0.223962886922715));
#25129=CARTESIAN_POINT('Ctrl Pts',(62.9962315570428,1.3722949487109,-0.112824996354674));
#25130=CARTESIAN_POINT('Ctrl Pts',(62.7603252963136,-0.939222336522784,
-0.00168710578663132));
#25131=CARTESIAN_POINT('Ctrl Pts',(64.5744186923722,-2.39105873890072,0.10945078478141));
#25132=CARTESIAN_POINT('Ctrl Pts',(66.5952919861857,-1.71543281453754,0.211371393197727));
#25133=CARTESIAN_POINT('Ctrl Pts',(67.0497995509631,-0.511440405058377,
0.276246038091363));
#25134=CARTESIAN_POINT('Ctrl Pts',(67.0544463703074,0.00187701683783252,
0.304074719462319));
#25135=CARTESIAN_POINT('Ctrl Pts',(67.0574561899986,0.00106563322408115,
-0.454074719462326));
#25136=CARTESIAN_POINT('Ctrl Pts',(67.057843018648,0.0623502628450632,-0.450739656990689));
#25137=CARTESIAN_POINT('Ctrl Pts',(67.0275621697751,0.8039986152436,-0.410358630996372));
#25138=CARTESIAN_POINT('Ctrl Pts',(66.1288520704621,2.15034287637184,-0.332931641479373));
#25139=CARTESIAN_POINT('Ctrl Pts',(63.8056023683761,2.11463875683278,-0.221793750911332));
#25140=CARTESIAN_POINT('Ctrl Pts',(62.5755981242121,0.143381478345983,-0.110655860343291));
#25141=CARTESIAN_POINT('Ctrl Pts',(63.5646765331008,-1.95911432942998,0.00048203022475183));
#25142=CARTESIAN_POINT('Ctrl Pts',(65.8675227272721,-2.26841065672895,0.111619920792793));
#25143=CARTESIAN_POINT('Ctrl Pts',(66.9782240837151,-0.967625288007803,
0.193434337563767));
#25144=CARTESIAN_POINT('Ctrl Pts',(67.0565942986505,-0.144137863188426,
0.238202790812061));
#25145=CARTESIAN_POINT('Ctrl Pts',(67.05528106155,-0.00183967754518099,
0.245925280537674));
#25146=CARTESIAN_POINT('Origin',(65.,0.,-3.54592528053767));
#25147=CARTESIAN_POINT('',(67.0520762837074,0.00116136879359838,-1.15407471946233));
#25148=CARTESIAN_POINT('',(67.0563730581704,-0.00160407492545605,-1.09592528053768));
#25149=CARTESIAN_POINT('',(67.05475,1.03216492799367E-13,-3.54592528053767));
#25150=CARTESIAN_POINT('Ctrl Pts',(67.0563730581704,-0.00160407492545608,
-1.09592528053768));
#25151=CARTESIAN_POINT('Ctrl Pts',(67.051425463294,0.574948872440279,-1.06459289399146));
#25152=CARTESIAN_POINT('Ctrl Pts',(66.4979405147664,1.84151750410659,-0.99621454392255));
#25153=CARTESIAN_POINT('Ctrl Pts',(64.3510553719621,2.34032995360773,-0.890790230330967));
#25154=CARTESIAN_POINT('Ctrl Pts',(62.6818041989874,0.724051597351488,-0.779652339762924));
#25155=CARTESIAN_POINT('Ctrl Pts',(63.1344238327198,-1.55496249063293,-0.668514449194883));
#25156=CARTESIAN_POINT('Ctrl Pts',(65.2946265402067,-2.41070020734327,-0.55737655862684));
#25157=CARTESIAN_POINT('Ctrl Pts',(66.8402661138972,-1.30632380217904,-0.466513502407773));
#25158=CARTESIAN_POINT('Ctrl Pts',(67.0522391042067,-0.310990391240213,
-0.412696409711387));
#25159=CARTESIAN_POINT('Ctrl Pts',(67.0515283628764,-0.000525556153272815,
-0.39592528053768));
#25160=CARTESIAN_POINT('Ctrl Pts',(67.0520762837074,0.0011613687935982,
-1.15407471946233));
#25161=CARTESIAN_POINT('Ctrl Pts',(67.053454237916,0.267420438121936,-1.13968210479344));
#25162=CARTESIAN_POINT('Ctrl Pts',(66.8815877450925,1.2173135829094,-1.08824352660187));
#25163=CARTESIAN_POINT('Ctrl Pts',(65.4483108550045,2.38688976599863,-0.999758984887625));
#25164=CARTESIAN_POINT('Ctrl Pts',(63.2377776981899,1.67118490708906,-0.888621094319582));
#25165=CARTESIAN_POINT('Ctrl Pts',(62.6402125087857,-0.574193448178934,
-0.777483203751542));
#25166=CARTESIAN_POINT('Ctrl Pts',(64.2025947176117,-2.29399639382145,-0.666345313183498));
#25167=CARTESIAN_POINT('Ctrl Pts',(66.4260607263055,-1.92548386768538,-0.558542485087094));
#25168=CARTESIAN_POINT('Ctrl Pts',(67.0535461156186,-0.61840104923623,-0.48778562051337));
#25169=CARTESIAN_POINT('Ctrl Pts',(67.0574561899986,0.00106563322408115,
-0.454074719462326));
#25170=CARTESIAN_POINT('Origin',(65.,0.,-3.54592528053767));
#25171=CARTESIAN_POINT('',(67.052679279082,-0.00238369513522838,-1.85407471946233));
#25172=CARTESIAN_POINT('',(67.0565599569794,0.00149374744778724,-1.79592528053768));
#25173=CARTESIAN_POINT('',(67.05475,1.03216492799367E-13,-3.54592528053767));
#25174=CARTESIAN_POINT('',(65.5301702171886,-1.98517432567172,-2.));
#25175=CARTESIAN_POINT('Ctrl Pts',(65.5301702171886,-1.98517432567172,-2.));
#25176=CARTESIAN_POINT('Ctrl Pts',(66.1902879097456,-1.80888011517988,-1.96295403647732));
#25177=CARTESIAN_POINT('Ctrl Pts',(66.9249664054372,-1.11286144556363,-1.91431227629809));
#25178=CARTESIAN_POINT('Ctrl Pts',(67.0542991139265,-0.216633244974144,
-1.86567051611887));
#25179=CARTESIAN_POINT('Ctrl Pts',(67.052679279082,-0.0023836951352286,
-1.85407471946232));
#25180=CARTESIAN_POINT('',(64.468704775017,-1.98873730573667,-2.));
#25181=CARTESIAN_POINT('Origin',(65.,0.,-2.));
#25182=CARTESIAN_POINT('Ctrl Pts',(64.4687042096542,-1.98873909628092,-2.));
#25183=CARTESIAN_POINT('Ctrl Pts',(65.1133181823237,-2.16007183004145,-1.96367708181445));
#25184=CARTESIAN_POINT('Ctrl Pts',(66.4930415100228,-1.84061483765584,-1.89565217532701));
#25185=CARTESIAN_POINT('Ctrl Pts',(67.051699865038,-0.581583302606355,-1.82762726883957));
#25186=CARTESIAN_POINT('Ctrl Pts',(67.0565599569794,0.0014937474477871,
-1.79592528053768));
#25187=CARTESIAN_POINT('Origin',(32.5,56.2916512459885,17.));
#25188=CARTESIAN_POINT('',(31.6672724934037,54.8468960395935,13.8714803633902));
#25189=CARTESIAN_POINT('',(31.6651566506305,54.8475988206466,13.6785196366098));
#25190=CARTESIAN_POINT('',(31.667,54.8488529232836,17.));
#25191=CARTESIAN_POINT('',(31.9588970197441,54.7159724828016,13.));
#25192=CARTESIAN_POINT('Ctrl Pts',(31.6651566506305,54.8475988206466,13.6785196366098));
#25193=CARTESIAN_POINT('Ctrl Pts',(31.6146486514652,54.8762889946569,13.6746222055426));
#25194=CARTESIAN_POINT('Ctrl Pts',(31.5657632473174,54.9077117506004,13.6707247744754));
#25195=CARTESIAN_POINT('Ctrl Pts',(31.5188321868552,54.9418237568819,13.6668273434082));
#25196=CARTESIAN_POINT('Ctrl Pts',(31.0727418458088,55.2660660894878,13.6297813798856));
#25197=CARTESIAN_POINT('Ctrl Pts',(30.8032251342758,55.8332803703507,13.5927354163629));
#25198=CARTESIAN_POINT('Ctrl Pts',(30.8337540098497,56.3839156387153,13.5556894528402));
#25199=CARTESIAN_POINT('Ctrl Pts',(30.8642828854237,56.93455090708,13.5186434893175));
#25200=CARTESIAN_POINT('Ctrl Pts',(31.1948573481046,57.4686071629464,13.4815975257948));
#25201=CARTESIAN_POINT('Ctrl Pts',(31.6739356569701,57.7415946577538,13.4445515622722));
#25202=CARTESIAN_POINT('Ctrl Pts',(32.1530139658356,58.0145821525613,13.4075055987495));
#25203=CARTESIAN_POINT('Ctrl Pts',(32.7805961208856,58.0265008863098,13.3704596352268));
#25204=CARTESIAN_POINT('Ctrl Pts',(33.2699721109727,57.7720492096737,13.3334136717041));
#25205=CARTESIAN_POINT('Ctrl Pts',(33.7593481010598,57.5175975330377,13.2963677081814));
#25206=CARTESIAN_POINT('Ctrl Pts',(34.1105179261839,56.9967754460172,13.2593217446588));
#25207=CARTESIAN_POINT('Ctrl Pts',(34.1617369653364,56.4476202824107,13.2222757811361));
#25208=CARTESIAN_POINT('Ctrl Pts',(34.2129560044889,55.8984651188042,13.1852298176134));
#25209=CARTESIAN_POINT('Ctrl Pts',(33.9642242576698,55.3209768786118,13.1481838540907));
#25210=CARTESIAN_POINT('Ctrl Pts',(33.5316971804146,54.9803713160329,13.111137890568));
#25211=CARTESIAN_POINT('Ctrl Pts',(33.0991701031595,54.639765753454,13.0740919270454));
#25212=CARTESIAN_POINT('Ctrl Pts',(32.4828476954683,54.5360428684886,13.0370459635227));
#25213=CARTESIAN_POINT('Ctrl Pts',(31.9588970197441,54.7159724828016,13.));
#25214=CARTESIAN_POINT('',(31.0290140863628,57.0802261258961,13.));
#25215=CARTESIAN_POINT('Origin',(32.5,56.2916512459885,13.));
#25216=CARTESIAN_POINT('',(31.6688354432561,54.8507324474214,13.1714803633902));
#25217=CARTESIAN_POINT('Ctrl Pts',(31.0290124456509,57.0802271145804,13.));
#25218=CARTESIAN_POINT('Ctrl Pts',(30.774120583937,56.6032768580681,13.0363229181856));
#25219=CARTESIAN_POINT('Ctrl Pts',(30.7719333897513,55.9901147282721,13.0726458363711));
#25220=CARTESIAN_POINT('Ctrl Pts',(31.0246770579875,55.5119982833858,13.1089687545567));
#25221=CARTESIAN_POINT('Ctrl Pts',(31.1696673663398,55.2377194013227,13.1298059575012));
#25222=CARTESIAN_POINT('Ctrl Pts',(31.3985533923309,55.0078829792344,13.1506431604457));
#25223=CARTESIAN_POINT('Ctrl Pts',(31.6688354432561,54.8507324474214,13.1714803633902));
#25224=CARTESIAN_POINT('',(31.667,54.8488529232836,12.));
#25225=CARTESIAN_POINT('',(31.667,54.8488529232836,17.));
#25226=CARTESIAN_POINT('Origin',(32.5,56.2916512459885,12.));
#25227=CARTESIAN_POINT('Ctrl Pts',(31.6688354432561,54.8507324474214,13.1714803633902));
#25228=CARTESIAN_POINT('Ctrl Pts',(31.8790813703937,54.7284888165622,13.1876891239684));
#25229=CARTESIAN_POINT('Ctrl Pts',(32.1143756641562,54.6502267716398,13.2038978845465));
#25230=CARTESIAN_POINT('Ctrl Pts',(32.354714319885,54.6292400960994,13.2201066451247));
#25231=CARTESIAN_POINT('Ctrl Pts',(32.9040207909308,54.5812739599608,13.2571526086474));
#25232=CARTESIAN_POINT('Ctrl Pts',(33.4796777351052,54.8324998905166,13.2941985721701));
#25233=CARTESIAN_POINT('Ctrl Pts',(33.8179820369827,55.2680242179702,13.3312445356927));
#25234=CARTESIAN_POINT('Ctrl Pts',(34.1562863388601,55.7035485454237,13.3682904992154));
#25235=CARTESIAN_POINT('Ctrl Pts',(34.2572379984405,56.323371269775,13.4053364627381));
#25236=CARTESIAN_POINT('Ctrl Pts',(34.074760972003,56.8437863823056,13.4423824262608));
#25237=CARTESIAN_POINT('Ctrl Pts',(33.8922839455655,57.3642014948362,13.4794283897835));
#25238=CARTESIAN_POINT('Ctrl Pts',(33.4263782331101,57.7852089955461,13.5164743533061));
#25239=CARTESIAN_POINT('Ctrl Pts',(32.8902057561615,57.9141527098528,13.5535203168288));
#25240=CARTESIAN_POINT('Ctrl Pts',(32.3540332792128,58.0430964241595,13.5905662803515));
#25241=CARTESIAN_POINT('Ctrl Pts',(31.7475940377708,57.879976352063,13.6276122438742));
#25242=CARTESIAN_POINT('Ctrl Pts',(31.3484595971705,57.499435180452,13.6646582073969));
#25243=CARTESIAN_POINT('Ctrl Pts',(30.9493251565702,57.1188940088411,13.7017041709196));
#25244=CARTESIAN_POINT('Ctrl Pts',(30.7574955168115,56.5209317377157,13.7387501344422));
#25245=CARTESIAN_POINT('Ctrl Pts',(30.8607470097836,55.9792142563288,13.7757960979649));
#25246=CARTESIAN_POINT('Ctrl Pts',(30.9496414742062,55.5128221104133,13.8076908531067));
#25247=CARTESIAN_POINT('Ctrl Pts',(31.2572608237868,55.0881206516064,13.8395856082484));
#25248=CARTESIAN_POINT('Ctrl Pts',(31.6672724934037,54.8468960395935,13.8714803633902));
#25249=CARTESIAN_POINT('Origin',(32.5,56.2916512459885,17.));
#25250=CARTESIAN_POINT('',(31.6652293984911,54.8484357012869,14.5714803633902));
#25251=CARTESIAN_POINT('',(31.6674240358463,54.8512520230129,14.3785196366098));
#25252=CARTESIAN_POINT('',(31.667,54.8488529232836,17.));
#25253=CARTESIAN_POINT('Ctrl Pts',(31.6674240358463,54.8512520230129,14.3785196366098));
#25254=CARTESIAN_POINT('Ctrl Pts',(31.4726121759195,54.9625548712859,14.3635646533454));
#25255=CARTESIAN_POINT('Ctrl Pts',(31.2997293296831,55.1111079954895,14.3486096700809));
#25256=CARTESIAN_POINT('Ctrl Pts',(31.1659805795344,55.289072307877,14.3336546868165));
#25257=CARTESIAN_POINT('Ctrl Pts',(30.8346628353681,55.7299193023853,14.2966087232938));
#25258=CARTESIAN_POINT('Ctrl Pts',(30.7434854934753,56.3512435601479,14.2595627597711));
#25259=CARTESIAN_POINT('Ctrl Pts',(30.9341783443449,56.8686931008725,14.2225167962485));
#25260=CARTESIAN_POINT('Ctrl Pts',(31.1248711952145,57.386142641597,14.1854708327258));
#25261=CARTESIAN_POINT('Ctrl Pts',(31.5974342388466,57.7997174652835,14.1484248692031));
#25262=CARTESIAN_POINT('Ctrl Pts',(32.1355923903503,57.9201415291698,14.1113789056804));
#25263=CARTESIAN_POINT('Ctrl Pts',(32.6737505418539,58.0405655930561,14.0743329421577));
#25264=CARTESIAN_POINT('Ctrl Pts',(33.2775038012292,57.8678388971422,14.0372869786351));
#25265=CARTESIAN_POINT('Ctrl Pts',(33.6705489273999,57.4810131538507,14.0002410151124));
#25266=CARTESIAN_POINT('Ctrl Pts',(34.0635940535707,57.0941874105591,13.9631950515897));
#25267=CARTESIAN_POINT('Ctrl Pts',(34.2459310465369,56.4932626198898,13.926149088067));
#25268=CARTESIAN_POINT('Ctrl Pts',(34.1340966146064,55.9532506956148,13.8891031245443));
#25269=CARTESIAN_POINT('Ctrl Pts',(34.0222621826759,55.4132387713398,13.8520571610217));
#25270=CARTESIAN_POINT('Ctrl Pts',(33.6162563258486,54.934139713459,13.815011197499));
#25271=CARTESIAN_POINT('Ctrl Pts',(33.1019214121551,54.7352253766931,13.7779652339763));
#25272=CARTESIAN_POINT('Ctrl Pts',(32.6416972484852,54.5572378789698,13.7448167015208));
#25273=CARTESIAN_POINT('Ctrl Pts',(32.0947386036493,54.6035824036932,13.7116681690653));
#25274=CARTESIAN_POINT('Ctrl Pts',(31.6651566506305,54.8475988206466,13.6785196366098));
#25275=CARTESIAN_POINT('Ctrl Pts',(31.6672724934037,54.8468960395935,13.8714803633902));
#25276=CARTESIAN_POINT('Ctrl Pts',(31.7334920188215,54.8079367110906,13.8766315717711));
#25277=CARTESIAN_POINT('Ctrl Pts',(31.8023823793453,54.7737632532799,13.881782780152));
#25278=CARTESIAN_POINT('Ctrl Pts',(31.8734534906151,54.7449729811027,13.886933988533));
#25279=CARTESIAN_POINT('Ctrl Pts',(32.3845758527714,54.537921878912,13.9239799520556));
#25280=CARTESIAN_POINT('Ctrl Pts',(33.0084879513813,54.609292366179,13.9610259155783));
#25281=CARTESIAN_POINT('Ctrl Pts',(33.4596489857383,54.9264225988407,13.998071879101));
#25282=CARTESIAN_POINT('Ctrl Pts',(33.9108100200953,55.2435528315024,14.0351178426237));
#25283=CARTESIAN_POINT('Ctrl Pts',(34.1892199901994,55.8064428095589,14.0721638061464));
#25284=CARTESIAN_POINT('Ctrl Pts',(34.1674649383536,56.3574821112237,14.109209769669));
#25285=CARTESIAN_POINT('Ctrl Pts',(34.1457098865078,56.9085214128884,14.1462557331917));
#25286=CARTESIAN_POINT('Ctrl Pts',(33.8237898127121,57.4477100381615,14.1833016967144));
#25287=CARTESIAN_POINT('Ctrl Pts',(33.3490322930752,57.7282855707718,14.2203476602371));
#25288=CARTESIAN_POINT('Ctrl Pts',(32.8742747734382,58.0088611033821,14.2573936237598));
#25289=CARTESIAN_POINT('Ctrl Pts',(32.2466798079601,58.0308235433297,14.2944395872824));
#25290=CARTESIAN_POINT('Ctrl Pts',(31.7534702764192,57.7841214978257,14.3314855508051));
#25291=CARTESIAN_POINT('Ctrl Pts',(31.2602607448784,57.5374194523217,14.3685315143278));
#25292=CARTESIAN_POINT('Ctrl Pts',(30.9014366472749,57.022052921366,14.4055774778505));
#25293=CARTESIAN_POINT('Ctrl Pts',(30.8412156241946,56.4738823989159,14.4426234413732));
#25294=CARTESIAN_POINT('Ctrl Pts',(30.7809946011142,55.9257118764658,14.4796694048958));
#25295=CARTESIAN_POINT('Ctrl Pts',(31.019376652557,55.3447373625211,14.5167153684185));
#25296=CARTESIAN_POINT('Ctrl Pts',(31.4472650020351,54.9968450984029,14.5537613319412));
#25297=CARTESIAN_POINT('Ctrl Pts',(31.5154844642033,54.9413796406974,14.5596676757575));
#25298=CARTESIAN_POINT('Ctrl Pts',(31.5885209558805,54.8918388624727,14.5655740195739));
#25299=CARTESIAN_POINT('Ctrl Pts',(31.6652293984911,54.8484357012869,14.5714803633902));
#25300=CARTESIAN_POINT('Origin',(32.5,56.2916512459885,17.));
#25301=CARTESIAN_POINT('',(31.6679812524744,54.8513129979877,15.2714803633902));
#25302=CARTESIAN_POINT('',(31.6687468960361,54.8490160493388,15.0785196366098));
#25303=CARTESIAN_POINT('',(31.667,54.8488529232836,17.));
#25304=CARTESIAN_POINT('Ctrl Pts',(31.6687468960361,54.8490160493388,15.0785196366098));
#25305=CARTESIAN_POINT('Ctrl Pts',(31.3330220839914,55.0465316965332,15.0525071011481));
#25306=CARTESIAN_POINT('Ctrl Pts',(31.0621374285877,55.3603795470759,15.0264945656864));
#25307=CARTESIAN_POINT('Ctrl Pts',(30.930547953771,55.7245591059458,15.0004820302248));
#25308=CARTESIAN_POINT('Ctrl Pts',(30.7431437350931,56.2432083807723,14.9634360667021));
#25309=CARTESIAN_POINT('Ctrl Pts',(30.8382616710438,56.8639417522836,14.9263901031794));
#25310=CARTESIAN_POINT('Ctrl Pts',(31.1723705294372,57.3026770823852,14.8893441396567));
#25311=CARTESIAN_POINT('Ctrl Pts',(31.5064793878305,57.7414124124868,14.852298176134));
#25312=CARTESIAN_POINT('Ctrl Pts',(32.0795791686666,57.9981497011789,14.8152522126114));
#25313=CARTESIAN_POINT('Ctrl Pts',(32.6293874463964,57.9553916541296,14.7782062490887));
#25314=CARTESIAN_POINT('Ctrl Pts',(33.1791957241261,57.9126336070804,14.741160285566));
#25315=CARTESIAN_POINT('Ctrl Pts',(33.7057124987496,57.5703802242898,14.7041143220433));
#25316=CARTESIAN_POINT('Ctrl Pts',(33.9679745051883,57.0852657438482,14.6670683585206));
#25317=CARTESIAN_POINT('Ctrl Pts',(34.2302365116269,56.6001512634066,14.6300223949979));
#25318=CARTESIAN_POINT('Ctrl Pts',(34.2282437498807,55.972175685314,14.5929764314753));
#25319=CARTESIAN_POINT('Ctrl Pts',(33.9629079737486,55.4887355202075,14.5559304679526));
#25320=CARTESIAN_POINT('Ctrl Pts',(33.6975721976164,55.0052953551011,14.5188845044299));
#25321=CARTESIAN_POINT('Ctrl Pts',(33.1688934070983,54.6663906029808,14.4818385409072));
#25322=CARTESIAN_POINT('Ctrl Pts',(32.6188249386194,54.6271230925477,14.4447925773845));
#25323=CARTESIAN_POINT('Ctrl Pts',(32.2908120993686,54.6037073755496,14.4227015971263));
#25324=CARTESIAN_POINT('Ctrl Pts',(31.9551933282369,54.6868393332485,14.400610616868));
#25325=CARTESIAN_POINT('Ctrl Pts',(31.6674240358463,54.8512520230129,14.3785196366098));
#25326=CARTESIAN_POINT('Ctrl Pts',(31.6652293984911,54.8484357012869,14.5714803633902));
#25327=CARTESIAN_POINT('Ctrl Pts',(32.0696541670855,54.6196041304525,14.6026199830966));
#25328=CARTESIAN_POINT('Ctrl Pts',(32.5761460954187,54.5613764565911,14.6337596028029));
#25329=CARTESIAN_POINT('Ctrl Pts',(33.0168947227899,54.7049585292357,14.6648992225092));
#25330=CARTESIAN_POINT('Ctrl Pts',(33.5412414465535,54.8757742384787,14.7019451860319));
#25331=CARTESIAN_POINT('Ctrl Pts',(33.9725402465673,55.3322156712569,14.7389911495546));
#25332=CARTESIAN_POINT('Ctrl Pts',(34.1134048115911,55.8653898078431,14.7760371130773));
#25333=CARTESIAN_POINT('Ctrl Pts',(34.2542693766149,56.3985639444293,14.8130830766));
#25334=CARTESIAN_POINT('Ctrl Pts',(34.1046997066485,57.0084707848237,14.8501290401226));
#25335=CARTESIAN_POINT('Ctrl Pts',(33.7331471941746,57.415983010017,14.8871750036453));
#25336=CARTESIAN_POINT('Ctrl Pts',(33.3615946817007,57.8234952352103,14.924220967168));
#25337=CARTESIAN_POINT('Ctrl Pts',(32.7680593267191,58.0286128452026,14.9612669306907));
#25338=CARTESIAN_POINT('Ctrl Pts',(32.2241759575529,57.9374626002348,14.9983128942134));
#25339=CARTESIAN_POINT('Ctrl Pts',(31.6802925883866,57.8463123552671,15.0353588577361));
#25340=CARTESIAN_POINT('Ctrl Pts',(31.1860612050356,57.4588942553394,15.0724048212587));
#25341=CARTESIAN_POINT('Ctrl Pts',(30.9676695988056,56.9525123919175,15.1094507847814));
#25342=CARTESIAN_POINT('Ctrl Pts',(30.7492779925756,56.4461305284957,15.1464967483041));
#25343=CARTESIAN_POINT('Ctrl Pts',(30.8067261634667,55.8207849015799,15.1835427118268));
#25344=CARTESIAN_POINT('Ctrl Pts',(31.1137226321993,55.3626684826674,15.2205886753495));
#25345=CARTESIAN_POINT('Ctrl Pts',(31.2543008673673,55.1528901815095,15.237552571363));
#25346=CARTESIAN_POINT('Ctrl Pts',(31.4472058843405,54.9781775023347,15.2545164673766));
#25347=CARTESIAN_POINT('Ctrl Pts',(31.6679812524744,54.8513129979877,15.2714803633902));
#25348=CARTESIAN_POINT('Origin',(32.5,56.2916512459885,17.));
#25349=CARTESIAN_POINT('',(31.668393257303,54.8482192502339,15.9714803633902));
#25350=CARTESIAN_POINT('',(31.6656122060936,54.8464626161314,15.7785196366098));
#25351=CARTESIAN_POINT('',(31.667,54.8488529232836,17.));
#25352=CARTESIAN_POINT('Ctrl Pts',(31.6656122129471,54.8464626279357,15.7785196366098));
#25353=CARTESIAN_POINT('Ctrl Pts',(31.1876990498809,55.1223478631842,15.7414495489509));
#25354=CARTESIAN_POINT('Ctrl Pts',(30.860252864304,55.6587877650758,15.7043794612919));
#25355=CARTESIAN_POINT('Ctrl Pts',(30.8332370510141,56.2099535888295,15.667309373633));
#25356=CARTESIAN_POINT('Ctrl Pts',(30.8062388188308,56.7607607298753,15.6302634101103));
#25357=CARTESIAN_POINT('Ctrl Pts',(31.0792800051602,57.3262745318078,15.5932174465876));
#25358=CARTESIAN_POINT('Ctrl Pts',(31.5274017633055,57.6476843966343,15.556171483065));
#25359=CARTESIAN_POINT('Ctrl Pts',(31.9755235214509,57.9690942614607,15.5191255195423));
#25360=CARTESIAN_POINT('Ctrl Pts',(32.5987258514122,58.0464001891811,15.4820795560196));
#25361=CARTESIAN_POINT('Ctrl Pts',(33.1117966721331,57.8442226833339,15.4450335924969));
#25362=CARTESIAN_POINT('Ctrl Pts',(33.624867492854,57.6420451774866,15.4079876289742));
#25363=CARTESIAN_POINT('Ctrl Pts',(34.0278068043346,57.1603842380718,15.3709416654516));
#25364=CARTESIAN_POINT('Ctrl Pts',(34.1362071477595,56.6196747257879,15.3338957019289));
#25365=CARTESIAN_POINT('Ctrl Pts',(34.2446074911845,56.0789652135039,15.2968497384062));
#25366=CARTESIAN_POINT('Ctrl Pts',(34.0584688665537,55.479207128351,15.2598037748835));
#25367=CARTESIAN_POINT('Ctrl Pts',(33.6629786670948,55.094883157714,15.2227578113608));
#25368=CARTESIAN_POINT('Ctrl Pts',(33.267488467636,54.7105591870771,15.1857118478381));
#25369=CARTESIAN_POINT('Ctrl Pts',(32.662646693349,54.5416693309562,15.1486658843155));
#25370=CARTESIAN_POINT('Ctrl Pts',(32.1252626195522,54.6655069919667,15.1116199207928));
#25371=CARTESIAN_POINT('Ctrl Pts',(31.9652131038813,54.7023896586347,15.1005864927318));
#25372=CARTESIAN_POINT('Ctrl Pts',(31.8111473001584,54.7652381843378,15.0895530646708));
#25373=CARTESIAN_POINT('Ctrl Pts',(31.6687468960361,54.8490160493388,15.0785196366098));
#25374=CARTESIAN_POINT('Ctrl Pts',(31.6679812524744,54.8513129979877,15.2714803633902));
#25375=CARTESIAN_POINT('Ctrl Pts',(31.9293378325702,54.7011292466392,15.2915624308993));
#25376=CARTESIAN_POINT('Ctrl Pts',(32.2297522401559,54.6180004723649,15.3116444984084));
#25377=CARTESIAN_POINT('Ctrl Pts',(32.5286510627353,54.6231330317608,15.3317265659175));
#25378=CARTESIAN_POINT('Ctrl Pts',(33.0800382579645,54.6326012106758,15.3687725294402));
#25379=CARTESIAN_POINT('Ctrl Pts',(33.626267881849,54.942424779415,15.4058184929629));
#25380=CARTESIAN_POINT('Ctrl Pts',(33.917354850155,55.4108112247729,15.4428644564855));
#25381=CARTESIAN_POINT('Ctrl Pts',(34.2084418184611,55.8791976701309,15.4799104200082));
#25382=CARTESIAN_POINT('Ctrl Pts',(34.2443861311887,56.5061469921078,15.5169563835309));
#25383=CARTESIAN_POINT('Ctrl Pts',(34.0087376695652,57.0047322785327,15.5540023470536));
#25384=CARTESIAN_POINT('Ctrl Pts',(33.7730892079418,57.5033175649576,15.5910483105763));
#25385=CARTESIAN_POINT('Ctrl Pts',(33.2658479719673,57.8735388158304,15.6280942740989));
#25386=CARTESIAN_POINT('Ctrl Pts',(32.7191557896563,57.9459621763539,15.6651402376216));
#25387=CARTESIAN_POINT('Ctrl Pts',(32.1724636073452,58.0183855368774,15.7021862011443));
#25388=CARTESIAN_POINT('Ctrl Pts',(31.5863204786975,57.7930110070515,15.739232164667));
#25389=CARTESIAN_POINT('Ctrl Pts',(31.2289781301378,57.3729825184307,15.7762781281897));
#25390=CARTESIAN_POINT('Ctrl Pts',(30.8716357815781,56.9529540298098,15.8133240917123));
#25391=CARTESIAN_POINT('Ctrl Pts',(30.7430942131064,56.3382715823939,15.850370055235));
#25392=CARTESIAN_POINT('Ctrl Pts',(30.9021812024433,55.8102480837199,15.8874160187577));
#25393=CARTESIAN_POINT('Ctrl Pts',(31.022514091882,55.4108527997199,15.9154374669685));
#25394=CARTESIAN_POINT('Ctrl Pts',(31.3074096675184,55.0610382301548,15.9434589151794));
#25395=CARTESIAN_POINT('Ctrl Pts',(31.668393257303,54.8482192502339,15.9714803633902));
#25396=CARTESIAN_POINT('Origin',(32.5,56.2916512459885,17.));
#25397=CARTESIAN_POINT('',(31.6652521719754,54.8469263020216,16.6714803633902));
#25398=CARTESIAN_POINT('',(31.6662812667712,54.8504621893828,16.4785196366098));
#25399=CARTESIAN_POINT('',(31.667,54.8488529232836,17.));
#25400=CARTESIAN_POINT('Ctrl Pts',(31.6662812667712,54.8504621893828,16.4785196366098));
#25401=CARTESIAN_POINT('Ctrl Pts',(31.5218969898699,54.9322586741207,16.4674379602763));
#25402=CARTESIAN_POINT('Ctrl Pts',(31.3899082837209,55.0347971411717,16.4563562839428));
#25403=CARTESIAN_POINT('Ctrl Pts',(31.2776094808925,55.1556342327712,16.4452746076093));
#25404=CARTESIAN_POINT('Ctrl Pts',(30.9021953983998,55.5595917526322,16.4082286440866));
#25405=CARTESIAN_POINT('Ctrl Pts',(30.7468278084228,56.1680473893291,16.3711826805639));
#25406=CARTESIAN_POINT('Ctrl Pts',(30.882611569505,56.7025379705484,16.3341367170413));
#25407=CARTESIAN_POINT('Ctrl Pts',(31.0183953305873,57.2370285517677,16.2970907535186));
#25408=CARTESIAN_POINT('Ctrl Pts',(31.4453304427286,57.6975540775093,16.2600447899959));
#25409=CARTESIAN_POINT('Ctrl Pts',(31.9680276309783,57.8733524295625,16.2229988264732));
#25410=CARTESIAN_POINT('Ctrl Pts',(32.490724819228,58.0491507816157,16.1859528629505));
#25411=CARTESIAN_POINT('Ctrl Pts',(33.109184083586,57.9402219599804,16.1489068994279));
#25412=CARTESIAN_POINT('Ctrl Pts',(33.5403640348015,57.5964178575421,16.1118609359052));
#25413=CARTESIAN_POINT('Ctrl Pts',(33.971543986017,57.2526137551037,16.0748149723825));
#25414=CARTESIAN_POINT('Ctrl Pts',(34.2154446240901,56.6739343718623,16.0377690088598));
#25415=CARTESIAN_POINT('Ctrl Pts',(34.1604434390255,56.1252156089025,16.0007230453371));
#25416=CARTESIAN_POINT('Ctrl Pts',(34.1054422539609,55.5764968459426,15.9636770818144));
#25417=CARTESIAN_POINT('Ctrl Pts',(33.7515392457586,55.0577387032643,15.9266311182918));
#25418=CARTESIAN_POINT('Ctrl Pts',(33.2607001328297,54.8063537864051,15.8895851547691));
#25419=CARTESIAN_POINT('Ctrl Pts',(32.7701806517449,54.5551325700793,15.8525633153827));
#25420=CARTESIAN_POINT('Ctrl Pts',(32.1429033520047,54.5709364688817,15.8155414759962));
#25421=CARTESIAN_POINT('Ctrl Pts',(31.6656122129471,54.8464626279357,15.7785196366098));
#25422=CARTESIAN_POINT('Ctrl Pts',(31.668393257303,54.8482192502339,15.9714803633902));
#25423=CARTESIAN_POINT('Ctrl Pts',(31.7846507008451,54.7796793186609,15.980504878702));
#25424=CARTESIAN_POINT('Ctrl Pts',(31.9088000679097,54.7253487041335,15.9895293940139));
#25425=CARTESIAN_POINT('Ctrl Pts',(32.0378859406647,54.688147422912,15.9985539093257));
#25426=CARTESIAN_POINT('Ctrl Pts',(32.5677881424037,54.5354348107102,16.0355998728484));
#25427=CARTESIAN_POINT('Ctrl Pts',(33.180876998736,54.6713741362387,16.0726458363711));
#25428=CARTESIAN_POINT('Ctrl Pts',(33.5965689181183,55.0337519963386,16.1096917998938));
#25429=CARTESIAN_POINT('Ctrl Pts',(34.0122608375006,55.3961298564385,16.1467377634165));
#25430=CARTESIAN_POINT('Ctrl Pts',(34.2305558199328,55.9849462511098,16.1837837269391));
#25431=CARTESIAN_POINT('Ctrl Pts',(34.1515499288845,56.5307260185163,16.2208296904618));
#25432=CARTESIAN_POINT('Ctrl Pts',(34.0725440378362,57.0765057859228,16.2578756539845));
#25433=CARTESIAN_POINT('Ctrl Pts',(33.6962372733073,57.5792489260645,16.2949216175072));
#25434=CARTESIAN_POINT('Ctrl Pts',(33.1948485598908,57.8088721901076,16.3319675810299));
#25435=CARTESIAN_POINT('Ctrl Pts',(32.6934598464743,58.0384954541506,16.3690135445526));
#25436=CARTESIAN_POINT('Ctrl Pts',(32.0669891841703,57.9949988420949,16.4060595080752));
#25437=CARTESIAN_POINT('Ctrl Pts',(31.6021444239114,57.6982888250906,16.4431054715979));
#25438=CARTESIAN_POINT('Ctrl Pts',(31.1372996636525,57.4015788080863,16.4801514351206));
#25439=CARTESIAN_POINT('Ctrl Pts',(30.8340808054388,56.8516553861335,16.5171973986433));
#25440=CARTESIAN_POINT('Ctrl Pts',(30.8312576791002,56.3001941315665,16.554243362166));
#25441=CARTESIAN_POINT('Ctrl Pts',(30.8284345527615,55.7487328769996,16.5912893256886));
#25442=CARTESIAN_POINT('Ctrl Pts',(31.1260071582979,55.1957337898185,16.6283352892113));
#25443=CARTESIAN_POINT('Ctrl Pts',(31.5877897054339,54.8942800379899,16.665381252734));
#25444=CARTESIAN_POINT('Ctrl Pts',(31.6131317633018,54.8777366270907,16.6674142896194));
#25445=CARTESIAN_POINT('Ctrl Pts',(31.6389683688547,54.8619507900759,16.6694473265048));
#25446=CARTESIAN_POINT('Ctrl Pts',(31.6652521719754,54.8469263020216,16.6714803633902));
#25447=CARTESIAN_POINT('Origin',(32.5,56.2916512459885,17.));
#25448=CARTESIAN_POINT('',(31.6668674827448,54.8509763286063,17.3714803633902));
#25449=CARTESIAN_POINT('',(31.6688688935777,54.8504049148726,17.1785196366098));
#25450=CARTESIAN_POINT('',(31.667,54.8488529232836,17.));
#25451=CARTESIAN_POINT('Ctrl Pts',(31.6688688935777,54.8504049148726,17.1785196366098));
#25452=CARTESIAN_POINT('Ctrl Pts',(31.3819874737691,55.0177923404708,17.156380408079));
#25453=CARTESIAN_POINT('Ctrl Pts',(31.1417740021656,55.2676351144427,17.1342411795483));
#25454=CARTESIAN_POINT('Ctrl Pts',(30.9981174968784,55.5642433945469,17.1121019510175));
#25455=CARTESIAN_POINT('Ctrl Pts',(30.7577345202416,56.0605632870855,17.0750559874949));
#25456=CARTESIAN_POINT('Ctrl Pts',(30.7877102970592,56.6878262324661,17.0380100239722));
#25457=CARTESIAN_POINT('Ctrl Pts',(31.0743262430964,57.1589617869125,17.0009640604495));
#25458=CARTESIAN_POINT('Ctrl Pts',(31.3609421891337,57.6300973413589,16.9639180969268));
#25459=CARTESIAN_POINT('Ctrl Pts',(31.9041983043906,57.9451055048711,16.9268721334042));
#25460=CARTESIAN_POINT('Ctrl Pts',(32.4554703472483,57.9598210051999,16.8898261698815));
#25461=CARTESIAN_POINT('Ctrl Pts',(33.0067423901059,57.9745365055287,16.8527802063588));
#25462=CARTESIAN_POINT('Ctrl Pts',(33.5660303605644,57.6889593426742,16.8157342428361));
#25463=CARTESIAN_POINT('Ctrl Pts',(33.8773729475645,57.2337855245493,16.7786882793134));
#25464=CARTESIAN_POINT('Ctrl Pts',(34.1887155345647,56.7786117064244,16.7416423157907));
#25465=CARTESIAN_POINT('Ctrl Pts',(34.2521127381065,56.1538412330292,16.7045963522681));
#25466=CARTESIAN_POINT('Ctrl Pts',(34.0385504685031,55.6454038542026,16.6675503887454));
#25467=CARTESIAN_POINT('Ctrl Pts',(33.8249881988996,55.1369664753759,16.6305044252227));
#25468=CARTESIAN_POINT('Ctrl Pts',(33.3344664561508,54.7448621911179,16.5934584617));
#25469=CARTESIAN_POINT('Ctrl Pts',(32.7914752972722,54.6485397505015,16.5564124981773));
#25470=CARTESIAN_POINT('Ctrl Pts',(32.4109108025283,54.5810305464448,16.5304482109881));
#25471=CARTESIAN_POINT('Ctrl Pts',(32.0045725792269,54.658813619538,16.504483923799));
#25472=CARTESIAN_POINT('Ctrl Pts',(31.6662812667712,54.8504621893828,16.4785196366098));
#25473=CARTESIAN_POINT('Ctrl Pts',(31.6652521719754,54.8469263020216,16.6714803633902));
#25474=CARTESIAN_POINT('Ctrl Pts',(32.1179113819592,54.5881748244737,16.7064932900275));
#25475=CARTESIAN_POINT('Ctrl Pts',(32.7032079137753,54.5552369344614,16.7415062166648));
#25476=CARTESIAN_POINT('Ctrl Pts',(33.1792781595522,54.7673956583618,16.776519143302));
#25477=CARTESIAN_POINT('Ctrl Pts',(33.6829915777989,54.9918734470384,16.8135651068247));
#25478=CARTESIAN_POINT('Ctrl Pts',(34.0644259255566,55.4907374408677,16.8506110703474));
#25479=CARTESIAN_POINT('Ctrl Pts',(34.1490156106942,56.0356797043225,16.8876570338701));
#25480=CARTESIAN_POINT('Ctrl Pts',(34.2336052958317,56.5806219677773,16.9247029973928));
#25481=CARTESIAN_POINT('Ctrl Pts',(34.0213503183491,57.1716425008576,16.9617489609154));
#25482=CARTESIAN_POINT('Ctrl Pts',(33.6093903722588,57.5382574052848,16.9987949244381));
#25483=CARTESIAN_POINT('Ctrl Pts',(33.1974304261685,57.904872309712,17.0358408879608));
#25484=CARTESIAN_POINT('Ctrl Pts',(32.5857655114706,58.0470815854862,17.0728868514835));
#25485=CARTESIAN_POINT('Ctrl Pts',(32.0543275447524,57.8998023511679,17.1099328150062));
#25486=CARTESIAN_POINT('Ctrl Pts',(31.5228895780343,57.7525231168495,17.1469787785289));
#25487=CARTESIAN_POINT('Ctrl Pts',(31.071678559296,57.3157553724386,17.1840247420515));
#25488=CARTESIAN_POINT('Ctrl Pts',(30.9071937698036,56.7893883528063,17.2210707055742));
#25489=CARTESIAN_POINT('Ctrl Pts',(30.7427089803112,56.263021333174,17.2581166690969));
#25490=CARTESIAN_POINT('Ctrl Pts',(30.8649504200646,55.6470550383205,17.2951626326196));
#25491=CARTESIAN_POINT('Ctrl Pts',(31.2179736010047,55.2233899358517,17.3322085961422));
#25492=CARTESIAN_POINT('Ctrl Pts',(31.3427181334424,55.073683321751,17.3452991852249));
#25493=CARTESIAN_POINT('Ctrl Pts',(31.4962789539492,54.9479881676876,17.3583897743076));
#25494=CARTESIAN_POINT('Ctrl Pts',(31.6668674827448,54.8509763286063,17.3714803633902));
#25495=CARTESIAN_POINT('Origin',(32.5,56.2916512459885,17.));
#25496=CARTESIAN_POINT('',(31.6688993943412,54.8497298728322,18.0714803633902));
#25497=CARTESIAN_POINT('',(31.6668239490614,54.8465985185332,17.8785196366098));
#25498=CARTESIAN_POINT('',(31.667,54.8488529232836,17.));
#25499=CARTESIAN_POINT('Ctrl Pts',(31.6668239490614,54.8465985185332,17.8785196366098));
#25500=CARTESIAN_POINT('Ctrl Pts',(31.2400871420202,55.0969461017405,17.8453228558818));
#25501=CARTESIAN_POINT('Ctrl Pts',(30.9262488413014,55.5484932725246,17.8121260751538));
#25502=CARTESIAN_POINT('Ctrl Pts',(30.8508004340577,56.036868932597,17.7789292944258));
#25503=CARTESIAN_POINT('Ctrl Pts',(30.7666037474724,56.5818719868586,17.7418833309031));
#25504=CARTESIAN_POINT('Ctrl Pts',(30.9792848378897,57.1727392338966,17.7048373673804));
#25505=CARTESIAN_POINT('Ctrl Pts',(31.3915089982964,57.539056927659,17.6677914038578));
#25506=CARTESIAN_POINT('Ctrl Pts',(31.8037331587031,57.9053746214214,17.6307454403351));
#25507=CARTESIAN_POINT('Ctrl Pts',(32.4155003890991,58.0471427619081,17.5936994768124));
#25508=CARTESIAN_POINT('Ctrl Pts',(32.9468319475375,57.8994803557454,17.5566535132897));
#25509=CARTESIAN_POINT('Ctrl Pts',(33.4781635059759,57.7518179495826,17.519607549767));
#25510=CARTESIAN_POINT('Ctrl Pts',(33.9290593924568,57.3147249967705,17.4825615862444));
#25511=CARTESIAN_POINT('Ctrl Pts',(34.0931645477785,56.788239565649,17.4455156227217));
#25512=CARTESIAN_POINT('Ctrl Pts',(34.2572697031003,56.2617541345275,17.408469659199));
#25513=CARTESIAN_POINT('Ctrl Pts',(34.134584127263,55.6458762250967,17.3714236956763));
#25514=CARTESIAN_POINT('Ctrl Pts',(33.7812555697231,55.2224658548728,17.3343777321536));
#25515=CARTESIAN_POINT('Ctrl Pts',(33.4279270121832,54.799055484649,17.2973317686309));
#25516=CARTESIAN_POINT('Ctrl Pts',(32.8439554729406,54.568112653632,17.2602858051083));
#25517=CARTESIAN_POINT('Ctrl Pts',(32.2965988382737,54.6353296579719,17.2232398415856));
#25518=CARTESIAN_POINT('Ctrl Pts',(32.0763508133016,54.6623767631182,17.2083331065936));
#25519=CARTESIAN_POINT('Ctrl Pts',(31.8620312385645,54.7376999942423,17.1934263716017));
#25520=CARTESIAN_POINT('Ctrl Pts',(31.6688688935777,54.8504049148726,17.1785196366098));
#25521=CARTESIAN_POINT('Ctrl Pts',(31.6668674827448,54.8509763286063,17.3714803633902));
#25522=CARTESIAN_POINT('Ctrl Pts',(31.9790392312177,54.6734476539505,17.3954357378302));
#25523=CARTESIAN_POINT('Ctrl Pts',(32.3482331506335,54.5919732963168,17.4193911122703));
#25524=CARTESIAN_POINT('Ctrl Pts',(32.7022067343745,54.6351832109726,17.4433464867103));
#25525=CARTESIAN_POINT('Ctrl Pts',(33.2496117646775,54.702005498646,17.480392450233));
#25526=CARTESIAN_POINT('Ctrl Pts',(33.7606169031567,55.0670139840769,17.5174384137557));
#25527=CARTESIAN_POINT('Ctrl Pts',(34.001357750591,55.5631604641687,17.5544843772783));
#25528=CARTESIAN_POINT('Ctrl Pts',(34.2420985980252,56.0593069442606,17.591530340801));
#25529=CARTESIAN_POINT('Ctrl Pts',(34.2125751544145,56.6865914190135,17.6285763043237));
#25530=CARTESIAN_POINT('Ctrl Pts',(33.9262989911366,57.1579335916119,17.6656222678464));
#25531=CARTESIAN_POINT('Ctrl Pts',(33.6400228278586,57.6292757642103,17.7026682313691));
#25532=CARTESIAN_POINT('Ctrl Pts',(33.0969939449135,57.9446756346541,17.7397141948917));
#25533=CARTESIAN_POINT('Ctrl Pts',(32.5457325897642,57.959788663796,17.7767601584144));
#25534=CARTESIAN_POINT('Ctrl Pts',(31.9944712346149,57.9749016929378,17.8138061219371));
#25535=CARTESIAN_POINT('Ctrl Pts',(31.4349774072613,57.6897278807776,17.8508520854598));
#25536=CARTESIAN_POINT('Ctrl Pts',(31.1233066303378,57.2347786394959,17.8878980489825));
#25537=CARTESIAN_POINT('Ctrl Pts',(30.8116358534142,56.7798293982142,17.9249440125051));
#25538=CARTESIAN_POINT('Ctrl Pts',(30.7477881269206,56.1551047278111,17.9619899760278));
#25539=CARTESIAN_POINT('Ctrl Pts',(30.960983724928,55.6465134161264,17.9990359395505));
#25540=CARTESIAN_POINT('Ctrl Pts',(31.0999537214239,55.3149918769234,18.0231840808304));
#25541=CARTESIAN_POINT('Ctrl Pts',(31.3566391271215,55.0328152763439,18.0473322221103));
#25542=CARTESIAN_POINT('Ctrl Pts',(31.6688993943412,54.8497298728322,18.0714803633902));
#25543=CARTESIAN_POINT('Origin',(32.5,56.2916512459885,17.));
#25544=CARTESIAN_POINT('',(31.6661431441558,54.8463676572785,18.7714803633902));
#25545=CARTESIAN_POINT('',(31.6653993953823,54.8489980951737,18.5785196366098));
#25546=CARTESIAN_POINT('',(31.667,54.8488529232836,17.));
#25547=CARTESIAN_POINT('Ctrl Pts',(31.6653993953823,54.8489980951737,18.5785196366098));
#25548=CARTESIAN_POINT('Ctrl Pts',(31.5716723835922,54.901972129835,18.5713112672072));
#25549=CARTESIAN_POINT('Ctrl Pts',(31.4833584827506,54.9639737793168,18.5641028978047));
#25550=CARTESIAN_POINT('Ctrl Pts',(31.4025244101712,55.0345432294477,18.5568945284021));
#25551=CARTESIAN_POINT('Ctrl Pts',(30.9870939657909,55.3972207129895,18.5198485648794));
#25552=CARTESIAN_POINT('Ctrl Pts',(30.7692236712863,55.9861942986586,18.4828026013567));
#25553=CARTESIAN_POINT('Ctrl Pts',(30.8486231023463,56.5319168852662,18.445756637834));
#25554=CARTESIAN_POINT('Ctrl Pts',(30.9280225334064,57.0776394718738,18.4087106743114));
#25555=CARTESIAN_POINT('Ctrl Pts',(31.3046916900312,57.5801110594199,18.3716647107887));
#25556=CARTESIAN_POINT('Ctrl Pts',(31.8062457968318,57.8093726766562,18.334618747266));
#25557=CARTESIAN_POINT('Ctrl Pts',(32.3077999036324,58.0386342938926,18.2975727837433));
#25558=CARTESIAN_POINT('Ctrl Pts',(32.9342389606089,57.9946859408193,18.2605268202206));
#25559=CARTESIAN_POINT('Ctrl Pts',(33.3988695811848,57.6976408304244,18.223480856698));
#25560=CARTESIAN_POINT('Ctrl Pts',(33.8635002017608,57.4005957200295,18.1864348931753));
#25561=CARTESIAN_POINT('Ctrl Pts',(34.1663223859364,56.8504538523131,18.1493889296526));
#25562=CARTESIAN_POINT('Ctrl Pts',(34.168747844005,56.298990772552,18.1123429661299));
#25563=CARTESIAN_POINT('Ctrl Pts',(34.1711733020736,55.747527692791,18.0752970026072));
#25564=CARTESIAN_POINT('Ctrl Pts',(33.8732020340353,55.1947434009854,18.0382510390846));
#25565=CARTESIAN_POINT('Ctrl Pts',(33.4112022803197,54.8936227627802,18.0012050755619));
#25566=CARTESIAN_POINT('Ctrl Pts',(32.9492025266042,54.5925021245749,17.9641591120392));
#25567=CARTESIAN_POINT('Ctrl Pts',(32.3231742872114,54.5430451399701,17.9271131485165));
#25568=CARTESIAN_POINT('Ctrl Pts',(31.8196229357211,54.7678860784103,17.8900671849938));
#25569=CARTESIAN_POINT('Ctrl Pts',(31.7673024933817,54.791247702444,17.8862180021992));
#25570=CARTESIAN_POINT('Ctrl Pts',(31.7163042884046,54.8175705950767,17.8823688194045));
#25571=CARTESIAN_POINT('Ctrl Pts',(31.6668239490614,54.8465985185332,17.8785196366098));
#25572=CARTESIAN_POINT('Ctrl Pts',(31.6688993943412,54.8497298728322,18.0714803633902));
#25573=CARTESIAN_POINT('Ctrl Pts',(31.8356814821797,54.751941684401,18.084378185633));
#25574=CARTESIAN_POINT('Ctrl Pts',(32.0183177486645,54.6824218442404,18.0972760078758));
#25575=CARTESIAN_POINT('Ctrl Pts',(32.2073398697232,54.6487501647903,18.1101738301185));
#25576=CARTESIAN_POINT('Ctrl Pts',(32.7502614940028,54.5520361781053,18.1472197936412));
#25577=CARTESIAN_POINT('Ctrl Pts',(33.3458658200538,54.7510661577016,18.1842657571639));
#25578=CARTESIAN_POINT('Ctrl Pts',(33.7215711507525,55.1547529048404,18.2213117206866));
#25579=CARTESIAN_POINT('Ctrl Pts',(34.0972764814512,55.5584396519791,18.2583576842093));
#25580=CARTESIAN_POINT('Ctrl Pts',(34.2530828167975,56.1667831666603,18.2954036477319));
#25581=CARTESIAN_POINT('Ctrl Pts',(34.1176845039388,56.7013715898475,18.3324496112546));
#25582=CARTESIAN_POINT('Ctrl Pts',(33.98228619108,57.2359600130348,18.3694955747773));
#25583=CARTESIAN_POINT('Ctrl Pts',(33.5556832300161,57.696793344728,18.4065415383));
#25584=CARTESIAN_POINT('Ctrl Pts',(33.0331128848803,57.8729685975756,18.4435875018227));
#25585=CARTESIAN_POINT('Ctrl Pts',(32.5105425397446,58.0491438504232,18.4806334653453));
#25586=CARTESIAN_POINT('Ctrl Pts',(31.892004810537,57.940661024425,18.517679428868));
#25587=CARTESIAN_POINT('Ctrl Pts',(31.4605769963787,57.5971679000379,18.5547253923907));
#25588=CARTESIAN_POINT('Ctrl Pts',(31.0291491822204,57.2536747756508,18.5917713559134));
#25589=CARTESIAN_POINT('Ctrl Pts',(30.7848312831113,56.6751713528746,18.6288173194361));
#25590=CARTESIAN_POINT('Ctrl Pts',(30.839436770952,56.1264130034822,18.6658632829588));
#25591=CARTESIAN_POINT('Ctrl Pts',(30.89132971378,55.6049143999997,18.7010689764359));
#25592=CARTESIAN_POINT('Ctrl Pts',(31.2131854490111,55.1102790779514,18.736274669913));
#25593=CARTESIAN_POINT('Ctrl Pts',(31.6661431441558,54.8463676572785,18.7714803633902));
#25594=CARTESIAN_POINT('Origin',(32.5,56.2916512459885,17.));
#25595=CARTESIAN_POINT('',(31.6657991298123,54.8498167632728,19.4714803633902));
#25596=CARTESIAN_POINT('',(31.6682947036337,54.8512220664372,19.2785196366098));
#25597=CARTESIAN_POINT('',(31.667,54.8488529232836,17.));
#25598=CARTESIAN_POINT('Ctrl Pts',(31.6682947036337,54.8512220664372,19.2785196366098));
#25599=CARTESIAN_POINT('Ctrl Pts',(31.4307799124075,54.9882439463791,19.26025371501));
#25600=CARTESIAN_POINT('Ctrl Pts',(31.2253675580441,55.1807871169989,19.2419877934101));
#25601=CARTESIAN_POINT('Ctrl Pts',(31.0820105037967,55.4118336375308,19.2237218718103));
#25602=CARTESIAN_POINT('Ctrl Pts',(30.7912614072705,55.8804298112795,19.1866759082877));
#25603=CARTESIAN_POINT('Ctrl Pts',(30.7557692111823,56.5074048138577,19.149629944765));
#25604=CARTESIAN_POINT('Ctrl Pts',(30.9917771203569,57.0058199801505,19.1125839812423));
#25605=CARTESIAN_POINT('Ctrl Pts',(31.2277850295315,57.5042351464433,19.0755380177196));
#25606=CARTESIAN_POINT('Ctrl Pts',(31.7352930439689,57.8740904764507,19.0384920541969));
#25607=CARTESIAN_POINT('Ctrl Pts',(32.2820372430805,57.9461195811699,19.0014460906743));
#25608=CARTESIAN_POINT('Ctrl Pts',(32.828781442192,58.0181486858891,18.9644001271516));
#25609=CARTESIAN_POINT('Ctrl Pts',(33.4147618259776,57.7923515653202,18.9273541636289));
#25610=CARTESIAN_POINT('Ctrl Pts',(33.7718011490706,57.3720655520495,18.8903082001062));
#25611=CARTESIAN_POINT('Ctrl Pts',(34.1288404721637,56.9517795387787,18.8532622365835));
#25612=CARTESIAN_POINT('Ctrl Pts',(34.2569387345642,56.3370046328063,18.8162162730609));
#25613=CARTESIAN_POINT('Ctrl Pts',(34.0974710401143,55.8090960558605,18.7791703095382));
#25614=CARTESIAN_POINT('Ctrl Pts',(33.9380033456643,55.2811874789147,18.7421243460155));
#25615=CARTESIAN_POINT('Ctrl Pts',(33.4909696943638,54.8401452309957,18.7050783824928));
#25616=CARTESIAN_POINT('Ctrl Pts',(32.9609575715857,54.6878147977434,18.6680324189701));
#25617=CARTESIAN_POINT('Ctrl Pts',(32.5340747186531,54.565124679649,18.63819482485));
#25618=CARTESIAN_POINT('Ctrl Pts',(32.0533634937381,54.6297227421977,18.6083572307299));
#25619=CARTESIAN_POINT('Ctrl Pts',(31.6653993953823,54.8489980951737,18.5785196366098));
#25620=CARTESIAN_POINT('Ctrl Pts',(31.6661431441558,54.8463676572785,18.7714803633902));
#25621=CARTESIAN_POINT('Ctrl Pts',(31.6898201235287,54.832572494219,18.7733206334357));
#25622=CARTESIAN_POINT('Ctrl Pts',(31.7138553201483,54.819407751031,18.7751609034813));
#25623=CARTESIAN_POINT('Ctrl Pts',(31.7382289011373,54.8069025442232,18.7770011735268));
#25624=CARTESIAN_POINT('Ctrl Pts',(32.2288866686916,54.5551637103656,18.8140471370495));
#25625=CARTESIAN_POINT('Ctrl Pts',(32.8566733290096,54.5706993186593,18.8510931005722));
#25626=CARTESIAN_POINT('Ctrl Pts',(33.3342787571905,54.8463994098823,18.8881390640948));
#25627=CARTESIAN_POINT('Ctrl Pts',(33.8118841853713,55.1220995011053,18.9251850276175));
#25628=CARTESIAN_POINT('Ctrl Pts',(34.1393083814151,55.6579640752576,18.9622309911402));
#25629=CARTESIAN_POINT('Ctrl Pts',(34.1667038054086,56.2087516714065,18.9992769546629));
#25630=CARTESIAN_POINT('Ctrl Pts',(34.1940992294022,56.7595392675554,19.0363229181855));
#25631=CARTESIAN_POINT('Ctrl Pts',(33.9214658813456,57.325249885701,19.0733688817082));
#25632=CARTESIAN_POINT('Ctrl Pts',(33.4735759588574,57.6469828536777,19.1104148452309));
#25633=CARTESIAN_POINT('Ctrl Pts',(33.0256860363692,57.9687158216544,19.1474608087536));
#25634=CARTESIAN_POINT('Ctrl Pts',(32.4025395394495,58.0464711394622,19.1845067722763));
#25635=CARTESIAN_POINT('Ctrl Pts',(31.889322996006,57.8446636449513,19.221552735799));
#25636=CARTESIAN_POINT('Ctrl Pts',(31.3761064525625,57.6428561504404,19.2585986993216));
#25637=CARTESIAN_POINT('Ctrl Pts',(30.9728198625952,57.1614858436107,19.2956446628443));
#25638=CARTESIAN_POINT('Ctrl Pts',(30.86402962057,56.6208545750433,19.332690626367));
#25639=CARTESIAN_POINT('Ctrl Pts',(30.7552393785448,56.0802233064759,19.3697365898897));
#25640=CARTESIAN_POINT('Ctrl Pts',(30.9409454844617,55.4803310761708,19.4067825534124));
#25641=CARTESIAN_POINT('Ctrl Pts',(31.3361584863692,55.0957219647369,19.443828516935));
#25642=CARTESIAN_POINT('Ctrl Pts',(31.4344901101744,55.000028659418,19.4530457990868));
#25643=CARTESIAN_POINT('Ctrl Pts',(31.5457912060088,54.917662401762,19.4622630812385));
#25644=CARTESIAN_POINT('Ctrl Pts',(31.6657991298123,54.8498167632728,19.4714803633902));
#25645=CARTESIAN_POINT('Origin',(32.5,56.2916512459885,17.));
#25646=CARTESIAN_POINT('',(31.6686691446489,54.8508917236136,20.1714803633902));
#25647=CARTESIAN_POINT('',(31.6680707239275,54.8477242132621,19.9785196366098));
#25648=CARTESIAN_POINT('',(31.667,54.8488529232836,17.));
#25649=CARTESIAN_POINT('Ctrl Pts',(31.6680707239275,54.8477242132621,19.9785196366098));
#25650=CARTESIAN_POINT('Ctrl Pts',(31.2906837721071,55.0702773030723,19.9491961628127));
#25651=CARTESIAN_POINT('Ctrl Pts',(30.9974844080691,55.4444429123815,19.9198726890157));
#25652=CARTESIAN_POINT('Ctrl Pts',(30.8862884172365,55.8665534203839,19.8905492152186));
#25653=CARTESIAN_POINT('Ctrl Pts',(30.7458083824097,56.3998289316761,19.8535032516959));
#25654=CARTESIAN_POINT('Ctrl Pts',(30.8958178157836,57.0096276847031,19.8164572881732));
#25655=CARTESIAN_POINT('Ctrl Pts',(31.2676640515259,57.4168718226721,19.7794113246505));
#25656=CARTESIAN_POINT('Ctrl Pts',(31.6395102872682,57.8241159606411,19.7423653611279));
#25657=CARTESIAN_POINT('Ctrl Pts',(32.2331933253789,58.0288054835523,19.7053193976052));
#25658=CARTESIAN_POINT('Ctrl Pts',(32.7770107560741,57.9372630704146,19.6682734340825));
#25659=CARTESIAN_POINT('Ctrl Pts',(33.3208281867694,57.8457206572769,19.6312274705598));
#25660=CARTESIAN_POINT('Ctrl Pts',(33.8147800100492,57.4579463080904,19.5941815070371));
#25661=CARTESIAN_POINT('Ctrl Pts',(34.0328063735823,56.9514071526715,19.5571355435145));
#25662=CARTESIAN_POINT('Ctrl Pts',(34.2508327371153,56.4448679972525,19.5200895799918));
#25663=CARTESIAN_POINT('Ctrl Pts',(34.1929336409016,55.8195640356011,19.4830436164691));
#25664=CARTESIAN_POINT('Ctrl Pts',(33.8856069343887,55.3616691714411,19.4459976529464));
#25665=CARTESIAN_POINT('Ctrl Pts',(33.5782802278758,54.9037743072811,19.4089516894237));
#25666=CARTESIAN_POINT('Ctrl Pts',(33.0215259110637,54.6132885406125,19.3719057259011));
#25667=CARTESIAN_POINT('Ctrl Pts',(32.4701457541755,54.6231543297377,19.3348597623784));
#25668=CARTESIAN_POINT('Ctrl Pts',(32.1906296753062,54.6281556825372,19.3160797204555));
#25669=CARTESIAN_POINT('Ctrl Pts',(31.9124946862161,54.7103435109481,19.2972996785326));
#25670=CARTESIAN_POINT('Ctrl Pts',(31.6682947036337,54.8512220664372,19.2785196366098));
#25671=CARTESIAN_POINT('Ctrl Pts',(31.6657991298123,54.8498167632728,19.4714803633902));
#25672=CARTESIAN_POINT('Ctrl Pts',(32.0281252709183,54.6449782192373,19.4993090447612));
#25673=CARTESIAN_POINT('Ctrl Pts',(32.46981831913,54.5725020736119,19.5271377261321));
#25674=CARTESIAN_POINT('Ctrl Pts',(32.8735646889017,54.6652369881102,19.5549664075031));
#25675=CARTESIAN_POINT('Ctrl Pts',(33.4110379916282,54.7886871154801,19.5920123710258));
#25676=CARTESIAN_POINT('Ctrl Pts',(33.8812646991831,55.2049133627827,19.6290583345484));
#25677=CARTESIAN_POINT('Ctrl Pts',(34.069042894277,55.7234274269329,19.6661042980711));
#25678=CARTESIAN_POINT('Ctrl Pts',(34.2568210893708,56.2419414910831,19.7031502615938));
#25679=CARTESIAN_POINT('Ctrl Pts',(34.1621507720038,56.8627433720808,19.7401962251165));
#25680=CARTESIAN_POINT('Ctrl Pts',(33.8283583461529,57.3017195705904,19.7772421886392));
#25681=CARTESIAN_POINT('Ctrl Pts',(33.494565920302,57.7406957691,19.8142881521619));
#25682=CARTESIAN_POINT('Ctrl Pts',(32.9216513859673,57.9978462851214,19.8513341156845));
#25683=CARTESIAN_POINT('Ctrl Pts',(32.3718123356058,57.9554847234739,19.8883800792072));
#25684=CARTESIAN_POINT('Ctrl Pts',(31.8219732852442,57.9131231618264,19.9254260427299));
#25685=CARTESIAN_POINT('Ctrl Pts',(31.2952097188558,57.5712495225101,19.9624720062526));
#25686=CARTESIAN_POINT('Ctrl Pts',(31.0325979551939,57.086324221881,19.9995179697753));
#25687=CARTESIAN_POINT('Ctrl Pts',(30.769986191532,56.601398921252,20.0365639332979));
#25688=CARTESIAN_POINT('Ctrl Pts',(30.7715262305966,55.9734219593102,20.0736098968206));
#25689=CARTESIAN_POINT('Ctrl Pts',(31.0365132935154,55.489790540013,20.1106558603433));
#25690=CARTESIAN_POINT('Ctrl Pts',(31.1815376981853,55.225104566703,20.1309306946923));
#25691=CARTESIAN_POINT('Ctrl Pts',(31.4054710295806,55.0036536684416,20.1512055290412));
#25692=CARTESIAN_POINT('Ctrl Pts',(31.6686691446489,54.8508917236136,20.1714803633902));
#25693=CARTESIAN_POINT('Origin',(32.5,56.2916512459885,17.));
#25694=CARTESIAN_POINT('',(31.6674621971265,54.8470528177236,20.8714803633902));
#25695=CARTESIAN_POINT('',(31.6651488727496,54.8473747039336,20.6785196366098));
#25696=CARTESIAN_POINT('',(31.667,54.8488529232836,17.));
#25697=CARTESIAN_POINT('Ctrl Pts',(31.6651488727496,54.8473747039336,20.6785196366098));
#25698=CARTESIAN_POINT('Ctrl Pts',(31.6219590933013,54.8719481703147,20.6751845741382));
#25699=CARTESIAN_POINT('Ctrl Pts',(31.579962486587,54.8985363635017,20.6718495116665));
#25700=CARTESIAN_POINT('Ctrl Pts',(31.539367364925,54.9271153018697,20.6685144491949));
#25701=CARTESIAN_POINT('Ctrl Pts',(31.0884356630212,55.2445709169594,20.6314684856722));
#25702=CARTESIAN_POINT('Ctrl Pts',(30.8104307642169,55.8076611175674,20.5944225221495));
#25703=CARTESIAN_POINT('Ctrl Pts',(30.8325829345476,56.3586844387663,20.5573765586268));
#25704=CARTESIAN_POINT('Ctrl Pts',(30.8547351048784,56.9097077599651,20.5203305951042));
#25705=CARTESIAN_POINT('Ctrl Pts',(31.1770443443443,57.4486642017546,20.4832846315815));
#25706=CARTESIAN_POINT('Ctrl Pts',(31.6520041279563,57.7288973132865,20.4462386680588));
#25707=CARTESIAN_POINT('Ctrl Pts',(32.1269639115684,58.0091304248183,20.4091927045361));
#25708=CARTESIAN_POINT('Ctrl Pts',(32.7545742393267,58.0306402060925,20.3721467410134));
#25709=CARTESIAN_POINT('Ctrl Pts',(33.2476056229439,57.7835825733328,20.3351007774907));
#25710=CARTESIAN_POINT('Ctrl Pts',(33.7406370065611,57.5365249405731,20.2980548139681));
#25711=CARTESIAN_POINT('Ctrl Pts',(34.0990894460373,57.0208998937796,20.2610088504454));
#25712=CARTESIAN_POINT('Ctrl Pts',(34.158915181361,56.4726861646106,20.2239628869227));
#25713=CARTESIAN_POINT('Ctrl Pts',(34.2187409166848,55.9244724354416,20.1869169234));
#25714=CARTESIAN_POINT('Ctrl Pts',(33.9799399478562,55.3436700238972,20.1498709598773));
#25715=CARTESIAN_POINT('Ctrl Pts',(33.5518008766237,54.9960864443956,20.1128249963547));
#25716=CARTESIAN_POINT('Ctrl Pts',(33.1236618053912,54.648502864894,20.075779032832));
#25717=CARTESIAN_POINT('Ctrl Pts',(32.5061846317548,54.5341381174352,20.0387330693093));
#25718=CARTESIAN_POINT('Ctrl Pts',(31.9819612934228,54.7053318784847,20.0016871057866));
#25719=CARTESIAN_POINT('Ctrl Pts',(31.8726832787825,54.7410184131319,19.993964616061));
#25720=CARTESIAN_POINT('Ctrl Pts',(31.7674575454952,54.7891136966038,19.9862421263354));
#25721=CARTESIAN_POINT('Ctrl Pts',(31.6680707239275,54.8477242132621,19.9785196366098));
#25722=CARTESIAN_POINT('Ctrl Pts',(31.6686691446489,54.8508917236136,20.1714803633902));
#25723=CARTESIAN_POINT('Ctrl Pts',(31.8863838499881,54.724528653739,20.1882514925639));
#25724=CARTESIAN_POINT('Ctrl Pts',(32.1309651849205,54.6451654778256,20.2050226217376));
#25725=CARTESIAN_POINT('Ctrl Pts',(32.3799746400722,54.6272090425041,20.2217937509113));
#25726=CARTESIAN_POINT('Ctrl Pts',(32.9300148369371,54.587544840945,20.258839714434));
#25727=CARTESIAN_POINT('Ctrl Pts',(33.5016611438935,54.8475023144793,20.2958856779567));
#25728=CARTESIAN_POINT('Ctrl Pts',(33.8332965022582,55.2881103970044,20.3329316414794));
#25729=CARTESIAN_POINT('Ctrl Pts',(34.1649318606228,55.7287184795295,20.3699776050021));
#25730=CARTESIAN_POINT('Ctrl Pts',(34.2565562703956,56.3499771710453,20.4070235685247));
#25731=CARTESIAN_POINT('Ctrl Pts',(34.0662370704008,56.8675640172576,20.4440695320474));
#25732=CARTESIAN_POINT('Ctrl Pts',(33.8759178704059,57.3851508634698,20.4811154955701));
#25733=CARTESIAN_POINT('Ctrl Pts',(33.4036550606434,57.7990658643784,20.5181614590928));
#25734=CARTESIAN_POINT('Ctrl Pts',(32.8655828553033,57.9198782552653,20.5552074226155));
#25735=CARTESIAN_POINT('Ctrl Pts',(32.3275106499632,58.0406906461521,20.5922533861382));
#25736=CARTESIAN_POINT('Ctrl Pts',(31.7236290490454,57.8684004270172,20.6292993496608));
#25737=CARTESIAN_POINT('Ctrl Pts',(31.3303069678814,57.4818576289614,20.6663453131835));
#25738=CARTESIAN_POINT('Ctrl Pts',(30.9369848867174,57.0953148309056,20.7033912767062));
#25739=CARTESIAN_POINT('Ctrl Pts',(30.754222325307,56.494519453929,20.7404372402289));
#25740=CARTESIAN_POINT('Ctrl Pts',(30.8656634549365,55.954428037577,20.7774832037515));
#25741=CARTESIAN_POINT('Ctrl Pts',(30.959917085256,55.497634599958,20.8088155902978));
#25742=CARTESIAN_POINT('Ctrl Pts',(31.2646228230038,55.0842643987965,20.840147976844));
#25743=CARTESIAN_POINT('Ctrl Pts',(31.6674621971265,54.8470528177236,20.8714803633902));
#25744=CARTESIAN_POINT('Origin',(32.5,56.2916512459885,17.));
#25745=CARTESIAN_POINT('',(31.6652082225275,54.8481806306042,21.5714803633902));
#25746=CARTESIAN_POINT('',(31.667262219952,54.851191363199,21.3785196366098));
#25747=CARTESIAN_POINT('',(31.667,54.8488529232836,17.));
#25748=CARTESIAN_POINT('',(32.1997834265915,57.930378193668,22.));
#25749=CARTESIAN_POINT('Ctrl Pts',(31.6652082225275,54.8481806306042,21.5714803633902));
#25750=CARTESIAN_POINT('Ctrl Pts',(32.0766081468896,54.6152030336121,21.6031823516921));
#25751=CARTESIAN_POINT('Ctrl Pts',(32.5941722167266,54.5601311343425,21.634884339994));
#25752=CARTESIAN_POINT('Ctrl Pts',(33.0407304570643,54.7130293475826,21.6665863282959));
#25753=CARTESIAN_POINT('Ctrl Pts',(33.5625646122208,54.8917014730163,21.7036322918186));
#25754=CARTESIAN_POINT('Ctrl Pts',(33.987436493413,55.3543679573327,21.7406782553412));
#25755=CARTESIAN_POINT('Ctrl Pts',(34.119930861687,55.8897554009177,21.7777242188639));
#25756=CARTESIAN_POINT('Ctrl Pts',(34.2524252299611,56.4251428445027,21.8147701823866));
#25757=CARTESIAN_POINT('Ctrl Pts',(34.092542085317,57.0332512473564,21.8518161459093));
#25758=CARTESIAN_POINT('Ctrl Pts',(33.7156105587364,57.434517372925,21.888862109432));
#25759=CARTESIAN_POINT('Ctrl Pts',(33.3386790321557,57.8357834984935,21.9259080729546));
#25760=CARTESIAN_POINT('Ctrl Pts',(32.7446991236384,58.0302073467771,21.9629540364773));
#25761=CARTESIAN_POINT('Ctrl Pts',(32.1997834265915,57.930378193668,22.));
#25762=CARTESIAN_POINT('',(30.9279127562903,55.7311233941164,22.));
#25763=CARTESIAN_POINT('Origin',(32.5,56.2916512459885,22.));
#25764=CARTESIAN_POINT('Ctrl Pts',(30.9279109916837,55.7311226632894,22.));
#25765=CARTESIAN_POINT('Ctrl Pts',(30.7469516062031,56.2407356224363,21.9636770818144));
#25766=CARTESIAN_POINT('Ctrl Pts',(30.8361764319304,56.8473747622876,21.9273541636289));
#25767=CARTESIAN_POINT('Ctrl Pts',(31.157356786616,57.282481394961,21.8910312454433));
#25768=CARTESIAN_POINT('Ctrl Pts',(31.4849305691822,57.7262492761691,21.8539852819207));
#25769=CARTESIAN_POINT('Ctrl Pts',(32.053786423629,57.9915876156774,21.816939318398));
#25770=CARTESIAN_POINT('Ctrl Pts',(32.604106443046,57.9571481822401,21.7798933548753));
#25771=CARTESIAN_POINT('Ctrl Pts',(33.154426462463,57.9227087488028,21.7428473913526));
#25772=CARTESIAN_POINT('Ctrl Pts',(33.6862106468503,57.5884915424199,21.7058014278299));
#25773=CARTESIAN_POINT('Ctrl Pts',(33.9558248450097,57.1074100574699,21.6687554643072));
#25774=CARTESIAN_POINT('Ctrl Pts',(34.2254390431691,56.6263285725199,21.6317095007846));
#25775=CARTESIAN_POINT('Ctrl Pts',(34.2328832551006,55.9983828090028,21.5946635372619));
#25776=CARTESIAN_POINT('Ctrl Pts',(33.9748805050844,55.5109771631464,21.5576175737392));
#25777=CARTESIAN_POINT('Ctrl Pts',(33.7168777550681,55.02357151729,21.5205716102165));
#25778=CARTESIAN_POINT('Ctrl Pts',(33.1934280431042,54.6767059890943,21.4835256466938));
#25779=CARTESIAN_POINT('Ctrl Pts',(32.6440261878896,54.6291148312821,21.4464796831712));
#25780=CARTESIAN_POINT('Ctrl Pts',(32.3080707772689,54.6000131695149,21.4238263343174));
#25781=CARTESIAN_POINT('Ctrl Pts',(31.962411244236,54.6828172989956,21.4011729854636));
#25782=CARTESIAN_POINT('Ctrl Pts',(31.667262219952,54.851191363199,21.3785196366098));
#25783=CARTESIAN_POINT('Origin',(32.5,56.2916512459885,23.5459252805377));
#25784=CARTESIAN_POINT('',(31.4703515173367,54.5106388084307,13.4540747194623));
#25785=CARTESIAN_POINT('',(31.474888731711,54.5145036461351,13.3959252805377));
#25786=CARTESIAN_POINT('',(31.4726249999999,54.5121855475625,23.5459252805377));
#25787=CARTESIAN_POINT('',(34.1542537360139,57.5104384051693,13.));
#25788=CARTESIAN_POINT('Ctrl Pts',(31.474888731711,54.5145036461351,13.3959252805377));
#25789=CARTESIAN_POINT('Ctrl Pts',(31.1415381650012,54.7083242075053,13.3750880775932));
#25790=CARTESIAN_POINT('Ctrl Pts',(30.3573574995582,55.4957610011485,13.317204911126));
#25791=CARTESIAN_POINT('Ctrl Pts',(30.3807647535574,57.4808407355902,13.2222757811361));
#25792=CARTESIAN_POINT('Ctrl Pts',(32.3530480505924,58.7147951819942,13.1111378905681));
#25793=CARTESIAN_POINT('Ctrl Pts',(33.7489780094279,58.0605171287351,13.0370459635227));
#25794=CARTESIAN_POINT('Ctrl Pts',(34.1542537360139,57.5104384051693,13.));
#25795=CARTESIAN_POINT('',(34.5453697724994,56.5236298181907,13.));
#25796=CARTESIAN_POINT('Origin',(32.5,56.2916512459885,13.));
#25797=CARTESIAN_POINT('Ctrl Pts',(31.4703515173367,54.5106388084307,13.4540747194623));
#25798=CARTESIAN_POINT('Ctrl Pts',(31.4080578130841,54.5460236433933,13.4501772883951));
#25799=CARTESIAN_POINT('Ctrl Pts',(30.7746715994701,54.9531541715192,13.4092338938053));
#25800=CARTESIAN_POINT('Ctrl Pts',(30.0748873839319,56.4258925346357,13.3312445356927));
#25801=CARTESIAN_POINT('Ctrl Pts',(31.2980228170538,58.4019167094404,13.2201066451247));
#25802=CARTESIAN_POINT('Ctrl Pts',(33.60498859151,58.4457294765997,13.1096917998938));
#25803=CARTESIAN_POINT('Ctrl Pts',(34.469350039682,57.1862605871606,13.0363229181856));
#25804=CARTESIAN_POINT('Ctrl Pts',(34.5453721234943,56.5236299659801,13.));
#25805=CARTESIAN_POINT('Origin',(32.5,56.2916512459885,23.5459252805377));
#25806=CARTESIAN_POINT('',(31.4731479817858,54.5151444612292,14.1540747194623));
#25807=CARTESIAN_POINT('',(31.472961077924,54.5097720381012,14.0959252805377));
#25808=CARTESIAN_POINT('',(31.4726249999999,54.5121855475625,23.5459252805377));
#25809=CARTESIAN_POINT('Ctrl Pts',(31.472961077924,54.5097720381012,14.0959252805377));
#25810=CARTESIAN_POINT('Ctrl Pts',(30.9672759169724,54.8072848061285,14.0640305253959));
#25811=CARTESIAN_POINT('Ctrl Pts',(30.1471997784249,55.9394877473567,13.9950898067314));
#25812=CARTESIAN_POINT('Ctrl Pts',(30.8240773215828,58.0494183789814,13.8891031245444));
#25813=CARTESIAN_POINT('Ctrl Pts',(33.0679207153753,58.652967541299,13.7779652339763));
#25814=CARTESIAN_POINT('Ctrl Pts',(34.7917858342248,57.0952271533931,13.6668273434083));
#25815=CARTESIAN_POINT('Ctrl Pts',(34.4182616640155,54.8018644711708,13.5556894528402));
#25816=CARTESIAN_POINT('Ctrl Pts',(32.6876568692323,54.0466007600429,13.4653887652167));
#25817=CARTESIAN_POINT('Ctrl Pts',(31.734194145148,54.3637352784833,13.4121340411158));
#25818=CARTESIAN_POINT('Ctrl Pts',(31.474888731711,54.5145036461351,13.3959252805377));
#25819=CARTESIAN_POINT('Ctrl Pts',(31.4731479817858,54.5151444612292,14.1540747194623));
#25820=CARTESIAN_POINT('Ctrl Pts',(31.2328780723112,54.6524190875731,14.1391197361979));
#25821=CARTESIAN_POINT('Ctrl Pts',(30.4914633330274,55.2894948776179,14.0871187894108));
#25822=CARTESIAN_POINT('Ctrl Pts',(30.2211615693062,57.1314551632494,13.998071879101));
#25823=CARTESIAN_POINT('Ctrl Pts',(31.969659013309,58.6616944230992,13.886933988533));
#25824=CARTESIAN_POINT('Ctrl Pts',(34.2035641928434,58.0226004643432,13.7757960979649));
#25825=CARTESIAN_POINT('Ctrl Pts',(34.8782165391171,55.7991607039093,13.6646582073969));
#25826=CARTESIAN_POINT('Ctrl Pts',(33.428663662975,54.088644942548,13.557417747896));
#25827=CARTESIAN_POINT('Ctrl Pts',(32.0001735569317,54.2096827863809,13.4872232519178));
#25828=CARTESIAN_POINT('Ctrl Pts',(31.4703515173367,54.5106388084307,13.4540747194623));
#25829=CARTESIAN_POINT('Origin',(32.5,56.2916512459885,23.5459252805377));
#25830=CARTESIAN_POINT('',(31.4747795225871,54.5123867379958,14.8540747194623));
#25831=CARTESIAN_POINT('',(31.4704412404259,54.5116709695926,14.7959252805377));
#25832=CARTESIAN_POINT('',(31.4726249999999,54.5121855475625,23.5459252805377));
#25833=CARTESIAN_POINT('Ctrl Pts',(31.4704412404259,54.5116709695925,14.7959252805377));
#25834=CARTESIAN_POINT('Ctrl Pts',(31.3758333938148,54.5652019692603,14.7900189367213));
#25835=CARTESIAN_POINT('Ctrl Pts',(30.7207574218389,55.0095411304487,14.7470666293823));
#25836=CARTESIAN_POINT('Ctrl Pts',(30.0858692295542,56.5568634086541,14.6670683585206));
#25837=CARTESIAN_POINT('Ctrl Pts',(31.4135291597177,58.4637350403728,14.5559304679526));
#25838=CARTESIAN_POINT('Ctrl Pts',(33.73564936737,58.3824733534297,14.4447925773845));
#25839=CARTESIAN_POINT('Ctrl Pts',(34.926763301881,56.387459257788,14.3336546868165));
#25840=CARTESIAN_POINT('Ctrl Pts',(33.8966380568543,54.3047494455222,14.2225167962484));
#25841=CARTESIAN_POINT('Ctrl Pts',(32.2506444060776,54.1164611126689,14.1432736608222));
#25842=CARTESIAN_POINT('Ctrl Pts',(31.5546324883995,54.4617218098652,14.1010764889186));
#25843=CARTESIAN_POINT('Ctrl Pts',(31.472961077924,54.5097720381012,14.0959252805377));
#25844=CARTESIAN_POINT('Ctrl Pts',(31.4747795225871,54.5123867379958,14.8540747194623));
#25845=CARTESIAN_POINT('Ctrl Pts',(31.0607155624738,54.7559913454825,14.8280621840006));
#25846=CARTESIAN_POINT('Ctrl Pts',(30.250819401885,55.6943396944676,14.7650036850163));
#25847=CARTESIAN_POINT('Ctrl Pts',(30.5678191761536,57.7630592969624,14.6648992225092));
#25848=CARTESIAN_POINT('Ctrl Pts',(32.6883055651204,58.7129949703237,14.5537613319412));
#25849=CARTESIAN_POINT('Ctrl Pts',(34.6364334330514,57.4466471822884,14.4426234413732));
#25850=CARTESIAN_POINT('Ctrl Pts',(34.6290601547835,55.1231186965397,14.3314855508051));
#25851=CARTESIAN_POINT('Ctrl Pts',(32.9361539945055,54.0378965296929,14.2353026435015));
#25852=CARTESIAN_POINT('Ctrl Pts',(31.8280663212454,54.3123671657349,14.1761656997206));
#25853=CARTESIAN_POINT('Ctrl Pts',(31.4731479817858,54.5151444612292,14.1540747194623));
#25854=CARTESIAN_POINT('Origin',(32.5,56.2916512459885,23.5459252805377));
#25855=CARTESIAN_POINT('',(31.4709133736318,54.5092374781621,15.5540747194623));
#25856=CARTESIAN_POINT('',(31.4738352212016,54.515219664308,15.4959252805377));
#25857=CARTESIAN_POINT('',(31.4726249999999,54.5121855475625,23.5459252805377));
#25858=CARTESIAN_POINT('Ctrl Pts',(31.4738352212016,54.515219664308,15.4959252805377));
#25859=CARTESIAN_POINT('Ctrl Pts',(31.201543391866,54.6716871554887,15.4789613845241));
#25860=CARTESIAN_POINT('Ctrl Pts',(30.4440567807226,55.3577373025941,15.4249515249878));
#25861=CARTESIAN_POINT('Ctrl Pts',(30.269905357807,57.2534431023133,15.3338957019289));
#25862=CARTESIAN_POINT('Ctrl Pts',(32.0985763090804,58.6869016992398,15.2227578113608));
#25863=CARTESIAN_POINT('Ctrl Pts',(34.2946749356979,57.9279603862777,15.1116199207928));
#25864=CARTESIAN_POINT('Ctrl Pts',(34.848087203459,55.6712867722916,15.0004820302248));
#25865=CARTESIAN_POINT('Ctrl Pts',(33.3370773338915,54.0721923398817,14.895250483473));
#25866=CARTESIAN_POINT('Ctrl Pts',(31.9692358342251,54.2294430763321,14.827064900244));
#25867=CARTESIAN_POINT('Ctrl Pts',(31.4704412404259,54.5116709695925,14.7959252805377));
#25868=CARTESIAN_POINT('Ctrl Pts',(31.4709133820845,54.5092374927209,15.5540747194623));
#25869=CARTESIAN_POINT('Ctrl Pts',(31.4705297975013,54.5094589248369,15.5540505953261));
#25870=CARTESIAN_POINT('Ctrl Pts',(30.8812194784826,54.8499291446222,15.5169805076671));
#25871=CARTESIAN_POINT('Ctrl Pts',(30.074257404191,56.1727516226363,15.4428644564855));
#25872=CARTESIAN_POINT('Ctrl Pts',(31.0845179881232,58.2651696619898,15.3317265659175));
#25873=CARTESIAN_POINT('Ctrl Pts',(33.3903853125313,58.551203914661,15.2205886753495));
#25874=CARTESIAN_POINT('Ctrl Pts',(34.881272858026,56.7690439832157,15.1094507847814));
#25875=CARTESIAN_POINT('Ctrl Pts',(34.192554360499,54.5499210682071,14.9983128942134));
#25876=CARTESIAN_POINT('Ctrl Pts',(32.4784241363503,54.0712848045823,14.913187539107));
#25877=CARTESIAN_POINT('Ctrl Pts',(31.6504081122452,54.4090598663806,14.8651081475233));
#25878=CARTESIAN_POINT('Ctrl Pts',(31.4747795225871,54.5123867379958,14.8540747194623));
#25879=CARTESIAN_POINT('Origin',(32.5,56.2916512459885,23.5459252805377));
#25880=CARTESIAN_POINT('',(31.4717385551609,54.5141703251839,16.2540747194623));
#25881=CARTESIAN_POINT('',(31.4743433646119,54.5114040111285,16.1959252805377));
#25882=CARTESIAN_POINT('',(31.4726249999999,54.5121855475625,23.5459252805377));
#25883=CARTESIAN_POINT('Ctrl Pts',(31.4743433646119,54.5114040111285,16.1959252805377));
#25884=CARTESIAN_POINT('Ctrl Pts',(31.0291266592638,54.7738828820724,16.1679038323268));
#25885=CARTESIAN_POINT('Ctrl Pts',(30.2132159159802,55.7757147456512,16.1028364205933));
#25886=CARTESIAN_POINT('Ctrl Pts',(30.6502037274999,57.8653791294726,16.0007230453371));
#25887=CARTESIAN_POINT('Ctrl Pts',(32.8189508948268,58.6992716537698,15.8895851547691));
#25888=CARTESIAN_POINT('Ctrl Pts',(34.6957586912586,57.3294419144583,15.778447264201));
#25889=CARTESIAN_POINT('Ctrl Pts',(34.5627636554058,55.0097106071378,15.667309373633));
#25890=CARTESIAN_POINT('Ctrl Pts',(32.8501896837687,54.0383319846292,15.5731353790785));
#25891=CARTESIAN_POINT('Ctrl Pts',(31.7961776179314,54.3299915352064,15.5160073480468));
#25892=CARTESIAN_POINT('Ctrl Pts',(31.4738352212016,54.515219664308,15.4959252805377));
#25893=CARTESIAN_POINT('Ctrl Pts',(31.4717385551609,54.5141703251839,16.2540747194623));
#25894=CARTESIAN_POINT('Ctrl Pts',(31.2936631692287,54.6150534746527,16.2429930431288));
#25895=CARTESIAN_POINT('Ctrl Pts',(30.586678710615,55.1642906384242,16.1948654032726));
#25896=CARTESIAN_POINT('Ctrl Pts',(30.1461151763815,56.8896399584928,16.1096917998938));
#25897=CARTESIAN_POINT('Ctrl Pts',(31.7257879044833,58.5935982250311,15.9985539093258));
#25898=CARTESIAN_POINT('Ctrl Pts',(34.0141057438103,58.1905583158083,15.8874160187577));
#25899=CARTESIAN_POINT('Ctrl Pts',(34.9165454246276,56.0494272304867,15.7762781281897));
#25900=CARTESIAN_POINT('Ctrl Pts',(33.6073779089676,54.1304231724864,15.6651643617579));
#25901=CARTESIAN_POINT('Ctrl Pts',(32.0595772284103,54.1694191401902,15.5910965588487));
#25902=CARTESIAN_POINT('Ctrl Pts',(31.4709133820845,54.5092374927209,15.5540747194623));
#25903=CARTESIAN_POINT('Origin',(32.5,56.2916512459885,23.5459252805377));
#25904=CARTESIAN_POINT('',(31.4749299874422,54.5140996860483,16.9540747194623));
#25905=CARTESIAN_POINT('',(31.4704693279511,54.5098093620654,16.8959252805377));
#25906=CARTESIAN_POINT('',(31.4726249999999,54.5121855475625,23.5459252805377));
#25907=CARTESIAN_POINT('Ctrl Pts',(31.4704693279511,54.5098093620654,16.8959252805377));
#25908=CARTESIAN_POINT('Ctrl Pts',(31.4380523744924,54.528339714304,16.8938922436523));
#25909=CARTESIAN_POINT('Ctrl Pts',(30.8255360958299,54.9025793613845,16.8548132432442));
#25910=CARTESIAN_POINT('Ctrl Pts',(30.0713767023175,56.3040842326063,16.7786882793134));
#25911=CARTESIAN_POINT('Ctrl Pts',(31.1932955779139,58.3388173981362,16.6675503887454));
#25912=CARTESIAN_POINT('Ctrl Pts',(33.5112558300795,58.4997561681628,16.5564124981773));
#25913=CARTESIAN_POINT('Ctrl Pts',(34.9036021525568,56.6395914613089,16.4452746076093));
#25914=CARTESIAN_POINT('Ctrl Pts',(34.0959041660874,54.4609531294646,16.3341367170413));
#25915=CARTESIAN_POINT('Ctrl Pts',(32.3994057229947,54.0847909276367,16.251020274684));
#25916=CARTESIAN_POINT('Ctrl Pts',(31.6177287080201,54.4268707431815,16.2049497958495));
#25917=CARTESIAN_POINT('Ctrl Pts',(31.4743433646119,54.5114040111285,16.1959252805377));
#25918=CARTESIAN_POINT('Ctrl Pts',(31.4749299874422,54.5140996860483,16.9540747194623));
#25919=CARTESIAN_POINT('Ctrl Pts',(31.1211066997161,54.7205458521634,16.9319354909316));
#25920=CARTESIAN_POINT('Ctrl Pts',(30.3290943933324,55.5443071105387,16.8727502988782));
#25921=CARTESIAN_POINT('Ctrl Pts',(30.4251293279101,57.5539016004218,16.776519143302));
#25922=CARTESIAN_POINT('Ctrl Pts',(32.4351932585659,58.7194412594432,16.665381252734));
#25923=CARTESIAN_POINT('Ctrl Pts',(34.5045755346152,57.6627971861383,16.554243362166));
#25924=CARTESIAN_POINT('Ctrl Pts',(34.7391470903975,55.3511276839614,16.4431054715979));
#25925=CARTESIAN_POINT('Ctrl Pts',(33.1051720185616,54.0449906258011,16.3430492573634));
#25926=CARTESIAN_POINT('Ctrl Pts',(31.8889678914564,54.277801838456,16.2800390066515));
#25927=CARTESIAN_POINT('Ctrl Pts',(31.4717385551609,54.5141703251839,16.2540747194623));
#25928=CARTESIAN_POINT('Origin',(32.5,56.2916512459885,23.5459252805377));
#25929=CARTESIAN_POINT('',(31.4724078687478,54.5094050924838,17.6540747194623));
#25930=CARTESIAN_POINT('',(31.4724615607262,54.5148044353696,17.5959252805377));
#25931=CARTESIAN_POINT('',(31.4726249999999,54.5121855475625,23.5459252805377));
#25932=CARTESIAN_POINT('Ctrl Pts',(31.4724615607262,54.5148044353696,17.5959252805377));
#25933=CARTESIAN_POINT('Ctrl Pts',(31.2620673353104,54.6344533407431,17.582834691455));
#25934=CARTESIAN_POINT('Ctrl Pts',(30.5366971614125,55.228195386795,17.5326981388497));
#25935=CARTESIAN_POINT('Ctrl Pts',(30.181891163842,57.0160386595509,17.4455156227217));
#25936=CARTESIAN_POINT('Ctrl Pts',(31.8513854749211,58.6320924221469,17.3343777321536));
#25937=CARTESIAN_POINT('Ctrl Pts',(34.1145640165938,58.105913833797,17.2232398415856));
#25938=CARTESIAN_POINT('Ctrl Pts',(34.899913803477,55.9191201236888,17.1121019510176));
#25939=CARTESIAN_POINT('Ctrl Pts',(33.5144124105784,54.1070736669905,17.0029970973349));
#25940=CARTESIAN_POINT('Ctrl Pts',(32.0287535486679,54.190679951206,16.930938207175));
#25941=CARTESIAN_POINT('Ctrl Pts',(31.4704693279511,54.5098093620654,16.8959252805377));
#25942=CARTESIAN_POINT('Ctrl Pts',(31.4724078687478,54.5094050924838,17.6540747194623));
#25943=CARTESIAN_POINT('Ctrl Pts',(30.9460948709879,54.8181696162505,17.6208779387343));
#25944=CARTESIAN_POINT('Ctrl Pts',(30.1270731190026,55.9965693019247,17.5506351944836));
#25945=CARTESIAN_POINT('Ctrl Pts',(30.8867448926705,58.1070774278645,17.4433464867103));
#25946=CARTESIAN_POINT('Ctrl Pts',(33.1503020054966,58.6316238024116,17.3322085961423));
#25947=CARTESIAN_POINT('Ctrl Pts',(34.8186303177654,57.0143667589708,17.2210707055742));
#25948=CARTESIAN_POINT('Ctrl Pts',(34.3646900051272,54.7356000103461,17.1099328150062));
#25949=CARTESIAN_POINT('Ctrl Pts',(32.6344025598171,54.051324400594,17.0209341529688));
#25950=CARTESIAN_POINT('Ctrl Pts',(31.7131654786556,54.375095823104,16.9689814544542));
#25951=CARTESIAN_POINT('Ctrl Pts',(31.4749299874422,54.5140996860483,16.9540747194623));
#25952=CARTESIAN_POINT('Origin',(32.5,56.2916512459885,23.5459252805377));
#25953=CARTESIAN_POINT('',(31.470650904959,54.5123645943458,18.3540747194623));
#25954=CARTESIAN_POINT('',(31.4749676053556,54.5132671274454,18.2959252805377));
#25955=CARTESIAN_POINT('',(31.4726249999999,54.5121855475625,23.5459252805377));
#25956=CARTESIAN_POINT('Ctrl Pts',(31.4749676053556,54.5132671274454,18.2959252805377));
#25957=CARTESIAN_POINT('Ctrl Pts',(31.0898434852659,54.7390742900298,18.2717771392578));
#25958=CARTESIAN_POINT('Ctrl Pts',(30.2875910450901,55.6209976925706,18.2105830344552));
#25959=CARTESIAN_POINT('Ctrl Pts',(30.4964134968881,57.664242527379,18.1123429661299));
#25960=CARTESIAN_POINT('Ctrl Pts',(32.5665574496276,58.7193941910096,18.0012050755619));
#25961=CARTESIAN_POINT('Ctrl Pts',(34.57578061391,57.552405204585,17.8900671849938));
#25962=CARTESIAN_POINT('Ctrl Pts',(34.6850182413274,55.2314338219344,17.7789292944258));
#25963=CARTESIAN_POINT('Ctrl Pts',(33.0169876554982,54.0399676860015,17.6808819929404));
#25964=CARTESIAN_POINT('Ctrl Pts',(31.8574765068094,54.2958506272969,17.6198806549777));
#25965=CARTESIAN_POINT('Ctrl Pts',(31.4724615607262,54.5148044353696,17.5959252805377));
#25966=CARTESIAN_POINT('Ctrl Pts',(31.470650904959,54.5123645943458,18.3540747194623));
#25967=CARTESIAN_POINT('Ctrl Pts',(31.3550533194394,54.5776997670471,18.3468663500598));
#25968=CARTESIAN_POINT('Ctrl Pts',(30.6863525478933,55.0471677720896,18.3026120171345));
#25969=CARTESIAN_POINT('Ctrl Pts',(30.0966496704334,56.6413246029078,18.2213117206866));
#25970=CARTESIAN_POINT('Ctrl Pts',(31.4903368545417,58.5004845570079,18.1101738301185));
#25971=CARTESIAN_POINT('Ctrl Pts',(33.8081801660464,58.3378743316585,17.9990359395505));
#25972=CARTESIAN_POINT('Ctrl Pts',(34.9286313357969,56.3023329102471,17.8878980489824));
#25973=CARTESIAN_POINT('Ctrl Pts',(33.8261287013398,54.2570144404017,17.7767601584144));
#25974=CARTESIAN_POINT('Ctrl Pts',(32.2016889552716,54.1286817447541,17.6988190485744));
#25975=CARTESIAN_POINT('Ctrl Pts',(31.5334341156057,54.4736036964922,17.657923902257));
#25976=CARTESIAN_POINT('Ctrl Pts',(31.4724078687478,54.5094050924838,17.6540747194623));
#25977=CARTESIAN_POINT('Origin',(32.5,56.2916512459885,23.5459252805377));
#25978=CARTESIAN_POINT('',(31.4742218141003,54.5151075144861,19.0540747194623));
#25979=CARTESIAN_POINT('',(31.4715682025536,54.5091203612934,18.9959252805377));
#25980=CARTESIAN_POINT('',(31.4726249999999,54.5121855475625,23.5459252805377));
#25981=CARTESIAN_POINT('Ctrl Pts',(31.4715682025535,54.5091203612934,18.9959252805377));
#25982=CARTESIAN_POINT('Ctrl Pts',(30.9129158471523,54.834613753627,18.9607195870605));
#25983=CARTESIAN_POINT('Ctrl Pts',(30.0982487947041,56.0866128816227,18.8884679300607));
#25984=CARTESIAN_POINT('Ctrl Pts',(30.9872637967357,58.1916498987633,18.7791703095382));
#25985=CARTESIAN_POINT('Ctrl Pts',(33.275871958361,58.5930396107435,18.6680324189701));
#25986=CARTESIAN_POINT('Ctrl Pts',(34.8543157175076,56.8879424529462,18.5568945284021));
#25987=CARTESIAN_POINT('Ctrl Pts',(34.2778276006656,54.6370531910173,18.445756637834));
#25988=CARTESIAN_POINT('Ctrl Pts',(32.5529073535807,54.0606456221556,18.3587668885459));
#25989=CARTESIAN_POINT('Ctrl Pts',(31.6806671821781,54.3926607167737,18.3088231027804));
#25990=CARTESIAN_POINT('Ctrl Pts',(31.4749676053556,54.5132671274454,18.2959252805377));
#25991=CARTESIAN_POINT('Ctrl Pts',(31.4742218141003,54.5151075144861,19.0540747194623));
#25992=CARTESIAN_POINT('Ctrl Pts',(31.1812845288231,54.6841025371816,19.0358087978625));
#25993=CARTESIAN_POINT('Ctrl Pts',(30.4141219270718,55.4032020294196,18.98049691274));
#25994=CARTESIAN_POINT('Ctrl Pts',(30.3049905142645,57.3310249135316,18.8881390640948));
#25995=CARTESIAN_POINT('Ctrl Pts',(32.1827853990159,58.6995007346589,18.7770011735268));
#25996=CARTESIAN_POINT('Ctrl Pts',(34.3509304054687,57.8640446119295,18.6658632829587));
#25997=CARTESIAN_POINT('Ctrl Pts',(34.8248978208363,55.5893590092039,18.5547253923907));
#25998=CARTESIAN_POINT('Ctrl Pts',(33.2781402858533,54.0633320127348,18.4507958712252));
#25999=CARTESIAN_POINT('Ctrl Pts',(31.9491438407913,54.2419227987112,18.3839123135824));
#26000=CARTESIAN_POINT('Ctrl Pts',(31.470650904959,54.5123645943458,18.3540747194623));
#26001=CARTESIAN_POINT('Origin',(32.5,56.2916512459885,23.5459252805377));
#26002=CARTESIAN_POINT('',(31.4739455702221,54.5107934605777,19.7540747194623));
#26003=CARTESIAN_POINT('',(31.471143914755,54.5133742931913,19.6959252805377));
#26004=CARTESIAN_POINT('',(31.4726249999999,54.5121855475625,23.5459252805377));
#26005=CARTESIAN_POINT('Ctrl Pts',(31.471143914755,54.5133742931914,19.6959252805377));
#26006=CARTESIAN_POINT('Ctrl Pts',(31.3231329415045,54.5970512593892,19.686707998386));
#26007=CARTESIAN_POINT('Ctrl Pts',(30.6341370241162,55.106929574873,19.6404447527115));
#26008=CARTESIAN_POINT('Ctrl Pts',(30.1190717238489,56.77076109083,19.5571355435145));
#26009=CARTESIAN_POINT('Ctrl Pts',(31.6112442101669,58.5518456729879,19.4459976529464));
#26010=CARTESIAN_POINT('Ctrl Pts',(33.9169049506455,58.2641486635057,19.3348597623784));
#26011=CARTESIAN_POINT('Ctrl Pts',(34.9256565207284,56.1710023982575,19.2237218718104));
#26012=CARTESIAN_POINT('Ctrl Pts',(33.71417716871,54.1882873915237,19.1125839812423));
#26013=CARTESIAN_POINT('Ctrl Pts',(32.1271617475077,54.1490140977469,19.0366517841514));
#26014=CARTESIAN_POINT('Ctrl Pts',(31.5007700473113,54.4921061888466,18.9977655505832));
#26015=CARTESIAN_POINT('Ctrl Pts',(31.4715682025535,54.5091203612934,18.9959252805377));
#26016=CARTESIAN_POINT('Ctrl Pts',(31.4739455702221,54.5107934605777,19.7540747194623));
#26017=CARTESIAN_POINT('Ctrl Pts',(31.0084978875972,54.7852778310984,19.7247512456653));
#26018=CARTESIAN_POINT('Ctrl Pts',(30.190033600511,55.8297589120184,19.6583818083455));
#26019=CARTESIAN_POINT('Ctrl Pts',(30.7065057264144,57.9292539322016,19.5549664075031));
#26020=CARTESIAN_POINT('Ctrl Pts',(32.9031507850421,58.6866113101155,19.443828516935));
#26021=CARTESIAN_POINT('Ctrl Pts',(34.7307873556619,57.2518345802401,19.332690626367));
#26022=CARTESIAN_POINT('Ctrl Pts',(34.5165589620033,54.9381911555042,19.221552735799));
#26023=CARTESIAN_POINT('Ctrl Pts',(32.7951211292858,54.0400334340294,19.1286807668307));
#26024=CARTESIAN_POINT('Ctrl Pts',(31.7754042355957,54.3413558867002,19.0728547613852));
#26025=CARTESIAN_POINT('Ctrl Pts',(31.4742218141003,54.5151075144861,19.0540747194623));
#26026=CARTESIAN_POINT('Origin',(32.5,56.2916512459885,23.5459252805377));
#26027=CARTESIAN_POINT('',(31.4703419245392,54.5103623955759,20.4540747194623));
#26028=CARTESIAN_POINT('',(31.4746836284318,54.5147000883656,20.3959252805377));
#26029=CARTESIAN_POINT('',(31.4726249999999,54.5121855475625,23.5459252805377));
#26030=CARTESIAN_POINT('Ctrl Pts',(31.4746836284318,54.5147000883656,20.3959252805377));
#26031=CARTESIAN_POINT('Ctrl Pts',(31.1500699868132,54.7031080152175,20.3756504461887));
#26032=CARTESIAN_POINT('Ctrl Pts',(30.3692379110719,55.4752841065875,20.318329648317));
#26033=CARTESIAN_POINT('Ctrl Pts',(30.364399598909,57.4481876795404,20.2239628869227));
#26034=CARTESIAN_POINT('Ctrl Pts',(32.3134406037768,58.7131304053242,20.1128249963547));
#26035=CARTESIAN_POINT('Ctrl Pts',(34.4332415751289,57.7616657784424,20.0016871057866));
#26036=CARTESIAN_POINT('Ctrl Pts',(34.7835245906331,55.4646801872418,19.8905492152186));
#26037=CARTESIAN_POINT('Ctrl Pts',(33.187967321057,54.052355442598,19.7886286068023));
#26038=CARTESIAN_POINT('Ctrl Pts',(31.9180164468304,54.2607380396757,19.7237539619086));
#26039=CARTESIAN_POINT('Ctrl Pts',(31.471143914755,54.5133742931914,19.6959252805377));
#26040=CARTESIAN_POINT('Ctrl Pts',(31.4703419245392,54.5103623955759,20.4540747194623));
#26041=CARTESIAN_POINT('Ctrl Pts',(31.4170740978156,54.5406699166123,20.4507396569907));
#26042=CARTESIAN_POINT('Ctrl Pts',(30.7899238920755,54.9377208245812,20.4103586309964));
#26043=CARTESIAN_POINT('Ctrl Pts',(30.0733055503939,56.3892087930031,20.3329316414794));
#26044=CARTESIAN_POINT('Ctrl Pts',(31.2658594095642,58.3833638027877,20.2217937509113));
#26045=CARTESIAN_POINT('Ctrl Pts',(33.5880364581139,58.4629506390537,20.1106558603433));
#26046=CARTESIAN_POINT('Ctrl Pts',(34.914321242052,56.5551224909764,19.9995179697752));
#26047=CARTESIAN_POINT('Ctrl Pts',(34.0307504904903,54.406136137217,19.8883800792072));
#26048=CARTESIAN_POINT('Ctrl Pts',(32.3488749925858,54.0946310730832,19.8065656624362));
#26049=CARTESIAN_POINT('Ctrl Pts',(31.5965236444215,54.4385065703594,19.7617972091879));
#26050=CARTESIAN_POINT('Ctrl Pts',(31.4739455702221,54.5107934605777,19.7540747194623));
#26051=CARTESIAN_POINT('Origin',(32.5,56.2916512459885,23.5459252805377));
#26052=CARTESIAN_POINT('',(31.4729484072307,54.5150696468519,21.1540747194623));
#26053=CARTESIAN_POINT('',(31.4731950477465,54.5099653993635,21.0959252805377));
#26054=CARTESIAN_POINT('',(31.4726249999999,54.5121855475625,23.5459252805377));
#26055=CARTESIAN_POINT('Ctrl Pts',(31.4731950477465,54.5099653993635,21.0959252805377));
#26056=CARTESIAN_POINT('Ctrl Pts',(30.9763557896561,54.8025287224184,21.0645928939914));
#26057=CARTESIAN_POINT('Ctrl Pts',(30.1562124434263,55.91515240492,20.9962145439225));
#26058=CARTESIAN_POINT('Ctrl Pts',(30.7976747113088,58.0238313492005,20.890790230331));
#26059=CARTESIAN_POINT('Ctrl Pts',(33.0320547584019,58.6613103307746,20.7796523397629));
#26060=CARTESIAN_POINT('Ctrl Pts',(34.7794413280769,57.1298124049937,20.6685144491949));
#26061=CARTESIAN_POINT('Ctrl Pts',(34.4404282620852,54.8311366011664,20.5573765586268));
#26062=CARTESIAN_POINT('Ctrl Pts',(32.711178041167,54.0447560839335,20.4665135024078));
#26063=CARTESIAN_POINT('Ctrl Pts',(31.7432006097017,54.3588510380505,20.4126964097114));
#26064=CARTESIAN_POINT('Ctrl Pts',(31.4746836284318,54.5147000883656,20.3959252805377));
#26065=CARTESIAN_POINT('Ctrl Pts',(31.4729484072307,54.5150696468519,21.1540747194623));
#26066=CARTESIAN_POINT('Ctrl Pts',(31.2416713093181,54.6470066065867,21.1396821047934));
#26067=CARTESIAN_POINT('Ctrl Pts',(30.5049700979161,55.27079766484,21.0882435266019));
#26068=CARTESIAN_POINT('Ctrl Pts',(30.2087196709517,57.0968534624393,20.9997589848876));
#26069=CARTESIAN_POINT('Ctrl Pts',(31.9338196700205,58.6533891775714,20.8886210943196));
#26070=CARTESIAN_POINT('Ctrl Pts',(34.1771709144469,58.0482026788783,20.7774832037515));
#26071=CARTESIAN_POINT('Ctrl Pts',(34.8853786224564,55.8352230845946,20.6663453131835));
#26072=CARTESIAN_POINT('Ctrl Pts',(33.4544940412401,54.0938892869953,20.5585424850871));
#26073=CARTESIAN_POINT('Ctrl Pts',(32.0087745479626,54.2040131588077,20.4877856205134));
#26074=CARTESIAN_POINT('Ctrl Pts',(31.4703419245392,54.5103623955759,20.4540747194623));
#26075=CARTESIAN_POINT('Origin',(32.5,56.2916512459885,23.5459252805377));
#26076=CARTESIAN_POINT('',(31.4756555660462,54.5128362942924,21.8540747194623));
#26077=CARTESIAN_POINT('',(31.4704151231924,54.5113563798656,21.7959252805377));
#26078=CARTESIAN_POINT('',(31.4726249999999,54.5121855475625,23.5459252805377));
#26079=CARTESIAN_POINT('',(33.9541262883781,54.8399232067374,22.));
#26080=CARTESIAN_POINT('Ctrl Pts',(33.9541262883781,54.8399232067375,22.));
#26081=CARTESIAN_POINT('Ctrl Pts',(33.4713921772736,54.3563916207415,21.9629540364773));
#26082=CARTESIAN_POINT('Ctrl Pts',(32.5011748783928,54.0682382375652,21.9143122762981));
#26083=CARTESIAN_POINT('Ctrl Pts',(31.6603808354701,54.4043184181514,21.8656705161189));
#26084=CARTESIAN_POINT('Ctrl Pts',(31.4756555660462,54.5128362942924,21.8540747194623));
#26085=CARTESIAN_POINT('',(34.4879501863793,55.7574173922323,22.));
#26086=CARTESIAN_POINT('Origin',(32.5,56.2916512459885,22.));
#26087=CARTESIAN_POINT('Ctrl Pts',(34.4879524958972,55.7574168944053,22.));
#26088=CARTESIAN_POINT('Ctrl Pts',(34.3140194691063,55.1135181402384,21.9636770818144));
#26089=CARTESIAN_POINT('Ctrl Pts',(33.3475254337068,54.0782693974497,21.895652175327));
#26090=CARTESIAN_POINT('Ctrl Pts',(31.9778124788844,54.224015012867,21.8276272688396));
#26091=CARTESIAN_POINT('Ctrl Pts',(31.4704151231923,54.5113563798656,21.7959252805377));
#26092=CARTESIAN_POINT('Origin',(-32.5,56.2916512459885,17.));
#26093=CARTESIAN_POINT('',(-31.665169034441,54.8481104542882,13.8714803633902));
#26094=CARTESIAN_POINT('',(-31.6668355785528,54.8466294620446,13.6785196366098));
#26095=CARTESIAN_POINT('',(-31.667,54.8488529232836,17.));
#26096=CARTESIAN_POINT('',(-31.4059736530045,55.03520293743,13.));
#26097=CARTESIAN_POINT('Ctrl Pts',(-31.6668355785528,54.8466294620446,13.6785196366098));
#26098=CARTESIAN_POINT('Ctrl Pts',(-31.7169359983484,54.8172333383902,13.6746222055426));
#26099=CARTESIAN_POINT('Ctrl Pts',(-31.7685916060498,54.790608714332,13.6707247744754));
#26100=CARTESIAN_POINT('Ctrl Pts',(-31.8215990010623,54.7670212268678,13.6668273434082));
#26101=CARTESIAN_POINT('Ctrl Pts',(-32.3254462758995,54.5428168252686,13.6297813798856));
#26102=CARTESIAN_POINT('Ctrl Pts',(-32.951426619549,54.5930156597358,13.5927354163629));
#26103=CARTESIAN_POINT('Ctrl Pts',(-33.413026316092,54.8947720750737,13.5556894528402));
#26104=CARTESIAN_POINT('Ctrl Pts',(-33.8746260126349,55.1965284904116,13.5186434893175));
#26105=CARTESIAN_POINT('Ctrl Pts',(-34.1718450620713,55.74984248662,13.4815975257948));
#26106=CARTESIAN_POINT('Ctrl Pts',(-34.1687200176702,56.3012302340885,13.4445515622722));
#26107=CARTESIAN_POINT('Ctrl Pts',(-34.165594973269,56.852617981557,13.4075055987495));
#26108=CARTESIAN_POINT('Ctrl Pts',(-33.8621258350302,57.4020794802856,13.3704596352268));
#26109=CARTESIAN_POINT('Ctrl Pts',(-33.397076207884,57.6986656733007,13.3334136717041));
#26110=CARTESIAN_POINT('Ctrl Pts',(-32.9320265807378,57.9952518663159,13.2963677081814));
#26111=CARTESIAN_POINT('Ctrl Pts',(-32.3053964646841,58.0389627536176,13.2593217446587));
#26112=CARTESIAN_POINT('Ctrl Pts',(-31.8042046430419,57.8087421867188,13.2222757811361));
#26113=CARTESIAN_POINT('Ctrl Pts',(-31.3030128213997,57.5785216198199,13.1852298176134));
#26114=CARTESIAN_POINT('Ctrl Pts',(-30.927259294169,57.0743695987204,13.1481838540907));
#26115=CARTESIAN_POINT('Ctrl Pts',(-30.8485497633826,56.5294873752105,13.111137890568));
#26116=CARTESIAN_POINT('Ctrl Pts',(-30.7698402325962,55.9846051517008,13.0740919270453));
#26117=CARTESIAN_POINT('Ctrl Pts',(-30.9881746982541,55.3989927257806,13.0370459635227));
#26118=CARTESIAN_POINT('Ctrl Pts',(-31.4059736530044,55.03520293743,13.));
#26119=CARTESIAN_POINT('',(-33.9184188470959,55.4120275291384,13.));
#26120=CARTESIAN_POINT('Origin',(-32.5,56.2916512459885,13.));
#26121=CARTESIAN_POINT('',(-31.6677099856843,54.8513822049942,13.1714803633902));
#26122=CARTESIAN_POINT('Ctrl Pts',(-33.9184205240577,55.4120266023846,13.));
#26123=CARTESIAN_POINT('Ctrl Pts',(-33.6328154176796,54.9528086674659,13.0363229181856));
#26124=CARTESIAN_POINT('Ctrl Pts',(-33.1028950308971,54.6443333840239,13.0726458363711));
#26125=CARTESIAN_POINT('Ctrl Pts',(-32.5624622032656,54.6241575874771,13.1089687545567));
#26126=CARTESIAN_POINT('Ctrl Pts',(-32.2524345659017,54.6125834302173,13.1298059575012));
#26127=CARTESIAN_POINT('Ctrl Pts',(-31.9389473679306,54.6958863393048,13.1506431604457));
#26128=CARTESIAN_POINT('Ctrl Pts',(-31.6677099856843,54.8513822049942,13.1714803633902));
#26129=CARTESIAN_POINT('',(-31.667,54.8488529232836,12.));
#26130=CARTESIAN_POINT('',(-31.667,54.8488529232836,17.));
#26131=CARTESIAN_POINT('Origin',(-32.5,56.2916512459885,12.));
#26132=CARTESIAN_POINT('Ctrl Pts',(-31.6677099856843,54.8513822049942,13.1714803633902));
#26133=CARTESIAN_POINT('Ctrl Pts',(-31.456720929217,54.9723387107481,13.1876891239684));
#26134=CARTESIAN_POINT('Ctrl Pts',(-31.2712968605908,55.1369785326558,13.2038978845465));
#26135=CARTESIAN_POINT('Ctrl Pts',(-31.1329525371814,55.334624580881,13.2201066451247));
#26136=CARTESIAN_POINT('Ctrl Pts',(-30.8167594060732,55.7863548817661,13.2571526086474));
#26137=CARTESIAN_POINT('Ctrl Pts',(-30.74649897558,56.4105013743272,13.2941985721701));
#26138=CARTESIAN_POINT('Ctrl Pts',(-30.9545219587097,56.9212436588755,13.3312445356927));
#26139=CARTESIAN_POINT('Ctrl Pts',(-31.1625449418395,57.4319859434239,13.3682904992154));
#26140=CARTESIAN_POINT('Ctrl Pts',(-31.6488513385922,57.8293240199595,13.4053364627381));
#26141=CARTESIAN_POINT('Ctrl Pts',(-32.1907825642961,57.9315018386831,13.4423824262608));
#26142=CARTESIAN_POINT('Ctrl Pts',(-32.73271379,58.0336796574067,13.4794283897835));
#26143=CARTESIAN_POINT('Ctrl Pts',(-33.3302698446549,57.8406972183184,13.5164743533061));
#26144=CARTESIAN_POINT('Ctrl Pts',(-33.7100246193121,57.4408300847798,13.5535203168288));
#26145=CARTESIAN_POINT('Ctrl Pts',(-34.0897793939694,57.0409629512412,13.5905662803515));
#26146=CARTESIAN_POINT('Ctrl Pts',(-34.2517328886288,56.4342111232524,13.6276122438742));
#26147=CARTESIAN_POINT('Ctrl Pts',(-34.1217417856583,55.8982799679713,13.6646582073969));
#26148=CARTESIAN_POINT('Ctrl Pts',(-33.9917506826877,55.3623488126902,13.7017041709196));
#26149=CARTESIAN_POINT('Ctrl Pts',(-33.5698149820872,54.8972383301168,13.7387501344422));
#26150=CARTESIAN_POINT('Ctrl Pts',(-33.0490481303448,54.7157980032898,13.7757960979649));
#26151=CARTESIAN_POINT('Ctrl Pts',(-32.6006934475977,54.5595867930335,13.8076908531067));
#26152=CARTESIAN_POINT('Ctrl Pts',(-32.0790815152818,54.6136422361012,13.8395856082484));
#26153=CARTESIAN_POINT('Ctrl Pts',(-31.665169034441,54.8481104542882,13.8714803633902));
#26154=CARTESIAN_POINT('Origin',(-32.5,56.2916512459885,17.));
#26155=CARTESIAN_POINT('',(-31.6675239681331,54.8471109129233,14.5714803633902));
#26156=CARTESIAN_POINT('',(-31.6688656529171,54.8504196807178,14.3785196366098));
#26157=CARTESIAN_POINT('',(-31.667,54.8488529232836,17.));
#26158=CARTESIAN_POINT('Ctrl Pts',(-31.6688656529171,54.8504196807178,14.3785196366098));
#26159=CARTESIAN_POINT('Ctrl Pts',(-31.8626626794392,54.7373590837469,14.3635646533453));
#26160=CARTESIAN_POINT('Ctrl Pts',(-32.0777548846389,54.6619147081679,14.3486096700809));
#26161=CARTESIAN_POINT('Ctrl Pts',(-32.2987508779934,54.6350670487033,14.3336546868165));
#26162=CARTESIAN_POINT('Ctrl Pts',(-32.8461944534029,54.5685609620293,14.2966087232938));
#26163=CARTESIAN_POINT('Ctrl Pts',(-33.4298657229247,54.8002611998549,14.2595627597711));
#26164=CARTESIAN_POINT('Ctrl Pts',(-33.7826437493636,55.2241308285784,14.2225167962484));
#26165=CARTESIAN_POINT('Ctrl Pts',(-34.1354217758025,55.648000457302,14.1854708327258));
#26166=CARTESIAN_POINT('Ctrl Pts',(-34.2573065591586,56.2640394769235,14.1484248692031));
#26167=CARTESIAN_POINT('Ctrl Pts',(-34.0925177799173,56.7903101462247,14.1113789056804));
#26168=CARTESIAN_POINT('Ctrl Pts',(-33.9277290006759,57.316580815526,14.0743329421577));
#26169=CARTESIAN_POINT('Ctrl Pts',(-33.4762666588371,57.7530831345071,14.037286978635));
#26170=CARTESIAN_POINT('Ctrl Pts',(-32.9447431684491,57.9000573283161,14.0002410151124));
#26171=CARTESIAN_POINT('Ctrl Pts',(-32.4132196780611,58.0470315221252,13.9631950515897));
#26172=CARTESIAN_POINT('Ctrl Pts',(-31.8016350391239,57.9044775907622,13.926149088067));
#26173=CARTESIAN_POINT('Ctrl Pts',(-31.3898882053201,57.5376201658139,13.8891031245443));
#26174=CARTESIAN_POINT('Ctrl Pts',(-30.9781413715162,57.1707627408656,13.8520571610216));
#26175=CARTESIAN_POINT('Ctrl Pts',(-30.7662323428457,56.579601822332,13.815011197499));
#26176=CARTESIAN_POINT('Ctrl Pts',(-30.8511349315229,56.0347175442324,13.7779652339763));
#26177=CARTESIAN_POINT('Ctrl Pts',(-30.9271053193521,55.5471579706766,13.7448167015208));
#26178=CARTESIAN_POINT('Ctrl Pts',(-31.2407201802287,55.0966501403397,13.7116681690653));
#26179=CARTESIAN_POINT('Ctrl Pts',(-31.6668355785528,54.8466294620446,13.6785196366098));
#26180=CARTESIAN_POINT('Ctrl Pts',(-31.665169034441,54.8481104542882,13.8714803633902));
#26181=CARTESIAN_POINT('Ctrl Pts',(-31.5983195028865,54.885978581672,13.8766315717711));
#26182=CARTESIAN_POINT('Ctrl Pts',(-31.5342792394079,54.92855265549,13.881782780152));
#26183=CARTESIAN_POINT('Ctrl Pts',(-31.4738105761083,54.9757069077013,13.886933988533));
#26184=CARTESIAN_POINT('Ctrl Pts',(-31.0389378764983,55.3148263100205,13.9239799520556));
#26185=CARTESIAN_POINT('Ctrl Pts',(-30.7887904801626,55.8908352857396,13.9610259155783));
#26186=CARTESIAN_POINT('Ctrl Pts',(-30.83785280129,56.4401173240505,13.998071879101));
#26187=CARTESIAN_POINT('Ctrl Pts',(-30.8869151224175,56.9893993623614,14.0351178426237));
#26188=CARTESIAN_POINT('Ctrl Pts',(-31.235187161008,57.5119544632642,14.0721638061464));
#26189=CARTESIAN_POINT('Ctrl Pts',(-31.72327872518,57.7686336889847,14.109209769669));
#26190=CARTESIAN_POINT('Ctrl Pts',(-32.2113702893519,58.0253129147052,14.1462557331917));
#26191=CARTESIAN_POINT('Ctrl Pts',(-32.8392813791053,58.0161162652434,14.1833016967144));
#26192=CARTESIAN_POINT('Ctrl Pts',(-33.3196456823451,57.7452519563499,14.2203476602371));
#26193=CARTESIAN_POINT('Ctrl Pts',(-33.8000099855849,57.4743876474564,14.2573936237598));
#26194=CARTESIAN_POINT('Ctrl Pts',(-34.1328275023111,56.9418556791311,14.2944395872824));
#26195=CARTESIAN_POINT('Ctrl Pts',(-34.1657820298073,56.3913726675535,14.3314855508051));
#26196=CARTESIAN_POINT('Ctrl Pts',(-34.1987365573035,55.8408896559759,14.3685315143278));
#26197=CARTESIAN_POINT('Ctrl Pts',(-33.9318280955697,55.2724556011459,14.4055774778505));
#26198=CARTESIAN_POINT('Ctrl Pts',(-33.4872090049183,54.9462174010391,14.4426234413732));
#26199=CARTESIAN_POINT('Ctrl Pts',(-33.0425899142668,54.6199792009323,14.4796694048958));
#26200=CARTESIAN_POINT('Ctrl Pts',(-32.4202601946978,54.5359368555486,14.5167153684185));
#26201=CARTESIAN_POINT('Ctrl Pts',(-31.9050324766411,54.7325529059597,14.5537613319412));
#26202=CARTESIAN_POINT('Ctrl Pts',(-31.8228882493844,54.7638999646704,14.5596676757575));
#26203=CARTESIAN_POINT('Ctrl Pts',(-31.7434664303386,54.8023810331132,14.5655740195739));
#26204=CARTESIAN_POINT('Ctrl Pts',(-31.6675239681331,54.8471109129233,14.5714803633902));
#26205=CARTESIAN_POINT('Origin',(-32.5,56.2916512459885,17.));
#26206=CARTESIAN_POINT('',(-31.6686398531931,54.8509327367609,15.2714803633902));
#26207=CARTESIAN_POINT('',(-31.6662678127889,54.8504473245041,15.0785196366098));
#26208=CARTESIAN_POINT('',(-31.667,54.8488529232836,17.));
#26209=CARTESIAN_POINT('Ctrl Pts',(-31.6662678127889,54.8504473245041,15.0785196366098));
#26210=CARTESIAN_POINT('Ctrl Pts',(-32.0051837911953,54.6584589297703,15.0525071011481));
#26211=CARTESIAN_POINT('Ctrl Pts',(-32.4124263355195,54.5807898609867,15.0264945656864));
#26212=CARTESIAN_POINT('Ctrl Pts',(-32.7936098272491,54.6489198132192,15.0004820302247));
#26213=CARTESIAN_POINT('Ctrl Pts',(-33.3364753910795,54.745947637705,14.9634360667021));
#26214=CARTESIAN_POINT('Ctrl Pts',(-33.8264872979809,55.138688877304,14.9263901031794));
#26215=CARTESIAN_POINT('Ctrl Pts',(-34.0393888128716,55.6474033077565,14.8893441396567));
#26216=CARTESIAN_POINT('Ctrl Pts',(-34.2522903277622,56.1561177382089,14.852298176134));
#26217=CARTESIAN_POINT('Ctrl Pts',(-34.1880814506421,56.7808053595149,14.8152522126113));
#26218=CARTESIAN_POINT('Ctrl Pts',(-33.8761477528875,57.2355742774498,14.7782062490887));
#26219=CARTESIAN_POINT('Ctrl Pts',(-33.5642140551329,57.6903431953847,14.741160285566));
#26220=CARTESIAN_POINT('Ctrl Pts',(-33.0045555367438,57.9751934099486,14.7041143220433));
#26221=CARTESIAN_POINT('Ctrl Pts',(-32.4533030627753,57.959761729544,14.6670683585206));
#26222=CARTESIAN_POINT('Ctrl Pts',(-31.9020505888069,57.9443300491394,14.6300223949979));
#26223=CARTESIAN_POINT('Ctrl Pts',(-31.3592041592591,57.6286164737664,14.5929764314753));
#26224=CARTESIAN_POINT('Ctrl Pts',(-31.0732005795316,57.1571088626351,14.5559304679526));
#26225=CARTESIAN_POINT('Ctrl Pts',(-30.787196999804,56.6856012515039,14.5188845044299));
#26226=CARTESIAN_POINT('Ctrl Pts',(-30.7580362698967,56.0582996046144,14.4818385409072));
#26227=CARTESIAN_POINT('Ctrl Pts',(-30.9990638455916,55.5622925755827,14.4447925773845));
#26228=CARTESIAN_POINT('Ctrl Pts',(-31.142791661258,55.2665172617733,14.4227015971263));
#26229=CARTESIAN_POINT('Ctrl Pts',(-31.3825954370759,55.0174288556201,14.400610616868));
#26230=CARTESIAN_POINT('Ctrl Pts',(-31.6688656529171,54.8504196807178,14.3785196366098));
#26231=CARTESIAN_POINT('Ctrl Pts',(-31.6675239681331,54.8471109129233,14.5714803633902));
#26232=CARTESIAN_POINT('Ctrl Pts',(-31.2671376265686,55.0829372532297,14.6026199830965));
#26233=CARTESIAN_POINT('Ctrl Pts',(-30.9634650148059,55.4924582968624,14.6337596028029));
#26234=CARTESIAN_POINT('Ctrl Pts',(-30.8674364226636,55.9459488454016,14.6648992225092));
#26235=CARTESIAN_POINT('Ctrl Pts',(-30.7531938032872,56.4854542882262,14.7019451860319));
#26236=CARTESIAN_POINT('Ctrl Pts',(-30.9328342810788,57.0871907276693,14.7389911495546));
#26237=CARTESIAN_POINT('Ctrl Pts',(-31.3241443491424,57.4757700913935,14.7760371130773));
#26238=CARTESIAN_POINT('Ctrl Pts',(-31.715454417206,57.8643494551177,14.8130830766));
#26239=CARTESIAN_POINT('Ctrl Pts',(-32.3184340755416,58.039771743123,14.8501290401227));
#26240=CARTESIAN_POINT('Ctrl Pts',(-32.8571262761764,57.9217539399754,14.8871750036453));
#26241=CARTESIAN_POINT('Ctrl Pts',(-33.3958184768112,57.8037361368277,14.924220967168));
#26242=CARTESIAN_POINT('Ctrl Pts',(-33.8702232197452,57.3922782425271,14.9612669306907));
#26243=CARTESIAN_POINT('Ctrl Pts',(-34.063226478426,56.8756863008287,14.9983128942134));
#26244=CARTESIAN_POINT('Ctrl Pts',(-34.2562297371068,56.3590943591303,15.0353588577361));
#26245=CARTESIAN_POINT('Ctrl Pts',(-34.1678315115345,55.737368370034,15.0724048212587));
#26246=CARTESIAN_POINT('Ctrl Pts',(-33.8384877538371,55.2950447552266,15.1094507847814));
#26247=CARTESIAN_POINT('Ctrl Pts',(-33.5091439961397,54.8527211404192,15.1464967483041));
#26248=CARTESIAN_POINT('Ctrl Pts',(-32.9388547063171,54.5897998999006,15.1835427118268));
#26249=CARTESIAN_POINT('Ctrl Pts',(-32.3886160101468,54.6266084315825,15.2205886753495));
#26250=CARTESIAN_POINT('Ctrl Pts',(-32.1366535522459,54.6434636040355,15.237552571363));
#26251=CARTESIAN_POINT('Ctrl Pts',(-31.8888954229186,54.7231679104083,15.2545164673766));
#26252=CARTESIAN_POINT('Ctrl Pts',(-31.6686398531931,54.8509327367609,15.2714803633902));
#26253=CARTESIAN_POINT('Origin',(-32.5,56.2916512459885,17.));
#26254=CARTESIAN_POINT('',(-31.6657545866043,54.8497426695208,15.9714803633902));
#26255=CARTESIAN_POINT('',(-31.6656238197278,54.8464558867275,15.7785196366098));
#26256=CARTESIAN_POINT('',(-31.667,54.8488529232836,17.));
#26257=CARTESIAN_POINT('Ctrl Pts',(-31.6656238265237,54.8464558985647,15.7785196366098));
#26258=CARTESIAN_POINT('Ctrl Pts',(-32.1435040363299,54.5705135726952,15.7414495489508));
#26259=CARTESIAN_POINT('Ctrl Pts',(-32.7717977196734,54.5551568083656,15.7043794612919));
#26260=CARTESIAN_POINT('Ctrl Pts',(-33.2626292375688,54.8073433428058,15.667309373633));
#26261=CARTESIAN_POINT('Ctrl Pts',(-33.7531413365699,55.0593657615749,15.6302634101103));
#26262=CARTESIAN_POINT('Ctrl Pts',(-34.1063700665184,55.5785832727215,15.5932174465876));
#26263=CARTESIAN_POINT('Ctrl Pts',(-34.1606582960962,56.127373038589,15.5561714830649));
#26264=CARTESIAN_POINT('Ctrl Pts',(-34.2149465256739,56.6761628044566,15.5191255195423));
#26265=CARTESIAN_POINT('Ctrl Pts',(-33.9702942548808,57.254524825045,15.4820795560196));
#26266=CARTESIAN_POINT('Ctrl Pts',(-33.5386679829466,57.5977684411295,15.4450335924969));
#26267=CARTESIAN_POINT('Ctrl Pts',(-33.1070417110123,57.941012057214,15.4079876289742));
#26268=CARTESIAN_POINT('Ctrl Pts',(-32.4884414379368,58.0491372687945,15.3709416654515));
#26269=CARTESIAN_POINT('Ctrl Pts',(-31.9659730859382,57.8726599616145,15.3338957019289));
#26270=CARTESIAN_POINT('Ctrl Pts',(-31.4435047339396,57.6961826544345,15.2968497384062));
#26271=CARTESIAN_POINT('Ctrl Pts',(-31.0171683030177,57.2351028284939,15.2598037748835));
#26272=CARTESIAN_POINT('Ctrl Pts',(-30.8820790791908,56.7004362767628,15.2227578113608));
#26273=CARTESIAN_POINT('Ctrl Pts',(-30.7469898553639,56.1657697250316,15.1857118478381));
#26274=CARTESIAN_POINT('Ctrl Pts',(-30.9031478386319,55.5575164475099,15.1486658843155));
#26275=CARTESIAN_POINT('Ctrl Pts',(-31.2790864406456,55.1540470134353,15.1116199207928));
#26276=CARTESIAN_POINT('Ctrl Pts',(-31.391052526185,55.0338813988212,15.1005864927318));
#26277=CARTESIAN_POINT('Ctrl Pts',(-31.5225138495515,54.9318807605089,15.0895530646708));
#26278=CARTESIAN_POINT('Ctrl Pts',(-31.6662678127889,54.8504473245041,15.0785196366098));
#26279=CARTESIAN_POINT('Ctrl Pts',(-31.6686398531931,54.8509327367609,15.2714803633902));
#26280=CARTESIAN_POINT('Ctrl Pts',(-31.4078986168085,55.0021823003073,15.2915624308993));
#26281=CARTESIAN_POINT('Ctrl Pts',(-31.1856997806351,55.2207844238422,15.3116444984084));
#26282=CARTESIAN_POINT('Ctrl Pts',(-31.0406952948155,55.4822046794947,15.3317265659175));
#26283=CARTESIAN_POINT('Ctrl Pts',(-30.7732013781725,55.9644540918427,15.3687725294402));
#26284=CARTESIAN_POINT('Ctrl Pts',(-30.7684016474046,56.5924146126563,15.4058184929629));
#26285=CARTESIAN_POINT('Ctrl Pts',(-31.0284927261472,57.0786965491371,15.4428644564855));
#26286=CARTESIAN_POINT('Ctrl Pts',(-31.2885838048897,57.5649784856178,15.4799104200082));
#26287=CARTESIAN_POINT('Ctrl Pts',(-31.8135656931427,57.9095818377658,15.5169563835309));
#26288=CARTESIAN_POINT('Ctrl Pts',(-32.3631774530806,57.9547969272716,15.5540023470536));
#26289=CARTESIAN_POINT('Ctrl Pts',(-32.9127892130186,58.0000120167773,15.5910483105763));
#26290=CARTESIAN_POINT('Ctrl Pts',(-33.4870308446415,57.7458388436409,15.6280942740989));
#26291=CARTESIAN_POINT('Ctrl Pts',(-33.8230974089741,57.3086012018905,15.6651402376216));
#26292=CARTESIAN_POINT('Ctrl Pts',(-34.1591639733067,56.87136356014,15.7021862011443));
#26293=CARTESIAN_POINT('Ctrl Pts',(-34.257055470349,56.2510614497756,15.739232164667));
#26294=CARTESIAN_POINT('Ctrl Pts',(-34.0719713014427,55.7315796489165,15.7762781281897));
#26295=CARTESIAN_POINT('Ctrl Pts',(-33.8868871325364,55.2120978480574,15.8133240917123));
#26296=CARTESIAN_POINT('Ctrl Pts',(-33.4188272976816,54.7934363567036,15.850370055235));
#26297=CARTESIAN_POINT('Ctrl Pts',(-32.8820020343565,54.6671979803659,15.8874160187577));
#26298=CARTESIAN_POINT('Ctrl Pts',(-32.4759491237521,54.5717116766394,15.9154374669685));
#26299=CARTESIAN_POINT('Ctrl Pts',(-32.03055302792,54.6435311984541,15.9434589151794));
#26300=CARTESIAN_POINT('Ctrl Pts',(-31.6657545866043,54.8497426695208,15.9714803633902));
#26301=CARTESIAN_POINT('Origin',(-32.5,56.2916512459885,17.));
#26302=CARTESIAN_POINT('',(-31.6662054032747,54.8463759356941,16.6714803633902));
#26303=CARTESIAN_POINT('',(-31.6687530214683,54.8490350969289,16.4785196366098));
#26304=CARTESIAN_POINT('',(-31.667,54.8488529232836,17.));
#26305=CARTESIAN_POINT('Ctrl Pts',(-31.6687530214683,54.8490350969289,16.4785196366098));
#26306=CARTESIAN_POINT('Ctrl Pts',(-31.8117829954436,54.7648928865345,16.4674379602763));
#26307=CARTESIAN_POINT('Ctrl Pts',(-31.9665782677991,54.7018565467284,16.4563562839428));
#26308=CARTESIAN_POINT('Ctrl Pts',(-32.1273756622831,54.6650214760002,16.4452746076093));
#26309=CARTESIAN_POINT('Ctrl Pts',(-32.6649201845491,54.5418821020027,16.4082286440866));
#26310=CARTESIAN_POINT('Ctrl Pts',(-33.2695420256081,54.7115576426435,16.3711826805639));
#26311=CARTESIAN_POINT('Ctrl Pts',(-33.6645325714613,55.0963951246187,16.3341367170412));
#26312=CARTESIAN_POINT('Ctrl Pts',(-34.0595231173144,55.4812326065939,16.2970907535186));
#26313=CARTESIAN_POINT('Ctrl Pts',(-34.2448823679618,56.0812320299036,16.2600447899959));
#26314=CARTESIAN_POINT('Ctrl Pts',(-34.1357796112843,56.6218002562495,16.2229988264732));
#26315=CARTESIAN_POINT('Ctrl Pts',(-34.0266768546068,57.1623684825954,16.1859528629505));
#26316=CARTESIAN_POINT('Ctrl Pts',(-33.6231120906045,57.6435055119775,16.1489068994278));
#26317=CARTESIAN_POINT('Ctrl Pts',(-33.1097790218944,57.8450162546515,16.1118609359052));
#26318=CARTESIAN_POINT('Ctrl Pts',(-32.5964459531844,58.0465269973256,16.0748149723825));
#26319=CARTESIAN_POINT('Ctrl Pts',(-31.9733445797666,57.9684114532915,16.0377690088598));
#26320=CARTESIAN_POINT('Ctrl Pts',(-31.5256407784037,57.6464196442519,16.0007230453371));
#26321=CARTESIAN_POINT('Ctrl Pts',(-31.0779369770408,57.3244278352123,15.9636770818144));
#26322=CARTESIAN_POINT('Ctrl Pts',(-30.8056307477328,56.7585597611672,15.9266311182918));
#26323=CARTESIAN_POINT('Ctrl Pts',(-30.8333445804181,56.2077881548333,15.8895851547691));
#26324=CARTESIAN_POINT('Ctrl Pts',(-30.8610403660015,55.6573752080673,15.8525633153826));
#26325=CARTESIAN_POINT('Ctrl Pts',(-31.188365597836,55.1220390739338,15.8155414759962));
#26326=CARTESIAN_POINT('Ctrl Pts',(-31.6656238265237,54.8464558985647,15.7785196366098));
#26327=CARTESIAN_POINT('Ctrl Pts',(-31.6657545866043,54.8497426695208,15.9714803633902));
#26328=CARTESIAN_POINT('Ctrl Pts',(-31.5482685418209,54.9161546038405,15.9805048787021));
#26329=CARTESIAN_POINT('Ctrl Pts',(-31.4391421648863,54.9965058030685,15.9895293940139));
#26330=CARTESIAN_POINT('Ctrl Pts',(-31.3423819730147,55.0896968084029,15.9985539093258));
#26331=CARTESIAN_POINT('Ctrl Pts',(-30.9451778667933,55.4722492740994,16.0355998728484));
#26332=CARTESIAN_POINT('Ctrl Pts',(-30.7563603461461,56.0711694668139,16.0726458363711));
#26333=CARTESIAN_POINT('Ctrl Pts',(-30.8623428200595,56.6123581642473,16.1096917998938));
#26334=CARTESIAN_POINT('Ctrl Pts',(-30.968325293973,57.1535468616808,16.1467377634165));
#26335=CARTESIAN_POINT('Ctrl Pts',(-31.3691077624472,57.6370040638332,16.1837837269392));
#26336=CARTESIAN_POINT('Ctrl Pts',(-31.8812698561966,57.8414728407482,16.2208296904618));
#26337=CARTESIAN_POINT('Ctrl Pts',(-32.393431949946,58.0459416176631,16.2578756539845));
#26338=CARTESIAN_POINT('Ctrl Pts',(-33.0169736689706,57.9714219693406,16.2949216175072));
#26339=CARTESIAN_POINT('Ctrl Pts',(-33.4665276098354,57.6520182353919,16.3319675810299));
#26340=CARTESIAN_POINT('Ctrl Pts',(-33.9160815507002,57.3326145014431,16.3690135445526));
#26341=CARTESIAN_POINT('Ctrl Pts',(-34.1916477134051,56.7683266818682,16.4060595080752));
#26342=CARTESIAN_POINT('Ctrl Pts',(-34.1671116810226,56.2174042970244,16.4431054715979));
#26343=CARTESIAN_POINT('Ctrl Pts',(-34.14257564864,55.6664819121806,16.4801514351206));
#26344=CARTESIAN_POINT('Ctrl Pts',(-33.81793742117,55.128924962068,16.5171973986433));
#26345=CARTESIAN_POINT('Ctrl Pts',(-33.3417695242377,54.8507494330611,16.554243362166));
#26346=CARTESIAN_POINT('Ctrl Pts',(-32.8656016273055,54.5725739040542,16.5912893256886));
#26347=CARTESIAN_POINT('Ctrl Pts',(-32.237904060911,54.5537797961531,16.6283352892113));
#26348=CARTESIAN_POINT('Ctrl Pts',(-31.7459461756022,54.8029683394084,16.665381252734));
#26349=CARTESIAN_POINT('Ctrl Pts',(-31.7189481323125,54.8166434999842,16.6674142896194));
#26350=CARTESIAN_POINT('Ctrl Pts',(-31.692358893413,54.8311257383683,16.6694473265048));
#26351=CARTESIAN_POINT('Ctrl Pts',(-31.6662054032747,54.8463759356941,16.6714803633902));
#26352=CARTESIAN_POINT('Origin',(-32.5,56.2916512459885,17.));
#26353=CARTESIAN_POINT('',(-31.6689051738235,54.8497998491797,17.3714803633902));
#26354=CARTESIAN_POINT('',(-31.6674096068672,54.8512474102517,17.1785196366098));
#26355=CARTESIAN_POINT('',(-31.667,54.8488529232836,17.));
#26356=CARTESIAN_POINT('Ctrl Pts',(-31.6674096068672,54.8512474102517,17.1785196366098));
#26357=CARTESIAN_POINT('Ctrl Pts',(-31.955812083246,54.6864945235477,17.156380408079));
#26358=CARTESIAN_POINT('Ctrl Pts',(-32.2922890124973,54.603384940747,17.1342411795483));
#26359=CARTESIAN_POINT('Ctrl Pts',(-32.6209875748239,54.6272788981025,17.1121019510175));
#26360=CARTESIAN_POINT('Ctrl Pts',(-33.1710047054118,54.6672610804705,17.0750559874948));
#26361=CARTESIAN_POINT('Ctrl Pts',(-33.6992424692084,55.0068523416601,17.0380100239722));
#26362=CARTESIAN_POINT('Ctrl Pts',(-33.9639498583003,55.4906368153745,17.0009640604495));
#26363=CARTESIAN_POINT('Ctrl Pts',(-34.2286572473923,55.9744212890889,16.9639180969268));
#26364=CARTESIAN_POINT('Ctrl Pts',(-34.2298342617796,56.602398975328,16.9268721334041));
#26365=CARTESIAN_POINT('Ctrl Pts',(-33.9669422341539,57.087172325109,16.8898261698814));
#26366=CARTESIAN_POINT('Ctrl Pts',(-33.7040502065281,57.57194567489,16.8527802063588));
#26367=CARTESIAN_POINT('Ctrl Pts',(-33.1770891368891,57.9135146882128,16.8157342428361));
#26368=CARTESIAN_POINT('Ctrl Pts',(-32.6272257468299,57.955558369302,16.7786882793134));
#26369=CARTESIAN_POINT('Ctrl Pts',(-32.0773623567706,57.9976020503911,16.7416423157907));
#26370=CARTESIAN_POINT('Ctrl Pts',(-31.5045966462911,57.7401203992467,16.704596352268));
#26371=CARTESIAN_POINT('Ctrl Pts',(-31.1710580905945,57.3009513535357,16.6675503887454));
#26372=CARTESIAN_POINT('Ctrl Pts',(-30.8375195348979,56.8617823078246,16.6305044252227));
#26373=CARTESIAN_POINT('Ctrl Pts',(-30.7432081339843,56.2409258675469,16.5934584617));
#26374=CARTESIAN_POINT('Ctrl Pts',(-30.9312860352641,55.7225205030902,16.5564124981773));
#26375=CARTESIAN_POINT('Ctrl Pts',(-31.063103598594,55.3591873762591,16.5304482109881));
#26376=CARTESIAN_POINT('Ctrl Pts',(-31.333634830935,55.0461796849558,16.504483923799));
#26377=CARTESIAN_POINT('Ctrl Pts',(-31.6687530214683,54.8490350969289,16.4785196366098));
#26378=CARTESIAN_POINT('Ctrl Pts',(-31.6662054032747,54.8463759356941,16.6714803633902));
#26379=CARTESIAN_POINT('Ctrl Pts',(-31.2157904412561,55.1090145744741,16.7064932900275));
#26380=CARTESIAN_POINT('Ctrl Pts',(-30.8946171228531,55.5994272993444,16.7415062166648));
#26381=CARTESIAN_POINT('Ctrl Pts',(-30.8403168439901,56.1177955929608,16.776519143302));
#26382=CARTESIAN_POINT('Ctrl Pts',(-30.7828636019099,56.6662631088463,16.8135651068247));
#26383=CARTESIAN_POINT('Ctrl Pts',(-31.0241753219725,57.2460269462056,16.8506110703474));
#26384=CARTESIAN_POINT('Ctrl Pts',(-31.4538143271609,57.5917548973867,16.8876570338701));
#26385=CARTESIAN_POINT('Ctrl Pts',(-31.8834533323493,57.9374828485678,16.9247029973928));
#26386=CARTESIAN_POINT('Ctrl Pts',(-32.5014196226634,58.0491749135707,16.9617489609154));
#26387=CARTESIAN_POINT('Ctrl Pts',(-33.0248974212339,57.8757145855096,16.9987949244381));
#26388=CARTESIAN_POINT('Ctrl Pts',(-33.5483752198042,57.7022542574486,17.0358408879608));
#26389=CARTESIAN_POINT('Ctrl Pts',(-33.9773645266309,57.2436415363237,17.0728868514835));
#26390=CARTESIAN_POINT('Ctrl Pts',(-34.1155359529098,56.7097631344687,17.1099328150062));
#26391=CARTESIAN_POINT('Ctrl Pts',(-34.2537073791887,56.1758847326138,17.1469787785289));
#26392=CARTESIAN_POINT('Ctrl Pts',(-34.1010609249198,55.5667406500288,17.1840247420515));
#26393=CARTESIAN_POINT('Ctrl Pts',(-33.7274561054636,55.1611091301906,17.2210707055742));
#26394=CARTESIAN_POINT('Ctrl Pts',(-33.3538512860073,54.7554776103524,17.2581166690969));
#26395=CARTESIAN_POINT('Ctrl Pts',(-32.7592881013638,54.5533586532611,17.2951626326196));
#26396=CARTESIAN_POINT('Ctrl Pts',(-32.2158717643875,54.6472531457219,17.3322085961422));
#26397=CARTESIAN_POINT('Ctrl Pts',(-32.023849765451,54.6804317730554,17.3452991852249));
#26398=CARTESIAN_POINT('Ctrl Pts',(-31.8382141569136,54.7505717682631,17.3583897743076));
#26399=CARTESIAN_POINT('Ctrl Pts',(-31.6689051738235,54.8497998491797,17.3714803633902));
#26400=CARTESIAN_POINT('Origin',(-32.5,56.2916512459885,17.));
#26401=CARTESIAN_POINT('',(-31.6668097556407,54.850936308364,18.0714803633902));
#26402=CARTESIAN_POINT('',(-31.6651356431699,54.8475732381352,17.8785196366098));
#26403=CARTESIAN_POINT('',(-31.667,54.8488529232836,17.));
#26404=CARTESIAN_POINT('Ctrl Pts',(-31.6651356431699,54.8475732381352,17.8785196366098));
#26405=CARTESIAN_POINT('Ctrl Pts',(-32.0953114189421,54.6031821110332,17.8453228558818));
#26406=CARTESIAN_POINT('Ctrl Pts',(-32.6432818971092,54.5571637547426,17.8121260751538));
#26407=CARTESIAN_POINT('Ctrl Pts',(-33.1039518347459,54.7360113496833,17.7789292944258));
#26408=CARTESIAN_POINT('Ctrl Pts',(-33.618036674644,54.9355964098305,17.7418833309031));
#26409=CARTESIAN_POINT('Ctrl Pts',(-34.0234021807399,55.4152172665963,17.7048373673804));
#26410=CARTESIAN_POINT('Ctrl Pts',(-34.1345305305902,55.9553727152466,17.6677914038577));
#26411=CARTESIAN_POINT('Ctrl Pts',(-34.2456588804405,56.4955281638969,17.6307454403351));
#26412=CARTESIAN_POINT('Ctrl Pts',(-34.062550074045,57.0962182044316,17.5936994768124));
#26413=CARTESIAN_POINT('Ctrl Pts',(-33.6690048949483,57.4825336336559,17.5566535132897));
#26414=CARTESIAN_POINT('Ctrl Pts',(-33.2754597158516,57.8688490628802,17.519607549767));
#26415=CARTESIAN_POINT('Ctrl Pts',(-32.6714781640536,58.040789880794,17.4825615862443));
#26416=CARTESIAN_POINT('Ctrl Pts',(-32.133475821543,57.9196663971084,17.4455156227217));
#26417=CARTESIAN_POINT('Ctrl Pts',(-31.5954734790324,57.7985429134228,17.408469659199));
#26418=CARTESIAN_POINT('Ctrl Pts',(-31.1234503458092,57.3843551281376,17.3714236956763));
#26419=CARTESIAN_POINT('Ctrl Pts',(-30.9334304853463,56.8666584297933,17.3343777321536));
#26420=CARTESIAN_POINT('Ctrl Pts',(-30.7434106248833,56.3489617314489,17.2973317686309));
#26421=CARTESIAN_POINT('Ctrl Pts',(-30.8353940371805,55.7277561200453,17.2602858051083));
#26422=CARTESIAN_POINT('Ctrl Pts',(-31.1672839920187,55.2873398661167,17.2232398415856));
#26423=CARTESIAN_POINT('Ctrl Pts',(-31.3008314863423,55.1101230316987,17.2083331065936));
#26424=CARTESIAN_POINT('Ctrl Pts',(-31.4732231075307,54.9621784491468,17.1934263716017));
#26425=CARTESIAN_POINT('Ctrl Pts',(-31.6674096068672,54.8512474102517,17.1785196366098));
#26426=CARTESIAN_POINT('Ctrl Pts',(-31.6689051738235,54.8497998491797,17.3714803633902));
#26427=CARTESIAN_POINT('Ctrl Pts',(-31.3590749545435,55.0313841780677,17.3954357378302));
#26428=CARTESIAN_POINT('Ctrl Pts',(-31.1039191289866,55.3103783149913,17.4193911122703));
#26429=CARTESIAN_POINT('Ctrl Pts',(-30.9643532196009,55.6385333911701,17.4433464867103));
#26430=CARTESIAN_POINT('Ctrl Pts',(-30.7485205010994,56.1460112021445,17.480392450233));
#26431=CARTESIAN_POINT('Ctrl Pts',(-30.8091245534054,56.7710588820805,17.5174384137557));
#26432=CARTESIAN_POINT('Ctrl Pts',(-31.1184295883325,57.2276198159938,17.5544843772783));
#26433=CARTESIAN_POINT('Ctrl Pts',(-31.4277346232597,57.6841807499072,17.591530340801));
#26434=CARTESIAN_POINT('Ctrl Pts',(-31.9857406408082,57.9722549377979,17.6285763043237));
#26435=CARTESIAN_POINT('Ctrl Pts',(-32.5370730229375,57.9600035940862,17.6656222678464));
#26436=CARTESIAN_POINT('Ctrl Pts',(-33.0884054050668,57.9477522503744,17.7026682313691));
#26437=CARTESIAN_POINT('Ctrl Pts',(-33.633064151777,57.6351753750601,17.7397141948917));
#26438=CARTESIAN_POINT('Ctrl Pts',(-33.9217830992111,57.1653255475623,17.7767601584144));
#26439=CARTESIAN_POINT('Ctrl Pts',(-34.2105020466451,56.6954757200644,17.8138061219371));
#26440=CARTESIAN_POINT('Ctrl Pts',(-34.2432811948029,56.0683529403831,17.8508520854598));
#26441=CARTESIAN_POINT('Ctrl Pts',(-34.0051189806597,55.5709635046674,17.8878980489825));
#26442=CARTESIAN_POINT('Ctrl Pts',(-33.7669567665165,55.0735740689517,17.9249440125051));
#26443=CARTESIAN_POINT('Ctrl Pts',(-33.2578531900722,54.7059179772018,17.9619899760278));
#26444=CARTESIAN_POINT('Ctrl Pts',(-32.7108023899003,54.6362551245587,17.9990359395505));
#26445=CARTESIAN_POINT('Ctrl Pts',(-32.3542113134731,54.5908459018627,18.0231840808304));
#26446=CARTESIAN_POINT('Ctrl Pts',(-31.9814965026906,54.6720536844457,18.0473322221103));
#26447=CARTESIAN_POINT('Ctrl Pts',(-31.6668097556407,54.850936308364,18.0714803633902));
#26448=CARTESIAN_POINT('Origin',(-32.5,56.2916512459885,17.));
#26449=CARTESIAN_POINT('',(-31.6652761166365,54.8468682178694,18.7714803633902));
#26450=CARTESIAN_POINT('',(-31.6679260143736,54.8475393267799,18.5785196366098));
#26451=CARTESIAN_POINT('',(-31.667,54.8488529232836,17.));
#26452=CARTESIAN_POINT('Ctrl Pts',(-31.6679260143736,54.8475393267799,18.5785196366098));
#26453=CARTESIAN_POINT('Ctrl Pts',(-31.7606663811944,54.7928563701908,18.5713112672072));
#26454=CARTESIAN_POINT('Ctrl Pts',(-31.8585183363754,54.7473751127227,18.5641028978046));
#26455=CARTESIAN_POINT('Ctrl Pts',(-31.9600503104883,54.7126554770058,18.5568945284021));
#26456=CARTESIAN_POINT('Ctrl Pts',(-32.4818534533784,54.5342208981905,18.5198485648794));
#26457=CARTESIAN_POINT('Ctrl Pts',(-33.1008546957744,54.6400264825866,18.4828026013567));
#26458=CARTESIAN_POINT('Ctrl Pts',(-33.533764609118,54.9816497045372,18.445756637834));
#26459=CARTESIAN_POINT('Ctrl Pts',(-33.9666745224615,55.3232729264878,18.4087106743114));
#26460=CARTESIAN_POINT('Ctrl Pts',(-34.2134931067525,55.9007137859928,18.3716647107887));
#26461=CARTESIAN_POINT('Ctrl Pts',(-34.1612624373338,56.4497031993872,18.334618747266));
#26462=CARTESIAN_POINT('Ctrl Pts',(-34.109031767915,56.9986926127816,18.2975727837433));
#26463=CARTESIAN_POINT('Ctrl Pts',(-33.7577518447865,57.5192305800653,18.2605268202206));
#26464=CARTESIAN_POINT('Ctrl Pts',(-33.2681879166606,57.7730899488601,18.223480856698));
#26465=CARTESIAN_POINT('Ctrl Pts',(-32.7786239885347,58.0269493176549,18.1864348931753));
#26466=CARTESIAN_POINT('Ctrl Pts',(-32.1507760554113,58.0141300879608,18.1493889296526));
#26467=CARTESIAN_POINT('Ctrl Pts',(-31.6719822840244,57.7404990529372,18.1123429661299));
#26468=CARTESIAN_POINT('Ctrl Pts',(-31.1931885126375,57.4668680179136,18.0752970026072));
#26469=CARTESIAN_POINT('Ctrl Pts',(-30.863448902987,56.9324251775604,18.0382510390845));
#26470=CARTESIAN_POINT('Ctrl Pts',(-30.8336706571803,56.3817613282624,18.0012050755619));
#26471=CARTESIAN_POINT('Ctrl Pts',(-30.8038924113735,55.8310974789644,17.9641591120392));
#26472=CARTESIAN_POINT('Ctrl Pts',(-31.0740755294104,55.2642126207216,17.9271131485165));
#26473=CARTESIAN_POINT('Ctrl Pts',(-31.520569175279,54.9405448233645,17.8900671849938));
#26474=CARTESIAN_POINT('Ctrl Pts',(-31.5669611569199,54.9069148027547,17.8862180021991));
#26475=CARTESIAN_POINT('Ctrl Pts',(-31.6152565537378,54.8759105076229,17.8823688194045));
#26476=CARTESIAN_POINT('Ctrl Pts',(-31.6651356431699,54.8475732381352,17.8785196366098));
#26477=CARTESIAN_POINT('Ctrl Pts',(-31.6668097556407,54.850936308364,18.0714803633902));
#26478=CARTESIAN_POINT('Ctrl Pts',(-31.4987316547814,54.9464797400044,18.084378185633));
#26479=CARTESIAN_POINT('Ctrl Pts',(-31.3472075724788,55.0698874675039,18.0972760078758));
#26480=CARTESIAN_POINT('Ctrl Pts',(-31.2235359810035,55.2167495878635,18.1101738301185));
#26481=CARTESIAN_POINT('Ctrl Pts',(-30.8683183961782,55.6385765173477,18.1472197936412));
#26482=CARTESIAN_POINT('Ctrl Pts',(-30.7428812504272,56.2538999898523,18.1842657571639));
#26483=CARTESIAN_POINT('Ctrl Pts',(-30.9046315647806,56.7811137290641,18.2213117206866));
#26484=CARTESIAN_POINT('Ctrl Pts',(-31.066381879134,57.3083274682759,18.2583576842093));
#26485=CARTESIAN_POINT('Ctrl Pts',(-31.5153196535918,57.7474314741949,18.295403647732));
#26486=CARTESIAN_POINT('Ctrl Pts',(-32.0459859700228,57.8974673086234,18.3324496112546));
#26487=CARTESIAN_POINT('Ctrl Pts',(-32.5766522864537,58.0475031430519,18.3694955747773));
#26488=CARTESIAN_POINT('Ctrl Pts',(-33.1890471448578,57.90847080599,18.4065415383));
#26489=CARTESIAN_POINT('Ctrl Pts',(-33.602904565772,57.5439992348605,18.4435875018227));
#26490=CARTESIAN_POINT('Ctrl Pts',(-34.0167619866863,57.179527663731,18.4806334653453));
#26491=CARTESIAN_POINT('Ctrl Pts',(-34.2320819701108,56.5896168585338,18.517679428868));
#26492=CARTESIAN_POINT('Ctrl Pts',(-34.1503221046824,56.0442428442903,18.5547253923907));
#26493=CARTESIAN_POINT('Ctrl Pts',(-34.068562239254,55.4988688300469,18.5917713559134));
#26494=CARTESIAN_POINT('Ctrl Pts',(-33.6897225249727,54.9980316067572,18.6288173194361));
#26495=CARTESIAN_POINT('Ctrl Pts',(-33.1871811052498,54.7709421695977,18.6658632829587));
#26496=CARTESIAN_POINT('Ctrl Pts',(-32.709603590725,54.5551334726087,18.7010689764359));
#26497=CARTESIAN_POINT('Ctrl Pts',(-32.120308963107,54.5865510549416,18.7362746699131));
#26498=CARTESIAN_POINT('Ctrl Pts',(-31.6652761166365,54.8468682178694,18.7714803633902));
#26499=CARTESIAN_POINT('Origin',(-32.5,56.2916512459885,17.));
#26500=CARTESIAN_POINT('',(-31.6684351372492,54.8482948457192,19.4714803633902));
#26501=CARTESIAN_POINT('',(-31.6684043758654,54.8511587229547,19.2785196366098));
#26502=CARTESIAN_POINT('',(-31.667,54.8488529232836,17.));
#26503=CARTESIAN_POINT('Ctrl Pts',(-31.6684043758654,54.8511587229547,19.2785196366098));
#26504=CARTESIAN_POINT('Ctrl Pts',(-31.9058262033729,54.7139758182214,19.26025371501));
#26505=CARTESIAN_POINT('Ctrl Pts',(-32.1752796610303,54.6323550853735,19.2419877934101));
#26506=CARTESIAN_POINT('Ctrl Pts',(-32.4470503478135,54.6237274947408,19.2237218718103));
#26507=CARTESIAN_POINT('Ctrl Pts',(-32.9982410936014,54.6062294776757,19.1866759082876));
#26508=CARTESIAN_POINT('Ctrl Pts',(-33.5589634784782,54.8889798390775,19.149629944765));
#26509=CARTESIAN_POINT('Ctrl Pts',(-33.8725997234821,55.3425762727761,19.1125839812423));
#26510=CARTESIAN_POINT('Ctrl Pts',(-34.186235968486,55.7961727064748,19.0755380177196));
#26511=CARTESIAN_POINT('Ctrl Pts',(-34.252786073617,56.4206152124703,19.0384920541969));
#26512=CARTESIAN_POINT('Ctrl Pts',(-34.0417930059025,56.9301241370495,19.0014460906742));
#26513=CARTESIAN_POINT('Ctrl Pts',(-33.830799938188,57.4396330616286,18.9644001271515));
#26514=CARTESIAN_POINT('Ctrl Pts',(-33.3422636976281,57.8342084047915,18.9273541636289));
#26515=CARTESIAN_POINT('Ctrl Pts',(-32.7997656649011,57.9332705233524,18.8903082001062));
#26516=CARTESIAN_POINT('Ctrl Pts',(-32.2572676321741,58.0323326419133,18.8532622365835));
#26517=CARTESIAN_POINT('Ctrl Pts',(-31.6608078072802,57.8358815358723,18.8162162730608));
#26518=CARTESIAN_POINT('Ctrl Pts',(-31.2833594112405,57.4338241678589,18.7791703095382));
#26519=CARTESIAN_POINT('Ctrl Pts',(-30.9059110152008,57.0317667998456,18.7421243460155));
#26520=CARTESIAN_POINT('Ctrl Pts',(-30.7474740480155,56.4241031698599,18.7050783824928));
#26521=CARTESIAN_POINT('Ctrl Pts',(-30.8805580861148,55.8889339838537,18.6680324189701));
#26522=CARTESIAN_POINT('Ctrl Pts',(-30.987746754868,55.4578975242981,18.63819482485));
#26523=CARTESIAN_POINT('Ctrl Pts',(-31.2840459342598,55.0738884180752,18.6083572307299));
#26524=CARTESIAN_POINT('Ctrl Pts',(-31.6679260143736,54.8475393267799,18.5785196366098));
#26525=CARTESIAN_POINT('Ctrl Pts',(-31.6652761166365,54.8468682178694,18.7714803633902));
#26526=CARTESIAN_POINT('Ctrl Pts',(-31.6414906650693,54.8604755020885,18.7733206334357));
#26527=CARTESIAN_POINT('Ctrl Pts',(-31.6180720645058,54.8747082214848,18.7751609034813));
#26528=CARTESIAN_POINT('Ctrl Pts',(-31.5950554470214,54.8895637585373,18.7770011735268));
#26529=CARTESIAN_POINT('Ctrl Pts',(-31.1317143336805,55.1886164356654,18.8140471370495));
#26530=CARTESIAN_POINT('Ctrl Pts',(-30.8312752321632,55.7400634409509,18.8510931005722));
#26531=CARTESIAN_POINT('Ctrl Pts',(-30.8312358008972,56.2915319254989,18.8881390640948));
#26532=CARTESIAN_POINT('Ctrl Pts',(-30.8311963696312,56.8430004100469,18.9251850276175));
#26533=CARTESIAN_POINT('Ctrl Pts',(-31.1315566086164,57.3944903738573,18.9622309911402));
#26534=CARTESIAN_POINT('Ctrl Pts',(-31.5948549512976,57.6936093078491,18.9992769546629));
#26535=CARTESIAN_POINT('Ctrl Pts',(-32.0581532939788,57.9927282418409,19.0363229181856));
#26536=CARTESIAN_POINT('Ctrl Pts',(-32.684389740356,58.039476146014,19.0733688817082));
#26537=CARTESIAN_POINT('Ctrl Pts',(-33.1869636297931,57.81245857691,19.1104148452309));
#26538=CARTESIAN_POINT('Ctrl Pts',(-33.6895375192301,57.585441007806,19.1474608087536));
#26539=CARTESIAN_POINT('Ctrl Pts',(-34.068448851727,57.0846579654247,19.1845067722763));
#26540=CARTESIAN_POINT('Ctrl Pts',(-34.150286707292,56.5392956488152,19.221552735799));
#26541=CARTESIAN_POINT('Ctrl Pts',(-34.2321245628569,55.9939333322058,19.2585986993216));
#26542=CARTESIAN_POINT('Ctrl Pts',(-34.01688894149,55.4039917413681,19.2956446628443));
#26543=CARTESIAN_POINT('Ctrl Pts',(-33.6030836459812,55.0394609904048,19.332690626367));
#26544=CARTESIAN_POINT('Ctrl Pts',(-33.1892783504725,54.6749302394415,19.3697365898897));
#26545=CARTESIAN_POINT('Ctrl Pts',(-32.5769033808219,54.5358103283526,19.4067825534124));
#26546=CARTESIAN_POINT('Ctrl Pts',(-32.0462156138869,54.685770273593,19.4438285169351));
#26547=CARTESIAN_POINT('Ctrl Pts',(-31.9141769673738,54.7230813054923,19.4530457990868));
#26548=CARTESIAN_POINT('Ctrl Pts',(-31.7871951467268,54.7782877536412,19.4622630812385));
#26549=CARTESIAN_POINT('Ctrl Pts',(-31.6684351372492,54.8482948457192,19.4714803633902));
#26550=CARTESIAN_POINT('Origin',(-32.5,56.2916512459885,17.));
#26551=CARTESIAN_POINT('',(-31.667931072794,54.8513178316736,20.1714803633902));
#26552=CARTESIAN_POINT('',(-31.6654871359732,54.8492158242279,19.9785196366098));
#26553=CARTESIAN_POINT('',(-31.667,54.8488529232836,17.));
#26554=CARTESIAN_POINT('Ctrl Pts',(-31.6654871359732,54.8492158242279,19.9785196366098));
#26555=CARTESIAN_POINT('Ctrl Pts',(-32.0469172461538,54.6336656790848,19.9491961628127));
#26556=CARTESIAN_POINT('Ctrl Pts',(-32.517553856985,54.5668303852667,19.9198726890156));
#26557=CARTESIAN_POINT('Ctrl Pts',(-32.9387102808403,54.6815870878529,19.8905492152186));
#26558=CARTESIAN_POINT('Ctrl Pts',(-33.4707804449504,54.8265655664402,19.8535032516959));
#26559=CARTESIAN_POINT('Ctrl Pts',(-33.9238769452873,55.2613769285398,19.8164572881732));
#26560=CARTESIAN_POINT('Ctrl Pts',(-34.0906375985399,55.7870272905994,19.7794113246505));
#26561=CARTESIAN_POINT('Ctrl Pts',(-34.2573982517925,56.312677652659,19.7423653611279));
#26562=CARTESIAN_POINT('Ctrl Pts',(-34.1378230579607,56.9291670146787,19.7053193976052));
#26563=CARTESIAN_POINT('Ctrl Pts',(-33.786636282889,57.3543555234679,19.6682734340825));
#26564=CARTESIAN_POINT('Ctrl Pts',(-33.4354495078173,57.779544032257,19.6312274705598));
#26565=CARTESIAN_POINT('Ctrl Pts',(-32.8526511515056,58.0134316878157,19.5941815070371));
#26566=CARTESIAN_POINT('Ctrl Pts',(-32.3049621862367,57.9489784788088,19.5571355435145));
#26567=CARTESIAN_POINT('Ctrl Pts',(-31.7572732209677,57.884525269802,19.5200895799918));
#26568=CARTESIAN_POINT('Ctrl Pts',(-31.2446936467415,57.5217311962296,19.4830436164691));
#26569=CARTESIAN_POINT('Ctrl Pts',(-31.0018084123139,57.0266310228123,19.4459976529464));
#26570=CARTESIAN_POINT('Ctrl Pts',(-30.7589231778862,56.531530849395,19.4089516894237));
#26571=CARTESIAN_POINT('Ctrl Pts',(-30.7857322832571,55.9041245761326,19.3719057259011));
#26572=CARTESIAN_POINT('Ctrl Pts',(-31.069966389292,55.4315482417354,19.3348597623784));
#26573=CARTESIAN_POINT('Ctrl Pts',(-31.2140557291191,55.1919808900508,19.3160797204555));
#26574=CARTESIAN_POINT('Ctrl Pts',(-31.4242999735977,54.9922028355067,19.2972996785326));
#26575=CARTESIAN_POINT('Ctrl Pts',(-31.6684043758654,54.8511587229547,19.2785196366098));
#26576=CARTESIAN_POINT('Ctrl Pts',(-31.6684351372492,54.8482948457192,19.4714803633902));
#26577=CARTESIAN_POINT('Ctrl Pts',(-31.3098766805411,55.0596592183268,19.4993090447612));
#26578=CARTESIAN_POINT('Ctrl Pts',(-31.0262639705086,55.405938549172,19.5271377261321));
#26579=CARTESIAN_POINT('Ctrl Pts',(-30.9047015762615,55.801960623025,19.5549664075031));
#26580=CARTESIAN_POINT('Ctrl Pts',(-30.7428758697907,56.329151225647,19.5920123710258));
#26581=CARTESIAN_POINT('Ctrl Pts',(-30.8682250210687,56.9444926293215,19.6290583345484));
#26582=CARTESIAN_POINT('Ctrl Pts',(-31.2233822786099,57.3663703525617,19.6661042980711));
#26583=CARTESIAN_POINT('Ctrl Pts',(-31.5785395361512,57.7882480758019,19.7031502615938));
#26584=CARTESIAN_POINT('Ctrl Pts',(-32.1635048999558,58.0166621186078,19.7401962251165));
#26585=CARTESIAN_POINT('Ctrl Pts',(-32.7105656575522,57.9470774968357,19.7772421886392));
#26586=CARTESIAN_POINT('Ctrl Pts',(-33.2576264151486,57.8774928750636,19.8142881521619));
#26587=CARTESIAN_POINT('Ctrl Pts',(-33.7667825665369,57.5099095887134,19.8513341156845));
#26588=CARTESIAN_POINT('Ctrl Pts',(-34.005015905411,57.0125542176421,19.8883800792072));
#26589=CARTESIAN_POINT('Ctrl Pts',(-34.243249244285,56.5151988465708,19.9254260427299));
#26590=CARTESIAN_POINT('Ctrl Pts',(-34.2105597706448,55.8880713907783,19.9624720062526));
#26591=CARTESIAN_POINT('Ctrl Pts',(-33.9219080204981,55.4181802774153,19.9995179697753));
#26592=CARTESIAN_POINT('Ctrl Pts',(-33.6332562703514,54.9482891640523,20.0365639332979));
#26593=CARTESIAN_POINT('Ctrl Pts',(-33.0886422436983,54.6356343931188,20.0736098968206));
#26594=CARTESIAN_POINT('Ctrl Pts',(-32.5373116119164,54.623304211516,20.1106558603433));
#26595=CARTESIAN_POINT('Ctrl Pts',(-32.235574629855,54.6165560434103,20.1309306946923));
#26596=CARTESIAN_POINT('Ctrl Pts',(-31.9318258577411,54.6997625487969,20.1512055290412));
#26597=CARTESIAN_POINT('Ctrl Pts',(-31.667931072794,54.8513178316736,20.1714803633902));
#26598=CARTESIAN_POINT('Origin',(-32.5,56.2916512459885,17.));
#26599=CARTESIAN_POINT('',(-31.6652099567911,54.8483531313949,20.8714803633902));
#26600=CARTESIAN_POINT('',(-31.666645377609,54.8465106721999,20.6785196366098));
#26601=CARTESIAN_POINT('',(-31.667,54.8488529232836,17.));
#26602=CARTESIAN_POINT('Ctrl Pts',(-31.666645377609,54.8465106721999,20.6785196366098));
#26603=CARTESIAN_POINT('Ctrl Pts',(-31.7095215140164,54.8213939588906,20.6751845741381));
#26604=CARTESIAN_POINT('Ctrl Pts',(-31.7535458686671,54.7983179269085,20.6718495116665));
#26605=CARTESIAN_POINT('Ctrl Pts',(-31.7985935167041,54.7774509892024,20.6685144491949));
#26606=CARTESIAN_POINT('Ctrl Pts',(-32.2989840011864,54.545660484627,20.6314684856722));
#26607=CARTESIAN_POINT('Ctrl Pts',(-32.9256368768597,54.5864462806581,20.5944225221495));
#26608=CARTESIAN_POINT('Ctrl Pts',(-33.3917609918081,54.881142287214,20.5573765586268));
#26609=CARTESIAN_POINT('Ctrl Pts',(-33.8578851067565,55.1758382937699,20.5203305951041));
#26610=CARTESIAN_POINT('Ctrl Pts',(-34.16348046098,55.7244445108505,20.4832846315815));
#26611=CARTESIAN_POINT('Ctrl Pts',(-34.168689562804,56.2758883119516,20.4462386680588));
#26612=CARTESIAN_POINT('Ctrl Pts',(-34.1738986646279,56.8273321130526,20.4091927045361));
#26613=CARTESIAN_POINT('Ctrl Pts',(-33.8787215140524,57.3816134981739,20.3721467410134));
#26614=CARTESIAN_POINT('Ctrl Pts',(-33.4182476302774,57.6850623886884,20.3351007774907));
#26615=CARTESIAN_POINT('Ctrl Pts',(-32.9577737465024,57.9885112792029,20.2980548139681));
#26616=CARTESIAN_POINT('Ctrl Pts',(-32.3320031295279,58.0411276751107,20.2610088504454));
#26617=CARTESIAN_POINT('Ctrl Pts',(-31.8273232393449,57.8188314143185,20.2239628869227));
#26618=CARTESIAN_POINT('Ctrl Pts',(-31.3226433491619,57.5965351535262,20.1869169234));
#26619=CARTESIAN_POINT('Ctrl Pts',(-30.9390541857702,57.0993262360341,20.1498709598773));
#26620=CARTESIAN_POINT('Ctrl Pts',(-30.8521075105052,56.5547551273836,20.1128249963547));
#26621=CARTESIAN_POINT('Ctrl Pts',(-30.7651608352402,56.0101840187331,20.075779032832));
#26622=CARTESIAN_POINT('Ctrl Pts',(-30.9748566481018,55.4182507189243,20.0387330693093));
#26623=CARTESIAN_POINT('Ctrl Pts',(-31.3852264684743,55.0498568665574,20.0016871057866));
#26624=CARTESIAN_POINT('Ctrl Pts',(-31.4707709224493,54.9730625961603,19.993964616061));
#26625=CARTESIAN_POINT('Ctrl Pts',(-31.5650355275691,54.9059820788927,19.9862421263354));
#26626=CARTESIAN_POINT('Ctrl Pts',(-31.6654871359732,54.8492158242279,19.9785196366098));
#26627=CARTESIAN_POINT('Ctrl Pts',(-31.667931072794,54.8513178316736,20.1714803633902));
#26628=CARTESIAN_POINT('Ctrl Pts',(-31.4496400894775,54.9766827635065,20.1882514925639));
#26629=CARTESIAN_POINT('Ctrl Pts',(-31.2586188937636,55.1488148264988,20.2050226217376));
#26630=CARTESIAN_POINT('Ctrl Pts',(-31.1185634357287,55.3554851247115,20.2217937509113));
#26631=CARTESIAN_POINT('Ctrl Pts',(-30.8091931282335,55.8120018117817,20.258839714434));
#26632=CARTESIAN_POINT('Ctrl Pts',(-30.7484997501537,56.4370407781941,20.2958856779567));
#26633=CARTESIAN_POINT('Ctrl Pts',(-30.9642598655732,56.9445494693264,20.3329316414794));
#26634=CARTESIAN_POINT('Ctrl Pts',(-31.1800199809926,57.4520581604587,20.3699776050021));
#26635=CARTESIAN_POINT('Ctrl Pts',(-31.6722335899114,57.842036576311,20.4070235685247));
#26636=CARTESIAN_POINT('Ctrl Pts',(-32.215636552448,57.9360087382767,20.4440695320474));
#26637=CARTESIAN_POINT('Ctrl Pts',(-32.7590395149846,58.0299809002424,20.4811154955701));
#26638=CARTESIAN_POINT('Ctrl Pts',(-33.353631831139,57.8279468083215,20.5181614590928));
#26639=CARTESIAN_POINT('Ctrl Pts',(-33.727294536927,57.4223688010744,20.5552074226155));
#26640=CARTESIAN_POINT('Ctrl Pts',(-34.1009572427151,57.0167907938272,20.5922533861381));
#26641=CARTESIAN_POINT('Ctrl Pts',(-34.2536903381367,56.4076688712538,20.6292993496608));
#26642=CARTESIAN_POINT('Ctrl Pts',(-34.1155954946062,55.8737705531045,20.6663453131835));
#26643=CARTESIAN_POINT('Ctrl Pts',(-33.9775006510756,55.3398722349553,20.7033912767062));
#26644=CARTESIAN_POINT('Ctrl Pts',(-33.5485778685929,54.8811975212302,20.7404372402289));
#26645=CARTESIAN_POINT('Ctrl Pts',(-33.0251244120732,54.707662660689,20.7774832037515));
#26646=CARTESIAN_POINT('Ctrl Pts',(-32.5824028716121,54.5608919787389,20.8088155902978));
#26647=CARTESIAN_POINT('Ctrl Pts',(-32.0720609029457,54.6180897881501,20.840147976844));
#26648=CARTESIAN_POINT('Ctrl Pts',(-31.6652099567911,54.8483531313949,20.8714803633902));
#26649=CARTESIAN_POINT('Origin',(-32.5,56.2916512459885,17.));
#26650=CARTESIAN_POINT('',(-31.6673136634551,54.8469650373412,21.5714803633902));
#26651=CARTESIAN_POINT('',(-31.6688940285233,54.8502492137286,21.3785196366098));
#26652=CARTESIAN_POINT('',(-31.667,54.8488529232836,17.));
#26653=CARTESIAN_POINT('',(-34.0692874532608,56.8510195406194,22.));
#26654=CARTESIAN_POINT('Ctrl Pts',(-31.6673136634551,54.8469650373412,21.5714803633902));
#26655=CARTESIAN_POINT('Ctrl Pts',(-31.2598491701087,55.0867590255674,21.6031823516921));
#26656=CARTESIAN_POINT('Ctrl Pts',(-30.9533734485755,55.5074467114501,21.634884339994));
#26657=CARTESIAN_POINT('Ctrl Pts',(-30.8625080737328,55.9706266060894,21.6665863282959));
#26658=CARTESIAN_POINT('Ctrl Pts',(-30.7563256056226,56.511884312636,21.7036322918186));
#26659=CARTESIAN_POINT('Ctrl Pts',(-30.9445706465323,57.1111674125324,21.7406782553412));
#26660=CARTESIAN_POINT('Ctrl Pts',(-31.341982566131,57.4936046161573,21.7777242188639));
#26661=CARTESIAN_POINT('Ctrl Pts',(-31.7393944857298,57.8760418197822,21.8147701823866));
#26662=CARTESIAN_POINT('Ctrl Pts',(-32.3459732840176,58.0416331271358,21.8518161459093));
#26663=CARTESIAN_POINT('Ctrl Pts',(-32.8819457094272,57.9158339106246,21.888862109432));
#26664=CARTESIAN_POINT('Ctrl Pts',(-33.4179181348368,57.7900346941134,21.9259080729547));
#26665=CARTESIAN_POINT('Ctrl Pts',(-33.8832841873681,57.3728449537375,21.9629540364773));
#26666=CARTESIAN_POINT('Ctrl Pts',(-34.0692874532608,56.8510195406194,22.));
#26667=CARTESIAN_POINT('',(-32.8006122403834,54.64991982209,22.));
#26668=CARTESIAN_POINT('Origin',(-32.5,56.2916512459885,22.));
#26669=CARTESIAN_POINT('Ctrl Pts',(-32.8006124898337,54.6499179279034,22.));
#26670=CARTESIAN_POINT('Ctrl Pts',(-33.3324299245223,54.7480089912901,21.9636770818144));
#26671=CARTESIAN_POINT('Ctrl Pts',(-33.8131824856956,55.1285995043637,21.9273541636289));
#26672=CARTESIAN_POINT('Ctrl Pts',(-34.0294057231266,55.6243031692819,21.8910312454433));
#26673=CARTESIAN_POINT('Ctrl Pts',(-34.2499331082255,56.1298743294735,21.8539852819206));
#26674=CARTESIAN_POINT('Ctrl Pts',(-34.195294888985,56.7551871483463,21.816939318398));
#26675=CARTESIAN_POINT('Ctrl Pts',(-33.8903094432865,57.2145585578539,21.7798933548753));
#26676=CARTESIAN_POINT('Ctrl Pts',(-33.585323997588,57.6739299673614,21.7428473913526));
#26677=CARTESIAN_POINT('Ctrl Pts',(-33.0299913254315,57.9673599675038,21.7058014278299));
#26678=CARTESIAN_POINT('Ctrl Pts',(-32.4785554363758,57.9603119672566,21.6687554643072));
#26679=CARTESIAN_POINT('Ctrl Pts',(-31.9271195473201,57.9532639670095,21.6317095007846));
#26680=CARTESIAN_POINT('Ctrl Pts',(-31.3795804413653,57.6457379663728,21.5946635372619));
#26681=CARTESIAN_POINT('Ctrl Pts',(-31.0864761391558,57.1785982034713,21.5576175737392));
#26682=CARTESIAN_POINT('Ctrl Pts',(-30.7933718369464,56.7114584405698,21.5205716102165));
#26683=CARTESIAN_POINT('Ctrl Pts',(-30.7547023384823,56.0847049154035,21.4835256466938));
#26684=CARTESIAN_POINT('Ctrl Pts',(-30.9881881185804,55.5851133656589,21.4464796831712));
#26685=CARTESIAN_POINT('Ctrl Pts',(-31.1309630480468,55.2796166101529,21.4238263343174));
#26686=CARTESIAN_POINT('Ctrl Pts',(-31.3755032965772,55.0216687358222,21.4011729854636));
#26687=CARTESIAN_POINT('Ctrl Pts',(-31.6688940285233,54.8502492137286,21.3785196366098));
#26688=CARTESIAN_POINT('Origin',(-32.5,56.2916512459885,23.5459252805377));
#26689=CARTESIAN_POINT('',(-31.4724222119036,54.5094432564574,13.4540747194623));
#26690=CARTESIAN_POINT('',(-31.4735006561134,54.5153050203083,13.3959252805377));
#26691=CARTESIAN_POINT('',(-31.4726250000001,54.5121855475624,23.5459252805377));
#26692=CARTESIAN_POINT('',(-32.7283737736498,58.3336705852723,13.));
#26693=CARTESIAN_POINT('Ctrl Pts',(-31.4735006561133,54.5153050203083,13.3959252805377));
#26694=CARTESIAN_POINT('Ctrl Pts',(-31.808029474343,54.3235252303772,13.3750880775931));
#26695=CARTESIAN_POINT('Ctrl Pts',(-32.8820600904465,54.0381232256078,13.3172049111259));
#26696=CARTESIAN_POINT('Ctrl Pts',(-34.5894859509232,55.0509345423224,13.2222757811361));
#26697=CARTESIAN_POINT('Ctrl Pts',(-34.6719801790384,57.3759588223509,13.111137890568));
#26698=CARTESIAN_POINT('Ctrl Pts',(-33.4073937856322,58.2577308722945,13.0370459635227));
#26699=CARTESIAN_POINT('Ctrl Pts',(-32.7283737736498,58.3336705852723,13.));
#26700=CARTESIAN_POINT('',(-31.6782144221994,58.1789827080509,13.));
#26701=CARTESIAN_POINT('Origin',(-32.5,56.2916512459885,13.));
#26702=CARTESIAN_POINT('Ctrl Pts',(-31.4724222119036,54.5094432564574,13.4540747194623));
#26703=CARTESIAN_POINT('Ctrl Pts',(-31.5342132308563,54.4731877432048,13.4501772883951));
#26704=CARTESIAN_POINT('Ctrl Pts',(-32.2034917270507,54.1282244537508,13.4092338938053));
#26705=CARTESIAN_POINT('Ctrl Pts',(-33.8288126996591,54.2585627611561,13.3312445356927));
#26706=CARTESIAN_POINT('Ctrl Pts',(-34.9285321027134,56.3058411531895,13.2201066451247));
#26707=CARTESIAN_POINT('Ctrl Pts',(-33.8129922329338,58.3256386597759,13.1096917998938));
#26708=CARTESIAN_POINT('Ctrl Pts',(-32.2900793461073,58.444463046046,13.0363229181856));
#26709=CARTESIAN_POINT('Ctrl Pts',(-31.6782133743559,58.178984818602,13.));
#26710=CARTESIAN_POINT('Origin',(-32.5,56.2916512459885,23.5459252805377));
#26711=CARTESIAN_POINT('',(-31.4749259905952,54.514117897405,14.1540747194623));
#26712=CARTESIAN_POINT('',(-31.470366790827,54.5112698283738,14.0959252805377));
#26713=CARTESIAN_POINT('',(-31.4726250000001,54.5121855475624,23.5459252805377));
#26714=CARTESIAN_POINT('Ctrl Pts',(-31.470366790827,54.5112698283738,14.0959252805377));
#26715=CARTESIAN_POINT('Ctrl Pts',(-31.9808629913117,54.2220900136561,14.0640305253959));
#26716=CARTESIAN_POINT('Ctrl Pts',(-33.371417583723,54.0779847124814,13.9950898067314));
#26717=CARTESIAN_POINT('Ctrl Pts',(-34.8602323505772,55.7191431963174,13.8891031245444));
#26718=CARTESIAN_POINT('Ctrl Pts',(-34.2609995597881,57.9641431697148,13.7779652339763));
#26719=CARTESIAN_POINT('Ctrl Pts',(-32.0500242237096,58.6781839861315,13.6668273434083));
#26720=CARTESIAN_POINT('Ctrl Pts',(-30.2506759606945,57.2080211780376,13.5556894528402));
#26721=CARTESIAN_POINT('Ctrl Pts',(-30.46190078674,55.3316416370552,13.4653887652167));
#26722=CARTESIAN_POINT('Ctrl Pts',(-31.2132787090688,54.6644859207873,13.4121340411158));
#26723=CARTESIAN_POINT('Ctrl Pts',(-31.4735006561133,54.5153050203083,13.3959252805377));
#26724=CARTESIAN_POINT('Ctrl Pts',(-31.4749259905952,54.514117897405,14.1540747194623));
#26725=CARTESIAN_POINT('Ctrl Pts',(-31.7139442620515,54.3746753634158,14.1391197361979));
#26726=CARTESIAN_POINT('Ctrl Pts',(-32.6363754616289,54.0511292553545,14.0871187894108));
#26727=CARTESIAN_POINT('Ctrl Pts',(-34.3667107654438,54.7380212138031,13.998071879101));
#26728=CARTESIAN_POINT('Ctrl Pts',(-34.817688121868,57.0173840749687,13.886933988533));
#26729=CARTESIAN_POINT('Ctrl Pts',(-33.1472639077745,58.6324557555082,13.7757960979649));
#26730=CARTESIAN_POINT('Ctrl Pts',(-30.8843823888258,58.105001931136,13.6646582073969));
#26731=CARTESIAN_POINT('Ctrl Pts',(-30.1278087167359,55.9943944231075,13.557417747896));
#26732=CARTESIAN_POINT('Ctrl Pts',(-30.9468756244448,54.8178045942286,13.4872232519178));
#26733=CARTESIAN_POINT('Ctrl Pts',(-31.4724222119036,54.5094432564574,13.4540747194623));
#26734=CARTESIAN_POINT('Origin',(-32.5,56.2916512459885,23.5459252805377));
#26735=CARTESIAN_POINT('',(-31.4717219617817,54.5141519916847,14.8540747194623));
#26736=CARTESIAN_POINT('',(-31.4732712326059,54.510037050691,14.7959252805377));
#26737=CARTESIAN_POINT('',(-31.4726250000001,54.5121855475624,23.5459252805377));
#26738=CARTESIAN_POINT('Ctrl Pts',(-31.4732712326059,54.510037050691,14.7959252805377));
#26739=CARTESIAN_POINT('Ctrl Pts',(-31.5669343623879,54.4548697514474,14.7900189367213));
#26740=CARTESIAN_POINT('Ctrl Pts',(-32.279281356511,54.1097268956778,14.7470666293823));
#26741=CARTESIAN_POINT('Ctrl Pts',(-33.9367458689222,54.3335587337424,14.6670683585206));
#26742=CARTESIAN_POINT('Ctrl Pts',(-34.9243151877952,56.4367817964587,14.5559304679526));
#26743=CARTESIAN_POINT('Ctrl Pts',(-33.6928803873875,58.4071660616143,14.4447925773845));
#26744=CARTESIAN_POINT('Ctrl Pts',(-31.3695905104292,58.4411939406326,14.3336546868165));
#26745=CARTESIAN_POINT('Ctrl Pts',(-30.0809735153022,56.5077243843662,14.2225167962484));
#26746=CARTESIAN_POINT('Ctrl Pts',(-30.7409078667025,54.9881078888109,14.1432736608222));
#26747=CARTESIAN_POINT('Ctrl Pts',(-31.3879183664803,54.55797423098,14.1010764889186));
#26748=CARTESIAN_POINT('Ctrl Pts',(-31.470366790827,54.5112698283738,14.0959252805377));
#26749=CARTESIAN_POINT('Ctrl Pts',(-31.4717219617817,54.5141519916847,14.8540747194623));
#26750=CARTESIAN_POINT('Ctrl Pts',(-31.8897217256655,54.2773643841942,14.8280621840006));
#26751=CARTESIAN_POINT('Ctrl Pts',(-33.1073033291158,54.0451479062597,14.7650036850163));
#26752=CARTESIAN_POINT('Ctrl Pts',(-34.7403671916158,55.3540375815297,14.6648992225092));
#26753=CARTESIAN_POINT('Ctrl Pts',(-34.5027924192342,57.6654005284895,14.5537613319412));
#26754=CARTESIAN_POINT('Ctrl Pts',(-32.4320391047204,58.7193548713018,14.4426234413732));
#26755=CARTESIAN_POINT('Ctrl Pts',(-30.4234910234841,57.5512051672244,14.3314855508051));
#26756=CARTESIAN_POINT('Ctrl Pts',(-30.3301141372088,55.5424943178044,14.2353026435015));
#26757=CARTESIAN_POINT('Ctrl Pts',(-31.12185652721,54.7200975505445,14.1761656997206));
#26758=CARTESIAN_POINT('Ctrl Pts',(-31.4749259905952,54.514117897405,14.1540747194623));
#26759=CARTESIAN_POINT('Origin',(-32.5,56.2916512459885,23.5459252805377));
#26760=CARTESIAN_POINT('',(-31.4709276972304,54.5092291784965,15.5540747194623));
#26761=CARTESIAN_POINT('',(-31.47464750201,54.5147506716574,15.4959252805377));
#26762=CARTESIAN_POINT('',(-31.4726250000001,54.5121855475624,23.5459252805377));
#26763=CARTESIAN_POINT('Ctrl Pts',(-31.47464750201,54.5147506716575,15.4959252805377));
#26764=CARTESIAN_POINT('Ctrl Pts',(-31.7462982414418,54.3571727743297,15.4789613845241));
#26765=CARTESIAN_POINT('Ctrl Pts',(-32.7191784117559,54.0441951966849,15.4249515249878));
#26766=CARTESIAN_POINT('Ctrl Pts',(-34.4479835200066,54.8412285476315,15.3338957019289));
#26767=CARTESIAN_POINT('Ctrl Pts',(-34.7750596076319,57.1416333665308,15.2227578113608));
#26768=CARTESIAN_POINT('Ctrl Pts',(-33.0197478209391,58.6640399241194,15.1116199207928));
#26769=CARTESIAN_POINT('Ctrl Pts',(-30.7887049884687,58.0149721937252,15.0004820302248));
#26770=CARTESIAN_POINT('Ctrl Pts',(-30.1593535158744,55.9068520254157,14.895250483473));
#26771=CARTESIAN_POINT('Ctrl Pts',(-30.9794574058775,54.8008918962759,14.827064900244));
#26772=CARTESIAN_POINT('Ctrl Pts',(-31.4732712326059,54.510037050691,14.7959252805377));
#26773=CARTESIAN_POINT('Ctrl Pts',(-31.4709277056121,54.5092291930958,15.5540747194623));
#26774=CARTESIAN_POINT('Ctrl Pts',(-31.4713112637463,54.5090077151575,15.5540505953261));
#26775=CARTESIAN_POINT('Ctrl Pts',(-32.0608222902466,54.1688851137838,15.5169805076671));
#26776=CARTESIAN_POINT('Ctrl Pts',(-33.6099012175602,54.1314466960921,15.4428644564855));
#26777=CARTESIAN_POINT('Ctrl Pts',(-34.916858119472,56.052567070093,15.3317265659175));
#26778=CARTESIAN_POINT('Ctrl Pts',(-34.0116373750326,58.1925239040739,15.2205886753494));
#26779=CARTESIAN_POINT('Ctrl Pts',(-31.722797799219,58.5925904319764,15.1094507847814));
#26780=CARTESIAN_POINT('Ctrl Pts',(-30.1453402095974,56.8865812380663,14.9983128942134));
#26781=CARTESIAN_POINT('Ctrl Pts',(-30.5878941637737,55.1627827650417,14.913187539107));
#26782=CARTESIAN_POINT('Ctrl Pts',(-31.2944239690072,54.6145873774176,14.8651081475233));
#26783=CARTESIAN_POINT('Ctrl Pts',(-31.4717219617817,54.5141519916847,14.8540747194623));
#26784=CARTESIAN_POINT('Origin',(-32.5,56.2916512459885,23.5459252805377));
#26785=CARTESIAN_POINT('',(-31.4747870773482,54.5124102302141,16.2540747194623));
#26786=CARTESIAN_POINT('',(-31.4710889776862,54.513282910156,16.1959252805377));
#26787=CARTESIAN_POINT('',(-31.4726250000001,54.5121855475624,23.5459252805377));
#26788=CARTESIAN_POINT('Ctrl Pts',(-31.4710889776862,54.513282910156,16.1959252805377));
#26789=CARTESIAN_POINT('Ctrl Pts',(-31.9210107047531,54.2589533662338,16.1679038323268));
#26790=CARTESIAN_POINT('Ctrl Pts',(-33.1965779324789,54.0532698651996,16.1028364205933));
#26791=CARTESIAN_POINT('Ctrl Pts',(-34.7877864833416,55.4765446163128,16.0007230453371));
#26792=CARTESIAN_POINT('Ctrl Pts',(-34.4255850063652,57.7716810411711,15.8895851547691));
#26793=CARTESIAN_POINT('Ctrl Pts',(-32.3008737352177,58.7121294100224,15.778447264201));
#26794=CARTESIAN_POINT('Ctrl Pts',(-30.3584249929228,57.4370866648374,15.667309373633));
#26795=CARTESIAN_POINT('Ctrl Pts',(-30.3734734150964,55.4682647699114,15.5731353790785));
#26796=CARTESIAN_POINT('Ctrl Pts',(-31.1530640353465,54.7012933131322,15.5160073480468));
#26797=CARTESIAN_POINT('Ctrl Pts',(-31.47464750201,54.5147506716575,15.4959252805377));
#26798=CARTESIAN_POINT('Ctrl Pts',(-31.4747870773482,54.5124102302141,16.2540747194623));
#26799=CARTESIAN_POINT('Ctrl Pts',(-31.6511921427898,54.4086339956355,16.2429930431288));
#26800=CARTESIAN_POINT('Ctrl Pts',(-32.4803377190683,54.0709860720282,16.1948654032726));
#26801=CARTESIAN_POINT('Ctrl Pts',(-34.1948158493603,54.5521215254953,16.1096917998938));
#26802=CARTESIAN_POINT('Ctrl Pts',(-34.880650639758,56.7721373989267,15.9985539093257));
#26803=CARTESIAN_POINT('Ctrl Pts',(-33.387448901162,58.5523588475275,15.8874160187577));
#26804=CARTESIAN_POINT('Ctrl Pts',(-31.0819551189948,58.2633289901972,15.7762781281897));
#26805=CARTESIAN_POINT('Ctrl Pts',(-30.074632599944,56.1700546084616,15.6651643617579));
#26806=CARTESIAN_POINT('Ctrl Pts',(-30.8823044490718,54.8491178663189,15.5910965588487));
#26807=CARTESIAN_POINT('Ctrl Pts',(-31.4709277056121,54.5092291930958,15.5540747194623));
#26808=CARTESIAN_POINT('Origin',(-32.5,56.2916512459885,23.5459252805377));
#26809=CARTESIAN_POINT('',(-31.4731301859007,54.5151387721107,16.9540747194623));
#26810=CARTESIAN_POINT('',(-31.471644989423,54.5091305714222,16.8959252805377));
#26811=CARTESIAN_POINT('',(-31.4726250000001,54.5121855475624,23.5459252805377));
#26812=CARTESIAN_POINT('Ctrl Pts',(-31.471644989423,54.5091305714222,16.8959252805377));
#26813=CARTESIAN_POINT('Ctrl Pts',(-31.5039012222331,54.4903218421575,16.8938922436523));
#26814=CARTESIAN_POINT('Ctrl Pts',(-32.1342604089221,54.1469870049404,16.8548132432442));
#26815=CARTESIAN_POINT('Ctrl Pts',(-33.72507894253,54.1946182477114,16.7786882793134));
#26816=CARTESIAN_POINT('Ctrl Pts',(-34.9262501272131,56.1835950962899,16.6675503887454));
#26817=CARTESIAN_POINT('Ctrl Pts',(-33.9066470549119,58.2714769641261,16.5564124981773));
#26818=CARTESIAN_POINT('Ctrl Pts',(-31.5995239807838,58.5472018994032,16.4452746076093));
#26819=CARTESIAN_POINT('Ctrl Pts',(-30.1166168191438,56.7583957419196,16.3341367170413));
#26820=CARTESIAN_POINT('Ctrl Pts',(-30.6391000228397,55.1011038763401,16.251020274684));
#26821=CARTESIAN_POINT('Ctrl Pts',(-31.3261883471228,54.5951916268687,16.2049497958495));
#26822=CARTESIAN_POINT('Ctrl Pts',(-31.4710889776862,54.513282910156,16.1959252805377));
#26823=CARTESIAN_POINT('Ctrl Pts',(-31.4731301859007,54.5151387721107,16.9540747194623));
#26824=CARTESIAN_POINT('Ctrl Pts',(-31.8288294586133,54.3119418969877,16.9319354909316));
#26825=CARTESIAN_POINT('Ctrl Pts',(-32.9382338021844,54.0379197452859,16.8727502988782));
#26826=CARTESIAN_POINT('Ctrl Pts',(-34.6305762357544,55.1258856969253,16.776519143302));
#26827=CARTESIAN_POINT('Ctrl Pts',(-34.6349312243122,57.4494219828794,16.665381252734));
#26828=CARTESIAN_POINT('Ctrl Pts',(-32.6851594514901,58.7132375833447,16.554243362166));
#26829=CARTESIAN_POINT('Ctrl Pts',(-30.5659091328683,57.7605477465697,16.4431054715979));
#26830=CARTESIAN_POINT('Ctrl Pts',(-30.2517487916384,55.6924152700813,16.3430492573634));
#26831=CARTESIAN_POINT('Ctrl Pts',(-31.0614712898343,54.7555571943486,16.2800390066515));
#26832=CARTESIAN_POINT('Ctrl Pts',(-31.4747870773482,54.5124102302141,16.2540747194623));
#26833=CARTESIAN_POINT('Origin',(-32.5,56.2916512459885,23.5459252805377));
#26834=CARTESIAN_POINT('',(-31.4703256079253,54.5106072564107,17.6540747194623));
#26835=CARTESIAN_POINT('',(-31.4749747334417,54.5133534323073,17.5959252805377));
#26836=CARTESIAN_POINT('',(-31.4726250000001,54.5121855475624,23.5459252805377));
#26837=CARTESIAN_POINT('Ctrl Pts',(-31.4749747334417,54.5133534323073,17.5959252805377));
#26838=CARTESIAN_POINT('Ctrl Pts',(-31.6837908396868,54.3909711398323,17.582834691455));
#26839=CARTESIAN_POINT('Ctrl Pts',(-32.560671629995,54.0596531620232,17.5326981388497));
#26840=CARTESIAN_POINT('Ctrl Pts',(-34.2863923370768,54.6463037965648,17.4455156227217));
#26841=CARTESIAN_POINT('Ctrl Pts',(-34.8511887990978,56.9001551837646,17.3343777321536));
#26842=CARTESIAN_POINT('Ctrl Pts',(-33.26391548901,58.5970360158137,17.2232398415856));
#26843=CARTESIAN_POINT('Ctrl Pts',(-30.9774216684405,58.1837720232006,17.1121019510176));
#26844=CARTESIAN_POINT('Ctrl Pts',(-30.1008940923714,56.0778693719696,17.0029970973349));
#26845=CARTESIAN_POINT('Ctrl Pts',(-30.9161286969814,54.8330541866883,16.9309382071749));
#26846=CARTESIAN_POINT('Ctrl Pts',(-31.471644989423,54.5091305714222,16.8959252805377));
#26847=CARTESIAN_POINT('Ctrl Pts',(-31.4703256079253,54.5106072564107,17.6540747194623));
#26848=CARTESIAN_POINT('Ctrl Pts',(-32.0008800348569,54.2091890880957,17.6208779387343));
#26849=CARTESIAN_POINT('Ctrl Pts',(-33.4309149924661,54.0890952859489,17.5506351944836));
#26850=CARTESIAN_POINT('Ctrl Pts',(-34.8788327758259,55.8022444250302,17.4433464867103));
#26851=CARTESIAN_POINT('Ctrl Pts',(-34.2013246967004,58.0248156029211,17.3322085961422));
#26852=CARTESIAN_POINT('Ctrl Pts',(-31.9665748283507,58.6610017894909,17.2210707055742));
#26853=CARTESIAN_POINT('Ctrl Pts',(-30.2200750690644,57.1284945533303,17.1099328150062));
#26854=CARTESIAN_POINT('Ctrl Pts',(-30.4926187339169,55.2878838417841,17.0209341529689));
#26855=CARTESIAN_POINT('Ctrl Pts',(-31.2336315607436,54.6519548298357,16.9689814544542));
#26856=CARTESIAN_POINT('Ctrl Pts',(-31.4731301859007,54.5151387721107,16.9540747194623));
#26857=CARTESIAN_POINT('Origin',(-32.5,56.2916512459885,23.5459252805377));
#26858=CARTESIAN_POINT('',(-31.4737670936581,54.5105654320665,18.3540747194623));
#26859=CARTESIAN_POINT('',(-31.4723903633871,54.5147550766703,18.2959252805377));
#26860=CARTESIAN_POINT('',(-31.4726250000001,54.5121855475624,23.5459252805377));
#26861=CARTESIAN_POINT('Ctrl Pts',(-31.4723903633871,54.5147550766704,18.2959252805377));
#26862=CARTESIAN_POINT('Ctrl Pts',(-31.8605071662086,54.2941313842958,18.2717771392578));
#26863=CARTESIAN_POINT('Ctrl Pts',(-33.02540146796,54.0403220897572,18.2105830344552));
#26864=CARTESIAN_POINT('Ctrl Pts',(-34.6904921906955,55.242790066521,18.1123429661299));
#26865=CARTESIAN_POINT('Ctrl Pts',(-34.5692083587435,57.5631631725538,18.0012050755619));
#26866=CARTESIAN_POINT('Ctrl Pts',(-32.5539546496148,58.7197069922753,17.8900671849939));
#26867=CARTESIAN_POINT('Ctrl Pts',(-30.4893156378063,57.6538238513956,17.7789292944258));
#26868=CARTESIAN_POINT('Ctrl Pts',(-30.2914909874078,55.613533902771,17.6808819929404));
#26869=CARTESIAN_POINT('Ctrl Pts',(-31.0928476967877,54.7373092545057,17.6198806549777));
#26870=CARTESIAN_POINT('Ctrl Pts',(-31.4749747334417,54.5133534323073,17.5959252805377));
#26871=CARTESIAN_POINT('Ctrl Pts',(-31.4737670936581,54.5105654320665,18.3540747194623));
#26872=CARTESIAN_POINT('Ctrl Pts',(-31.5881478071784,54.4431225718916,18.3468663500598));
#26873=CARTESIAN_POINT('Ctrl Pts',(-32.3290694209142,54.0987447143864,18.3026120171345));
#26874=CARTESIAN_POINT('Ctrl Pts',(-34.004501193851,54.3851254608372,18.2213117206866));
#26875=CARTESIAN_POINT('Ctrl Pts',(-34.9177373632483,56.5216739711636,18.1101738301186));
#26876=CARTESIAN_POINT('Ctrl Pts',(-33.6179911050581,58.4476800725015,17.9990359395505));
#26877=CARTESIAN_POINT('Ctrl Pts',(-31.2949349095266,58.4002485379024,17.8878980489825));
#26878=CARTESIAN_POINT('Ctrl Pts',(-30.0748884576731,56.4227939888947,17.7767601584144));
#26879=CARTESIAN_POINT('Ctrl Pts',(-30.7759689649703,54.951821535532,17.6988190485744));
#26880=CARTESIAN_POINT('Ctrl Pts',(-31.4088075653018,54.5455568389317,17.657923902257));
#26881=CARTESIAN_POINT('Ctrl Pts',(-31.4703256079253,54.5106072564107,17.6540747194623));
#26882=CARTESIAN_POINT('Origin',(-32.5,56.2916512459885,23.5459252805377));
#26883=CARTESIAN_POINT('',(-31.4743570776169,54.5150293902239,19.0540747194623));
#26884=CARTESIAN_POINT('',(-31.4704988599393,54.5097377243633,18.9959252805377));
#26885=CARTESIAN_POINT('',(-31.4726250000001,54.5121855475624,23.5459252805377));
#26886=CARTESIAN_POINT('Ctrl Pts',(-31.4704988599393,54.5097377243633,18.9959252805377));
#26887=CARTESIAN_POINT('Ctrl Pts',(-32.0317105894022,54.1886772858723,18.9607195870605));
#26888=CARTESIAN_POINT('Ctrl Pts',(-33.5233071799065,54.1091544860817,18.8884679300607));
#26889=CARTESIAN_POINT('Ctrl Pts',(-34.9018152245058,55.9315825877643,18.7791703095382));
#26890=CARTESIAN_POINT('Ctrl Pts',(-34.1051248236508,58.1142702713998,18.6680324189701));
#26891=CARTESIAN_POINT('Ctrl Pts',(-31.8392454683584,58.628694091168,18.5568945284021));
#26892=CARTESIAN_POINT('Ctrl Pts',(-30.1781622293418,57.0039960908762,18.445756637834));
#26893=CARTESIAN_POINT('Ctrl Pts',(-30.5414387587065,55.2219675363373,18.3587668885459));
#26894=CARTESIAN_POINT('Ctrl Pts',(-31.2650923575404,54.6325929315102,18.3088231027804));
#26895=CARTESIAN_POINT('Ctrl Pts',(-31.4723903633871,54.5147550766704,18.2959252805377));
#26896=CARTESIAN_POINT('Ctrl Pts',(-31.4743570776169,54.5150293902239,19.0540747194623));
#26897=CARTESIAN_POINT('Ctrl Pts',(-31.767179706711,54.3458357686749,19.0358087978625));
#26898=CARTESIAN_POINT('Ctrl Pts',(-32.7735194483881,54.0410032090046,18.98049691274));
#26899=CARTESIAN_POINT('Ctrl Pts',(-34.4976287681445,54.9104040861686,18.8881390640948));
#26900=CARTESIAN_POINT('Ctrl Pts',(-34.7438661544312,57.2208600991234,18.7770011735268));
#26901=CARTESIAN_POINT('Ctrl Pts',(-32.9362674024074,58.680800710823,18.6658632829587));
#26902=CARTESIAN_POINT('Ctrl Pts',(-30.7293481493446,57.9539257225797,18.5547253923907));
#26903=CARTESIAN_POINT('Ctrl Pts',(-30.1811487641285,55.8513808790735,18.4507958712252));
#26904=CARTESIAN_POINT('Ctrl Pts',(-31.0003111545141,54.7897315757275,18.3839123135824));
#26905=CARTESIAN_POINT('Ctrl Pts',(-31.4737670936581,54.5105654320665,18.3540747194623));
#26906=CARTESIAN_POINT('Origin',(-32.5,56.2916512459885,23.5459252805377));
#26907=CARTESIAN_POINT('',(-31.4707591192323,54.5126331290241,19.7540747194623));
#26908=CARTESIAN_POINT('',(-31.4743950169646,54.5114972463166,19.6959252805377));
#26909=CARTESIAN_POINT('',(-31.4726250000001,54.5121855475624,23.5459252805377));
#26910=CARTESIAN_POINT('Ctrl Pts',(-31.4743950169646,54.5114972463166,19.6959252805377));
#26911=CARTESIAN_POINT('Ctrl Pts',(-31.6208668833956,54.425154465736,19.686707998386));
#26912=CARTESIAN_POINT('Ctrl Pts',(-32.4069324234732,54.0834056527267,19.6404447527116));
#26913=CARTESIAN_POINT('Ctrl Pts',(-34.1053854498936,54.4692617796665,19.5571355435145));
#26914=CARTESIAN_POINT('Ctrl Pts',(-34.9017637086039,56.6520633710957,19.4459976529464));
#26915=CARTESIAN_POINT('Ctrl Pts',(-33.4997804064767,58.5049756574094,19.3348597623784));
#26916=CARTESIAN_POINT('Ctrl Pts',(-31.1826867602698,58.3320070089704,19.2237218718103));
#26917=CARTESIAN_POINT('Ctrl Pts',(-30.0713448616116,56.2914775915524,19.1125839812423));
#26918=CARTESIAN_POINT('Ctrl Pts',(-30.8308409091996,54.8974452606956,19.0366517841514));
#26919=CARTESIAN_POINT('Ctrl Pts',(-31.4411632317234,54.5265201776941,18.9977655505832));
#26920=CARTESIAN_POINT('Ctrl Pts',(-31.4704988599393,54.5097377243633,18.9959252805377));
#26921=CARTESIAN_POINT('Ctrl Pts',(-31.4707591192323,54.5126331290241,19.7540747194623));
#26922=CARTESIAN_POINT('Ctrl Pts',(-31.9411934042825,54.2467857936503,19.7247512456653));
#26923=CARTESIAN_POINT('Ctrl Pts',(-33.2549727142225,54.0602154670517,19.6583818083455));
#26924=CARTESIAN_POINT('Ctrl Pts',(-34.8149526935152,55.5572409773789,19.5549664075031));
#26925=CARTESIAN_POINT('Ctrl Pts',(-34.3725208876465,57.8382701189333,19.443828516935));
#26926=CARTESIAN_POINT('Ctrl Pts',(-32.2161494783462,58.7036614639378,19.332690626367));
#26927=CARTESIAN_POINT('Ctrl Pts',(-30.3195896701686,57.3613125035425,19.221552735799));
#26928=CARTESIAN_POINT('Ctrl Pts',(-30.4024811841689,55.4214247242036,19.1286807668307));
#26929=CARTESIAN_POINT('Ctrl Pts',(-31.1732925394658,54.6889852067103,19.0728547613852));
#26930=CARTESIAN_POINT('Ctrl Pts',(-31.4743570776169,54.5150293902239,19.0540747194623));
#26931=CARTESIAN_POINT('Origin',(-32.5,56.2916512459885,23.5459252805377));
#26932=CARTESIAN_POINT('',(-31.4721876288368,54.5092967477939,20.4540747194623));
#26933=CARTESIAN_POINT('',(-31.4737733324271,54.5152256259023,20.3959252805377));
#26934=CARTESIAN_POINT('',(-31.4726250000001,54.5121855475624,23.5459252805377));
#26935=CARTESIAN_POINT('Ctrl Pts',(-31.4737733324271,54.5152256259023,20.3959252805377));
#26936=CARTESIAN_POINT('Ctrl Pts',(-31.799246207199,54.3283059275284,20.3756504461887));
#26937=CARTESIAN_POINT('Ctrl Pts',(-32.8583863662624,54.0381735568298,20.318329648317));
#26938=CARTESIAN_POINT('Ctrl Pts',(-34.5693901517228,55.0204352512209,20.2239628869227));
#26939=CARTESIAN_POINT('Ctrl Pts',(-34.6903421852682,57.3408256590054,20.1128249963547));
#26940=CARTESIAN_POINT('Ctrl Pts',(-32.8064491443347,58.7008948504121,20.0016871057866));
#26941=CARTESIAN_POINT('Ctrl Pts',(-30.6420597422744,57.8557560368672,19.8905492152186));
#26942=CARTESIAN_POINT('Ctrl Pts',(-30.2167292658396,55.767800516413,19.7886286068022));
#26943=CARTESIAN_POINT('Ctrl Pts',(-31.0321693333385,54.7721820870222,19.7237539619086));
#26944=CARTESIAN_POINT('Ctrl Pts',(-31.4743950169646,54.5114972463166,19.6959252805377));
#26945=CARTESIAN_POINT('Ctrl Pts',(-31.4721876288368,54.5092967477939,20.4540747194623));
#26946=CARTESIAN_POINT('Ctrl Pts',(-31.5250686260056,54.4783192167782,20.4507396569907));
#26947=CARTESIAN_POINT('Ctrl Pts',(-32.182499910029,54.133716656297,20.4103586309964));
#26948=CARTESIAN_POINT('Ctrl Pts',(-33.7978345552325,54.2388509530007,20.3329316414794));
#26949=CARTESIAN_POINT('Ctrl Pts',(-34.9285465373885,56.2687104209715,20.2217937509113));
#26950=CARTESIAN_POINT('Ctrl Pts',(-33.8363822214011,58.3195681810162,20.1106558603433));
#26951=CARTESIAN_POINT('Ctrl Pts',(-31.5210121579647,58.5142504249981,19.9995179697753));
#26952=CARTESIAN_POINT('Ctrl Pts',(-30.101720741136,56.674562508041,19.8883800792072));
#26953=CARTESIAN_POINT('Ctrl Pts',(-30.6728871983316,55.0622630484846,19.8065656624362));
#26954=CARTESIAN_POINT('Ctrl Pts',(-31.3468677972825,54.5826454110005,19.7617972091879));
#26955=CARTESIAN_POINT('Ctrl Pts',(-31.4707591192323,54.5126331290241,19.7540747194623));
#26956=CARTESIAN_POINT('Origin',(-32.5,56.2916512459885,23.5459252805377));
#26957=CARTESIAN_POINT('',(-31.47496098746,54.5139076530798,21.1540747194623));
#26958=CARTESIAN_POINT('',(-31.4704172621348,54.5115691325664,21.0959252805377));
#26959=CARTESIAN_POINT('',(-31.4726250000001,54.5121855475624,23.5459252805377));
#26960=CARTESIAN_POINT('Ctrl Pts',(-31.4704172621348,54.5115691325664,21.0959252805377));
#26961=CARTESIAN_POINT('Ctrl Pts',(-31.9722041658629,54.227575372343,21.0645928939915));
#26962=CARTESIAN_POINT('Ctrl Pts',(-33.3458362247711,54.0736222398741,20.9962145439225));
#26963=CARTESIAN_POINT('Ctrl Pts',(-34.8512746399183,55.6834843462922,20.8907902303309));
#26964=CARTESIAN_POINT('Ctrl Pts',(-34.2861576030319,57.9372537407841,20.7796523397629));
#26965=CARTESIAN_POINT('Ctrl Pts',(-32.0861481883531,58.6847859443394,20.6685144491949));
#26966=CARTESIAN_POINT('Ctrl Pts',(-30.2649430630365,57.2418541016518,20.5573765586268));
#26967=CARTESIAN_POINT('Ctrl Pts',(-30.4485426703035,55.3510892045502,20.4665135024078));
#26968=CARTESIAN_POINT('Ctrl Pts',(-31.2045456025534,54.6698436293139,20.4126964097114));
#26969=CARTESIAN_POINT('Ctrl Pts',(-31.4737733324271,54.5152256259023,20.3959252805377));
#26970=CARTESIAN_POINT('Ctrl Pts',(-31.47496098746,54.5139076530797,21.1540747194623));
#26971=CARTESIAN_POINT('Ctrl Pts',(-31.70486029749,54.3795842898515,21.1396821047934));
#26972=CARTESIAN_POINT('Ctrl Pts',(-32.6134298152417,54.053477853398,21.0882435266019));
#26973=CARTESIAN_POINT('Ctrl Pts',(-34.3429657642117,54.7099453599152,20.9997589848876));
#26974=CARTESIAN_POINT('Ctrl Pts',(-34.8284152391772,56.982193672835,20.8886210943196));
#26975=CARTESIAN_POINT('Ctrl Pts',(-33.18263271582,58.6223996095027,20.7774832037515));
#26976=CARTESIAN_POINT('Ctrl Pts',(-30.9120322857352,58.129235673502,20.6663453131835));
#26977=CARTESIAN_POINT('Ctrl Pts',(-30.1194352615649,56.0193863503515,20.5585424850871));
#26978=CARTESIAN_POINT('Ctrl Pts',(-30.9376650889446,54.8224184634311,20.4877856205134));
#26979=CARTESIAN_POINT('Ctrl Pts',(-31.4721876288368,54.5092967477939,20.4540747194623));
#26980=CARTESIAN_POINT('Origin',(-32.5,56.2916512459885,23.5459252805377));
#26981=CARTESIAN_POINT('',(-31.4716734168817,54.5151354051885,21.8540747194623));
#26982=CARTESIAN_POINT('',(-31.4730118547325,54.5098571360137,21.7959252805377));
#26983=CARTESIAN_POINT('',(-31.4726250000001,54.5121855475624,23.5459252805377));
#26984=CARTESIAN_POINT('',(-30.5157034944334,56.8250975324092,22.));
#26985=CARTESIAN_POINT('Ctrl Pts',(-30.5157034944334,56.8250975324092,22.));
#26986=CARTESIAN_POINT('Ctrl Pts',(-30.3383199129809,56.1652717359214,21.9629540364773));
#26987=CARTESIAN_POINT('Ctrl Pts',(-30.5738806361657,55.1809621297242,21.9143122762981));
#26988=CARTESIAN_POINT('Ctrl Pts',(-31.2853315674048,54.6208532363719,21.8656705161189));
#26989=CARTESIAN_POINT('Ctrl Pts',(-31.4716734168817,54.5151354051885,21.8540747194623));
#26990=CARTESIAN_POINT('',(-31.043364830276,57.7461496994442,22.));
#26991=CARTESIAN_POINT('Origin',(-32.5,56.2916512459885,22.));
#26992=CARTESIAN_POINT('Ctrl Pts',(-31.0433632440414,57.7461514510325,22.));
#26993=CARTESIAN_POINT('Ctrl Pts',(-30.5726971034828,57.2735716615611,21.9636770818144));
#26994=CARTESIAN_POINT('Ctrl Pts',(-30.1593922934378,55.9189388685996,21.895652175327));
#26995=CARTESIAN_POINT('Ctrl Pts',(-30.9704682366631,54.8056054537255,21.8276272688396));
#26996=CARTESIAN_POINT('Ctrl Pts',(-31.4730118547325,54.5098571360137,21.7959252805377));
#26997=CARTESIAN_POINT('Origin',(-65.,8.88178419700125E-15,17.));
#26998=CARTESIAN_POINT('',(-63.3324486297716,0.0012143596160653,13.8714803633902));
#26999=CARTESIAN_POINT('',(-63.3320009243657,-0.000968828099756215,13.6785196366098));
#27000=CARTESIAN_POINT('',(-63.334,8.44655409538511E-15,17.));
#27001=CARTESIAN_POINT('',(-63.3648706727485,0.319230454628309,13.));
#27002=CARTESIAN_POINT('Ctrl Pts',(-63.3320009243657,-0.000968828099756215,
13.6785196366098));
#27003=CARTESIAN_POINT('Ctrl Pts',(-63.3315933114009,-0.0590548763034475,
13.6746222055426));
#27004=CARTESIAN_POINT('Ctrl Pts',(-63.3343634348107,-0.117102016123696,
13.6707247744754));
#27005=CARTESIAN_POINT('Ctrl Pts',(-63.3404396356832,-0.174801282227219,
13.6668273434083));
#27006=CARTESIAN_POINT('Ctrl Pts',(-63.3981952988365,-0.723245852641092,
13.6297813798856));
#27007=CARTESIAN_POINT('Ctrl Pts',(-63.7546528235523,-1.24026026815387,
13.5927354163629));
#27008=CARTESIAN_POINT('Ctrl Pts',(-64.2467810781753,-1.48913792445444,
13.5556894528402));
#27009=CARTESIAN_POINT('Ctrl Pts',(-64.7389093327983,-1.738015580755,13.5186434893175));
#27010=CARTESIAN_POINT('Ctrl Pts',(-65.3667083173286,-1.71875647784334,
13.4815975257948));
#27011=CARTESIAN_POINT('Ctrl Pts',(-65.8426564295865,-1.44035726535854,
13.4445515622722));
#27012=CARTESIAN_POINT('Ctrl Pts',(-66.3186045418444,-1.16195805287374,
13.4075055987495));
#27013=CARTESIAN_POINT('Ctrl Pts',(-66.6427017818299,-0.624418730815817,
13.3704596352268));
#27014=CARTESIAN_POINT('Ctrl Pts',(-66.6670336186705,-0.0733842827933133,
13.3334136717041));
#27015=CARTESIAN_POINT('Ctrl Pts',(-66.691365455511,0.477650165229191,13.2963677081814));
#27016=CARTESIAN_POINT('Ctrl Pts',(-66.4159318892067,1.04217973921627,13.2593217446588));
#27017=CARTESIAN_POINT('Ctrl Pts',(-65.9659478490025,1.36111593499209,13.2222757811361));
#27018=CARTESIAN_POINT('Ctrl Pts',(-65.5159638087983,1.68005213076791,13.1852298176134));
#27019=CARTESIAN_POINT('Ctrl Pts',(-64.8914292946943,1.75339494833248,13.1481838540907));
#27020=CARTESIAN_POINT('Ctrl Pts',(-64.3801939409253,1.54911937996348,13.111137890568));
#27021=CARTESIAN_POINT('Ctrl Pts',(-63.8689585871564,1.3448438115945,13.0740919270454));
#27022=CARTESIAN_POINT('Ctrl Pts',(-63.4710223937224,0.86294985729197,13.0370459635227));
#27023=CARTESIAN_POINT('Ctrl Pts',(-63.3648706727485,0.319230454628356,
13.));
#27024=CARTESIAN_POINT('',(-64.9474239245698,-1.66819769235426,13.));
#27025=CARTESIAN_POINT('Origin',(-65.,8.88178419700125E-15,13.));
#27026=CARTESIAN_POINT('',(-63.3365558121435,0.000651319618130558,13.1714803633902));
#27027=CARTESIAN_POINT('Ctrl Pts',(-64.9474239513002,-1.66819938802346,
13.));
#27028=CARTESIAN_POINT('Ctrl Pts',(-64.4069183000551,-1.65047139087789,
13.0363229181856));
#27029=CARTESIAN_POINT('Ctrl Pts',(-63.874833765777,-1.34577267304802,13.0726458363711));
#27030=CARTESIAN_POINT('Ctrl Pts',(-63.5871509129382,-0.887831743084588,
13.1089687545567));
#27031=CARTESIAN_POINT('Ctrl Pts',(-63.42211720178,-0.625126856723237,13.1298059575012));
#27032=CARTESIAN_POINT('Ctrl Pts',(-63.3375141386089,-0.311991178117355,
13.1506431604457));
#27033=CARTESIAN_POINT('Ctrl Pts',(-63.3365558121435,0.000651319618130558,
13.1714803633902));
#27034=CARTESIAN_POINT('',(-63.334,8.85460640886101E-15,12.));
#27035=CARTESIAN_POINT('',(-63.334,8.44655409538511E-15,17.));
#27036=CARTESIAN_POINT('Origin',(-65.,8.88178419700125E-15,12.));
#27037=CARTESIAN_POINT('Ctrl Pts',(-63.3365558121435,0.000651319618130558,
13.1714803633902));
#27038=CARTESIAN_POINT('Ctrl Pts',(-63.3358103529628,0.243848422696133,
13.1876891239684));
#27039=CARTESIAN_POINT('Ctrl Pts',(-63.385677580256,0.486747106414457,13.2038978845465));
#27040=CARTESIAN_POINT('Ctrl Pts',(-63.4876703201545,0.705378176395509,
13.2201066451247));
#27041=CARTESIAN_POINT('Ctrl Pts',(-63.7207800205315,1.20507083360909,13.2571526086474));
#27042=CARTESIAN_POINT('Ctrl Pts',(-64.2261802362228,1.57799560462436,13.2941985721701));
#27043=CARTESIAN_POINT('Ctrl Pts',(-64.7725065735009,1.65321436231665,13.3312445356927));
#27044=CARTESIAN_POINT('Ctrl Pts',(-65.318832910779,1.72843312000894,13.3682904992154));
#27045=CARTESIAN_POINT('Ctrl Pts',(-65.906085369644,1.50594586437825,13.4053364627381));
#27046=CARTESIAN_POINT('Ctrl Pts',(-66.265537296365,1.0877096323259,13.4423824262608));
#27047=CARTESIAN_POINT('Ctrl Pts',(-66.6249892230859,0.669473400273544,
13.4794283897835));
#27048=CARTESIAN_POINT('Ctrl Pts',(-66.7566406176629,0.0554881917995234,
13.5164743533061));
#27049=CARTESIAN_POINT('Ctrl Pts',(-66.6002239654009,-0.4733199493701,13.5535203168288));
#27050=CARTESIAN_POINT('Ctrl Pts',(-66.4438073131388,-1.00212809053972,
13.5905662803515));
#27051=CARTESIAN_POINT('Ctrl Pts',(-65.9993226140377,-1.44575916440495,
13.6276122438742));
#27052=CARTESIAN_POINT('Ctrl Pts',(-65.470199129815,-1.60114874218548,13.6646582073969));
#27053=CARTESIAN_POINT('Ctrl Pts',(-64.9410756455923,-1.75653831996601,
13.7017041709195));
#27054=CARTESIAN_POINT('Ctrl Pts',(-64.327313376248,-1.62368640166185,13.7387501344422));
#27055=CARTESIAN_POINT('Ctrl Pts',(-63.9097999122987,-1.26341063241475,
13.7757960979649));
#27056=CARTESIAN_POINT('Ctrl Pts',(-63.550341325322,-0.953230889441883,
13.8076908531067));
#27057=CARTESIAN_POINT('Ctrl Pts',(-63.3363495020968,-0.474476303274688,
13.8395856082484));
#27058=CARTESIAN_POINT('Ctrl Pts',(-63.3324486297716,0.0012143596160653,
13.8714803633902));
#27059=CARTESIAN_POINT('Origin',(-65.,8.88178419700125E-15,17.));
#27060=CARTESIAN_POINT('',(-63.3327604959513,-0.00132477262096475,14.5714803633902));
#27061=CARTESIAN_POINT('',(-63.3362968330887,-0.00083230422485394,14.3785196366098));
#27062=CARTESIAN_POINT('',(-63.334,8.44655409538511E-15,17.));
#27063=CARTESIAN_POINT('Ctrl Pts',(-63.3362968330887,-0.00083230422485394,
14.3785196366098));
#27064=CARTESIAN_POINT('Ctrl Pts',(-63.3352820110227,-0.225194784962803,
14.3635646533454));
#27065=CARTESIAN_POINT('Ctrl Pts',(-63.3774911908197,-0.449191325190206,
14.3486096700809));
#27066=CARTESIAN_POINT('Ctrl Pts',(-63.4647380475121,-0.654002427856251,
14.3336546868165));
#27067=CARTESIAN_POINT('Ctrl Pts',(-63.6808629212981,-1.16135335592135,
14.2966087232938));
#27068=CARTESIAN_POINT('Ctrl Pts',(-64.1733546191173,-1.55097577727798,
14.2595627597711));
#27069=CARTESIAN_POINT('Ctrl Pts',(-64.7168232236993,-1.64455527160812,
14.2225167962485));
#27070=CARTESIAN_POINT('Ctrl Pts',(-65.2602918282814,-1.73813476593826,
14.1854708327258));
#27071=CARTESIAN_POINT('Ctrl Pts',(-65.8547373396264,-1.53567133324192,
14.1484248692031));
#27072=CARTESIAN_POINT('Ctrl Pts',(-66.2281050246363,-1.12982650677501,
14.1113789056804));
#27073=CARTESIAN_POINT('Ctrl Pts',(-66.6014727096463,-0.723981680308087,
14.0743329421577));
#27074=CARTESIAN_POINT('Ctrl Pts',(-66.7537625683213,-0.114755460070592,
14.0372869786351));
#27075=CARTESIAN_POINT('Ctrl Pts',(-66.6152849767096,0.419042261543978,
14.0002410151124));
#27076=CARTESIAN_POINT('Ctrl Pts',(-66.4768073850979,0.952839983158533,
13.9631950515897));
#27077=CARTESIAN_POINT('Ctrl Pts',(-66.0475623431996,1.41120920615017,13.926149088067));
#27078=CARTESIAN_POINT('Ctrl Pts',(-65.5239830002582,1.58436286925844,13.8891031245443));
#27079=CARTESIAN_POINT('Ctrl Pts',(-65.0004036573169,1.75751653236672,13.8520571610217));
#27080=CARTESIAN_POINT('Ctrl Pts',(-64.3824900133324,1.64545463559163,13.815011197499));
#27081=CARTESIAN_POINT('Ctrl Pts',(-63.9530600921357,1.29948632454661,13.7779652339763));
#27082=CARTESIAN_POINT('Ctrl Pts',(-63.5688084672201,0.989915707487903,
13.7448167015208));
#27083=CARTESIAN_POINT('Ctrl Pts',(-63.3354677647952,0.493066145425921,
13.7116681690653));
#27084=CARTESIAN_POINT('Ctrl Pts',(-63.3320009243657,-0.000968828099756215,
13.6785196366098));
#27085=CARTESIAN_POINT('Ctrl Pts',(-63.3324486297716,0.0012143596160653,
13.8714803633902));
#27086=CARTESIAN_POINT('Ctrl Pts',(-63.3318186137667,0.0780414654682698,
13.8766315717711));
#27087=CARTESIAN_POINT('Ctrl Pts',(-63.3366686795385,0.154788650933419,
13.881782780152));
#27088=CARTESIAN_POINT('Ctrl Pts',(-63.3472710750459,0.230732838385412,
13.8869339885329));
#27089=CARTESIAN_POINT('Ctrl Pts',(-63.4235203602966,0.776900919748422,
13.9239799520556));
#27090=CARTESIAN_POINT('Ctrl Pts',(-63.7972835893523,1.28153746228441,13.9610259155783));
#27091=CARTESIAN_POINT('Ctrl Pts',(-64.2975048362999,1.51368831950506,13.998071879101));
#27092=CARTESIAN_POINT('Ctrl Pts',(-64.7977260832475,1.74583917672571,14.0351178426237));
#27093=CARTESIAN_POINT('Ctrl Pts',(-65.424405348087,1.70550434863099,14.0721638061464));
#27094=CARTESIAN_POINT('Ctrl Pts',(-65.8907398483472,1.41114550098829,14.109209769669));
#27095=CARTESIAN_POINT('Ctrl Pts',(-66.3570743486074,1.1167866533456,14.1462557331917));
#27096=CARTESIAN_POINT('Ctrl Pts',(-66.6630640842882,0.568403786154946,
14.1833016967144));
#27097=CARTESIAN_POINT('Ctrl Pts',(-66.6686708473517,0.0169663179122643,
14.2203476602371));
#27098=CARTESIAN_POINT('Ctrl Pts',(-66.6742776104151,-0.534471150330418,
14.2573936237598));
#27099=CARTESIAN_POINT('Ctrl Pts',(-66.3795014008612,-1.08896321962512,
14.2944395872824));
#27100=CARTESIAN_POINT('Ctrl Pts',(-65.9192483587705,-1.39274289076841,
14.3314855508051));
#27101=CARTESIAN_POINT('Ctrl Pts',(-65.4589953166798,-1.6965225619117,14.3685315143278));
#27102=CARTESIAN_POINT('Ctrl Pts',(-64.8332654420522,-1.74958983490357,
14.4055774778505));
#27103=CARTESIAN_POINT('Ctrl Pts',(-64.3284274914591,-1.5276584533176,14.4426234413732));
#27104=CARTESIAN_POINT('Ctrl Pts',(-63.823589540866,-1.30572707173164,14.4796694048958));
#27105=CARTESIAN_POINT('Ctrl Pts',(-63.4396435143075,-0.808797035567833,
14.5167153684185));
#27106=CARTESIAN_POINT('Ctrl Pts',(-63.352304522573,-0.264291051559223,
14.5537613319412));
#27107=CARTESIAN_POINT('Ctrl Pts',(-63.3383798175659,-0.177478906704707,
14.5596676757575));
#27108=CARTESIAN_POINT('Ctrl Pts',(-63.3319945181308,-0.0894574366348098,
14.5655740195739));
#27109=CARTESIAN_POINT('Ctrl Pts',(-63.3327604959513,-0.00132477262096475,
14.5714803633902));
#27110=CARTESIAN_POINT('Origin',(-65.,8.88178419700125E-15,17.));
#27111=CARTESIAN_POINT('',(-63.3366282199437,-0.000380246208307872,15.2714803633902));
#27112=CARTESIAN_POINT('',(-63.3350218272016,0.00143128727517339,15.0785196366098));
#27113=CARTESIAN_POINT('',(-63.334,8.44655409538511E-15,17.));
#27114=CARTESIAN_POINT('Ctrl Pts',(-63.3350218272016,0.00143128727517339,
15.0785196366098));
#27115=CARTESIAN_POINT('Ctrl Pts',(-63.3382129761596,-0.388071089145991,
15.0525071011481));
#27116=CARTESIAN_POINT('Ctrl Pts',(-63.4745702784036,-0.779586335762523,
15.0264945656864));
#27117=CARTESIAN_POINT('Ctrl Pts',(-63.7241632245643,-1.07563467970708,
15.0004820302248));
#27118=CARTESIAN_POINT('Ctrl Pts',(-64.0796230447962,-1.49725433177355,
14.9634360667021));
#27119=CARTESIAN_POINT('Ctrl Pts',(-64.6647503809125,-1.72524549701853,
14.9263901031794));
#27120=CARTESIAN_POINT('Ctrl Pts',(-65.2117584175496,-1.65526670109562,
14.8893441396567));
#27121=CARTESIAN_POINT('Ctrl Pts',(-65.7587664541868,-1.58528790517271,
14.852298176134));
#27122=CARTESIAN_POINT('Ctrl Pts',(-66.2676551913447,-1.21733914808191,
14.8152522126113));
#27123=CARTESIAN_POINT('Ctrl Pts',(-66.5055287575052,-0.719814314063376,
14.7782062490887));
#27124=CARTESIAN_POINT('Ctrl Pts',(-66.7434023236657,-0.222289480044837,
14.741160285566));
#27125=CARTESIAN_POINT('Ctrl Pts',(-66.7102607188288,0.40481143090144,14.7041143220433));
#27126=CARTESIAN_POINT('Ctrl Pts',(-66.4212714962,0.874492228471364,14.6670683585206));
#27127=CARTESIAN_POINT('Ctrl Pts',(-66.1322822735712,1.34417302604129,14.630022394998));
#27128=CARTESIAN_POINT('Ctrl Pts',(-65.5874454331506,1.65643371023486,14.5929764314753));
#27129=CARTESIAN_POINT('Ctrl Pts',(-65.0361084265221,1.66836621488623,14.5559304679526));
#27130=CARTESIAN_POINT('Ctrl Pts',(-64.4847714198936,1.68029871953761,14.5188845044299));
#27131=CARTESIAN_POINT('Ctrl Pts',(-63.9269342470572,1.39190304464679,14.4818385409072));
#27132=CARTESIAN_POINT('Ctrl Pts',(-63.6178946855153,0.935165489814596,
14.4447925773845));
#27133=CARTESIAN_POINT('Ctrl Pts',(-63.4336104557676,0.662807064022201,
14.4227015971263));
#27134=CARTESIAN_POINT('Ctrl Pts',(-63.3377958928888,0.330588135707235,
14.400610616868));
#27135=CARTESIAN_POINT('Ctrl Pts',(-63.3362968330887,-0.00083230422485394,
14.3785196366098));
#27136=CARTESIAN_POINT('Ctrl Pts',(-63.3327604959513,-0.00132477262096475,
14.5714803633902));
#27137=CARTESIAN_POINT('Ctrl Pts',(-63.336798909355,0.463331150982527,14.6026199830965));
#27138=CARTESIAN_POINT('Ctrl Pts',(-63.5396173640042,0.931077870254266,
14.6337596028029));
#27139=CARTESIAN_POINT('Ctrl Pts',(-63.8843359278475,1.24098501894125,14.6648992225092));
#27140=CARTESIAN_POINT('Ctrl Pts',(-64.294438281767,1.6096731735797,14.7019451860319));
#27141=CARTESIAN_POINT('Ctrl Pts',(-64.9053749465165,1.75496755100318,14.7389911495546));
#27142=CARTESIAN_POINT('Ctrl Pts',(-65.4375473020178,1.6103733915995,14.7760371130773));
#27143=CARTESIAN_POINT('Ctrl Pts',(-65.9697196575191,1.46577923219582,14.8130830766));
#27144=CARTESIAN_POINT('Ctrl Pts',(-66.4231277037722,1.03129653596499,14.8501290401226));
#27145=CARTESIAN_POINT('Ctrl Pts',(-66.5902666729806,0.505768754333094,
14.8871750036453));
#27146=CARTESIAN_POINT('Ctrl Pts',(-66.757405642189,-0.0197590272988146,
14.924220967168));
#27147=CARTESIAN_POINT('Ctrl Pts',(-66.6382755343526,-0.636331894331805,
14.9612669306907));
#27148=CARTESIAN_POINT('Ctrl Pts',(-66.2873969210692,-1.061771768796,14.9983128942134));
#27149=CARTESIAN_POINT('Ctrl Pts',(-65.9365183077858,-1.48721164326019,
15.0353588577361));
#27150=CARTESIAN_POINT('Ctrl Pts',(-65.3538911890554,-1.72151852515559,
15.0724048212587));
#27151=CARTESIAN_POINT('Ctrl Pts',(-64.8061581683602,-1.65746054599184,
15.1094507847814));
#27152=CARTESIAN_POINT('Ctrl Pts',(-64.2584251476649,-1.59340256682809,
15.1464967483041));
#27153=CARTESIAN_POINT('Ctrl Pts',(-63.7455862250048,-1.23097972660521,
15.1835427118268));
#27154=CARTESIAN_POINT('Ctrl Pts',(-63.5023450418969,-0.736056890900427,
15.2205886753495));
#27155=CARTESIAN_POINT('Ctrl Pts',(-63.390961297378,-0.509424385728733,
15.237552571363));
#27156=CARTESIAN_POINT('Ctrl Pts',(-63.336108421692,-0.25500848787214,15.2545164673766));
#27157=CARTESIAN_POINT('Ctrl Pts',(-63.3366282199437,-0.000380246208307872,
15.2714803633902));
#27158=CARTESIAN_POINT('Origin',(-65.,8.88178419700125E-15,17.));
#27159=CARTESIAN_POINT('',(-63.3341549687971,0.00152342623459117,15.9714803633902));
#27160=CARTESIAN_POINT('',(-63.3312431600774,-6.71117919643557E-6,15.7785196366098));
#27161=CARTESIAN_POINT('',(-63.334,8.44655409538511E-15,17.));
#27162=CARTESIAN_POINT('Ctrl Pts',(-63.3312431738575,-6.71114565062814E-6,
15.7785196366098));
#27163=CARTESIAN_POINT('Ctrl Pts',(-63.3312102147262,-0.551831913054096,
15.7414495489509));
#27164=CARTESIAN_POINT('Ctrl Pts',(-63.6320564203023,-1.10362622346452,
15.7043794612919));
#27165=CARTESIAN_POINT('Ctrl Pts',(-64.0958701387024,-1.40260423963279,
15.667309373633));
#27166=CARTESIAN_POINT('Ctrl Pts',(-64.5593820206073,-1.70138768959275,
15.6302634101103));
#27167=CARTESIAN_POINT('Ctrl Pts',(-65.1856492588609,-1.74768378931891,
15.5932174465876));
#27168=CARTESIAN_POINT('Ctrl Pts',(-65.6880571011575,-1.52030486584838,
15.556171483065));
#27169=CARTESIAN_POINT('Ctrl Pts',(-66.1904649434542,-1.29292594237784,
15.5191255195423));
#27170=CARTESIAN_POINT('Ctrl Pts',(-66.569013389794,-0.791871995710595,
15.4820795560196));
#27171=CARTESIAN_POINT('Ctrl Pts',(-66.6504575962853,-0.246453206514422,
15.4450335924969));
#27172=CARTESIAN_POINT('Ctrl Pts',(-66.7319018027767,0.29896558268175,15.4079876289742));
#27173=CARTESIAN_POINT('Ctrl Pts',(-66.5162417694196,0.888749214406848,
15.3709416654516));
#27174=CARTESIAN_POINT('Ctrl Pts',(-66.1021755351577,1.25297986690094,15.3338957019289));
#27175=CARTESIAN_POINT('Ctrl Pts',(-65.6881093008957,1.61721051939502,15.2968497384062));
#27176=CARTESIAN_POINT('Ctrl Pts',(-65.0756368657288,1.75588819265809,15.2598037748835));
#27177=CARTESIAN_POINT('Ctrl Pts',(-64.5450597089912,1.60554625999199,15.2227578113608));
#27178=CARTESIAN_POINT('Ctrl Pts',(-64.0144825522536,1.45520432732588,15.1857118478382));
#27179=CARTESIAN_POINT('Ctrl Pts',(-63.5658006739452,1.01584278873058,15.1486658843155));
#27180=CARTESIAN_POINT('Ctrl Pts',(-63.4043558869649,0.488537949988949,
15.1116199207928));
#27181=CARTESIAN_POINT('Ctrl Pts',(-63.3562726607889,0.331490340715371,
15.1005864927318));
#27182=CARTESIAN_POINT('Ctrl Pts',(-63.3336682754684,0.166641881842649,
15.0895530646708));
#27183=CARTESIAN_POINT('Ctrl Pts',(-63.3350218272016,0.00143128727517339,
15.0785196366098));
#27184=CARTESIAN_POINT('Ctrl Pts',(-63.3366282199437,-0.000380246208307872,
15.2714803633902));
#27185=CARTESIAN_POINT('Ctrl Pts',(-63.3372435634692,0.301051779472634,
15.2915624308993));
#27186=CARTESIAN_POINT('Ctrl Pts',(-63.4154588028067,0.602781386183106,
15.3116444984084));
#27187=CARTESIAN_POINT('Ctrl Pts',(-63.5693524834351,0.859067985064386,
15.3317265659175));
#27188=CARTESIAN_POINT('Ctrl Pts',(-63.8532445516371,1.33184719413771,15.3687725294402));
#27189=CARTESIAN_POINT('Ctrl Pts',(-64.3946721315968,1.64998278109767,15.4058184929629));
#27190=CARTESIAN_POINT('Ctrl Pts',(-64.9458478213867,1.66787819121185,15.4428644564855));
#27191=CARTESIAN_POINT('Ctrl Pts',(-65.4970235111765,1.68577360132602,15.4799104200082));
#27192=CARTESIAN_POINT('Ctrl Pts',(-66.0579473107965,1.4034288345944,15.5169563835309));
#27193=CARTESIAN_POINT('Ctrl Pts',(-66.3719092626235,0.950060574217461,
15.5540023470536));
#27194=CARTESIAN_POINT('Ctrl Pts',(-66.6858712144506,0.496692313840518,
15.5910483105763));
#27195=CARTESIAN_POINT('Ctrl Pts',(-66.7528713184848,-0.127699440181744,
15.6280942740989));
#27196=CARTESIAN_POINT('Ctrl Pts',(-66.542246597235,-0.637358260928825,
15.6651402376216));
#27197=CARTESIAN_POINT('Ctrl Pts',(-66.3316218759853,-1.1470170816759,15.7021862011443));
#27198=CARTESIAN_POINT('Ctrl Pts',(-65.8433723294516,-1.5419429691478,15.739232164667));
#27199=CARTESIAN_POINT('Ctrl Pts',(-65.3009481311498,-1.64139585163659,
15.7762781281897));
#27200=CARTESIAN_POINT('Ctrl Pts',(-64.7585239328481,-1.74084873412537,
15.8133240917123));
#27201=CARTESIAN_POINT('Ctrl Pts',(-64.1619250827784,-1.54482861163105,
15.850370055235));
#27202=CARTESIAN_POINT('Ctrl Pts',(-63.7841884276299,-1.14304520468471,
15.8874160187577));
#27203=CARTESIAN_POINT('Ctrl Pts',(-63.4984696309493,-0.839137521926598,
15.9154374669685));
#27204=CARTESIAN_POINT('Ctrl Pts',(-63.3379698006251,-0.417505232584549,
15.9434589151794));
#27205=CARTESIAN_POINT('Ctrl Pts',(-63.3341549687971,0.00152342623459117,
15.9714803633902));
#27206=CARTESIAN_POINT('Origin',(-65.,8.88178419700125E-15,17.));
#27207=CARTESIAN_POINT('',(-63.3314647116295,-0.000550350488415785,16.6714803633902));
#27208=CARTESIAN_POINT('',(-63.3350414063796,-0.00142706819227155,16.4785196366098));
#27209=CARTESIAN_POINT('',(-63.334,8.44655409538511E-15,17.));
#27210=CARTESIAN_POINT('Ctrl Pts',(-63.3350414063796,-0.00142706819227155,
16.4785196366098));
#27211=CARTESIAN_POINT('Ctrl Pts',(-63.3336871074336,-0.167365053879273,
16.4674379602763));
#27212=CARTESIAN_POINT('Ctrl Pts',(-63.3564935743301,-0.332939153110412,
16.4563562839428));
#27213=CARTESIAN_POINT('Ctrl Pts',(-63.4049919569221,-0.490610641878076,
16.4452746076093));
#27214=CARTESIAN_POINT('Ctrl Pts',(-63.5671216977971,-1.01770528403039,
16.4082286440866));
#27215=CARTESIAN_POINT('Ctrl Pts',(-64.0163740234165,-1.45648350908885,
16.3711826805639));
#27216=CARTESIAN_POINT('Ctrl Pts',(-64.5471460595228,-1.60613597431705,
16.3341367170413));
#27217=CARTESIAN_POINT('Ctrl Pts',(-65.0779180956292,-1.75578843954525,
16.2970907535186));
#27218=CARTESIAN_POINT('Ctrl Pts',(-65.6902098422225,-1.61631514494319,
16.2600447899959));
#27219=CARTESIAN_POINT('Ctrl Pts',(-66.1038025095515,-1.25154683464619,
16.2229988264732));
#27220=CARTESIAN_POINT('Ctrl Pts',(-66.5173951768805,-0.886778524349203,
16.1859528629505));
#27221=CARTESIAN_POINT('Ctrl Pts',(-66.7322887649452,-0.296715198357285,
16.1489068994279));
#27222=CARTESIAN_POINT('Ctrl Pts',(-66.6501360046234,0.248597316289499,
16.1118609359052));
#27223=CARTESIAN_POINT('Ctrl Pts',(-66.5679832443015,0.793909830936282,
16.0748149723825));
#27224=CARTESIAN_POINT('Ctrl Pts',(-66.1887841355932,1.29447153423794,16.0377690088598));
#27225=CARTESIAN_POINT('Ctrl Pts',(-65.6860813008334,1.5211975243268,16.0007230453371));
#27226=CARTESIAN_POINT('Ctrl Pts',(-65.1833784660736,1.74792351441566,15.9636770818144));
#27227=CARTESIAN_POINT('Ctrl Pts',(-64.5571719052625,1.70081379129174,15.9266311182918));
#27228=CARTESIAN_POINT('Ctrl Pts',(-64.0940486017292,1.40142838682092,15.8895851547691));
#27229=CARTESIAN_POINT('Ctrl Pts',(-63.631226881651,1.10223794054802,15.8525633153827));
#27230=CARTESIAN_POINT('Ctrl Pts',(-63.3312760900911,0.551100267138441,
15.8155414759962));
#27231=CARTESIAN_POINT('Ctrl Pts',(-63.3312431738575,-6.71114565062814E-6,
15.7785196366098));
#27232=CARTESIAN_POINT('Ctrl Pts',(-63.3341549687971,0.00152342623459117,
15.9714803633902));
#27233=CARTESIAN_POINT('Ctrl Pts',(-63.3329263739013,0.136474714946144,
15.980504878702));
#27234=CARTESIAN_POINT('Ctrl Pts',(-63.3479493008663,0.271155952543891,
15.9895293940139));
#27235=CARTESIAN_POINT('Ctrl Pts',(-63.3802748445461,0.401547681148712,
15.9985539093257));
#27236=CARTESIAN_POINT('Ctrl Pts',(-63.5129723768379,0.936810468637382,
16.0355998728484));
#27237=CARTESIAN_POINT('Ctrl Pts',(-63.9372419016487,1.39978935221635,16.0726458363711));
#27238=CARTESIAN_POINT('Ctrl Pts',(-64.4589140651794,1.57859942055654,16.1096917998938));
#27239=CARTESIAN_POINT('Ctrl Pts',(-64.9805862287101,1.75740948889675,16.1467377634165));
#27240=CARTESIAN_POINT('Ctrl Pts',(-65.5996610309607,1.65205074199819,16.1837837269391));
#27241=CARTESIAN_POINT('Ctrl Pts',(-66.0328153782871,1.31074120779884,16.2208296904618));
#27242=CARTESIAN_POINT('Ctrl Pts',(-66.4659697256135,0.969431673599491,
16.2578756539845));
#27243=CARTESIAN_POINT('Ctrl Pts',(-66.7132036180157,0.392171352099354,
16.2949216175072));
#27244=CARTESIAN_POINT('Ctrl Pts',(-66.661369062725,-0.156853297275919,
16.3319675810299));
#27245=CARTESIAN_POINT('Ctrl Pts',(-66.6095345074342,-0.705877946651196,
16.3690135445526));
#27246=CARTESIAN_POINT('Ctrl Pts',(-66.2586315044505,-1.22666692390161,
16.4060595080752));
#27247=CARTESIAN_POINT('Ctrl Pts',(-65.7692528028443,-1.4808782005154,16.4431054715979));
#27248=CARTESIAN_POINT('Ctrl Pts',(-65.2798741012382,-1.73508947712918,
16.4801514351206));
#27249=CARTESIAN_POINT('Ctrl Pts',(-64.6520197010096,-1.72272305310635,
16.5171973986433));
#27250=CARTESIAN_POINT('Ctrl Pts',(-64.1730307286,-1.44943849252271,16.5542433621659));
#27251=CARTESIAN_POINT('Ctrl Pts',(-63.6940417561904,-1.17615393193907,
16.5912893256886));
#27252=CARTESIAN_POINT('Ctrl Pts',(-63.3639182115997,-0.641951234794631,
16.6283352892113));
#27253=CARTESIAN_POINT('Ctrl Pts',(-63.3337430069376,-0.0913112945731656,
16.665381252734));
#27254=CARTESIAN_POINT('Ctrl Pts',(-63.3320870288426,-0.0610928523301586,
16.6674142896194));
#27255=CARTESIAN_POINT('Ctrl Pts',(-63.3313343989597,-0.0308249063821139,
16.6694473265048));
#27256=CARTESIAN_POINT('Ctrl Pts',(-63.3314647116295,-0.000550350488415785,
16.6714803633902));
#27257=CARTESIAN_POINT('Origin',(-65.,8.88178419700125E-15,17.));
#27258=CARTESIAN_POINT('',(-63.3357797744869,-0.00117646094452181,17.3714803633902));
#27259=CARTESIAN_POINT('',(-63.3362856132907,0.000842509924184317,17.1785196366098));
#27260=CARTESIAN_POINT('',(-63.334,8.44655409538511E-15,17.));
#27261=CARTESIAN_POINT('Ctrl Pts',(-63.3362856132907,0.000842509924184317,
17.1785196366098));
#27262=CARTESIAN_POINT('Ctrl Pts',(-63.3378066597351,-0.331296382409449,
17.156380408079));
#27263=CARTESIAN_POINT('Ctrl Pts',(-63.4340697022003,-0.664247316775257,
17.1342411795483));
#27264=CARTESIAN_POINT('Ctrl Pts',(-63.6191109651628,-0.936960475618677,
17.1121019510176));
#27265=CARTESIAN_POINT('Ctrl Pts',(-63.9287437903708,-1.39329623820573,
17.0750559874949));
#27266=CARTESIAN_POINT('Ctrl Pts',(-64.4869549413411,-1.68096669861506,
17.0380100239722));
#27267=CARTESIAN_POINT('Ctrl Pts',(-65.0382759195595,-1.66831783943795,
17.0009640604495));
#27268=CARTESIAN_POINT('Ctrl Pts',(-65.5895968977779,-1.65566898026084,
16.9639180969268));
#27269=CARTESIAN_POINT('Ctrl Pts',(-66.1340277032444,-1.34270080149728,
16.9268721334041));
#27270=CARTESIAN_POINT('Ctrl Pts',(-66.4224064907048,-0.872644964808584,
16.8898261698815));
#27271=CARTESIAN_POINT('Ctrl Pts',(-66.7107852781652,-0.402589128119889,
16.8527802063588));
#27272=CARTESIAN_POINT('Ctrl Pts',(-66.7431120476195,0.224554366493944,
16.8157342428361));
#27273=CARTESIAN_POINT('Ctrl Pts',(-66.5045922697214,0.721769742577195,
16.7786882793134));
#27274=CARTESIAN_POINT('Ctrl Pts',(-66.2660724918233,1.21898511866045,16.7416423157907));
#27275=CARTESIAN_POINT('Ctrl Pts',(-65.7567061665729,1.58627237621312,16.7045963522681));
#27276=CARTESIAN_POINT('Ctrl Pts',(-65.2096076810249,1.65554041915625,16.6675503887454));
#27277=CARTESIAN_POINT('Ctrl Pts',(-64.6625091954769,1.72480846209939,16.6305044252227));
#27278=CARTESIAN_POINT('Ctrl Pts',(-64.0776785496314,1.496057290433,16.5934584617));
#27279=CARTESIAN_POINT('Ctrl Pts',(-63.7227668047739,1.07397617497671,16.5564124981773));
#27280=CARTESIAN_POINT('Ctrl Pts',(-63.4740209335901,0.778153519638634,
16.5304482109881));
#27281=CARTESIAN_POINT('Ctrl Pts',(-63.338214518977,0.387364427454228,16.504483923799));
#27282=CARTESIAN_POINT('Ctrl Pts',(-63.3350414063796,-0.00142706819227155,
16.4785196366098));
#27283=CARTESIAN_POINT('Ctrl Pts',(-63.3314647116295,-0.000550350488415785,
16.6714803633902));
#27284=CARTESIAN_POINT('Ctrl Pts',(-63.3337089542098,0.520837535827173,
16.7064932900275));
#27285=CARTESIAN_POINT('Ctrl Pts',(-63.5978310421932,1.04418591019568,16.7415062166648));
#27286=CARTESIAN_POINT('Ctrl Pts',(-64.0195992076647,1.35039416683957,16.776519143302));
#27287=CARTESIAN_POINT('Ctrl Pts',(-64.4658574777874,1.67438250473234,16.8135651068247));
#27288=CARTESIAN_POINT('Ctrl Pts',(-65.0886008827663,1.75528199721941,16.8506110703474));
#27289=CARTESIAN_POINT('Ctrl Pts',(-65.6028273721175,1.55606853283267,16.8876570338701));
#27290=CARTESIAN_POINT('Ctrl Pts',(-66.1170538614687,1.35685506844593,16.9247029973928));
#27291=CARTESIAN_POINT('Ctrl Pts',(-66.5227634351922,0.877528647185364,
16.9617489609154));
#27292=CARTESIAN_POINT('Ctrl Pts',(-66.6342808063438,0.337455723706583,
16.9987949244381));
#27293=CARTESIAN_POINT('Ctrl Pts',(-66.7457981774953,-0.202617199772189,
17.0358408879608));
#27294=CARTESIAN_POINT('Ctrl Pts',(-66.5631233460748,-0.803436625469172,
17.0728868514835));
#27295=CARTESIAN_POINT('Ctrl Pts',(-66.1698584845187,-1.1900341363363,17.1099328150062));
#27296=CARTESIAN_POINT('Ctrl Pts',(-65.7765936229625,-1.57663164720343,
17.1469787785288));
#27297=CARTESIAN_POINT('Ctrl Pts',(-65.1727387312707,-1.74900724324071,
17.1840247420515));
#27298=CARTESIAN_POINT('Ctrl Pts',(-64.6346514247161,-1.62827225548556,
17.2210707055742));
#27299=CARTESIAN_POINT('Ctrl Pts',(-64.0965641181614,-1.50753726773041,
17.2581166690969));
#27300=CARTESIAN_POINT('Ctrl Pts',(-63.624244396744,-1.09369169618283,17.2951626326196));
#27301=CARTESIAN_POINT('Ctrl Pts',(-63.4338520592054,-0.57613431332557,
17.3322085961422));
#27302=CARTESIAN_POINT('Ctrl Pts',(-63.3665748819314,-0.393249853550889,
17.3452991852249));
#27303=CARTESIAN_POINT('Ctrl Pts',(-63.334500232668,-0.197415541610626,
17.3583897743076));
#27304=CARTESIAN_POINT('Ctrl Pts',(-63.3357797744869,-0.00117646094452181,
17.3714803633902));
#27305=CARTESIAN_POINT('Origin',(-65.,8.88178419700125E-15,17.));
#27306=CARTESIAN_POINT('',(-63.3357162681914,0.001206443822575,18.0714803633902));
#27307=CARTESIAN_POINT('',(-63.331966723543,0.00097473362895843,17.8785196366098));
#27308=CARTESIAN_POINT('',(-63.334,8.44655409538511E-15,17.));
#27309=CARTESIAN_POINT('Ctrl Pts',(-63.331966723543,0.00097473362895843,
17.8785196366098));
#27310=CARTESIAN_POINT('Ctrl Pts',(-63.3354056721751,-0.493761861582906,
17.8453228558818));
#27311=CARTESIAN_POINT('Ctrl Pts',(-63.569536843221,-0.991325263991029,
17.8121260751538));
#27312=CARTESIAN_POINT('Ctrl Pts',(-63.9547567233169,-1.30085201001266,
17.7789292944258));
#27313=CARTESIAN_POINT('Ctrl Pts',(-64.3846430349799,-1.64626853206535,
17.7418833309031));
#27314=CARTESIAN_POINT('Ctrl Pts',(-65.002686987972,-1.75751445347198,17.7048373673804));
#27315=CARTESIAN_POINT('Ctrl Pts',(-65.5260372626587,-1.58367744749353,
17.6677914038578));
#27316=CARTESIAN_POINT('Ctrl Pts',(-66.0493875373455,-1.40984044151509,
17.6307454403351));
#27317=CARTESIAN_POINT('Ctrl Pts',(-66.4780441337267,-0.95092050815156,
17.5936994768124));
#27318=CARTESIAN_POINT('Ctrl Pts',(-66.6158299298206,-0.416944957159781,
17.5566535132897));
#27319=CARTESIAN_POINT('Ctrl Pts',(-66.7536157259145,0.117030593831996,
17.519607549767));
#27320=CARTESIAN_POINT('Ctrl Pts',(-66.6005307217209,0.726061762452023,
17.4825615862444));
#27321=CARTESIAN_POINT('Ctrl Pts',(-66.22663513746,1.13142198093974,17.4455156227217));
#27322=CARTESIAN_POINT('Ctrl Pts',(-65.8527395531992,1.53678219942746,17.408469659199));
#27323=CARTESIAN_POINT('Ctrl Pts',(-65.258033388871,1.73847146778286,17.3714236956763));
#27324=CARTESIAN_POINT('Ctrl Pts',(-64.7146872927936,1.64418554868717,17.3343777321536));
#27325=CARTESIAN_POINT('Ctrl Pts',(-64.1713411967163,1.54989962959147,17.2973317686309));
#27326=CARTESIAN_POINT('Ctrl Pts',(-63.6793551688898,1.15963852304468,17.2602858051083));
#27327=CARTESIAN_POINT('Ctrl Pts',(-63.4638894046994,0.652007437388906,
17.2232398415856));
#27328=CARTESIAN_POINT('Ctrl Pts',(-63.37718924249,0.447744372051051,17.2083331065937));
#27329=CARTESIAN_POINT('Ctrl Pts',(-63.3352614657588,0.224477513359583,
17.1934263716017));
#27330=CARTESIAN_POINT('Ctrl Pts',(-63.3362856132907,0.000842509924184317,
17.1785196366098));
#27331=CARTESIAN_POINT('Ctrl Pts',(-63.3357797744869,-0.00117646094452181,
17.3714803633902));
#27332=CARTESIAN_POINT('Ctrl Pts',(-63.3381212965673,0.35793500664807,17.3954357378302));
#27333=CARTESIAN_POINT('Ctrl Pts',(-63.4521589055967,0.718401958553989,
17.4193911122702));
#27334=CARTESIAN_POINT('Ctrl Pts',(-63.6665656652298,1.00334589962882,17.4433464867103));
#27335=CARTESIAN_POINT('Ctrl Pts',(-63.9981365624523,1.44399953555901,17.480392450233));
#27336=CARTESIAN_POINT('Ctrl Pts',(-64.569743310557,1.70403761325246,17.5174384137557));
#27337=CARTESIAN_POINT('Ctrl Pts',(-65.1197868400431,1.66445223193655,17.5544843772783));
#27338=CARTESIAN_POINT('Ctrl Pts',(-65.6698303695292,1.62486685062065,17.591530340801));
#27339=CARTESIAN_POINT('Ctrl Pts',(-66.1983106803967,1.28565801029539,17.6285763043237));
#27340=CARTESIAN_POINT('Ctrl Pts',(-66.4633657616898,0.802066560180599,
17.6656222678464));
#27341=CARTESIAN_POINT('Ctrl Pts',(-66.728420842983,0.318475110065811,17.702668231369));
#27342=CARTESIAN_POINT('Ctrl Pts',(-66.7300506947019,-0.309498949838504,
17.7397141948917));
#27343=CARTESIAN_POINT('Ctrl Pts',(-66.4675094059654,-0.794459730162069,
17.7767601584144));
#27344=CARTESIAN_POINT('Ctrl Pts',(-66.2049681172289,-1.27942051048564,
17.8138061219371));
#27345=CARTESIAN_POINT('Ctrl Pts',(-65.6782556880371,-1.62136801122844,
17.8508520854598));
#27346=CARTESIAN_POINT('Ctrl Pts',(-65.1284250482722,-1.6638080197013,17.8878980489824));
#27347=CARTESIAN_POINT('Ctrl Pts',(-64.5785944085073,-1.70624802817415,
17.9249440125051));
#27348=CARTESIAN_POINT('Ctrl Pts',(-64.0056455581693,-1.44918054437704,
17.9619899760278));
#27349=CARTESIAN_POINT('Ctrl Pts',(-63.6717917874564,-1.01025395994158,
17.9990359395505));
#27350=CARTESIAN_POINT('Ctrl Pts',(-63.4541716406064,-0.72414286538296,
18.0231840808304));
#27351=CARTESIAN_POINT('Ctrl Pts',(-63.3381427347181,-0.360760035483751,
18.0473322221103));
#27352=CARTESIAN_POINT('Ctrl Pts',(-63.3357162681914,0.001206443822575,
18.0714803633902));
#27353=CARTESIAN_POINT('Origin',(-65.,8.88178419700125E-15,17.));
#27354=CARTESIAN_POINT('',(-63.3314263973441,0.000500571934799431,18.7714803633902));
#27355=CARTESIAN_POINT('',(-63.3333325352018,-0.00145874397799977,18.5785196366098));
#27356=CARTESIAN_POINT('',(-63.334,8.44655409538511E-15,17.));
#27357=CARTESIAN_POINT('Ctrl Pts',(-63.3333325352018,-0.00145874397799977,
18.5785196366098));
#27358=CARTESIAN_POINT('Ctrl Pts',(-63.3323458932764,-0.109115274956348,
18.5713112672072));
#27359=CARTESIAN_POINT('Ctrl Pts',(-63.3418839056658,-0.216597722493267,
18.5641028978047));
#27360=CARTESIAN_POINT('Ctrl Pts',(-63.3625817175621,-0.321886358428994,
18.5568945284021));
#27361=CARTESIAN_POINT('Ctrl Pts',(-63.4689539553991,-0.862996108553313,
18.5198485648794));
#27362=CARTESIAN_POINT('Ctrl Pts',(-63.8700831830826,-1.34616204853444,
18.4828026013567));
#27363=CARTESIAN_POINT('Ctrl Pts',(-64.382390335006,-1.55026054620227,18.445756637834));
#27364=CARTESIAN_POINT('Ctrl Pts',(-64.8946974869294,-1.75435904387011,
18.4087106743114));
#27365=CARTESIAN_POINT('Ctrl Pts',(-65.5181825630929,-1.67939009922465,
18.3716647107887));
#27366=CARTESIAN_POINT('Ctrl Pts',(-65.9675040829891,-1.35966367488599,
18.334618747266));
#27367=CARTESIAN_POINT('Ctrl Pts',(-66.4168256028854,-1.03993725054732,
18.2975727837433));
#27368=CARTESIAN_POINT('Ctrl Pts',(-66.6919835665143,-0.475453346515448,
18.2605268202206));
#27369=CARTESIAN_POINT('Ctrl Pts',(-66.6670503715696,0.0754487776881411,
18.223480856698));
#27370=CARTESIAN_POINT('Ctrl Pts',(-66.6421171766249,0.626350901891734,
18.1864348931753));
#27371=CARTESIAN_POINT('Ctrl Pts',(-66.3170928231065,1.16367124626704,18.1493889296526));
#27372=CARTESIAN_POINT('Ctrl Pts',(-65.8407265494155,1.44150210839706,18.1123429661299));
#27373=CARTESIAN_POINT('Ctrl Pts',(-65.3643602757244,1.71933297052707,18.0752970026072));
#27374=CARTESIAN_POINT('Ctrl Pts',(-64.7366520818608,1.7376743504118,18.0382510390846));
#27375=CARTESIAN_POINT('Ctrl Pts',(-64.2448761820938,1.48813221154433,18.0012050755619));
#27376=CARTESIAN_POINT('Ctrl Pts',(-63.7531002823268,1.23859007267687,17.9641591120392));
#27377=CARTESIAN_POINT('Ctrl Pts',(-63.3972566766564,0.721164415057202,
17.9271131485165));
#27378=CARTESIAN_POINT('Ctrl Pts',(-63.3401992089882,0.172658024897994,
17.8900671849938));
#27379=CARTESIAN_POINT('Ctrl Pts',(-63.3342707730138,0.115666623973004,
17.8862180021992));
#27380=CARTESIAN_POINT('Ctrl Pts',(-63.3315679757844,0.0583396813265098,
17.8823688194045));
#27381=CARTESIAN_POINT('Ctrl Pts',(-63.331966723543,0.00097473362895843,
17.8785196366098));
#27382=CARTESIAN_POINT('Ctrl Pts',(-63.3357162681914,0.001206443822575,
18.0714803633902));
#27383=CARTESIAN_POINT('Ctrl Pts',(-63.3344202622762,0.194537237022054,
18.084378185633));
#27384=CARTESIAN_POINT('Ctrl Pts',(-63.3655323149503,0.38746397927637,18.0972760078758));
#27385=CARTESIAN_POINT('Ctrl Pts',(-63.4308825664874,0.567997006411733,
18.1101738301185));
#27386=CARTESIAN_POINT('Ctrl Pts',(-63.6185858073192,1.08653570325578,18.1472197936412));
#27387=CARTESIAN_POINT('Ctrl Pts',(-64.0887509800707,1.50282741187006,18.1842657571639));
#27388=CARTESIAN_POINT('Ctrl Pts',(-64.6262043274144,1.62635387127239,18.2213117206866));
#27389=CARTESIAN_POINT('Ctrl Pts',(-65.1636576747581,1.74988033067473,18.2583576842093));
#27390=CARTESIAN_POINT('Ctrl Pts',(-65.768399196694,1.58064154086511,18.2954036477319));
#27391=CARTESIAN_POINT('Ctrl Pts',(-66.1636655065904,1.19609059364976,18.3324496112546));
#27392=CARTESIAN_POINT('Ctrl Pts',(-66.5589318164868,0.811539646434416,
18.3694955747773));
#27393=CARTESIAN_POINT('Ctrl Pts',(-66.7447229143437,0.211676541813339,
18.4065415383));
#27394=CARTESIAN_POINT('Ctrl Pts',(-66.6360104507197,-0.328967968929756,
18.4435875018227));
#27395=CARTESIAN_POINT('Ctrl Pts',(-66.5272979870957,-0.869612479672855,
18.4806334653453));
#27396=CARTESIAN_POINT('Ctrl Pts',(-66.1240819619909,-1.35103839653797,
18.517679428868));
#27397=CARTESIAN_POINT('Ctrl Pts',(-65.6108964756848,-1.55291841879864,
18.5547253923907));
#27398=CARTESIAN_POINT('Ctrl Pts',(-65.0977109893788,-1.7547984410593,18.5917713559134));
#27399=CARTESIAN_POINT('Ctrl Pts',(-64.4745560418716,-1.67713256871552,
18.6288173194361));
#27400=CARTESIAN_POINT('Ctrl Pts',(-64.0266220284185,-1.35546502864589,
18.6658632829587));
#27401=CARTESIAN_POINT('Ctrl Pts',(-63.6009392798522,-1.04977642615326,
18.7010689764359));
#27402=CARTESIAN_POINT('Ctrl Pts',(-63.3335015355576,-0.523725769548784,
18.7362746699131));
#27403=CARTESIAN_POINT('Ctrl Pts',(-63.3314263973441,0.000500571934799431,
18.7714803633902));
#27404=CARTESIAN_POINT('Origin',(-65.,8.88178419700125E-15,17.));
#27405=CARTESIAN_POINT('',(-63.3342413915565,-0.00152189757969434,19.4714803633902));
#27406=CARTESIAN_POINT('',(-63.3367061905351,-6.33250723186663E-5,19.2785196366098));
#27407=CARTESIAN_POINT('',(-63.334,8.44655409538511E-15,17.));
#27408=CARTESIAN_POINT('Ctrl Pts',(-63.3367061905351,-6.33250723186663E-5,
19.2785196366098));
#27409=CARTESIAN_POINT('Ctrl Pts',(-63.336613224224,-0.274266937448918,
19.26025371501));
#27410=CARTESIAN_POINT('Ctrl Pts',(-63.4006540507369,-0.548429669491744,
19.2419877934101));
#27411=CARTESIAN_POINT('Ctrl Pts',(-63.5290671316579,-0.788102757387643,
19.2237218718103));
#27412=CARTESIAN_POINT('Ctrl Pts',(-63.7895076621637,-1.27419487286282,
19.1866759082877));
#27413=CARTESIAN_POINT('Ctrl Pts',(-64.3147356017013,-1.61841804812354,
19.149629944765));
#27414=CARTESIAN_POINT('Ctrl Pts',(-64.8643774055205,-1.66323659510228,
19.1125839812423));
#27415=CARTESIAN_POINT('Ctrl Pts',(-65.4140192093397,-1.70805514208102,
19.0755380177196));
#27416=CARTESIAN_POINT('Ctrl Pts',(-65.9880748774405,-1.45346906077779,
19.0384920541969));
#27417=CARTESIAN_POINT('Ctrl Pts',(-66.3238245781873,-1.01599111491804,
19.0014460906742));
#27418=CARTESIAN_POINT('Ctrl Pts',(-66.6595742789341,-0.578513169058296,
18.9644001271516));
#27419=CARTESIAN_POINT('Ctrl Pts',(-66.757018012327,0.0418566413579672,
18.9273541636289));
#27420=CARTESIAN_POINT('Ctrl Pts',(-66.5715601012413,0.561202554865611,
18.8903082001062));
#27421=CARTESIAN_POINT('Ctrl Pts',(-66.3861021901555,1.08054846837325,18.8532622365835));
#27422=CARTESIAN_POINT('Ctrl Pts',(-65.9177426345912,1.49887048497227,18.8162162730609));
#27423=CARTESIAN_POINT('Ctrl Pts',(-65.3808288409285,1.62472116171496,18.7791703095382));
#27424=CARTESIAN_POINT('Ctrl Pts',(-64.8439150472658,1.75057183845764,18.7421243460155));
#27425=CARTESIAN_POINT('Ctrl Pts',(-64.2384470155047,1.58395117534399,18.7050783824928));
#27426=CARTESIAN_POINT('Ctrl Pts',(-63.8415206236195,1.20111406365342,18.6680324189701));
#27427=CARTESIAN_POINT('Ctrl Pts',(-63.5218278028516,0.89276904393903,18.63819482485));
#27428=CARTESIAN_POINT('Ctrl Pts',(-63.3374165408442,0.444163795089785,
18.6083572307299));
#27429=CARTESIAN_POINT('Ctrl Pts',(-63.3333325352018,-0.00145874397799977,
18.5785196366098));
#27430=CARTESIAN_POINT('Ctrl Pts',(-63.3314263973441,0.000500571934799431,
18.7714803633902));
#27431=CARTESIAN_POINT('Ctrl Pts',(-63.3313179258352,0.0279029020134445,
18.7733206334357));
#27432=CARTESIAN_POINT('Ctrl Pts',(-63.3319345194755,0.0553002474134458,
18.7751609034813));
#27433=CARTESIAN_POINT('Ctrl Pts',(-63.3332914773975,0.0826608742403348,
18.7770011735268));
#27434=CARTESIAN_POINT('Ctrl Pts',(-63.3606080192284,0.633450029261455,
18.8140471370495));
#27435=CARTESIAN_POINT('Ctrl Pts',(-63.6879541822893,1.16935913150821,18.8510931005721));
#27436=CARTESIAN_POINT('Ctrl Pts',(-64.1655181388753,1.44512634150633,18.8881390640948));
#27437=CARTESIAN_POINT('Ctrl Pts',(-64.6430820954612,1.72089355150444,18.9251850276175));
#27438=CARTESIAN_POINT('Ctrl Pts',(-65.2708638455722,1.73651886925393,18.9622309911402));
#27439=CARTESIAN_POINT('Ctrl Pts',(-65.7615555115074,1.48485127952435,18.9992769546629));
#27440=CARTESIAN_POINT('Ctrl Pts',(-66.2522471774427,1.23318368979477,19.0363229181856));
#27441=CARTESIAN_POINT('Ctrl Pts',(-66.6058487592021,0.714223192586123,
19.0733688817082));
#27442=CARTESIAN_POINT('Ctrl Pts',(-66.6605324878321,0.165475002074336,
19.1104148452309));
#27443=CARTESIAN_POINT('Ctrl Pts',(-66.715216216462,-0.383273188437459,
19.1474608087536));
#27444=CARTESIAN_POINT('Ctrl Pts',(-66.4709820919624,-0.961809072252402,
19.1845067722763));
#27445=CARTESIAN_POINT('Ctrl Pts',(-66.0396052463205,-1.30536242146666,
19.221552735799));
#27446=CARTESIAN_POINT('Ctrl Pts',(-65.6082284006786,-1.64891577068092,
19.2585986993216));
#27447=CARTESIAN_POINT('Ctrl Pts',(-64.9897088338945,-1.75748658529449,
19.2956446628443));
#27448=CARTESIAN_POINT('Ctrl Pts',(-64.4671155329348,-1.58138681666734,
19.332690626367));
#27449=CARTESIAN_POINT('Ctrl Pts',(-63.9445222319752,-1.40528704804019,
19.3697365898897));
#27450=CARTESIAN_POINT('Ctrl Pts',(-63.5178551968399,-0.944516696172312,
19.4067825534124));
#27451=CARTESIAN_POINT('Ctrl Pts',(-63.3823810155581,-0.409949924733961,
19.443828516935));
#27452=CARTESIAN_POINT('Ctrl Pts',(-63.34867413809,-0.276946156097573,19.4530457990868));
#27453=CARTESIAN_POINT('Ctrl Pts',(-63.3329934814549,-0.139374038553363,
19.4622630812385));
#27454=CARTESIAN_POINT('Ctrl Pts',(-63.3342413915565,-0.00152189757969434,
19.4714803633902));
#27455=CARTESIAN_POINT('Origin',(-65.,8.88178419700125E-15,17.));
#27456=CARTESIAN_POINT('',(-63.33660733148,0.000426122236803078,20.1714803633902));
#27457=CARTESIAN_POINT('',(-63.3335649842428,0.0014916225119581,19.9785196366098));
#27458=CARTESIAN_POINT('',(-63.334,8.44655409538511E-15,17.));
#27459=CARTESIAN_POINT('Ctrl Pts',(-63.3335649842428,0.0014916225119581,
19.9785196366098));
#27460=CARTESIAN_POINT('Ctrl Pts',(-63.3376081205507,-0.436609739463921,
19.9491961628127));
#27461=CARTESIAN_POINT('Ctrl Pts',(-63.5150446040949,-0.877608758866617,
19.9198726890157));
#27462=CARTESIAN_POINT('Ctrl Pts',(-63.8250037086467,-1.18496125357118,
19.8905492152186));
#27463=CARTESIAN_POINT('Ctrl Pts',(-64.2165921595995,-1.57325663038184,
19.8535032516959));
#27464=CARTESIAN_POINT('Ctrl Pts',(-64.8196955128484,-1.74824327998199,
19.8164572881732));
#27465=CARTESIAN_POINT('Ctrl Pts',(-65.3583001004237,-1.62983756803352,
19.7794113246505));
#27466=CARTESIAN_POINT('Ctrl Pts',(-65.896904687999,-1.51143185608504,19.7423653611279));
#27467=CARTESIAN_POINT('Ctrl Pts',(-66.3710105099008,-1.09963378258793,
19.7053193976052));
#27468=CARTESIAN_POINT('Ctrl Pts',(-66.5636403476301,-0.582905071893245,
19.6682734340825));
#27469=CARTESIAN_POINT('Ctrl Pts',(-66.7562701853594,-0.06617636119856,
19.6312274705598));
#27470=CARTESIAN_POINT('Ctrl Pts',(-66.6674240389162,0.555482986693699,
19.5941815070372));
#27471=CARTESIAN_POINT('Ctrl Pts',(-66.3377628513866,0.997567046656923,
19.5571355435145));
#27472=CARTESIAN_POINT('Ctrl Pts',(-66.008101663857,1.43965110662014,19.5200895799918));
#27473=CARTESIAN_POINT('Ctrl Pts',(-65.437625435241,1.70215987865433,19.4830436164691));
#27474=CARTESIAN_POINT('Ctrl Pts',(-64.8874158461961,1.66495473446781,19.4459976529464));
#27475=CARTESIAN_POINT('Ctrl Pts',(-64.3372062571513,1.62774959028128,19.4089516894237));
#27476=CARTESIAN_POINT('Ctrl Pts',(-63.8072633076776,1.29083052987405,19.3719057259011));
#27477=CARTESIAN_POINT('Ctrl Pts',(-63.5401183936778,0.808390471825612,
19.3348597623784));
#27478=CARTESIAN_POINT('Ctrl Pts',(-63.404692230951,0.563822814410774,19.3160797204555));
#27479=CARTESIAN_POINT('Ctrl Pts',(-63.3368017735151,0.281858137674118,
19.2972996785327));
#27480=CARTESIAN_POINT('Ctrl Pts',(-63.3367061905351,-6.33250723186663E-5,
19.2785196366098));
#27481=CARTESIAN_POINT('Ctrl Pts',(-63.3342413915565,-0.00152189757969434,
19.4714803633902));
#27482=CARTESIAN_POINT('Ctrl Pts',(-63.3380090632001,0.414679238971572,
19.4993090447612));
#27483=CARTESIAN_POINT('Ctrl Pts',(-63.496088728647,0.833432923200615,19.5271377261321));
#27484=CARTESIAN_POINT('Ctrl Pts',(-63.778271499721,1.13671878306761,19.5549664075031));
#27485=CARTESIAN_POINT('Ctrl Pts',(-64.1539174925939,1.540457528422,19.5920123710258));
#27486=CARTESIAN_POINT('Ctrl Pts',(-64.7494908057681,1.73957182812195,19.6290583345484));
#27487=CARTESIAN_POINT('Ctrl Pts',(-65.2924239354676,1.64293589624756,19.6661042980711));
#27488=CARTESIAN_POINT('Ctrl Pts',(-65.835357065167,1.54629996437316,19.7031502615938));
#27489=CARTESIAN_POINT('Ctrl Pts',(-66.3256500113918,1.15391380092444,19.7401962251165));
#27490=CARTESIAN_POINT('Ctrl Pts',(-66.5389174268969,0.645355153836879,
19.7772421886392));
#27491=CARTESIAN_POINT('Ctrl Pts',(-66.7521848424021,0.136796506749319,
19.8142881521618));
#27492=CARTESIAN_POINT('Ctrl Pts',(-66.6884267271877,-0.487934623977076,
19.8513341156845));
#27493=CARTESIAN_POINT('Ctrl Pts',(-66.3768223447206,-0.942926484478215,
19.8883800792072));
#27494=CARTESIAN_POINT('Ctrl Pts',(-66.0652179622535,-1.39791834497936,
19.9254260427299));
#27495=CARTESIAN_POINT('Ctrl Pts',(-65.5057673125336,-1.68317093525525,
19.9624720062526));
#27496=CARTESIAN_POINT('Ctrl Pts',(-64.9545061567026,-1.66813680856719,
19.9995179697752));
#27497=CARTESIAN_POINT('Ctrl Pts',(-64.4032450008716,-1.65310268187914,
20.0365639332979));
#27498=CARTESIAN_POINT('Ctrl Pts',(-63.8601733389293,-1.33778183822714,
20.0736098968206));
#27499=CARTESIAN_POINT('Ctrl Pts',(-63.5738309983811,-0.866482612606725,
20.1106558603433));
#27500=CARTESIAN_POINT('Ctrl Pts',(-63.4171190932323,-0.608545908587603,
20.1309306946923));
#27501=CARTESIAN_POINT('Ctrl Pts',(-63.3373039960783,-0.303889805224311,
20.1512055290412));
#27502=CARTESIAN_POINT('Ctrl Pts',(-63.33660733148,0.000426122236803078,
20.1714803633902));
#27503=CARTESIAN_POINT('Origin',(-65.,8.88178419700125E-15,17.));
#27504=CARTESIAN_POINT('',(-63.3326792503596,0.00130047270867312,20.8714803633902));
#27505=CARTESIAN_POINT('',(-63.3318013787731,-0.000864016794193591,20.6785196366098));
#27506=CARTESIAN_POINT('',(-63.334,8.44655409538511E-15,17.));
#27507=CARTESIAN_POINT('Ctrl Pts',(-63.3318013787731,-0.000864016794193591,
20.6785196366098));
#27508=CARTESIAN_POINT('Ctrl Pts',(-63.3314877360124,-0.0505539851742854,
20.6751845741382));
#27509=CARTESIAN_POINT('Ctrl Pts',(-63.3335154742976,-0.100217999006543,
20.6718495116665));
#27510=CARTESIAN_POINT('Ctrl Pts',(-63.3379679807618,-0.149663664483458,
20.6685144491949));
#27511=CARTESIAN_POINT('Ctrl Pts',(-63.3874265421712,-0.698907444829369,
20.6314684856722));
#27512=CARTESIAN_POINT('Ctrl Pts',(-63.7360730319708,-1.22120960136621,
20.5944225221495));
#27513=CARTESIAN_POINT('Ctrl Pts',(-64.2243472290266,-1.47753582103745,
20.5573765586268));
#27514=CARTESIAN_POINT('Ctrl Pts',(-64.7126214260825,-1.73386204070869,
20.5203305951042));
#27515=CARTESIAN_POINT('Ctrl Pts',(-65.3405233303947,-1.72421232351431,
20.4832846315815));
#27516=CARTESIAN_POINT('Ctrl Pts',(-65.8206901647961,-1.45300280103399,
20.4462386680588));
#27517=CARTESIAN_POINT('Ctrl Pts',(-66.3008569991975,-1.18179327855367,
20.4091927045361));
#27518=CARTESIAN_POINT('Ctrl Pts',(-66.6332887636883,-0.649023950787419,
20.3721467410134));
#27519=CARTESIAN_POINT('Ctrl Pts',(-66.6658461309716,-0.098519780176524,
20.3351007774908));
#27520=CARTESIAN_POINT('Ctrl Pts',(-66.698403498255,0.451984390434375,20.2980548139681));
#27521=CARTESIAN_POINT('Ctrl Pts',(-66.431086468331,1.02022340388992,20.2610088504454));
#27522=CARTESIAN_POINT('Ctrl Pts',(-65.9862342185508,1.34613948307829,20.2239628869227));
#27523=CARTESIAN_POINT('Ctrl Pts',(-65.5413819687707,1.67205556226665,20.1869169234));
#27524=CARTESIAN_POINT('Ctrl Pts',(-64.9189944991343,1.75564870718785,20.1498709598773));
#27525=CARTESIAN_POINT('Ctrl Pts',(-64.4039109527966,1.55866202617725,20.1128249963547));
#27526=CARTESIAN_POINT('Ctrl Pts',(-63.8888274064588,1.36167534516665,20.075779032832));
#27527=CARTESIAN_POINT('Ctrl Pts',(-63.4810477834196,0.88410883822424,20.0387330693093));
#27528=CARTESIAN_POINT('Ctrl Pts',(-63.3671947462284,0.344523532742449,
20.0016871057866));
#27529=CARTESIAN_POINT('Ctrl Pts',(-63.3434612857827,0.232043208803146,
19.993964616061));
#27530=CARTESIAN_POINT('Ctrl Pts',(-63.332500203214,0.116867900576733,19.9862421263354));
#27531=CARTESIAN_POINT('Ctrl Pts',(-63.3335649842428,0.0014916225119581,
19.9785196366098));
#27532=CARTESIAN_POINT('Ctrl Pts',(-63.33660733148,0.000426122236803078,
20.1714803633902));
#27533=CARTESIAN_POINT('Ctrl Pts',(-63.3360310578706,0.252153048396664,
20.1882514925639));
#27534=CARTESIAN_POINT('Ctrl Pts',(-63.3895909699888,0.503647211782724,
20.2050226217376));
#27535=CARTESIAN_POINT('Ctrl Pts',(-63.4985445030998,0.728272982538817,
20.2217937509113));
#27536=CARTESIAN_POINT('Ctrl Pts',(-63.7392133675209,1.22445174447511,20.258839714434));
#27537=CARTESIAN_POINT('Ctrl Pts',(-64.2501641155174,1.58953166075887,20.2958856779567));
#27538=CARTESIAN_POINT('Ctrl Pts',(-64.7975572478224,1.65643198360556,20.3329316414794));
#27539=CARTESIAN_POINT('Ctrl Pts',(-65.3449503801273,1.72333230645225,20.369977605002));
#27540=CARTESIAN_POINT('Ctrl Pts',(-65.9287858967409,1.49205303586186,20.4070235685247));
#27541=CARTESIAN_POINT('Ctrl Pts',(-66.2818681473523,1.06844015166584,20.4440695320474));
#27542=CARTESIAN_POINT('Ctrl Pts',(-66.6349503979637,0.644827267469811,
20.4811154955701));
#27543=CARTESIAN_POINT('Ctrl Pts',(-66.757279382573,0.0288807696681399,
20.5181614590928));
#27544=CARTESIAN_POINT('Ctrl Pts',(-66.5928705785965,-0.497507359328862,
20.5552074226155));
#27545=CARTESIAN_POINT('Ctrl Pts',(-66.42846177462,-1.02389548832586,20.5922533861381));
#27546=CARTESIAN_POINT('Ctrl Pts',(-65.9773151820577,-1.46072524851819,
20.6292993496608));
#27547=CARTESIAN_POINT('Ctrl Pts',(-65.4459005359057,-1.60808016419333,
20.6663453131835));
#27548=CARTESIAN_POINT('Ctrl Pts',(-64.9144858897538,-1.75543507986847,
20.7033912767062));
#27549=CARTESIAN_POINT('Ctrl Pts',(-64.3028031900122,-1.61331515102642,
20.7404372402289));
#27550=CARTESIAN_POINT('Ctrl Pts',(-63.8907926142615,-1.24676010485228,
20.7774832037515));
#27551=CARTESIAN_POINT('Ctrl Pts',(-63.5423261851822,-0.936738625989558,
20.8088155902978));
#27552=CARTESIAN_POINT('Ctrl Pts',(-63.3366907965296,-0.466172446764649,
20.840147976844));
#27553=CARTESIAN_POINT('Ctrl Pts',(-63.3326792503596,0.00130047270867312,
20.8714803633902));
#27554=CARTESIAN_POINT('Origin',(-65.,8.88178419700125E-15,17.));
#27555=CARTESIAN_POINT('',(-63.3325282901756,-0.00121307831917494,21.5714803633902));
#27556=CARTESIAN_POINT('',(-63.3361634080255,-0.000941845566861395,21.3785196366098));
#27557=CARTESIAN_POINT('',(-63.334,8.44655409538511E-15,17.));
#27558=CARTESIAN_POINT('',(-66.2690708798524,-1.07935865304852,22.));
#27559=CARTESIAN_POINT('Ctrl Pts',(-63.3325282901756,-0.00121307831917494,
21.5714803633902));
#27560=CARTESIAN_POINT('Ctrl Pts',(-63.3364666394986,0.471552579298233,
21.6031823516921));
#27561=CARTESIAN_POINT('Ctrl Pts',(-63.5475594887738,0.947301871471172,
21.634884339994));
#27562=CARTESIAN_POINT('Ctrl Pts',(-63.9032471486994,1.25758535694562,21.6665863282959));
#27563=CARTESIAN_POINT('Ctrl Pts',(-64.3188927526783,1.62017304624496,21.7036322918186));
#27564=CARTESIAN_POINT('Ctrl Pts',(-64.9319903369098,1.75680828918912,21.7406782553412));
#27565=CARTESIAN_POINT('Ctrl Pts',(-65.4619049207954,1.60385028487086,21.7777242188639));
#27566=CARTESIAN_POINT('Ctrl Pts',(-65.991819504681,1.4508922805526,21.8147701823866));
#27567=CARTESIAN_POINT('Ctrl Pts',(-66.4385510882207,1.00834102897191,21.8518161459093));
#27568=CARTESIAN_POINT('Ctrl Pts',(-66.5975920398021,0.481277360573874,
21.8888621094319));
#27569=CARTESIAN_POINT('Ctrl Pts',(-66.7566329913835,-0.0457863078241613,
21.9259080729546));
#27570=CARTESIAN_POINT('Ctrl Pts',(-66.6279833110066,-0.657362393039546,
21.9629540364773));
#27571=CARTESIAN_POINT('Ctrl Pts',(-66.2690708798524,-1.07935865304854,
22.));
#27572=CARTESIAN_POINT('',(-63.7285313545748,-1.0812100993933,22.));
#27573=CARTESIAN_POINT('Origin',(-65.,8.88178419700125E-15,22.));
#27574=CARTESIAN_POINT('Ctrl Pts',(-63.7285300176229,-1.0812111317272,22.));
#27575=CARTESIAN_POINT('Ctrl Pts',(-64.0793901440197,-1.49274250755581,
21.9636770818144));
#27576=CARTESIAN_POINT('Ctrl Pts',(-64.6493623256457,-1.71876565001735,
21.9273541636289));
#27577=CARTESIAN_POINT('Ctrl Pts',(-65.1867621807782,-1.65816351020321,
21.8910312454434));
#27578=CARTESIAN_POINT('Ctrl Pts',(-65.7348595370708,-1.5963550219787,21.8539852819207));
#27579=CARTESIAN_POINT('Ctrl Pts',(-66.2490748882323,-1.2363965294347,21.816939318398));
#27580=CARTESIAN_POINT('Ctrl Pts',(-66.4944088007071,-0.742590901212604,
21.7798933548753));
#27581=CARTESIAN_POINT('Ctrl Pts',(-66.7397427131819,-0.248785272990512,
21.7428473913526));
#27582=CARTESIAN_POINT('Ctrl Pts',(-66.71619518697,0.378867490909668,21.7058014278299));
#27583=CARTESIAN_POINT('Ctrl Pts',(-66.4343747134738,0.852900746623167,
21.6687554643073));
#27584=CARTESIAN_POINT('Ctrl Pts',(-66.1525542399776,1.32693400233667,21.6317095007846));
#27585=CARTESIAN_POINT('Ctrl Pts',(-65.6124608191971,1.64734774986349,21.5946635372619));
#27586=CARTESIAN_POINT('Ctrl Pts',(-65.061356017574,1.66761252399563,21.5576175737392));
#27587=CARTESIAN_POINT('Ctrl Pts',(-64.5102512159508,1.68787729812776,21.5205716102165));
#27588=CARTESIAN_POINT('Ctrl Pts',(-63.9481350334849,1.40799309886521,21.4835256466939));
#27589=CARTESIAN_POINT('Ctrl Pts',(-63.6322204085561,0.955995223624118,
21.4464796831712));
#27590=CARTESIAN_POINT('Ctrl Pts',(-63.4390408141815,0.679601668824523,
21.4238263343174));
#27591=CARTESIAN_POINT('Ctrl Pts',(-63.3379218264913,0.338850724949929,
21.4011729854636));
#27592=CARTESIAN_POINT('Ctrl Pts',(-63.3361634080255,-0.000941845566861395,
21.3785196366098));
#27593=CARTESIAN_POINT('Origin',(-65.,8.88178419700125E-15,23.5459252805377));
#27594=CARTESIAN_POINT('',(-62.9427844533856,-0.00119489768197589,13.4540747194623));
#27595=CARTESIAN_POINT('',(-62.9484021938786,0.000803300711494623,13.3959252805377));
#27596=CARTESIAN_POINT('',(-62.94525,-1.20379215794662E-13,23.5459252805377));
#27597=CARTESIAN_POINT('',(-66.8826275096638,0.823232180103066,13.));
#27598=CARTESIAN_POINT('Ctrl Pts',(-62.9484021938786,0.000803300711494474,
13.3959252805377));
#27599=CARTESIAN_POINT('Ctrl Pts',(-62.9495841394398,-0.384792240838309,
13.3750880775932));
#27600=CARTESIAN_POINT('Ctrl Pts',(-63.239440569463,-1.45761852527273,13.3172049111259));
#27601=CARTESIAN_POINT('Ctrl Pts',(-64.970198323091,-2.42992595215151,13.2222757811361));
#27602=CARTESIAN_POINT('Ctrl Pts',(-67.0251392906009,-1.33877286094185,
13.111137890568));
#27603=CARTESIAN_POINT('Ctrl Pts',(-67.1563717950601,0.197213743559495,
13.0370459635227));
#27604=CARTESIAN_POINT('Ctrl Pts',(-66.8826275096638,0.823232180103066,
13.));
#27605=CARTESIAN_POINT('',(-66.2235927967208,1.65534565011394,13.));
#27606=CARTESIAN_POINT('Origin',(-65.,8.88178419700125E-15,13.));
#27607=CARTESIAN_POINT('Ctrl Pts',(-62.9427844533856,-0.00119489768197575,
13.4540747194623));
#27608=CARTESIAN_POINT('Ctrl Pts',(-62.9422817266512,-0.0728349382260852,
13.4501772883951));
#27609=CARTESIAN_POINT('Ctrl Pts',(-62.9781729708452,-0.824925643882587,
13.4092338938053));
#27610=CARTESIAN_POINT('Ctrl Pts',(-63.9036938704104,-2.16732302296763,
13.3312445356927));
#27611=CARTESIAN_POINT('Ctrl Pts',(-66.2265689546786,-2.09606376419021,
13.2201066451247));
#27612=CARTESIAN_POINT('Ctrl Pts',(-67.4179368644029,-0.120091680801057,
13.1096917998938));
#27613=CARTESIAN_POINT('Ctrl Pts',(-66.7594496906129,1.25819328818367,13.0363229181856));
#27614=CARTESIAN_POINT('Ctrl Pts',(-66.2235939546714,1.65534738192937,13.));
#27615=CARTESIAN_POINT('Origin',(-65.,8.88178419700125E-15,23.5459252805377));
#27616=CARTESIAN_POINT('',(-62.9480827837869,-0.00102651687047844,14.1540747194623));
#27617=CARTESIAN_POINT('',(-62.9433366278651,0.00149772234160084,14.0959252805377));
#27618=CARTESIAN_POINT('',(-62.94525,-1.20379215794662E-13,23.5459252805377));
#27619=CARTESIAN_POINT('Ctrl Pts',(-62.9433366278651,0.0014977223416008,
14.0959252805377));
#27620=CARTESIAN_POINT('Ctrl Pts',(-62.9481477427571,-0.585192187367149,
14.0640305253959));
#27621=CARTESIAN_POINT('Ctrl Pts',(-63.5186241718586,-1.86149425637257,
13.9950898067315));
#27622=CARTESIAN_POINT('Ctrl Pts',(-65.684305645688,-2.33026686199619,13.8891031245443));
#27623=CARTESIAN_POINT('Ctrl Pts',(-67.3289123722387,-0.688818574436933,
13.7779652339763));
#27624=CARTESIAN_POINT('Ctrl Pts',(-66.8417982611818,1.58294512384397,13.6668273434083));
#27625=CARTESIAN_POINT('Ctrl Pts',(-64.6689465387577,2.4061546469661,13.5556894528402));
#27626=CARTESIAN_POINT('Ctrl Pts',(-63.14955544062,1.28502616351136,13.4653887652167));
#27627=CARTESIAN_POINT('Ctrl Pts',(-62.9474827867649,0.300748827451906,
13.4121340411158));
#27628=CARTESIAN_POINT('Ctrl Pts',(-62.9484021938786,0.000803300711494474,
13.3959252805377));
#27629=CARTESIAN_POINT('Ctrl Pts',(-62.9480827837869,-0.00102651687047834,
14.1540747194623));
#27630=CARTESIAN_POINT('Ctrl Pts',(-62.9468311597533,-0.277742487636526,
14.1391197361979));
#27631=CARTESIAN_POINT('Ctrl Pts',(-63.1278468516848,-1.23836027065323,
14.0871187894108));
#27632=CARTESIAN_POINT('Ctrl Pts',(-64.5878737813476,-2.39342385873017,
13.998071879101));
#27633=CARTESIAN_POINT('Ctrl Pts',(-66.7873400138256,-1.64430308142018,
13.8869339885329));
#27634=CARTESIAN_POINT('Ctrl Pts',(-67.3508170614469,0.60985221755875,13.7757960979649));
#27635=CARTESIAN_POINT('Ctrl Pts',(-65.7625975239189,2.30583209920717,13.6646582073969));
#27636=CARTESIAN_POINT('Ctrl Pts',(-63.5564754082319,1.90574022357352,13.557417747896));
#27637=CARTESIAN_POINT('Ctrl Pts',(-62.9470602579309,0.608119845326397,
13.4872232519178));
#27638=CARTESIAN_POINT('Ctrl Pts',(-62.9427844533856,-0.00119489768197575,
13.4540747194623));
#27639=CARTESIAN_POINT('Origin',(-65.,8.88178419700125E-15,23.5459252805377));
#27640=CARTESIAN_POINT('',(-62.946510263771,0.00176526862452855,14.8540747194623));
#27641=CARTESIAN_POINT('',(-62.94372126594,-0.00163389948555286,14.7959252805377));
#27642=CARTESIAN_POINT('',(-62.94525,-1.20379215794662E-13,23.5459252805377));
#27643=CARTESIAN_POINT('Ctrl Pts',(-62.94372126594,-0.00163389948555279,
14.7959252805377));
#27644=CARTESIAN_POINT('Ctrl Pts',(-62.9427765522985,-0.110331733448607,
14.7900189367213));
#27645=CARTESIAN_POINT('Ctrl Pts',(-63.0000473239053,-0.899810372641744,
14.7470666293823));
#27646=CARTESIAN_POINT('Ctrl Pts',(-64.0226192720082,-2.2232951335223,14.6670683585206));
#27647=CARTESIAN_POINT('Ctrl Pts',(-66.3378385875382,-2.02694463079713,
14.5559304679526));
#27648=CARTESIAN_POINT('Ctrl Pts',(-67.4285194097127,0.0246926670119235,
14.4447925773845));
#27649=CARTESIAN_POINT('Ctrl Pts',(-66.2963482043283,2.05372573368661,14.3336546868165));
#27650=CARTESIAN_POINT('Ctrl Pts',(-63.9776161165208,2.20296580816612,14.2225167962485));
#27651=CARTESIAN_POINT('Ctrl Pts',(-62.9915607037629,0.87164277914502,14.1432736608222));
#27652=CARTESIAN_POINT('Ctrl Pts',(-62.942559601823,0.0962519214711429,
14.1010764889186));
#27653=CARTESIAN_POINT('Ctrl Pts',(-62.9433366278651,0.0014977223416008,
14.0959252805377));
#27654=CARTESIAN_POINT('Ctrl Pts',(-62.946510263771,0.00176526862452855,
14.8540747194623));
#27655=CARTESIAN_POINT('Ctrl Pts',(-62.9504460460768,-0.4786248922106,14.8280621840006));
#27656=CARTESIAN_POINT('Ctrl Pts',(-63.3581297348818,-1.64918471803045,
14.7650036850163));
#27657=CARTESIAN_POINT('Ctrl Pts',(-65.3081850174459,-2.40901142364103,
14.6648992225093));
#27658=CARTESIAN_POINT('Ctrl Pts',(-67.1910886177016,-1.04758997952521,
14.5537613319412));
#27659=CARTESIAN_POINT('Ctrl Pts',(-67.068463685159,1.27270221153157,14.4426234413732));
#27660=CARTESIAN_POINT('Ctrl Pts',(-65.0525510239567,2.42807611461694,14.3314855508051));
#27661=CARTESIAN_POINT('Ctrl Pts',(-63.2662754947239,1.50459133827138,14.2353026435015));
#27662=CARTESIAN_POINT('Ctrl Pts',(-62.9499316392037,0.407728674576415,
14.1761656997206));
#27663=CARTESIAN_POINT('Ctrl Pts',(-62.9480827837869,-0.00102651687047834,
14.1540747194623));
#27664=CARTESIAN_POINT('Origin',(-65.,8.88178419700125E-15,23.5459252805377));
#27665=CARTESIAN_POINT('',(-62.9418498698494,-8.27718826610594E-6,15.5540747194623));
#27666=CARTESIAN_POINT('',(-62.9484914975566,-0.00046897412753623,15.4959252805377));
#27667=CARTESIAN_POINT('',(-62.94525,-1.20379215794662E-13,23.5459252805377));
#27668=CARTESIAN_POINT('Ctrl Pts',(-62.9484914975566,-0.000468974127536166,
15.4959252805377));
#27669=CARTESIAN_POINT('Ctrl Pts',(-62.9478504078462,-0.314513019480932,
15.4789613845241));
#27670=CARTESIAN_POINT('Ctrl Pts',(-63.1632430376845,-1.31353647315872,
15.4249515249878));
#27671=CARTESIAN_POINT('Ctrl Pts',(-64.7178900651262,-2.41220423477673,
15.3338957019289));
#27672=CARTESIAN_POINT('Ctrl Pts',(-66.8736278902366,-1.54526173974447,
15.2227578113608));
#27673=CARTESIAN_POINT('Ctrl Pts',(-67.3144128645646,0.736076372865376,
15.1116199207928));
#27674=CARTESIAN_POINT('Ctrl Pts',(-65.6367894857436,2.34367538861625,15.0004820302248));
#27675=CARTESIAN_POINT('Ctrl Pts',(-63.4964372981478,1.83465185719793,14.895250483473));
#27676=CARTESIAN_POINT('Ctrl Pts',(-62.9487020162047,0.571446388044023,
14.827064900244));
#27677=CARTESIAN_POINT('Ctrl Pts',(-62.94372126594,-0.00163389948555279,
14.7959252805377));
#27678=CARTESIAN_POINT('Ctrl Pts',(-62.9418498868449,-8.27714689220955E-6,
15.5540747194623));
#27679=CARTESIAN_POINT('Ctrl Pts',(-62.9418498603911,-0.000451185307763086,
15.5540505953261));
#27680=CARTESIAN_POINT('Ctrl Pts',(-62.9420505595996,-0.681041096754107,
15.5169805076671));
#27681=CARTESIAN_POINT('Ctrl Pts',(-63.6841642251148,-2.04129618504103,
15.4428644564855));
#27682=CARTESIAN_POINT('Ctrl Pts',(-66.0013718021885,-2.21259314346662,
15.3317265659175));
#27683=CARTESIAN_POINT('Ctrl Pts',(-67.4020124146433,-0.358678503164364,
15.2205886753494));
#27684=CARTESIAN_POINT('Ctrl Pts',(-66.6040638188323,1.82353863480769,15.1094507847814));
#27685=CARTESIAN_POINT('Ctrl Pts',(-64.3378974271891,2.33665018787606,14.9983128942134));
#27686=CARTESIAN_POINT('Ctrl Pts',(-63.0663265778663,1.09149331437409,14.913187539107));
#27687=CARTESIAN_POINT('Ctrl Pts',(-62.9448408697591,0.205526654691516,
14.8651081475233));
#27688=CARTESIAN_POINT('Ctrl Pts',(-62.946510263771,0.00176526862452855,
14.8540747194623));
#27689=CARTESIAN_POINT('Origin',(-65.,8.88178419700125E-15,23.5459252805377));
#27690=CARTESIAN_POINT('',(-62.9465344116198,-0.00176006504695014,16.2540747194623));
#27691=CARTESIAN_POINT('',(-62.9454411297334,0.00187890759641046,16.1959252805377));
#27692=CARTESIAN_POINT('',(-62.94525,-1.20379215794662E-13,23.5459252805377));
#27693=CARTESIAN_POINT('Ctrl Pts',(-62.9454411297334,0.00187890759641044,
16.1959252805377));
#27694=CARTESIAN_POINT('Ctrl Pts',(-62.9501461271515,-0.514927296910581,
16.1679038323268));
#27695=CARTESIAN_POINT('Ctrl Pts',(-63.4098006358751,-1.72243750067869,
16.1028364205933));
#27696=CARTESIAN_POINT('Ctrl Pts',(-65.4379883182475,-2.38882429960344,
16.0007230453371));
#27697=CARTESIAN_POINT('Ctrl Pts',(-67.24452629377,-0.927586663439792,15.8895851547691));
#27698=CARTESIAN_POINT('Ctrl Pts',(-66.996623898036,1.38268156569091,15.7784472642011));
#27699=CARTESIAN_POINT('Ctrl Pts',(-64.9211890049946,2.42736567633039,15.667309373633));
#27700=CARTESIAN_POINT('Ctrl Pts',(-63.223670707888,1.42992668390708,15.5731353790785));
#27701=CARTESIAN_POINT('Ctrl Pts',(-62.9492504273939,0.371300206405418,
15.5160073480468));
#27702=CARTESIAN_POINT('Ctrl Pts',(-62.9484914975566,-0.000468974127536166,
15.4959252805377));
#27703=CARTESIAN_POINT('Ctrl Pts',(-62.9465344116198,-0.00176006504695018,
16.2540747194623));
#27704=CARTESIAN_POINT('Ctrl Pts',(-62.944864096038,-0.206418574104765,
16.2429930431288));
#27705=CARTESIAN_POINT('Ctrl Pts',(-63.0670246817589,-1.09329987115451,
16.1948654032727));
#27706=CARTESIAN_POINT('Ctrl Pts',(-64.3409338179361,-2.33750843231644,
16.1096917998938));
#27707=CARTESIAN_POINT('Ctrl Pts',(-66.6064316564341,-1.82145305641562,
15.9985539093258));
#27708=CARTESIAN_POINT('Ctrl Pts',(-67.401544381661,0.361798958737847,15.8874160187577));
#27709=CARTESIAN_POINT('Ctrl Pts',(-65.9984962989145,2.21389228381421,15.7762781281897));
#27710=CARTESIAN_POINT('Ctrl Pts',(-63.6820161659208,2.03962273041629,15.6651643617579));
#27711=CARTESIAN_POINT('Ctrl Pts',(-62.9418904838623,0.679695842678611,
15.5910965588488));
#27712=CARTESIAN_POINT('Ctrl Pts',(-62.9418498868449,-8.27714689220955E-6,
15.5540747194623));
#27713=CARTESIAN_POINT('Origin',(-65.,8.88178419700125E-15,23.5459252805377));
#27714=CARTESIAN_POINT('',(-62.9480689459238,0.00103910400151244,16.9540747194623));
#27715=CARTESIAN_POINT('',(-62.9421231189799,-0.000678771108088527,16.8959252805377));
#27716=CARTESIAN_POINT('',(-62.94525,-1.20379215794662E-13,23.5459252805377));
#27717=CARTESIAN_POINT('Ctrl Pts',(-62.9421231189799,-0.000678771108088587,
16.8959252805377));
#27718=CARTESIAN_POINT('Ctrl Pts',(-62.9419623987169,-0.038017692910355,
16.8938922436523));
#27719=CARTESIAN_POINT('Ctrl Pts',(-62.9598052246296,-0.755589108274127,
16.8548132432442));
#27720=CARTESIAN_POINT('Ctrl Pts',(-63.7964607753782,-2.1094569529468,16.7786882793134));
#27721=CARTESIAN_POINT('Ctrl Pts',(-66.119540899393,-2.15521309297246,16.6675503887454));
#27722=CARTESIAN_POINT('Ctrl Pts',(-67.4178925417354,-0.228278247224643,
16.5564124981773));
#27723=CARTESIAN_POINT('Ctrl Pts',(-66.5031197198625,1.9076022670654,16.4452746076093));
#27724=CARTESIAN_POINT('Ctrl Pts',(-64.2125243718594,2.29743279261729,16.3341367170413));
#27725=CARTESIAN_POINT('Ctrl Pts',(-63.0385141433925,1.01630861777054,16.251020274684));
#27726=CARTESIAN_POINT('Ctrl Pts',(-62.9439258504044,0.168320180393547,
16.2049497958495));
#27727=CARTESIAN_POINT('Ctrl Pts',(-62.9454411297334,0.00187890759641044,
16.1959252805377));
#27728=CARTESIAN_POINT('Ctrl Pts',(-62.9480689459238,0.00103910400151244,
16.9540747194623));
#27729=CARTESIAN_POINT('Ctrl Pts',(-62.9499449184218,-0.408602185927941,
16.9319354909316));
#27730=CARTESIAN_POINT('Ctrl Pts',(-63.2673355867028,-1.50638090616107,
16.8727502988781));
#27731=CARTESIAN_POINT('Ctrl Pts',(-65.0557052990257,-2.42800552371271,
16.776519143302));
#27732=CARTESIAN_POINT('Ctrl Pts',(-67.0701156187118,-1.27001386948507,
16.665381252734));
#27733=CARTESIAN_POINT('Ctrl Pts',(-67.1897256358837,1.05043588241969,16.5542433621659));
#27734=CARTESIAN_POINT('Ctrl Pts',(-65.3050549453524,2.4094097583915,16.4431054715979));
#27735=CARTESIAN_POINT('Ctrl Pts',(-63.3569278527547,1.6474176190389,16.3430492573633));
#27736=CARTESIAN_POINT('Ctrl Pts',(-62.9504479489003,0.477753335721173,
16.2800390066515));
#27737=CARTESIAN_POINT('Ctrl Pts',(-62.9465344116198,-0.00176006504695018,
16.2540747194623));
#27738=CARTESIAN_POINT('Origin',(-65.,8.88178419700125E-15,23.5459252805377));
#27739=CARTESIAN_POINT('',(-62.9427422720288,0.00120218122683403,17.6540747194623));
#27740=CARTESIAN_POINT('',(-62.9474450730054,-0.0014509802675629,17.5959252805377));
#27741=CARTESIAN_POINT('',(-62.94525,-1.20379215794662E-13,23.5459252805377));
#27742=CARTESIAN_POINT('Ctrl Pts',(-62.9474450730054,-0.00145098026756288,
17.5959252805377));
#27743=CARTESIAN_POINT('Ctrl Pts',(-62.9458669586282,-0.243481142931835,
17.582834691455));
#27744=CARTESIAN_POINT('Ctrl Pts',(-63.0973769195488,-1.16853721152032,
17.5326981388497));
#27745=CARTESIAN_POINT('Ctrl Pts',(-64.4682857559272,-2.36972472329319,
17.4455156227217));
#27746=CARTESIAN_POINT('Ctrl Pts',(-66.7025669780829,-1.73192984461803,
17.3343777321536));
#27747=CARTESIAN_POINT('Ctrl Pts',(-67.3784693367765,0.491120062256299,
17.2232398415856));
#27748=CARTESIAN_POINT('Ctrl Pts',(-65.8773317378418,2.26464220646723,17.1121019510175));
#27749=CARTESIAN_POINT('Ctrl Pts',(-63.6153124412349,1.97078728704394,17.0029970973349));
#27750=CARTESIAN_POINT('Ctrl Pts',(-62.9448910406138,0.642371504646387,
16.930938207175));
#27751=CARTESIAN_POINT('Ctrl Pts',(-62.9421231189799,-0.000678771108088587,
16.8959252805377));
#27752=CARTESIAN_POINT('Ctrl Pts',(-62.9427422720288,0.00120218122683403,
17.6540747194623));
#27753=CARTESIAN_POINT('Ctrl Pts',(-62.9469836764117,-0.608977902213451,
17.6208779387343));
#27754=CARTESIAN_POINT('Ctrl Pts',(-63.5579942556341,-1.90746584530598,
17.5506351944836));
#27755=CARTESIAN_POINT('Ctrl Pts',(-65.7655743703156,-2.30482315743207,
17.4433464867103));
#27756=CARTESIAN_POINT('Ctrl Pts',(-67.3516166417705,-0.606805630879782,
17.3322085961422));
#27757=CARTESIAN_POINT('Ctrl Pts',(-66.7851975318663,1.6466279712607,17.2210707055742));
#27758=CARTESIAN_POINT('Ctrl Pts',(-64.5847668755277,2.39288431727496,17.1099328150062));
#27759=CARTESIAN_POINT('Ctrl Pts',(-63.1270293146865,1.23655417501042,17.0209341529689));
#27760=CARTESIAN_POINT('Ctrl Pts',(-62.9468058203889,0.276857845483475,
16.9689814544543));
#27761=CARTESIAN_POINT('Ctrl Pts',(-62.9480689459238,0.00103910400151244,
16.9540747194623));
#27762=CARTESIAN_POINT('Origin',(-65.,8.88178419700125E-15,23.5459252805377));
#27763=CARTESIAN_POINT('',(-62.9444267867382,-0.0017991321662611,18.3540747194623));
#27764=CARTESIAN_POINT('',(-62.9473667479389,0.00148795945043925,18.2959252805377));
#27765=CARTESIAN_POINT('',(-62.94525,-1.20379215794662E-13,23.5459252805377));
#27766=CARTESIAN_POINT('Ctrl Pts',(-62.9473667479389,0.00148795945043927,
18.2959252805377));
#27767=CARTESIAN_POINT('Ctrl Pts',(-62.9503594142629,-0.444940986140601,
18.2717771392578));
#27768=CARTESIAN_POINT('Ctrl Pts',(-63.3129997156342,-1.58066882860308,
18.2105830344552));
#27769=CARTESIAN_POINT('Ctrl Pts',(-65.1869048686148,-2.42144210577607,
18.1123429661299));
#27770=CARTESIAN_POINT('Ctrl Pts',(-67.1357566643205,-1.15622609049766,
18.0012050755618));
#27771=CARTESIAN_POINT('Ctrl Pts',(-67.1297261640456,1.16729677790886,17.8900671849939));
#27772=CARTESIAN_POINT('Ctrl Pts',(-65.1743331530824,2.42237966744963,17.7789292944258));
#27773=CARTESIAN_POINT('Ctrl Pts',(-63.3084858902886,1.5735595002714,17.6808819929404));
#27774=CARTESIAN_POINT('Ctrl Pts',(-62.9503329736625,0.44145675564833,17.6198806549777));
#27775=CARTESIAN_POINT('Ctrl Pts',(-62.9474450730054,-0.00145098026756288,
17.5959252805377));
#27776=CARTESIAN_POINT('Ctrl Pts',(-62.9444267867382,-0.0017991321662612,
18.3540747194623));
#27777=CARTESIAN_POINT('Ctrl Pts',(-62.9432099184932,-0.13457659736896,
18.3468663500598));
#27778=CARTESIAN_POINT('Ctrl Pts',(-63.0154304430432,-0.948418981304482,
18.3026120171345));
#27779=CARTESIAN_POINT('Ctrl Pts',(-64.1011546824859,-2.25618948643599,
18.2213117206866));
#27780=CARTESIAN_POINT('Ctrl Pts',(-66.4080681763277,-1.97880214127948,
18.1101738301185));
#27781=CARTESIAN_POINT('Ctrl Pts',(-67.4261608997972,0.109805244932097,
17.9990359395505));
#27782=CARTESIAN_POINT('Ctrl Pts',(-66.2235610371465,2.09790664518148,17.8878980489825));
#27783=CARTESIAN_POINT('Ctrl Pts',(-63.9010218810697,2.16577030121657,17.7767601584144));
#27784=CARTESIAN_POINT('Ctrl Pts',(-62.9776665752518,0.823136293702514,
17.6988190485744));
#27785=CARTESIAN_POINT('Ctrl Pts',(-62.9422504791375,0.0719528572662148,
17.657923902257));
#27786=CARTESIAN_POINT('Ctrl Pts',(-62.9427422720288,0.00120218122683403,
17.6540747194623));
#27787=CARTESIAN_POINT('Origin',(-65.,8.88178419700125E-15,23.5459252805377));
#27788=CARTESIAN_POINT('',(-62.948587662066,-7.81015561640563E-5,19.0540747194623));
#27789=CARTESIAN_POINT('',(-62.9420758643114,0.000617377060639333,18.9959252805377));
#27790=CARTESIAN_POINT('',(-62.94525,-1.20379215794662E-13,23.5459252805377));
#27791=CARTESIAN_POINT('Ctrl Pts',(-62.9420758643114,0.000617377060639374,
18.9959252805377));
#27792=CARTESIAN_POINT('Ctrl Pts',(-62.9446352222011,-0.645933688463607,
18.9607195870605));
#27793=CARTESIAN_POINT('Ctrl Pts',(-63.621561854257,-1.97744992677628,18.8884679300607));
#27794=CARTESIAN_POINT('Ctrl Pts',(-65.88907520037,-2.26005765183972,18.7791703095382));
#27795=CARTESIAN_POINT('Ctrl Pts',(-67.3809865945794,-0.478767310881874,
18.6680324189701));
#27796=CARTESIAN_POINT('Ctrl Pts',(-66.6935539565454,1.74074417931049,18.5568945284021));
#27797=CARTESIAN_POINT('Ctrl Pts',(-64.4559921758773,2.36693278080145,18.445756637834));
#27798=CARTESIAN_POINT('Ctrl Pts',(-63.0943542721865,1.1613169625899,18.3587668885459));
#27799=CARTESIAN_POINT('Ctrl Pts',(-62.9457683276783,0.239931205144695,
18.3088231027804));
#27800=CARTESIAN_POINT('Ctrl Pts',(-62.9473667479389,0.00148795945043927,
18.2959252805377));
#27801=CARTESIAN_POINT('Ctrl Pts',(-62.948587662066,-7.81015561641604E-5,
19.0540747194623));
#27802=CARTESIAN_POINT('Ctrl Pts',(-62.9484730026856,-0.33826529995397,
19.0358087978625));
#27803=CARTESIAN_POINT('Ctrl Pts',(-63.1876491089047,-1.36219297688966,
18.98049691274));
#27804=CARTESIAN_POINT('Ctrl Pts',(-64.8026200998564,-2.42061047643985,
18.8881390640948));
#27805=CARTESIAN_POINT('Ctrl Pts',(-66.9266433003906,-1.4786343349792,18.7770011735268));
#27806=CARTESIAN_POINT('Ctrl Pts',(-67.2871880384261,0.816752582102682,
18.6658632829587));
#27807=CARTESIAN_POINT('Ctrl Pts',(-65.5542436264288,2.36455659820144,18.5547253923907));
#27808=CARTESIAN_POINT('Ctrl Pts',(-63.4592956564195,1.78804123877569,18.4507958712252));
#27809=CARTESIAN_POINT('Ctrl Pts',(-62.9494637678869,0.547806457359306,
18.3839123135824));
#27810=CARTESIAN_POINT('Ctrl Pts',(-62.9444267867382,-0.0017991321662612,
18.3540747194623));
#27811=CARTESIAN_POINT('Origin',(-65.,8.88178419700125E-15,23.5459252805377));
#27812=CARTESIAN_POINT('',(-62.9447134762142,0.00183968268686788,19.7540747194623));
#27813=CARTESIAN_POINT('',(-62.9455477186679,-0.00187702223999529,19.6959252805377));
#27814=CARTESIAN_POINT('',(-62.94525,-1.20379215794662E-13,23.5459252805377));
#27815=CARTESIAN_POINT('Ctrl Pts',(-62.9455477186679,-0.00187702223999513,
19.6959252805377));
#27816=CARTESIAN_POINT('Ctrl Pts',(-62.9440086170586,-0.171896041847231,
19.6867079983859));
#27817=CARTESIAN_POINT('Ctrl Pts',(-63.0410778177033,-1.02351952878432,
19.6404447527115));
#27818=CARTESIAN_POINT('Ctrl Pts',(-64.2244604721458,-2.30148946126117,
19.5571355435145));
#27819=CARTESIAN_POINT('Ctrl Pts',(-66.5130014322595,-1.89977418876313,
19.4459976529464));
#27820=CARTESIAN_POINT('Ctrl Pts',(-67.4166750228636,0.24082594437386,19.3348597623784));
#27821=CARTESIAN_POINT('Ctrl Pts',(-66.1083385580613,2.16099535909079,19.2237218718103));
#27822=CARTESIAN_POINT('Ctrl Pts',(-63.7855272416617,2.10318121447059,19.1125839812423));
#27823=CARTESIAN_POINT('Ctrl Pts',(-62.9580113964128,0.748427978399207,
19.0366517841514));
#27824=CARTESIAN_POINT('Ctrl Pts',(-62.9419420816985,0.034413858290589,
18.9977655505832));
#27825=CARTESIAN_POINT('Ctrl Pts',(-62.9420758643114,0.000617377060639374,
18.9959252805377));
#27826=CARTESIAN_POINT('Ctrl Pts',(-62.9447134762142,0.00183968268686788,
19.7540747194623));
#27827=CARTESIAN_POINT('Ctrl Pts',(-62.9497000514415,-0.538489713183419,
19.7247512456653));
#27828=CARTESIAN_POINT('Ctrl Pts',(-63.44501294369,-1.76953586229589,19.6583818083455));
#27829=CARTESIAN_POINT('Ctrl Pts',(-65.5214561645339,-2.37200281981328,
19.5549664075031));
#27830=CARTESIAN_POINT('Ctrl Pts',(-67.2756619344365,-0.848337588988209,
19.443828516935));
#27831=CARTESIAN_POINT('Ctrl Pts',(-66.9469285261459,1.45182065545647,19.332690626367));
#27832=CARTESIAN_POINT('Ctrl Pts',(-64.8361493591312,2.42311099039749,19.221552735799));
#27833=CARTESIAN_POINT('Ctrl Pts',(-63.1976100342287,1.38138540402115,19.1286807668307));
#27834=CARTESIAN_POINT('Ctrl Pts',(-62.9487055486976,0.347627856173917,
19.0728547613852));
#27835=CARTESIAN_POINT('Ctrl Pts',(-62.948587662066,-7.81015561641604E-5,
19.0540747194623));
#27836=CARTESIAN_POINT('Origin',(-65.,8.88178419700125E-15,23.5459252805377));
#27837=CARTESIAN_POINT('',(-62.9425383451584,-0.00106562935658971,20.4540747194623));
#27838=CARTESIAN_POINT('',(-62.9484657349091,0.000525555021686121,20.3959252805377));
#27839=CARTESIAN_POINT('',(-62.94525,-1.20379215794662E-13,23.5459252805377));
#27840=CARTESIAN_POINT('Ctrl Pts',(-62.9484657349091,0.000525555021685942,
20.3959252805377));
#27841=CARTESIAN_POINT('Ctrl Pts',(-62.9493249615497,-0.374800466557392,
20.3756504461887));
#27842=CARTESIAN_POINT('Ctrl Pts',(-63.2276318468978,-1.43710439466947,
20.318329648317));
#27843=CARTESIAN_POINT('Ctrl Pts',(-64.9337900137556,-2.42774204026717,
20.2239628869227));
#27844=CARTESIAN_POINT('Ctrl Pts',(-67.0037742079544,-1.37229889524426,
20.1128249963547));
#27845=CARTESIAN_POINT('Ctrl Pts',(-67.2396811477566,0.939225037877063,
20.0016871057866));
#27846=CARTESIAN_POINT('Ctrl Pts',(-65.4255825320509,2.3910656189328,19.8905492152186));
#27847=CARTESIAN_POINT('Ctrl Pts',(-63.4047034238819,1.71543774995269,19.7886286068023));
#27848=CARTESIAN_POINT('Ctrl Pts',(-62.9501945513868,0.511441876516725,
19.7237539619086));
#27849=CARTESIAN_POINT('Ctrl Pts',(-62.9455477186679,-0.00187702223999513,
19.6959252805377));
#27850=CARTESIAN_POINT('Ctrl Pts',(-62.9425383451584,-0.00106562935658957,
20.4540747194623));
#27851=CARTESIAN_POINT('Ctrl Pts',(-62.9421515159492,-0.0623504207905182,
20.4507396569907));
#27852=CARTESIAN_POINT('Ctrl Pts',(-62.9724324501069,-0.804000733271024,
20.4103586309964));
#27853=CARTESIAN_POINT('Ctrl Pts',(-63.8711449203827,-2.15034861017486,
20.3329316414794));
#27854=CARTESIAN_POINT('Ctrl Pts',(-66.1944008109328,-2.11464436694831,
20.2217937509113));
#27855=CARTESIAN_POINT('Ctrl Pts',(-67.4244083164919,-0.143381864737536,
20.1106558603433));
#27856=CARTESIAN_POINT('Ctrl Pts',(-66.4353272830534,1.95911953903996,19.9995179697752));
#27857=CARTESIAN_POINT('Ctrl Pts',(-64.132474966303,2.26841668404626,19.8883800792072));
#27858=CARTESIAN_POINT('Ctrl Pts',(-63.0217706588138,0.967627859876304,
19.8065656624362));
#27859=CARTESIAN_POINT('Ctrl Pts',(-62.9434002356266,0.144138246524585,
19.7617972091879));
#27860=CARTESIAN_POINT('Ctrl Pts',(-62.9447134762142,0.00183968268686788,
19.7540747194623));
#27861=CARTESIAN_POINT('Origin',(-65.,8.88178419700125E-15,23.5459252805377));
#27862=CARTESIAN_POINT('',(-62.9479182248742,-0.00116161895480638,21.1540747194623));
#27863=CARTESIAN_POINT('',(-62.9436210622307,0.00160392935066218,21.0959252805377));
#27864=CARTESIAN_POINT('',(-62.94525,-1.20379215794662E-13,23.5459252805377));
#27865=CARTESIAN_POINT('Ctrl Pts',(-62.9436210622307,0.00160392935066219,
21.0959252805377));
#27866=CARTESIAN_POINT('Ctrl Pts',(-62.9485686759719,-0.574950681266282,
21.0645928939915));
#27867=CARTESIAN_POINT('Ctrl Pts',(-63.5020551216143,-1.84152256699687,
20.9962145439225));
#27868=CARTESIAN_POINT('Ctrl Pts',(-65.648946524169,-2.34033682721966,20.8907902303309));
#27869=CARTESIAN_POINT('Ctrl Pts',(-67.3182024564633,-0.724053604371166,
20.7796523397629));
#27870=CARTESIAN_POINT('Ctrl Pts',(-66.865581542071,1.55496692328426,20.6685144491949));
#27871=CARTESIAN_POINT('Ctrl Pts',(-64.7053726085262,2.41070716562326,20.5573765586268));
#27872=CARTESIAN_POINT('Ctrl Pts',(-63.1597285921146,1.30632755500752,20.4665135024078));
#27873=CARTESIAN_POINT('Ctrl Pts',(-62.9477549916925,0.310991282228741,
20.4126964097114));
#27874=CARTESIAN_POINT('Ctrl Pts',(-62.9484657349091,0.000525555021685942,
20.3959252805377));
#27875=CARTESIAN_POINT('Ctrl Pts',(-62.9479182248742,-0.00116161895480603,
21.1540747194623));
#27876=CARTESIAN_POINT('Ctrl Pts',(-62.9465403381585,-0.267421145958312,
21.1396821047934));
#27877=CARTESIAN_POINT('Ctrl Pts',(-63.1184075387479,-1.21731587450749,
21.0882435266019));
#27878=CARTESIAN_POINT('Ctrl Pts',(-64.5516876929394,-2.38689686810909,
20.9997589848876));
#27879=CARTESIAN_POINT('Ctrl Pts',(-66.7622271403759,-1.67118893435551,
20.8886210943196));
#27880=CARTESIAN_POINT('Ctrl Pts',(-67.3597936726881,0.574194749175807,
20.7774832037516));
#27881=CARTESIAN_POINT('Ctrl Pts',(-65.7974074532359,2.29400261230211,20.6663453131835));
#27882=CARTESIAN_POINT('Ctrl Pts',(-63.573935456952,1.92548892520574,20.5585424850871));
#27883=CARTESIAN_POINT('Ctrl Pts',(-62.9464484251963,0.618402688713493,
20.4877856205134));
#27884=CARTESIAN_POINT('Ctrl Pts',(-62.9425383451584,-0.00106562935658957,
20.4540747194623));
#27885=CARTESIAN_POINT('Origin',(-65.,8.88178419700125E-15,23.5459252805377));
#27886=CARTESIAN_POINT('',(-62.9473239618077,0.00235074752841319,21.8540747194623));
#27887=CARTESIAN_POINT('',(-62.9434348764936,-0.00149614206265777,21.7959252805377));
#27888=CARTESIAN_POINT('',(-62.94525,-1.20379215794662E-13,23.5459252805377));
#27889=CARTESIAN_POINT('',(-64.4698297828114,1.98517432567172,22.));
#27890=CARTESIAN_POINT('Ctrl Pts',(-64.4698297828114,1.98517432567173,22.));
#27891=CARTESIAN_POINT('Ctrl Pts',(-63.8097120902545,1.8088801151799,21.9629540364773));
#27892=CARTESIAN_POINT('Ctrl Pts',(-63.0750422655367,1.11280694816752,21.9143122762981));
#27893=CARTESIAN_POINT('Ctrl Pts',(-62.9457054195483,0.216594706141787,
21.8656705161189));
#27894=CARTESIAN_POINT('Ctrl Pts',(-62.9473239618077,0.00235074752841319,
21.8540747194623));
#27895=CARTESIAN_POINT('',(-65.5313040526013,1.98873440678486,22.));
#27896=CARTESIAN_POINT('Origin',(-65.,8.88178419700125E-15,22.));
#27897=CARTESIAN_POINT('Ctrl Pts',(-65.5313046873329,1.98873639975132,22.));
#27898=CARTESIAN_POINT('Ctrl Pts',(-64.8866967734446,2.16006352763734,21.9636770818144));
#27899=CARTESIAN_POINT('Ctrl Pts',(-63.5069411366323,1.84063802220702,21.895652175327));
#27900=CARTESIAN_POINT('Ctrl Pts',(-62.9482922133912,0.581586231880553,
21.8276272688395));
#27901=CARTESIAN_POINT('Ctrl Pts',(-62.9434348764936,-0.00149614206265759,
21.7959252805377));
#27902=CARTESIAN_POINT('Origin',(-32.5,-56.2916512459885,17.));
#27903=CARTESIAN_POINT('',(-31.6672724934037,-54.8468960395934,13.8714803633902));
#27904=CARTESIAN_POINT('',(-31.6651566506306,-54.8475988206465,13.6785196366098));
#27905=CARTESIAN_POINT('',(-31.667,-54.8488529232836,17.));
#27906=CARTESIAN_POINT('',(-31.9588970197441,-54.7159724828016,13.));
#27907=CARTESIAN_POINT('Ctrl Pts',(-31.6651566506306,-54.8475988206465,
13.6785196366098));
#27908=CARTESIAN_POINT('Ctrl Pts',(-31.6146486514652,-54.8762889946568,
13.6746222055426));
#27909=CARTESIAN_POINT('Ctrl Pts',(-31.5657632473174,-54.9077117506003,
13.6707247744754));
#27910=CARTESIAN_POINT('Ctrl Pts',(-31.5188321868552,-54.9418237568819,
13.6668273434082));
#27911=CARTESIAN_POINT('Ctrl Pts',(-31.0727418458088,-55.2660660894878,
13.6297813798856));
#27912=CARTESIAN_POINT('Ctrl Pts',(-30.8032251342758,-55.8332803703507,
13.5927354163629));
#27913=CARTESIAN_POINT('Ctrl Pts',(-30.8337540098498,-56.3839156387154,
13.5556894528402));
#27914=CARTESIAN_POINT('Ctrl Pts',(-30.8642828854237,-56.93455090708,13.5186434893175));
#27915=CARTESIAN_POINT('Ctrl Pts',(-31.1948573481046,-57.4686071629464,
13.4815975257948));
#27916=CARTESIAN_POINT('Ctrl Pts',(-31.6739356569701,-57.7415946577538,
13.4445515622722));
#27917=CARTESIAN_POINT('Ctrl Pts',(-32.1530139658356,-58.0145821525613,
13.4075055987495));
#27918=CARTESIAN_POINT('Ctrl Pts',(-32.7805961208857,-58.0265008863097,
13.3704596352268));
#27919=CARTESIAN_POINT('Ctrl Pts',(-33.2699721109727,-57.7720492096737,
13.3334136717041));
#27920=CARTESIAN_POINT('Ctrl Pts',(-33.7593481010598,-57.5175975330377,
13.2963677081814));
#27921=CARTESIAN_POINT('Ctrl Pts',(-34.1105179261839,-56.9967754460171,
13.2593217446588));
#27922=CARTESIAN_POINT('Ctrl Pts',(-34.1617369653364,-56.4476202824107,
13.2222757811361));
#27923=CARTESIAN_POINT('Ctrl Pts',(-34.2129560044889,-55.8984651188042,
13.1852298176134));
#27924=CARTESIAN_POINT('Ctrl Pts',(-33.9642242576698,-55.3209768786118,
13.1481838540907));
#27925=CARTESIAN_POINT('Ctrl Pts',(-33.5316971804146,-54.9803713160329,
13.111137890568));
#27926=CARTESIAN_POINT('Ctrl Pts',(-33.0991701031595,-54.639765753454,13.0740919270454));
#27927=CARTESIAN_POINT('Ctrl Pts',(-32.4828476954683,-54.5360428684886,
13.0370459635227));
#27928=CARTESIAN_POINT('Ctrl Pts',(-31.9588970197442,-54.7159724828016,
13.));
#27929=CARTESIAN_POINT('',(-31.0290140863629,-57.0802261258962,13.));
#27930=CARTESIAN_POINT('Origin',(-32.5,-56.2916512459885,13.));
#27931=CARTESIAN_POINT('',(-31.6688354432562,-54.8507324474214,13.1714803633902));
#27932=CARTESIAN_POINT('Ctrl Pts',(-31.029012445651,-57.0802271145805,13.));
#27933=CARTESIAN_POINT('Ctrl Pts',(-30.774120583937,-56.6032768580682,13.0363229181856));
#27934=CARTESIAN_POINT('Ctrl Pts',(-30.7719333897513,-55.9901147282721,
13.0726458363711));
#27935=CARTESIAN_POINT('Ctrl Pts',(-31.0246770579875,-55.5119982833858,
13.1089687545567));
#27936=CARTESIAN_POINT('Ctrl Pts',(-31.1696673663398,-55.2377194013227,
13.1298059575012));
#27937=CARTESIAN_POINT('Ctrl Pts',(-31.3985533923309,-55.0078829792344,
13.1506431604457));
#27938=CARTESIAN_POINT('Ctrl Pts',(-31.6688354432562,-54.8507324474214,
13.1714803633902));
#27939=CARTESIAN_POINT('',(-31.667,-54.8488529232836,12.));
#27940=CARTESIAN_POINT('',(-31.667,-54.8488529232836,17.));
#27941=CARTESIAN_POINT('Origin',(-32.5,-56.2916512459885,12.));
#27942=CARTESIAN_POINT('Ctrl Pts',(-31.6688354432562,-54.8507324474214,
13.1714803633902));
#27943=CARTESIAN_POINT('Ctrl Pts',(-31.8790813703937,-54.7284888165622,
13.1876891239684));
#27944=CARTESIAN_POINT('Ctrl Pts',(-32.1143756641563,-54.6502267716398,
13.2038978845465));
#27945=CARTESIAN_POINT('Ctrl Pts',(-32.3547143198851,-54.6292400960994,
13.2201066451247));
#27946=CARTESIAN_POINT('Ctrl Pts',(-32.9040207909308,-54.5812739599609,
13.2571526086474));
#27947=CARTESIAN_POINT('Ctrl Pts',(-33.4796777351052,-54.8324998905166,
13.2941985721701));
#27948=CARTESIAN_POINT('Ctrl Pts',(-33.8179820369827,-55.2680242179701,
13.3312445356928));
#27949=CARTESIAN_POINT('Ctrl Pts',(-34.1562863388601,-55.7035485454237,
13.3682904992154));
#27950=CARTESIAN_POINT('Ctrl Pts',(-34.2572379984406,-56.323371269775,13.4053364627381));
#27951=CARTESIAN_POINT('Ctrl Pts',(-34.0747609720031,-56.8437863823056,
13.4423824262608));
#27952=CARTESIAN_POINT('Ctrl Pts',(-33.8922839455656,-57.3642014948362,
13.4794283897835));
#27953=CARTESIAN_POINT('Ctrl Pts',(-33.4263782331101,-57.7852089955461,
13.5164743533062));
#27954=CARTESIAN_POINT('Ctrl Pts',(-32.8902057561615,-57.9141527098528,
13.5535203168288));
#27955=CARTESIAN_POINT('Ctrl Pts',(-32.3540332792128,-58.0430964241595,
13.5905662803515));
#27956=CARTESIAN_POINT('Ctrl Pts',(-31.7475940377709,-57.879976352063,13.6276122438742));
#27957=CARTESIAN_POINT('Ctrl Pts',(-31.3484595971706,-57.499435180452,13.6646582073969));
#27958=CARTESIAN_POINT('Ctrl Pts',(-30.9493251565703,-57.1188940088411,
13.7017041709196));
#27959=CARTESIAN_POINT('Ctrl Pts',(-30.7574955168115,-56.5209317377157,
13.7387501344422));
#27960=CARTESIAN_POINT('Ctrl Pts',(-30.8607470097836,-55.9792142563288,
13.7757960979649));
#27961=CARTESIAN_POINT('Ctrl Pts',(-30.9496414742062,-55.5128221104134,
13.8076908531067));
#27962=CARTESIAN_POINT('Ctrl Pts',(-31.2572608237869,-55.0881206516064,
13.8395856082484));
#27963=CARTESIAN_POINT('Ctrl Pts',(-31.6672724934037,-54.8468960395934,
13.8714803633902));
#27964=CARTESIAN_POINT('Origin',(-32.5,-56.2916512459885,17.));
#27965=CARTESIAN_POINT('',(-31.6652293984911,-54.8484357012869,14.5714803633902));
#27966=CARTESIAN_POINT('',(-31.6674240358463,-54.8512520230129,14.3785196366098));
#27967=CARTESIAN_POINT('',(-31.667,-54.8488529232836,17.));
#27968=CARTESIAN_POINT('Ctrl Pts',(-31.6674240358463,-54.8512520230129,
14.3785196366098));
#27969=CARTESIAN_POINT('Ctrl Pts',(-31.4726121759195,-54.9625548712859,
14.3635646533454));
#27970=CARTESIAN_POINT('Ctrl Pts',(-31.2997293296832,-55.1111079954895,
14.3486096700809));
#27971=CARTESIAN_POINT('Ctrl Pts',(-31.1659805795344,-55.289072307877,14.3336546868165));
#27972=CARTESIAN_POINT('Ctrl Pts',(-30.8346628353681,-55.7299193023853,
14.2966087232938));
#27973=CARTESIAN_POINT('Ctrl Pts',(-30.7434854934753,-56.3512435601479,
14.2595627597711));
#27974=CARTESIAN_POINT('Ctrl Pts',(-30.9341783443449,-56.8686931008725,
14.2225167962484));
#27975=CARTESIAN_POINT('Ctrl Pts',(-31.1248711952146,-57.386142641597,14.1854708327258));
#27976=CARTESIAN_POINT('Ctrl Pts',(-31.5974342388466,-57.7997174652835,
14.1484248692031));
#27977=CARTESIAN_POINT('Ctrl Pts',(-32.1355923903503,-57.9201415291698,
14.1113789056804));
#27978=CARTESIAN_POINT('Ctrl Pts',(-32.6737505418539,-58.0405655930561,
14.0743329421577));
#27979=CARTESIAN_POINT('Ctrl Pts',(-33.2775038012292,-57.8678388971422,
14.037286978635));
#27980=CARTESIAN_POINT('Ctrl Pts',(-33.6705489274,-57.4810131538507,14.0002410151124));
#27981=CARTESIAN_POINT('Ctrl Pts',(-34.0635940535707,-57.0941874105591,
13.9631950515897));
#27982=CARTESIAN_POINT('Ctrl Pts',(-34.245931046537,-56.4932626198898,13.926149088067));
#27983=CARTESIAN_POINT('Ctrl Pts',(-34.1340966146064,-55.9532506956148,
13.8891031245443));
#27984=CARTESIAN_POINT('Ctrl Pts',(-34.0222621826759,-55.4132387713397,
13.8520571610216));
#27985=CARTESIAN_POINT('Ctrl Pts',(-33.6162563258487,-54.934139713459,13.815011197499));
#27986=CARTESIAN_POINT('Ctrl Pts',(-33.1019214121551,-54.7352253766931,
13.7779652339763));
#27987=CARTESIAN_POINT('Ctrl Pts',(-32.6416972484853,-54.5572378789698,
13.7448167015208));
#27988=CARTESIAN_POINT('Ctrl Pts',(-32.0947386036493,-54.6035824036932,
13.7116681690653));
#27989=CARTESIAN_POINT('Ctrl Pts',(-31.6651566506306,-54.8475988206465,
13.6785196366098));
#27990=CARTESIAN_POINT('Ctrl Pts',(-31.6672724934037,-54.8468960395934,
13.8714803633902));
#27991=CARTESIAN_POINT('Ctrl Pts',(-31.7334920188216,-54.8079367110906,
13.8766315717711));
#27992=CARTESIAN_POINT('Ctrl Pts',(-31.8023823793453,-54.7737632532799,
13.881782780152));
#27993=CARTESIAN_POINT('Ctrl Pts',(-31.8734534906151,-54.7449729811027,
13.886933988533));
#27994=CARTESIAN_POINT('Ctrl Pts',(-32.3845758527715,-54.537921878912,13.9239799520556));
#27995=CARTESIAN_POINT('Ctrl Pts',(-33.0084879513813,-54.609292366179,13.9610259155783));
#27996=CARTESIAN_POINT('Ctrl Pts',(-33.4596489857383,-54.9264225988407,
13.998071879101));
#27997=CARTESIAN_POINT('Ctrl Pts',(-33.9108100200953,-55.2435528315024,
14.0351178426237));
#27998=CARTESIAN_POINT('Ctrl Pts',(-34.1892199901994,-55.8064428095589,
14.0721638061464));
#27999=CARTESIAN_POINT('Ctrl Pts',(-34.1674649383537,-56.3574821112236,
14.109209769669));
#28000=CARTESIAN_POINT('Ctrl Pts',(-34.1457098865079,-56.9085214128884,
14.1462557331917));
#28001=CARTESIAN_POINT('Ctrl Pts',(-33.8237898127121,-57.4477100381614,
14.1833016967144));
#28002=CARTESIAN_POINT('Ctrl Pts',(-33.3490322930752,-57.7282855707718,
14.2203476602371));
#28003=CARTESIAN_POINT('Ctrl Pts',(-32.8742747734383,-58.0088611033821,
14.2573936237598));
#28004=CARTESIAN_POINT('Ctrl Pts',(-32.2466798079601,-58.0308235433297,
14.2944395872824));
#28005=CARTESIAN_POINT('Ctrl Pts',(-31.7534702764193,-57.7841214978257,
14.3314855508051));
#28006=CARTESIAN_POINT('Ctrl Pts',(-31.2602607448784,-57.5374194523217,
14.3685315143278));
#28007=CARTESIAN_POINT('Ctrl Pts',(-30.901436647275,-57.0220529213661,14.4055774778505));
#28008=CARTESIAN_POINT('Ctrl Pts',(-30.8412156241946,-56.4738823989159,
14.4426234413732));
#28009=CARTESIAN_POINT('Ctrl Pts',(-30.7809946011143,-55.9257118764658,
14.4796694048958));
#28010=CARTESIAN_POINT('Ctrl Pts',(-31.0193766525571,-55.3447373625211,
14.5167153684185));
#28011=CARTESIAN_POINT('Ctrl Pts',(-31.4472650020351,-54.9968450984028,
14.5537613319412));
#28012=CARTESIAN_POINT('Ctrl Pts',(-31.5154844642033,-54.9413796406974,
14.5596676757575));
#28013=CARTESIAN_POINT('Ctrl Pts',(-31.5885209558805,-54.8918388624727,
14.5655740195739));
#28014=CARTESIAN_POINT('Ctrl Pts',(-31.6652293984911,-54.8484357012869,
14.5714803633902));
#28015=CARTESIAN_POINT('Origin',(-32.5,-56.2916512459885,17.));
#28016=CARTESIAN_POINT('',(-31.6679812524744,-54.8513129979877,15.2714803633902));
#28017=CARTESIAN_POINT('',(-31.6687468960362,-54.8490160493388,15.0785196366098));
#28018=CARTESIAN_POINT('',(-31.667,-54.8488529232836,17.));
#28019=CARTESIAN_POINT('Ctrl Pts',(-31.6687468960362,-54.8490160493388,
15.0785196366098));
#28020=CARTESIAN_POINT('Ctrl Pts',(-31.3330220839915,-55.0465316965332,
15.0525071011481));
#28021=CARTESIAN_POINT('Ctrl Pts',(-31.0621374285877,-55.3603795470759,
15.0264945656864));
#28022=CARTESIAN_POINT('Ctrl Pts',(-30.930547953771,-55.7245591059458,15.0004820302247));
#28023=CARTESIAN_POINT('Ctrl Pts',(-30.7431437350931,-56.2432083807723,
14.9634360667021));
#28024=CARTESIAN_POINT('Ctrl Pts',(-30.8382616710438,-56.8639417522836,
14.9263901031794));
#28025=CARTESIAN_POINT('Ctrl Pts',(-31.1723705294372,-57.3026770823852,
14.8893441396567));
#28026=CARTESIAN_POINT('Ctrl Pts',(-31.5064793878306,-57.7414124124868,
14.852298176134));
#28027=CARTESIAN_POINT('Ctrl Pts',(-32.0795791686666,-57.9981497011789,
14.8152522126113));
#28028=CARTESIAN_POINT('Ctrl Pts',(-32.6293874463964,-57.9553916541296,
14.7782062490887));
#28029=CARTESIAN_POINT('Ctrl Pts',(-33.1791957241262,-57.9126336070803,
14.741160285566));
#28030=CARTESIAN_POINT('Ctrl Pts',(-33.7057124987497,-57.5703802242898,
14.7041143220433));
#28031=CARTESIAN_POINT('Ctrl Pts',(-33.9679745051883,-57.0852657438482,
14.6670683585206));
#28032=CARTESIAN_POINT('Ctrl Pts',(-34.230236511627,-56.6001512634066,14.6300223949979));
#28033=CARTESIAN_POINT('Ctrl Pts',(-34.2282437498808,-55.9721756853139,
14.5929764314753));
#28034=CARTESIAN_POINT('Ctrl Pts',(-33.9629079737486,-55.4887355202075,
14.5559304679526));
#28035=CARTESIAN_POINT('Ctrl Pts',(-33.6975721976164,-55.0052953551011,
14.5188845044299));
#28036=CARTESIAN_POINT('Ctrl Pts',(-33.1688934070984,-54.6663906029808,
14.4818385409072));
#28037=CARTESIAN_POINT('Ctrl Pts',(-32.6188249386194,-54.6271230925477,
14.4447925773845));
#28038=CARTESIAN_POINT('Ctrl Pts',(-32.2908120993686,-54.6037073755496,
14.4227015971263));
#28039=CARTESIAN_POINT('Ctrl Pts',(-31.955193328237,-54.6868393332485,14.400610616868));
#28040=CARTESIAN_POINT('Ctrl Pts',(-31.6674240358463,-54.8512520230129,
14.3785196366098));
#28041=CARTESIAN_POINT('Ctrl Pts',(-31.6652293984911,-54.8484357012869,
14.5714803633902));
#28042=CARTESIAN_POINT('Ctrl Pts',(-32.0696541670855,-54.6196041304525,
14.6026199830966));
#28043=CARTESIAN_POINT('Ctrl Pts',(-32.5761460954187,-54.5613764565911,
14.6337596028029));
#28044=CARTESIAN_POINT('Ctrl Pts',(-33.0168947227899,-54.7049585292357,
14.6648992225093));
#28045=CARTESIAN_POINT('Ctrl Pts',(-33.5412414465535,-54.8757742384787,
14.7019451860319));
#28046=CARTESIAN_POINT('Ctrl Pts',(-33.9725402465673,-55.3322156712569,
14.7389911495546));
#28047=CARTESIAN_POINT('Ctrl Pts',(-34.1134048115911,-55.8653898078431,
14.7760371130773));
#28048=CARTESIAN_POINT('Ctrl Pts',(-34.2542693766149,-56.3985639444293,
14.8130830766));
#28049=CARTESIAN_POINT('Ctrl Pts',(-34.1046997066486,-57.0084707848236,
14.8501290401227));
#28050=CARTESIAN_POINT('Ctrl Pts',(-33.7331471941746,-57.415983010017,14.8871750036453));
#28051=CARTESIAN_POINT('Ctrl Pts',(-33.3615946817007,-57.8234952352103,
14.924220967168));
#28052=CARTESIAN_POINT('Ctrl Pts',(-32.7680593267192,-58.0286128452026,
14.9612669306907));
#28053=CARTESIAN_POINT('Ctrl Pts',(-32.2241759575529,-57.9374626002348,
14.9983128942134));
#28054=CARTESIAN_POINT('Ctrl Pts',(-31.6802925883866,-57.8463123552671,
15.0353588577361));
#28055=CARTESIAN_POINT('Ctrl Pts',(-31.1860612050356,-57.4588942553394,
15.0724048212587));
#28056=CARTESIAN_POINT('Ctrl Pts',(-30.9676695988057,-56.9525123919175,
15.1094507847814));
#28057=CARTESIAN_POINT('Ctrl Pts',(-30.7492779925757,-56.4461305284957,
15.1464967483041));
#28058=CARTESIAN_POINT('Ctrl Pts',(-30.8067261634667,-55.8207849015799,
15.1835427118268));
#28059=CARTESIAN_POINT('Ctrl Pts',(-31.1137226321993,-55.3626684826674,
15.2205886753495));
#28060=CARTESIAN_POINT('Ctrl Pts',(-31.2543008673673,-55.1528901815095,
15.2375525713631));
#28061=CARTESIAN_POINT('Ctrl Pts',(-31.4472058843405,-54.9781775023347,
15.2545164673766));
#28062=CARTESIAN_POINT('Ctrl Pts',(-31.6679812524744,-54.8513129979877,
15.2714803633902));
#28063=CARTESIAN_POINT('Origin',(-32.5,-56.2916512459885,17.));
#28064=CARTESIAN_POINT('',(-31.668393257303,-54.8482192502339,15.9714803633902));
#28065=CARTESIAN_POINT('',(-31.6656122060936,-54.8464626161313,15.7785196366098));
#28066=CARTESIAN_POINT('',(-31.667,-54.8488529232836,17.));
#28067=CARTESIAN_POINT('Ctrl Pts',(-31.6656122129471,-54.8464626279357,
15.7785196366098));
#28068=CARTESIAN_POINT('Ctrl Pts',(-31.187699049881,-55.1223478631842,15.7414495489509));
#28069=CARTESIAN_POINT('Ctrl Pts',(-30.860252864304,-55.6587877650758,15.7043794612919));
#28070=CARTESIAN_POINT('Ctrl Pts',(-30.8332370510141,-56.2099535888295,
15.667309373633));
#28071=CARTESIAN_POINT('Ctrl Pts',(-30.8062388188308,-56.7607607298753,
15.6302634101103));
#28072=CARTESIAN_POINT('Ctrl Pts',(-31.0792800051602,-57.3262745318078,
15.5932174465876));
#28073=CARTESIAN_POINT('Ctrl Pts',(-31.5274017633056,-57.6476843966343,
15.556171483065));
#28074=CARTESIAN_POINT('Ctrl Pts',(-31.9755235214509,-57.9690942614608,
15.5191255195423));
#28075=CARTESIAN_POINT('Ctrl Pts',(-32.5987258514122,-58.0464001891811,
15.4820795560196));
#28076=CARTESIAN_POINT('Ctrl Pts',(-33.1117966721332,-57.8442226833339,
15.4450335924969));
#28077=CARTESIAN_POINT('Ctrl Pts',(-33.6248674928541,-57.6420451774866,
15.4079876289742));
#28078=CARTESIAN_POINT('Ctrl Pts',(-34.0278068043346,-57.1603842380717,
15.3709416654516));
#28079=CARTESIAN_POINT('Ctrl Pts',(-34.1362071477596,-56.6196747257878,
15.3338957019289));
#28080=CARTESIAN_POINT('Ctrl Pts',(-34.2446074911845,-56.0789652135039,
15.2968497384062));
#28081=CARTESIAN_POINT('Ctrl Pts',(-34.0584688665537,-55.479207128351,15.2598037748835));
#28082=CARTESIAN_POINT('Ctrl Pts',(-33.6629786670949,-55.0948831577141,
15.2227578113608));
#28083=CARTESIAN_POINT('Ctrl Pts',(-33.267488467636,-54.7105591870771,15.1857118478381));
#28084=CARTESIAN_POINT('Ctrl Pts',(-32.662646693349,-54.5416693309562,15.1486658843155));
#28085=CARTESIAN_POINT('Ctrl Pts',(-32.1252626195522,-54.6655069919667,
15.1116199207928));
#28086=CARTESIAN_POINT('Ctrl Pts',(-31.9652131038814,-54.7023896586347,
15.1005864927318));
#28087=CARTESIAN_POINT('Ctrl Pts',(-31.8111473001585,-54.7652381843378,
15.0895530646708));
#28088=CARTESIAN_POINT('Ctrl Pts',(-31.6687468960362,-54.8490160493388,
15.0785196366098));
#28089=CARTESIAN_POINT('Ctrl Pts',(-31.6679812524744,-54.8513129979877,
15.2714803633902));
#28090=CARTESIAN_POINT('Ctrl Pts',(-31.9293378325702,-54.7011292466392,
15.2915624308993));
#28091=CARTESIAN_POINT('Ctrl Pts',(-32.2297522401559,-54.6180004723649,
15.3116444984084));
#28092=CARTESIAN_POINT('Ctrl Pts',(-32.5286510627353,-54.6231330317608,
15.3317265659175));
#28093=CARTESIAN_POINT('Ctrl Pts',(-33.0800382579646,-54.6326012106758,
15.3687725294402));
#28094=CARTESIAN_POINT('Ctrl Pts',(-33.626267881849,-54.9424247794149,15.4058184929629));
#28095=CARTESIAN_POINT('Ctrl Pts',(-33.9173548501551,-55.4108112247729,
15.4428644564855));
#28096=CARTESIAN_POINT('Ctrl Pts',(-34.2084418184611,-55.8791976701309,
15.4799104200082));
#28097=CARTESIAN_POINT('Ctrl Pts',(-34.2443861311887,-56.5061469921078,
15.5169563835309));
#28098=CARTESIAN_POINT('Ctrl Pts',(-34.0087376695652,-57.0047322785327,
15.5540023470536));
#28099=CARTESIAN_POINT('Ctrl Pts',(-33.7730892079418,-57.5033175649576,
15.5910483105763));
#28100=CARTESIAN_POINT('Ctrl Pts',(-33.2658479719674,-57.8735388158304,
15.628094274099));
#28101=CARTESIAN_POINT('Ctrl Pts',(-32.7191557896563,-57.9459621763539,
15.6651402376216));
#28102=CARTESIAN_POINT('Ctrl Pts',(-32.1724636073452,-58.0183855368774,
15.7021862011443));
#28103=CARTESIAN_POINT('Ctrl Pts',(-31.5863204786975,-57.7930110070515,
15.739232164667));
#28104=CARTESIAN_POINT('Ctrl Pts',(-31.2289781301378,-57.3729825184307,
15.7762781281897));
#28105=CARTESIAN_POINT('Ctrl Pts',(-30.8716357815781,-56.9529540298098,
15.8133240917123));
#28106=CARTESIAN_POINT('Ctrl Pts',(-30.7430942131064,-56.3382715823939,
15.850370055235));
#28107=CARTESIAN_POINT('Ctrl Pts',(-30.9021812024434,-55.8102480837199,
15.8874160187577));
#28108=CARTESIAN_POINT('Ctrl Pts',(-31.022514091882,-55.4108527997199,15.9154374669685));
#28109=CARTESIAN_POINT('Ctrl Pts',(-31.3074096675184,-55.0610382301548,
15.9434589151794));
#28110=CARTESIAN_POINT('Ctrl Pts',(-31.668393257303,-54.8482192502339,15.9714803633902));
#28111=CARTESIAN_POINT('Origin',(-32.5,-56.2916512459885,17.));
#28112=CARTESIAN_POINT('',(-31.6652521719754,-54.8469263020217,16.6714803633902));
#28113=CARTESIAN_POINT('',(-31.6662812667712,-54.8504621893828,16.4785196366098));
#28114=CARTESIAN_POINT('',(-31.667,-54.8488529232836,17.));
#28115=CARTESIAN_POINT('Ctrl Pts',(-31.6662812667712,-54.8504621893828,
16.4785196366098));
#28116=CARTESIAN_POINT('Ctrl Pts',(-31.5218969898699,-54.9322586741207,
16.4674379602763));
#28117=CARTESIAN_POINT('Ctrl Pts',(-31.3899082837209,-55.0347971411717,
16.4563562839428));
#28118=CARTESIAN_POINT('Ctrl Pts',(-31.2776094808925,-55.1556342327712,
16.4452746076093));
#28119=CARTESIAN_POINT('Ctrl Pts',(-30.9021953983998,-55.5595917526322,
16.4082286440866));
#28120=CARTESIAN_POINT('Ctrl Pts',(-30.7468278084228,-56.1680473893291,
16.3711826805639));
#28121=CARTESIAN_POINT('Ctrl Pts',(-30.8826115695051,-56.7025379705484,
16.3341367170412));
#28122=CARTESIAN_POINT('Ctrl Pts',(-31.0183953305873,-57.2370285517677,
16.2970907535186));
#28123=CARTESIAN_POINT('Ctrl Pts',(-31.4453304427287,-57.6975540775093,
16.2600447899959));
#28124=CARTESIAN_POINT('Ctrl Pts',(-31.9680276309783,-57.8733524295625,
16.2229988264732));
#28125=CARTESIAN_POINT('Ctrl Pts',(-32.490724819228,-58.0491507816157,16.1859528629505));
#28126=CARTESIAN_POINT('Ctrl Pts',(-33.109184083586,-57.9402219599804,16.1489068994278));
#28127=CARTESIAN_POINT('Ctrl Pts',(-33.5403640348016,-57.596417857542,16.1118609359052));
#28128=CARTESIAN_POINT('Ctrl Pts',(-33.9715439860171,-57.2526137551037,
16.0748149723825));
#28129=CARTESIAN_POINT('Ctrl Pts',(-34.2154446240901,-56.6739343718623,
16.0377690088598));
#28130=CARTESIAN_POINT('Ctrl Pts',(-34.1604434390255,-56.1252156089025,
16.0007230453371));
#28131=CARTESIAN_POINT('Ctrl Pts',(-34.1054422539609,-55.5764968459426,
15.9636770818144));
#28132=CARTESIAN_POINT('Ctrl Pts',(-33.7515392457587,-55.0577387032643,
15.9266311182918));
#28133=CARTESIAN_POINT('Ctrl Pts',(-33.2607001328297,-54.8063537864051,
15.8895851547691));
#28134=CARTESIAN_POINT('Ctrl Pts',(-32.7701806517449,-54.5551325700793,
15.8525633153826));
#28135=CARTESIAN_POINT('Ctrl Pts',(-32.1429033520047,-54.5709364688817,
15.8155414759962));
#28136=CARTESIAN_POINT('Ctrl Pts',(-31.6656122129471,-54.8464626279357,
15.7785196366098));
#28137=CARTESIAN_POINT('Ctrl Pts',(-31.668393257303,-54.8482192502339,15.9714803633902));
#28138=CARTESIAN_POINT('Ctrl Pts',(-31.7846507008451,-54.7796793186608,
15.9805048787021));
#28139=CARTESIAN_POINT('Ctrl Pts',(-31.9088000679097,-54.7253487041335,
15.9895293940139));
#28140=CARTESIAN_POINT('Ctrl Pts',(-32.0378859406647,-54.688147422912,15.9985539093258));
#28141=CARTESIAN_POINT('Ctrl Pts',(-32.5677881424037,-54.5354348107102,
16.0355998728484));
#28142=CARTESIAN_POINT('Ctrl Pts',(-33.180876998736,-54.6713741362387,16.0726458363711));
#28143=CARTESIAN_POINT('Ctrl Pts',(-33.5965689181183,-55.0337519963386,
16.1096917998938));
#28144=CARTESIAN_POINT('Ctrl Pts',(-34.0122608375006,-55.3961298564385,
16.1467377634165));
#28145=CARTESIAN_POINT('Ctrl Pts',(-34.2305558199328,-55.9849462511098,
16.1837837269391));
#28146=CARTESIAN_POINT('Ctrl Pts',(-34.1515499288845,-56.5307260185163,
16.2208296904618));
#28147=CARTESIAN_POINT('Ctrl Pts',(-34.0725440378362,-57.0765057859228,
16.2578756539845));
#28148=CARTESIAN_POINT('Ctrl Pts',(-33.6962372733073,-57.5792489260645,
16.2949216175072));
#28149=CARTESIAN_POINT('Ctrl Pts',(-33.1948485598908,-57.8088721901075,
16.3319675810299));
#28150=CARTESIAN_POINT('Ctrl Pts',(-32.6934598464744,-58.0384954541505,
16.3690135445526));
#28151=CARTESIAN_POINT('Ctrl Pts',(-32.0669891841703,-57.9949988420949,
16.4060595080752));
#28152=CARTESIAN_POINT('Ctrl Pts',(-31.6021444239114,-57.6982888250906,
16.4431054715979));
#28153=CARTESIAN_POINT('Ctrl Pts',(-31.1372996636525,-57.4015788080863,
16.4801514351206));
#28154=CARTESIAN_POINT('Ctrl Pts',(-30.8340808054389,-56.8516553861334,
16.5171973986433));
#28155=CARTESIAN_POINT('Ctrl Pts',(-30.8312576791002,-56.3001941315665,
16.554243362166));
#28156=CARTESIAN_POINT('Ctrl Pts',(-30.8284345527615,-55.7487328769995,
16.5912893256886));
#28157=CARTESIAN_POINT('Ctrl Pts',(-31.1260071582979,-55.1957337898185,
16.6283352892113));
#28158=CARTESIAN_POINT('Ctrl Pts',(-31.5877897054339,-54.8942800379899,
16.665381252734));
#28159=CARTESIAN_POINT('Ctrl Pts',(-31.6131317633018,-54.8777366270908,
16.6674142896194));
#28160=CARTESIAN_POINT('Ctrl Pts',(-31.6389683688547,-54.8619507900759,
16.6694473265048));
#28161=CARTESIAN_POINT('Ctrl Pts',(-31.6652521719754,-54.8469263020217,
16.6714803633902));
#28162=CARTESIAN_POINT('Origin',(-32.5,-56.2916512459885,17.));
#28163=CARTESIAN_POINT('',(-31.6668674827448,-54.8509763286063,17.3714803633902));
#28164=CARTESIAN_POINT('',(-31.6688688935778,-54.8504049148725,17.1785196366098));
#28165=CARTESIAN_POINT('',(-31.667,-54.8488529232836,17.));
#28166=CARTESIAN_POINT('Ctrl Pts',(-31.6688688935778,-54.8504049148725,
17.1785196366098));
#28167=CARTESIAN_POINT('Ctrl Pts',(-31.3819874737692,-55.0177923404707,
17.156380408079));
#28168=CARTESIAN_POINT('Ctrl Pts',(-31.1417740021657,-55.2676351144426,
17.1342411795483));
#28169=CARTESIAN_POINT('Ctrl Pts',(-30.9981174968785,-55.5642433945469,
17.1121019510175));
#28170=CARTESIAN_POINT('Ctrl Pts',(-30.7577345202416,-56.0605632870855,
17.0750559874949));
#28171=CARTESIAN_POINT('Ctrl Pts',(-30.7877102970592,-56.6878262324662,
17.0380100239722));
#28172=CARTESIAN_POINT('Ctrl Pts',(-31.0743262430964,-57.1589617869126,
17.0009640604495));
#28173=CARTESIAN_POINT('Ctrl Pts',(-31.3609421891337,-57.630097341359,16.9639180969268));
#28174=CARTESIAN_POINT('Ctrl Pts',(-31.9041983043906,-57.9451055048711,
16.9268721334041));
#28175=CARTESIAN_POINT('Ctrl Pts',(-32.4554703472483,-57.9598210051999,
16.8898261698815));
#28176=CARTESIAN_POINT('Ctrl Pts',(-33.006742390106,-57.9745365055287,16.8527802063588));
#28177=CARTESIAN_POINT('Ctrl Pts',(-33.5660303605644,-57.6889593426742,
16.8157342428361));
#28178=CARTESIAN_POINT('Ctrl Pts',(-33.8773729475645,-57.2337855245493,
16.7786882793134));
#28179=CARTESIAN_POINT('Ctrl Pts',(-34.1887155345647,-56.7786117064244,
16.7416423157907));
#28180=CARTESIAN_POINT('Ctrl Pts',(-34.2521127381066,-56.1538412330292,
16.704596352268));
#28181=CARTESIAN_POINT('Ctrl Pts',(-34.0385504685031,-55.6454038542025,
16.6675503887454));
#28182=CARTESIAN_POINT('Ctrl Pts',(-33.8249881988997,-55.1369664753759,
16.6305044252227));
#28183=CARTESIAN_POINT('Ctrl Pts',(-33.3344664561509,-54.7448621911179,
16.5934584617));
#28184=CARTESIAN_POINT('Ctrl Pts',(-32.7914752972722,-54.6485397505015,
16.5564124981773));
#28185=CARTESIAN_POINT('Ctrl Pts',(-32.4109108025283,-54.5810305464448,
16.5304482109881));
#28186=CARTESIAN_POINT('Ctrl Pts',(-32.0045725792269,-54.658813619538,16.504483923799));
#28187=CARTESIAN_POINT('Ctrl Pts',(-31.6662812667712,-54.8504621893828,
16.4785196366098));
#28188=CARTESIAN_POINT('Ctrl Pts',(-31.6652521719754,-54.8469263020217,
16.6714803633902));
#28189=CARTESIAN_POINT('Ctrl Pts',(-32.1179113819592,-54.5881748244737,
16.7064932900275));
#28190=CARTESIAN_POINT('Ctrl Pts',(-32.7032079137753,-54.5552369344614,
16.7415062166648));
#28191=CARTESIAN_POINT('Ctrl Pts',(-33.1792781595522,-54.7673956583618,
16.776519143302));
#28192=CARTESIAN_POINT('Ctrl Pts',(-33.6829915777989,-54.9918734470383,
16.8135651068247));
#28193=CARTESIAN_POINT('Ctrl Pts',(-34.0644259255566,-55.4907374408677,
16.8506110703474));
#28194=CARTESIAN_POINT('Ctrl Pts',(-34.1490156106942,-56.0356797043225,
16.8876570338701));
#28195=CARTESIAN_POINT('Ctrl Pts',(-34.2336052958317,-56.5806219677773,
16.9247029973928));
#28196=CARTESIAN_POINT('Ctrl Pts',(-34.0213503183491,-57.1716425008576,
16.9617489609154));
#28197=CARTESIAN_POINT('Ctrl Pts',(-33.6093903722588,-57.5382574052848,
16.9987949244381));
#28198=CARTESIAN_POINT('Ctrl Pts',(-33.1974304261685,-57.904872309712,17.0358408879608));
#28199=CARTESIAN_POINT('Ctrl Pts',(-32.5857655114706,-58.0470815854862,
17.0728868514835));
#28200=CARTESIAN_POINT('Ctrl Pts',(-32.0543275447525,-57.8998023511678,
17.1099328150062));
#28201=CARTESIAN_POINT('Ctrl Pts',(-31.5228895780343,-57.7525231168495,
17.1469787785289));
#28202=CARTESIAN_POINT('Ctrl Pts',(-31.071678559296,-57.3157553724386,17.1840247420515));
#28203=CARTESIAN_POINT('Ctrl Pts',(-30.9071937698036,-56.7893883528063,
17.2210707055742));
#28204=CARTESIAN_POINT('Ctrl Pts',(-30.7427089803112,-56.2630213331741,
17.2581166690969));
#28205=CARTESIAN_POINT('Ctrl Pts',(-30.8649504200647,-55.6470550383205,
17.2951626326196));
#28206=CARTESIAN_POINT('Ctrl Pts',(-31.2179736010048,-55.2233899358517,
17.3322085961423));
#28207=CARTESIAN_POINT('Ctrl Pts',(-31.3427181334424,-55.073683321751,17.3452991852249));
#28208=CARTESIAN_POINT('Ctrl Pts',(-31.4962789539492,-54.9479881676876,
17.3583897743076));
#28209=CARTESIAN_POINT('Ctrl Pts',(-31.6668674827448,-54.8509763286063,
17.3714803633902));
#28210=CARTESIAN_POINT('Origin',(-32.5,-56.2916512459885,17.));
#28211=CARTESIAN_POINT('',(-31.6688993943412,-54.8497298728322,18.0714803633902));
#28212=CARTESIAN_POINT('',(-31.6668239490615,-54.8465985185331,17.8785196366098));
#28213=CARTESIAN_POINT('',(-31.667,-54.8488529232836,17.));
#28214=CARTESIAN_POINT('Ctrl Pts',(-31.6668239490615,-54.8465985185331,
17.8785196366098));
#28215=CARTESIAN_POINT('Ctrl Pts',(-31.2400871420202,-55.0969461017405,
17.8453228558818));
#28216=CARTESIAN_POINT('Ctrl Pts',(-30.9262488413014,-55.5484932725245,
17.8121260751538));
#28217=CARTESIAN_POINT('Ctrl Pts',(-30.8508004340577,-56.036868932597,17.7789292944258));
#28218=CARTESIAN_POINT('Ctrl Pts',(-30.7666037474724,-56.5818719868586,
17.7418833309031));
#28219=CARTESIAN_POINT('Ctrl Pts',(-30.9792848378898,-57.1727392338966,
17.7048373673804));
#28220=CARTESIAN_POINT('Ctrl Pts',(-31.3915089982965,-57.539056927659,17.6677914038577));
#28221=CARTESIAN_POINT('Ctrl Pts',(-31.8037331587031,-57.9053746214214,
17.6307454403351));
#28222=CARTESIAN_POINT('Ctrl Pts',(-32.4155003890991,-58.0471427619081,
17.5936994768124));
#28223=CARTESIAN_POINT('Ctrl Pts',(-32.9468319475375,-57.8994803557453,
17.5566535132897));
#28224=CARTESIAN_POINT('Ctrl Pts',(-33.4781635059759,-57.7518179495826,
17.519607549767));
#28225=CARTESIAN_POINT('Ctrl Pts',(-33.9290593924568,-57.3147249967705,
17.4825615862443));
#28226=CARTESIAN_POINT('Ctrl Pts',(-34.0931645477786,-56.788239565649,17.4455156227217));
#28227=CARTESIAN_POINT('Ctrl Pts',(-34.2572697031003,-56.2617541345275,
17.408469659199));
#28228=CARTESIAN_POINT('Ctrl Pts',(-34.134584127263,-55.6458762250967,17.3714236956763));
#28229=CARTESIAN_POINT('Ctrl Pts',(-33.7812555697231,-55.2224658548728,
17.3343777321536));
#28230=CARTESIAN_POINT('Ctrl Pts',(-33.4279270121832,-54.7990554846489,
17.2973317686309));
#28231=CARTESIAN_POINT('Ctrl Pts',(-32.8439554729406,-54.568112653632,17.2602858051083));
#28232=CARTESIAN_POINT('Ctrl Pts',(-32.2965988382737,-54.6353296579719,
17.2232398415856));
#28233=CARTESIAN_POINT('Ctrl Pts',(-32.0763508133016,-54.6623767631182,
17.2083331065936));
#28234=CARTESIAN_POINT('Ctrl Pts',(-31.8620312385645,-54.7376999942423,
17.1934263716017));
#28235=CARTESIAN_POINT('Ctrl Pts',(-31.6688688935778,-54.8504049148725,
17.1785196366098));
#28236=CARTESIAN_POINT('Ctrl Pts',(-31.6668674827448,-54.8509763286063,
17.3714803633902));
#28237=CARTESIAN_POINT('Ctrl Pts',(-31.9790392312177,-54.6734476539504,
17.3954357378302));
#28238=CARTESIAN_POINT('Ctrl Pts',(-32.3482331506335,-54.5919732963168,
17.4193911122703));
#28239=CARTESIAN_POINT('Ctrl Pts',(-32.7022067343745,-54.6351832109726,
17.4433464867103));
#28240=CARTESIAN_POINT('Ctrl Pts',(-33.2496117646775,-54.702005498646,17.480392450233));
#28241=CARTESIAN_POINT('Ctrl Pts',(-33.7606169031567,-55.0670139840768,
17.5174384137557));
#28242=CARTESIAN_POINT('Ctrl Pts',(-34.001357750591,-55.5631604641687,17.5544843772783));
#28243=CARTESIAN_POINT('Ctrl Pts',(-34.2420985980252,-56.0593069442606,
17.591530340801));
#28244=CARTESIAN_POINT('Ctrl Pts',(-34.2125751544145,-56.6865914190135,
17.6285763043237));
#28245=CARTESIAN_POINT('Ctrl Pts',(-33.9262989911366,-57.1579335916119,
17.6656222678464));
#28246=CARTESIAN_POINT('Ctrl Pts',(-33.6400228278587,-57.6292757642103,
17.7026682313691));
#28247=CARTESIAN_POINT('Ctrl Pts',(-33.0969939449135,-57.9446756346541,
17.7397141948917));
#28248=CARTESIAN_POINT('Ctrl Pts',(-32.5457325897642,-57.959788663796,17.7767601584144));
#28249=CARTESIAN_POINT('Ctrl Pts',(-31.9944712346149,-57.9749016929378,
17.8138061219371));
#28250=CARTESIAN_POINT('Ctrl Pts',(-31.4349774072614,-57.6897278807776,
17.8508520854598));
#28251=CARTESIAN_POINT('Ctrl Pts',(-31.1233066303378,-57.2347786394959,
17.8878980489825));
#28252=CARTESIAN_POINT('Ctrl Pts',(-30.8116358534142,-56.7798293982142,
17.9249440125051));
#28253=CARTESIAN_POINT('Ctrl Pts',(-30.7477881269207,-56.1551047278111,
17.9619899760278));
#28254=CARTESIAN_POINT('Ctrl Pts',(-30.960983724928,-55.6465134161264,17.9990359395505));
#28255=CARTESIAN_POINT('Ctrl Pts',(-31.0999537214239,-55.3149918769235,
18.0231840808304));
#28256=CARTESIAN_POINT('Ctrl Pts',(-31.3566391271215,-55.0328152763439,
18.0473322221103));
#28257=CARTESIAN_POINT('Ctrl Pts',(-31.6688993943412,-54.8497298728322,
18.0714803633902));
#28258=CARTESIAN_POINT('Origin',(-32.5,-56.2916512459885,17.));
#28259=CARTESIAN_POINT('',(-31.6661431441559,-54.8463676572785,18.7714803633902));
#28260=CARTESIAN_POINT('',(-31.6653993953823,-54.8489980951737,18.5785196366098));
#28261=CARTESIAN_POINT('',(-31.667,-54.8488529232836,17.));
#28262=CARTESIAN_POINT('Ctrl Pts',(-31.6653993953823,-54.8489980951737,
18.5785196366098));
#28263=CARTESIAN_POINT('Ctrl Pts',(-31.5716723835923,-54.901972129835,18.5713112672072));
#28264=CARTESIAN_POINT('Ctrl Pts',(-31.4833584827506,-54.9639737793168,
18.5641028978046));
#28265=CARTESIAN_POINT('Ctrl Pts',(-31.4025244101713,-55.0345432294477,
18.5568945284021));
#28266=CARTESIAN_POINT('Ctrl Pts',(-30.987093965791,-55.3972207129895,18.5198485648794));
#28267=CARTESIAN_POINT('Ctrl Pts',(-30.7692236712863,-55.9861942986586,
18.4828026013567));
#28268=CARTESIAN_POINT('Ctrl Pts',(-30.8486231023463,-56.5319168852662,
18.445756637834));
#28269=CARTESIAN_POINT('Ctrl Pts',(-30.9280225334064,-57.0776394718738,
18.4087106743114));
#28270=CARTESIAN_POINT('Ctrl Pts',(-31.3046916900312,-57.5801110594199,
18.3716647107887));
#28271=CARTESIAN_POINT('Ctrl Pts',(-31.8062457968319,-57.8093726766562,
18.334618747266));
#28272=CARTESIAN_POINT('Ctrl Pts',(-32.3077999036325,-58.0386342938926,
18.2975727837433));
#28273=CARTESIAN_POINT('Ctrl Pts',(-32.9342389606089,-57.9946859408192,
18.2605268202206));
#28274=CARTESIAN_POINT('Ctrl Pts',(-33.3988695811849,-57.6976408304243,
18.223480856698));
#28275=CARTESIAN_POINT('Ctrl Pts',(-33.8635002017609,-57.4005957200295,
18.1864348931753));
#28276=CARTESIAN_POINT('Ctrl Pts',(-34.1663223859365,-56.850453852313,18.1493889296526));
#28277=CARTESIAN_POINT('Ctrl Pts',(-34.1687478440051,-56.298990772552,18.1123429661299));
#28278=CARTESIAN_POINT('Ctrl Pts',(-34.1711733020737,-55.747527692791,18.0752970026072));
#28279=CARTESIAN_POINT('Ctrl Pts',(-33.8732020340353,-55.1947434009853,
18.0382510390845));
#28280=CARTESIAN_POINT('Ctrl Pts',(-33.4112022803197,-54.8936227627801,
18.0012050755619));
#28281=CARTESIAN_POINT('Ctrl Pts',(-32.9492025266041,-54.5925021245749,
17.9641591120392));
#28282=CARTESIAN_POINT('Ctrl Pts',(-32.3231742872114,-54.5430451399701,
17.9271131485165));
#28283=CARTESIAN_POINT('Ctrl Pts',(-31.8196229357211,-54.7678860784103,
17.8900671849938));
#28284=CARTESIAN_POINT('Ctrl Pts',(-31.7673024933817,-54.791247702444,17.8862180021991));
#28285=CARTESIAN_POINT('Ctrl Pts',(-31.7163042884046,-54.8175705950767,
17.8823688194045));
#28286=CARTESIAN_POINT('Ctrl Pts',(-31.6668239490615,-54.8465985185331,
17.8785196366098));
#28287=CARTESIAN_POINT('Ctrl Pts',(-31.6688993943412,-54.8497298728322,
18.0714803633902));
#28288=CARTESIAN_POINT('Ctrl Pts',(-31.8356814821797,-54.751941684401,18.084378185633));
#28289=CARTESIAN_POINT('Ctrl Pts',(-32.0183177486645,-54.6824218442403,
18.0972760078758));
#28290=CARTESIAN_POINT('Ctrl Pts',(-32.2073398697232,-54.6487501647903,
18.1101738301185));
#28291=CARTESIAN_POINT('Ctrl Pts',(-32.7502614940028,-54.5520361781053,
18.1472197936412));
#28292=CARTESIAN_POINT('Ctrl Pts',(-33.3458658200538,-54.7510661577016,
18.1842657571639));
#28293=CARTESIAN_POINT('Ctrl Pts',(-33.7215711507525,-55.1547529048404,
18.2213117206866));
#28294=CARTESIAN_POINT('Ctrl Pts',(-34.0972764814512,-55.5584396519791,
18.2583576842093));
#28295=CARTESIAN_POINT('Ctrl Pts',(-34.2530828167976,-56.1667831666603,
18.2954036477319));
#28296=CARTESIAN_POINT('Ctrl Pts',(-34.1176845039388,-56.7013715898475,
18.3324496112546));
#28297=CARTESIAN_POINT('Ctrl Pts',(-33.98228619108,-57.2359600130347,18.3694955747773));
#28298=CARTESIAN_POINT('Ctrl Pts',(-33.5556832300161,-57.696793344728,18.4065415383));
#28299=CARTESIAN_POINT('Ctrl Pts',(-33.0331128848803,-57.8729685975756,
18.4435875018227));
#28300=CARTESIAN_POINT('Ctrl Pts',(-32.5105425397446,-58.0491438504232,
18.4806334653454));
#28301=CARTESIAN_POINT('Ctrl Pts',(-31.892004810537,-57.9406610244251,18.517679428868));
#28302=CARTESIAN_POINT('Ctrl Pts',(-31.4605769963787,-57.5971679000379,
18.5547253923907));
#28303=CARTESIAN_POINT('Ctrl Pts',(-31.0291491822204,-57.2536747756508,
18.5917713559134));
#28304=CARTESIAN_POINT('Ctrl Pts',(-30.7848312831114,-56.6751713528747,
18.6288173194361));
#28305=CARTESIAN_POINT('Ctrl Pts',(-30.839436770952,-56.1264130034822,18.6658632829588));
#28306=CARTESIAN_POINT('Ctrl Pts',(-30.89132971378,-55.6049143999997,18.7010689764359));
#28307=CARTESIAN_POINT('Ctrl Pts',(-31.2131854490112,-55.1102790779514,
18.7362746699131));
#28308=CARTESIAN_POINT('Ctrl Pts',(-31.6661431441559,-54.8463676572785,
18.7714803633902));
#28309=CARTESIAN_POINT('Origin',(-32.5,-56.2916512459885,17.));
#28310=CARTESIAN_POINT('',(-31.6657991298123,-54.8498167632728,19.4714803633902));
#28311=CARTESIAN_POINT('',(-31.6682947036337,-54.8512220664372,19.2785196366098));
#28312=CARTESIAN_POINT('',(-31.667,-54.8488529232836,17.));
#28313=CARTESIAN_POINT('Ctrl Pts',(-31.6682947036337,-54.8512220664372,
19.2785196366098));
#28314=CARTESIAN_POINT('Ctrl Pts',(-31.4307799124075,-54.9882439463791,
19.26025371501));
#28315=CARTESIAN_POINT('Ctrl Pts',(-31.2253675580441,-55.1807871169989,
19.2419877934101));
#28316=CARTESIAN_POINT('Ctrl Pts',(-31.0820105037967,-55.4118336375308,
19.2237218718103));
#28317=CARTESIAN_POINT('Ctrl Pts',(-30.7912614072705,-55.8804298112795,
19.1866759082876));
#28318=CARTESIAN_POINT('Ctrl Pts',(-30.7557692111823,-56.5074048138577,
19.149629944765));
#28319=CARTESIAN_POINT('Ctrl Pts',(-30.9917771203569,-57.0058199801505,
19.1125839812423));
#28320=CARTESIAN_POINT('Ctrl Pts',(-31.2277850295315,-57.5042351464432,
19.0755380177196));
#28321=CARTESIAN_POINT('Ctrl Pts',(-31.735293043969,-57.8740904764506,19.0384920541969));
#28322=CARTESIAN_POINT('Ctrl Pts',(-32.2820372430805,-57.9461195811699,
19.0014460906742));
#28323=CARTESIAN_POINT('Ctrl Pts',(-32.828781442192,-58.0181486858891,18.9644001271516));
#28324=CARTESIAN_POINT('Ctrl Pts',(-33.4147618259776,-57.7923515653202,
18.9273541636289));
#28325=CARTESIAN_POINT('Ctrl Pts',(-33.7718011490707,-57.3720655520494,
18.8903082001062));
#28326=CARTESIAN_POINT('Ctrl Pts',(-34.1288404721637,-56.9517795387787,
18.8532622365835));
#28327=CARTESIAN_POINT('Ctrl Pts',(-34.2569387345642,-56.3370046328062,
18.8162162730608));
#28328=CARTESIAN_POINT('Ctrl Pts',(-34.0974710401143,-55.8090960558605,
18.7791703095382));
#28329=CARTESIAN_POINT('Ctrl Pts',(-33.9380033456643,-55.2811874789147,
18.7421243460155));
#28330=CARTESIAN_POINT('Ctrl Pts',(-33.4909696943638,-54.8401452309956,
18.7050783824928));
#28331=CARTESIAN_POINT('Ctrl Pts',(-32.9609575715857,-54.6878147977434,
18.6680324189701));
#28332=CARTESIAN_POINT('Ctrl Pts',(-32.5340747186532,-54.565124679649,18.63819482485));
#28333=CARTESIAN_POINT('Ctrl Pts',(-32.0533634937382,-54.6297227421977,
18.6083572307299));
#28334=CARTESIAN_POINT('Ctrl Pts',(-31.6653993953823,-54.8489980951737,
18.5785196366098));
#28335=CARTESIAN_POINT('Ctrl Pts',(-31.6661431441559,-54.8463676572785,
18.7714803633902));
#28336=CARTESIAN_POINT('Ctrl Pts',(-31.6898201235287,-54.832572494219,18.7733206334357));
#28337=CARTESIAN_POINT('Ctrl Pts',(-31.7138553201483,-54.819407751031,18.7751609034813));
#28338=CARTESIAN_POINT('Ctrl Pts',(-31.7382289011374,-54.8069025442232,
18.7770011735268));
#28339=CARTESIAN_POINT('Ctrl Pts',(-32.2288866686916,-54.5551637103656,
18.8140471370495));
#28340=CARTESIAN_POINT('Ctrl Pts',(-32.8566733290096,-54.5706993186593,
18.8510931005722));
#28341=CARTESIAN_POINT('Ctrl Pts',(-33.3342787571905,-54.8463994098822,
18.8881390640948));
#28342=CARTESIAN_POINT('Ctrl Pts',(-33.8118841853713,-55.1220995011052,
18.9251850276175));
#28343=CARTESIAN_POINT('Ctrl Pts',(-34.1393083814151,-55.6579640752576,
18.9622309911402));
#28344=CARTESIAN_POINT('Ctrl Pts',(-34.1667038054087,-56.2087516714065,
18.9992769546629));
#28345=CARTESIAN_POINT('Ctrl Pts',(-34.1940992294022,-56.7595392675554,
19.0363229181855));
#28346=CARTESIAN_POINT('Ctrl Pts',(-33.9214658813456,-57.3252498857009,
19.0733688817082));
#28347=CARTESIAN_POINT('Ctrl Pts',(-33.4735759588574,-57.6469828536776,
19.1104148452309));
#28348=CARTESIAN_POINT('Ctrl Pts',(-33.0256860363693,-57.9687158216544,
19.1474608087536));
#28349=CARTESIAN_POINT('Ctrl Pts',(-32.4025395394495,-58.0464711394622,
19.1845067722763));
#28350=CARTESIAN_POINT('Ctrl Pts',(-31.889322996006,-57.8446636449513,19.221552735799));
#28351=CARTESIAN_POINT('Ctrl Pts',(-31.3761064525625,-57.6428561504404,
19.2585986993216));
#28352=CARTESIAN_POINT('Ctrl Pts',(-30.9728198625952,-57.1614858436107,
19.2956446628443));
#28353=CARTESIAN_POINT('Ctrl Pts',(-30.86402962057,-56.6208545750433,19.332690626367));
#28354=CARTESIAN_POINT('Ctrl Pts',(-30.7552393785448,-56.0802233064759,
19.3697365898897));
#28355=CARTESIAN_POINT('Ctrl Pts',(-30.9409454844617,-55.4803310761708,
19.4067825534124));
#28356=CARTESIAN_POINT('Ctrl Pts',(-31.3361584863693,-55.0957219647369,
19.443828516935));
#28357=CARTESIAN_POINT('Ctrl Pts',(-31.4344901101744,-55.000028659418,19.4530457990868));
#28358=CARTESIAN_POINT('Ctrl Pts',(-31.5457912060088,-54.917662401762,19.4622630812385));
#28359=CARTESIAN_POINT('Ctrl Pts',(-31.6657991298123,-54.8498167632728,
19.4714803633902));
#28360=CARTESIAN_POINT('Origin',(-32.5,-56.2916512459885,17.));
#28361=CARTESIAN_POINT('',(-31.6686691446489,-54.8508917236136,20.1714803633902));
#28362=CARTESIAN_POINT('',(-31.6680707239276,-54.8477242132621,19.9785196366098));
#28363=CARTESIAN_POINT('',(-31.667,-54.8488529232836,17.));
#28364=CARTESIAN_POINT('Ctrl Pts',(-31.6680707239276,-54.8477242132621,
19.9785196366098));
#28365=CARTESIAN_POINT('Ctrl Pts',(-31.2906837721071,-55.0702773030723,
19.9491961628127));
#28366=CARTESIAN_POINT('Ctrl Pts',(-30.9974844080692,-55.4444429123815,
19.9198726890156));
#28367=CARTESIAN_POINT('Ctrl Pts',(-30.8862884172365,-55.8665534203839,
19.8905492152186));
#28368=CARTESIAN_POINT('Ctrl Pts',(-30.7458083824097,-56.3998289316761,
19.8535032516959));
#28369=CARTESIAN_POINT('Ctrl Pts',(-30.8958178157836,-57.0096276847031,
19.8164572881732));
#28370=CARTESIAN_POINT('Ctrl Pts',(-31.2676640515259,-57.4168718226721,
19.7794113246505));
#28371=CARTESIAN_POINT('Ctrl Pts',(-31.6395102872682,-57.8241159606411,
19.7423653611279));
#28372=CARTESIAN_POINT('Ctrl Pts',(-32.2331933253789,-58.0288054835522,
19.7053193976052));
#28373=CARTESIAN_POINT('Ctrl Pts',(-32.7770107560741,-57.9372630704145,
19.6682734340825));
#28374=CARTESIAN_POINT('Ctrl Pts',(-33.3208281867694,-57.8457206572769,
19.6312274705598));
#28375=CARTESIAN_POINT('Ctrl Pts',(-33.8147800100492,-57.4579463080904,
19.5941815070371));
#28376=CARTESIAN_POINT('Ctrl Pts',(-34.0328063735823,-56.9514071526715,
19.5571355435145));
#28377=CARTESIAN_POINT('Ctrl Pts',(-34.2508327371153,-56.4448679972525,
19.5200895799918));
#28378=CARTESIAN_POINT('Ctrl Pts',(-34.1929336409016,-55.8195640356011,
19.4830436164691));
#28379=CARTESIAN_POINT('Ctrl Pts',(-33.8856069343887,-55.3616691714411,
19.4459976529464));
#28380=CARTESIAN_POINT('Ctrl Pts',(-33.5782802278758,-54.9037743072811,
19.4089516894237));
#28381=CARTESIAN_POINT('Ctrl Pts',(-33.0215259110637,-54.6132885406125,
19.3719057259011));
#28382=CARTESIAN_POINT('Ctrl Pts',(-32.4701457541755,-54.6231543297377,
19.3348597623784));
#28383=CARTESIAN_POINT('Ctrl Pts',(-32.1906296753062,-54.6281556825373,
19.3160797204555));
#28384=CARTESIAN_POINT('Ctrl Pts',(-31.9124946862162,-54.7103435109481,
19.2972996785326));
#28385=CARTESIAN_POINT('Ctrl Pts',(-31.6682947036337,-54.8512220664372,
19.2785196366098));
#28386=CARTESIAN_POINT('Ctrl Pts',(-31.6657991298123,-54.8498167632728,
19.4714803633902));
#28387=CARTESIAN_POINT('Ctrl Pts',(-32.0281252709183,-54.6449782192373,
19.4993090447612));
#28388=CARTESIAN_POINT('Ctrl Pts',(-32.4698183191301,-54.5725020736119,
19.5271377261321));
#28389=CARTESIAN_POINT('Ctrl Pts',(-32.8735646889017,-54.6652369881101,
19.5549664075031));
#28390=CARTESIAN_POINT('Ctrl Pts',(-33.4110379916282,-54.7886871154801,
19.5920123710258));
#28391=CARTESIAN_POINT('Ctrl Pts',(-33.8812646991831,-55.2049133627827,
19.6290583345484));
#28392=CARTESIAN_POINT('Ctrl Pts',(-34.069042894277,-55.7234274269329,19.6661042980711));
#28393=CARTESIAN_POINT('Ctrl Pts',(-34.2568210893709,-56.2419414910831,
19.7031502615938));
#28394=CARTESIAN_POINT('Ctrl Pts',(-34.1621507720038,-56.8627433720808,
19.7401962251165));
#28395=CARTESIAN_POINT('Ctrl Pts',(-33.8283583461529,-57.3017195705904,
19.7772421886392));
#28396=CARTESIAN_POINT('Ctrl Pts',(-33.494565920302,-57.7406957690999,19.8142881521619));
#28397=CARTESIAN_POINT('Ctrl Pts',(-32.9216513859674,-57.9978462851214,
19.8513341156845));
#28398=CARTESIAN_POINT('Ctrl Pts',(-32.3718123356058,-57.9554847234739,
19.8883800792072));
#28399=CARTESIAN_POINT('Ctrl Pts',(-31.8219732852443,-57.9131231618264,
19.9254260427299));
#28400=CARTESIAN_POINT('Ctrl Pts',(-31.2952097188559,-57.5712495225101,
19.9624720062526));
#28401=CARTESIAN_POINT('Ctrl Pts',(-31.0325979551939,-57.086324221881,19.9995179697753));
#28402=CARTESIAN_POINT('Ctrl Pts',(-30.769986191532,-56.601398921252,20.0365639332979));
#28403=CARTESIAN_POINT('Ctrl Pts',(-30.7715262305966,-55.9734219593102,
20.0736098968206));
#28404=CARTESIAN_POINT('Ctrl Pts',(-31.0365132935154,-55.489790540013,20.1106558603433));
#28405=CARTESIAN_POINT('Ctrl Pts',(-31.1815376981853,-55.225104566703,20.1309306946923));
#28406=CARTESIAN_POINT('Ctrl Pts',(-31.4054710295806,-55.0036536684416,
20.1512055290412));
#28407=CARTESIAN_POINT('Ctrl Pts',(-31.6686691446489,-54.8508917236136,
20.1714803633902));
#28408=CARTESIAN_POINT('Origin',(-32.5,-56.2916512459885,17.));
#28409=CARTESIAN_POINT('',(-31.6674621971265,-54.8470528177236,20.8714803633902));
#28410=CARTESIAN_POINT('',(-31.6651488727497,-54.8473747039335,20.6785196366098));
#28411=CARTESIAN_POINT('',(-31.667,-54.8488529232836,17.));
#28412=CARTESIAN_POINT('Ctrl Pts',(-31.6651488727497,-54.8473747039335,
20.6785196366098));
#28413=CARTESIAN_POINT('Ctrl Pts',(-31.6219590933013,-54.8719481703147,
20.6751845741381));
#28414=CARTESIAN_POINT('Ctrl Pts',(-31.579962486587,-54.8985363635017,20.6718495116665));
#28415=CARTESIAN_POINT('Ctrl Pts',(-31.539367364925,-54.9271153018696,20.6685144491949));
#28416=CARTESIAN_POINT('Ctrl Pts',(-31.0884356630213,-55.2445709169594,
20.6314684856722));
#28417=CARTESIAN_POINT('Ctrl Pts',(-30.8104307642169,-55.8076611175675,
20.5944225221495));
#28418=CARTESIAN_POINT('Ctrl Pts',(-30.8325829345476,-56.3586844387663,
20.5573765586268));
#28419=CARTESIAN_POINT('Ctrl Pts',(-30.8547351048784,-56.9097077599651,
20.5203305951041));
#28420=CARTESIAN_POINT('Ctrl Pts',(-31.1770443443443,-57.4486642017546,
20.4832846315815));
#28421=CARTESIAN_POINT('Ctrl Pts',(-31.6520041279564,-57.7288973132864,
20.4462386680588));
#28422=CARTESIAN_POINT('Ctrl Pts',(-32.1269639115685,-58.0091304248183,
20.4091927045361));
#28423=CARTESIAN_POINT('Ctrl Pts',(-32.7545742393267,-58.0306402060925,
20.3721467410134));
#28424=CARTESIAN_POINT('Ctrl Pts',(-33.2476056229439,-57.7835825733328,
20.3351007774907));
#28425=CARTESIAN_POINT('Ctrl Pts',(-33.7406370065611,-57.5365249405731,
20.2980548139681));
#28426=CARTESIAN_POINT('Ctrl Pts',(-34.0990894460373,-57.0208998937796,
20.2610088504454));
#28427=CARTESIAN_POINT('Ctrl Pts',(-34.1589151813611,-56.4726861646106,
20.2239628869227));
#28428=CARTESIAN_POINT('Ctrl Pts',(-34.2187409166848,-55.9244724354416,
20.1869169234));
#28429=CARTESIAN_POINT('Ctrl Pts',(-33.9799399478562,-55.3436700238972,
20.1498709598773));
#28430=CARTESIAN_POINT('Ctrl Pts',(-33.5518008766237,-54.9960864443956,
20.1128249963547));
#28431=CARTESIAN_POINT('Ctrl Pts',(-33.1236618053912,-54.648502864894,20.075779032832));
#28432=CARTESIAN_POINT('Ctrl Pts',(-32.5061846317548,-54.5341381174352,
20.0387330693093));
#28433=CARTESIAN_POINT('Ctrl Pts',(-31.9819612934229,-54.7053318784846,
20.0016871057866));
#28434=CARTESIAN_POINT('Ctrl Pts',(-31.8726832787826,-54.7410184131319,
19.993964616061));
#28435=CARTESIAN_POINT('Ctrl Pts',(-31.7674575454953,-54.7891136966038,
19.9862421263354));
#28436=CARTESIAN_POINT('Ctrl Pts',(-31.6680707239276,-54.8477242132621,
19.9785196366098));
#28437=CARTESIAN_POINT('Ctrl Pts',(-31.6686691446489,-54.8508917236136,
20.1714803633902));
#28438=CARTESIAN_POINT('Ctrl Pts',(-31.8863838499881,-54.724528653739,20.1882514925639));
#28439=CARTESIAN_POINT('Ctrl Pts',(-32.1309651849206,-54.6451654778256,
20.2050226217376));
#28440=CARTESIAN_POINT('Ctrl Pts',(-32.3799746400723,-54.6272090425041,
20.2217937509113));
#28441=CARTESIAN_POINT('Ctrl Pts',(-32.9300148369371,-54.5875448409449,
20.258839714434));
#28442=CARTESIAN_POINT('Ctrl Pts',(-33.5016611438935,-54.8475023144793,
20.2958856779567));
#28443=CARTESIAN_POINT('Ctrl Pts',(-33.8332965022582,-55.2881103970044,
20.3329316414794));
#28444=CARTESIAN_POINT('Ctrl Pts',(-34.1649318606228,-55.7287184795295,
20.3699776050021));
#28445=CARTESIAN_POINT('Ctrl Pts',(-34.2565562703957,-56.3499771710453,
20.4070235685247));
#28446=CARTESIAN_POINT('Ctrl Pts',(-34.0662370704008,-56.8675640172575,
20.4440695320474));
#28447=CARTESIAN_POINT('Ctrl Pts',(-33.875917870406,-57.3851508634698,20.4811154955701));
#28448=CARTESIAN_POINT('Ctrl Pts',(-33.4036550606434,-57.7990658643784,
20.5181614590928));
#28449=CARTESIAN_POINT('Ctrl Pts',(-32.8655828553033,-57.9198782552652,
20.5552074226155));
#28450=CARTESIAN_POINT('Ctrl Pts',(-32.3275106499632,-58.0406906461521,
20.5922533861382));
#28451=CARTESIAN_POINT('Ctrl Pts',(-31.7236290490455,-57.8684004270172,
20.6292993496608));
#28452=CARTESIAN_POINT('Ctrl Pts',(-31.3303069678814,-57.4818576289614,
20.6663453131835));
#28453=CARTESIAN_POINT('Ctrl Pts',(-30.9369848867174,-57.0953148309056,
20.7033912767062));
#28454=CARTESIAN_POINT('Ctrl Pts',(-30.754222325307,-56.494519453929,20.7404372402289));
#28455=CARTESIAN_POINT('Ctrl Pts',(-30.8656634549365,-55.954428037577,20.7774832037516));
#28456=CARTESIAN_POINT('Ctrl Pts',(-30.959917085256,-55.4976345999579,20.8088155902978));
#28457=CARTESIAN_POINT('Ctrl Pts',(-31.2646228230038,-55.0842643987964,
20.840147976844));
#28458=CARTESIAN_POINT('Ctrl Pts',(-31.6674621971265,-54.8470528177236,
20.8714803633902));
#28459=CARTESIAN_POINT('Origin',(-32.5,-56.2916512459885,17.));
#28460=CARTESIAN_POINT('',(-31.6652082225275,-54.8481806306043,21.5714803633902));
#28461=CARTESIAN_POINT('',(-31.667262219952,-54.851191363199,21.3785196366098));
#28462=CARTESIAN_POINT('',(-31.667,-54.8488529232836,17.));
#28463=CARTESIAN_POINT('',(-32.1997834265916,-57.9303781936679,22.));
#28464=CARTESIAN_POINT('Ctrl Pts',(-31.6652082225275,-54.8481806306043,
21.5714803633902));
#28465=CARTESIAN_POINT('Ctrl Pts',(-32.0766081468896,-54.6152030336121,
21.6031823516921));
#28466=CARTESIAN_POINT('Ctrl Pts',(-32.5941722167266,-54.5601311343425,
21.634884339994));
#28467=CARTESIAN_POINT('Ctrl Pts',(-33.0407304570642,-54.7130293475825,
21.6665863282959));
#28468=CARTESIAN_POINT('Ctrl Pts',(-33.5625646122208,-54.8917014730163,
21.7036322918186));
#28469=CARTESIAN_POINT('Ctrl Pts',(-33.987436493413,-55.3543679573327,21.7406782553412));
#28470=CARTESIAN_POINT('Ctrl Pts',(-34.1199308616871,-55.8897554009177,
21.7777242188639));
#28471=CARTESIAN_POINT('Ctrl Pts',(-34.2524252299611,-56.4251428445027,
21.8147701823866));
#28472=CARTESIAN_POINT('Ctrl Pts',(-34.0925420853171,-57.0332512473563,
21.8518161459093));
#28473=CARTESIAN_POINT('Ctrl Pts',(-33.7156105587364,-57.4345173729249,
21.888862109432));
#28474=CARTESIAN_POINT('Ctrl Pts',(-33.3386790321557,-57.8357834984935,
21.9259080729546));
#28475=CARTESIAN_POINT('Ctrl Pts',(-32.7446991236385,-58.0302073467771,
21.9629540364773));
#28476=CARTESIAN_POINT('Ctrl Pts',(-32.1997834265916,-57.930378193668,22.));
#28477=CARTESIAN_POINT('',(-30.9279127562904,-55.7311233941162,22.));
#28478=CARTESIAN_POINT('Origin',(-32.5,-56.2916512459885,22.));
#28479=CARTESIAN_POINT('Ctrl Pts',(-30.9279109916838,-55.7311226632893,
22.));
#28480=CARTESIAN_POINT('Ctrl Pts',(-30.7469516062031,-56.2407356224362,
21.9636770818144));
#28481=CARTESIAN_POINT('Ctrl Pts',(-30.8361764319304,-56.8473747622875,
21.9273541636289));
#28482=CARTESIAN_POINT('Ctrl Pts',(-31.157356786616,-57.282481394961,21.8910312454433));
#28483=CARTESIAN_POINT('Ctrl Pts',(-31.4849305691822,-57.726249276169,21.8539852819207));
#28484=CARTESIAN_POINT('Ctrl Pts',(-32.053786423629,-57.9915876156774,21.816939318398));
#28485=CARTESIAN_POINT('Ctrl Pts',(-32.604106443046,-57.9571481822401,21.7798933548753));
#28486=CARTESIAN_POINT('Ctrl Pts',(-33.1544264624631,-57.9227087488028,
21.7428473913526));
#28487=CARTESIAN_POINT('Ctrl Pts',(-33.6862106468504,-57.5884915424199,
21.7058014278299));
#28488=CARTESIAN_POINT('Ctrl Pts',(-33.9558248450097,-57.1074100574699,
21.6687554643072));
#28489=CARTESIAN_POINT('Ctrl Pts',(-34.2254390431691,-56.6263285725199,
21.6317095007845));
#28490=CARTESIAN_POINT('Ctrl Pts',(-34.2328832551006,-55.9983828090028,
21.5946635372619));
#28491=CARTESIAN_POINT('Ctrl Pts',(-33.9748805050844,-55.5109771631464,
21.5576175737392));
#28492=CARTESIAN_POINT('Ctrl Pts',(-33.7168777550681,-55.02357151729,21.5205716102165));
#28493=CARTESIAN_POINT('Ctrl Pts',(-33.1934280431042,-54.6767059890943,
21.4835256466938));
#28494=CARTESIAN_POINT('Ctrl Pts',(-32.6440261878896,-54.6291148312821,
21.4464796831712));
#28495=CARTESIAN_POINT('Ctrl Pts',(-32.3080707772689,-54.6000131695149,
21.4238263343174));
#28496=CARTESIAN_POINT('Ctrl Pts',(-31.9624112442361,-54.6828172989955,
21.4011729854636));
#28497=CARTESIAN_POINT('Ctrl Pts',(-31.667262219952,-54.851191363199,21.3785196366098));
#28498=CARTESIAN_POINT('Origin',(-32.5,-56.2916512459885,23.5459252805377));
#28499=CARTESIAN_POINT('',(-31.4703515173367,-54.5106388084307,13.4540747194623));
#28500=CARTESIAN_POINT('',(-31.474888731711,-54.5145036461352,13.3959252805377));
#28501=CARTESIAN_POINT('',(-31.4726249999999,-54.5121855475625,23.5459252805377));
#28502=CARTESIAN_POINT('',(-34.1542537360139,-57.5104384051693,13.));
#28503=CARTESIAN_POINT('Ctrl Pts',(-31.474888731711,-54.5145036461352,13.3959252805377));
#28504=CARTESIAN_POINT('Ctrl Pts',(-31.1415381650012,-54.7083242075053,
13.3750880775932));
#28505=CARTESIAN_POINT('Ctrl Pts',(-30.3573574995583,-55.4957610011486,
13.317204911126));
#28506=CARTESIAN_POINT('Ctrl Pts',(-30.3807647535574,-57.4808407355902,
13.2222757811361));
#28507=CARTESIAN_POINT('Ctrl Pts',(-32.3530480505925,-58.7147951819942,
13.1111378905681));
#28508=CARTESIAN_POINT('Ctrl Pts',(-33.748978009428,-58.0605171287351,13.0370459635227));
#28509=CARTESIAN_POINT('Ctrl Pts',(-34.1542537360139,-57.5104384051693,
13.));
#28510=CARTESIAN_POINT('',(-34.5453697724995,-56.5236298181907,13.));
#28511=CARTESIAN_POINT('Origin',(-32.5,-56.2916512459885,13.));
#28512=CARTESIAN_POINT('Ctrl Pts',(-31.4703515173367,-54.5106388084307,
13.4540747194623));
#28513=CARTESIAN_POINT('Ctrl Pts',(-31.4080578130841,-54.5460236433933,
13.4501772883951));
#28514=CARTESIAN_POINT('Ctrl Pts',(-30.7746715994702,-54.9531541715192,
13.4092338938053));
#28515=CARTESIAN_POINT('Ctrl Pts',(-30.074887383932,-56.4258925346357,13.3312445356927));
#28516=CARTESIAN_POINT('Ctrl Pts',(-31.2980228170538,-58.4019167094403,
13.2201066451247));
#28517=CARTESIAN_POINT('Ctrl Pts',(-33.60498859151,-58.4457294765997,13.1096917998938));
#28518=CARTESIAN_POINT('Ctrl Pts',(-34.469350039682,-57.1862605871605,13.0363229181856));
#28519=CARTESIAN_POINT('Ctrl Pts',(-34.5453721234944,-56.52362996598,13.));
#28520=CARTESIAN_POINT('Origin',(-32.5,-56.2916512459885,23.5459252805377));
#28521=CARTESIAN_POINT('',(-31.4731479817858,-54.5151444612292,14.1540747194623));
#28522=CARTESIAN_POINT('',(-31.472961077924,-54.5097720381012,14.0959252805377));
#28523=CARTESIAN_POINT('',(-31.4726249999999,-54.5121855475625,23.5459252805377));
#28524=CARTESIAN_POINT('Ctrl Pts',(-31.472961077924,-54.5097720381012,14.0959252805377));
#28525=CARTESIAN_POINT('Ctrl Pts',(-30.9672759169724,-54.8072848061286,
14.0640305253959));
#28526=CARTESIAN_POINT('Ctrl Pts',(-30.1471997784249,-55.9394877473567,
13.9950898067314));
#28527=CARTESIAN_POINT('Ctrl Pts',(-30.8240773215828,-58.0494183789814,
13.8891031245444));
#28528=CARTESIAN_POINT('Ctrl Pts',(-33.0679207153753,-58.6529675412989,
13.7779652339763));
#28529=CARTESIAN_POINT('Ctrl Pts',(-34.7917858342248,-57.0952271533932,
13.6668273434083));
#28530=CARTESIAN_POINT('Ctrl Pts',(-34.4182616640155,-54.8018644711707,
13.5556894528402));
#28531=CARTESIAN_POINT('Ctrl Pts',(-32.6876568692322,-54.0466007600429,
13.4653887652167));
#28532=CARTESIAN_POINT('Ctrl Pts',(-31.7341941451479,-54.3637352784833,
13.4121340411158));
#28533=CARTESIAN_POINT('Ctrl Pts',(-31.474888731711,-54.5145036461352,13.3959252805377));
#28534=CARTESIAN_POINT('Ctrl Pts',(-31.4731479817858,-54.5151444612292,
14.1540747194623));
#28535=CARTESIAN_POINT('Ctrl Pts',(-31.2328780723112,-54.6524190875731,
14.1391197361979));
#28536=CARTESIAN_POINT('Ctrl Pts',(-30.4914633330274,-55.2894948776179,
14.0871187894108));
#28537=CARTESIAN_POINT('Ctrl Pts',(-30.2211615693062,-57.1314551632494,
13.998071879101));
#28538=CARTESIAN_POINT('Ctrl Pts',(-31.9696590133091,-58.6616944230991,
13.886933988533));
#28539=CARTESIAN_POINT('Ctrl Pts',(-34.2035641928434,-58.0226004643432,
13.7757960979649));
#28540=CARTESIAN_POINT('Ctrl Pts',(-34.8782165391171,-55.7991607039093,
13.6646582073969));
#28541=CARTESIAN_POINT('Ctrl Pts',(-33.4286636629751,-54.0886449425481,
13.557417747896));
#28542=CARTESIAN_POINT('Ctrl Pts',(-32.0001735569318,-54.2096827863809,
13.4872232519178));
#28543=CARTESIAN_POINT('Ctrl Pts',(-31.4703515173367,-54.5106388084307,
13.4540747194623));
#28544=CARTESIAN_POINT('Origin',(-32.5,-56.2916512459885,23.5459252805377));
#28545=CARTESIAN_POINT('',(-31.4747795225871,-54.5123867379958,14.8540747194623));
#28546=CARTESIAN_POINT('',(-31.4704412404259,-54.5116709695925,14.7959252805377));
#28547=CARTESIAN_POINT('',(-31.4726249999999,-54.5121855475625,23.5459252805377));
#28548=CARTESIAN_POINT('Ctrl Pts',(-31.4704412404259,-54.5116709695925,
14.7959252805377));
#28549=CARTESIAN_POINT('Ctrl Pts',(-31.3758333938148,-54.5652019692603,
14.7900189367213));
#28550=CARTESIAN_POINT('Ctrl Pts',(-30.720757421839,-55.0095411304486,14.7470666293823));
#28551=CARTESIAN_POINT('Ctrl Pts',(-30.0858692295543,-56.5568634086542,
14.6670683585206));
#28552=CARTESIAN_POINT('Ctrl Pts',(-31.4135291597177,-58.4637350403727,
14.5559304679526));
#28553=CARTESIAN_POINT('Ctrl Pts',(-33.73564936737,-58.3824733534297,14.4447925773845));
#28554=CARTESIAN_POINT('Ctrl Pts',(-34.926763301881,-56.3874592577879,14.3336546868165));
#28555=CARTESIAN_POINT('Ctrl Pts',(-33.8966380568543,-54.3047494455222,
14.2225167962484));
#28556=CARTESIAN_POINT('Ctrl Pts',(-32.2506444060776,-54.1164611126689,
14.1432736608222));
#28557=CARTESIAN_POINT('Ctrl Pts',(-31.5546324883995,-54.4617218098652,
14.1010764889186));
#28558=CARTESIAN_POINT('Ctrl Pts',(-31.472961077924,-54.5097720381012,14.0959252805377));
#28559=CARTESIAN_POINT('Ctrl Pts',(-31.4747795225871,-54.5123867379958,
14.8540747194623));
#28560=CARTESIAN_POINT('Ctrl Pts',(-31.0607155624738,-54.7559913454825,
14.8280621840006));
#28561=CARTESIAN_POINT('Ctrl Pts',(-30.2508194018851,-55.6943396944676,
14.7650036850163));
#28562=CARTESIAN_POINT('Ctrl Pts',(-30.5678191761536,-57.7630592969624,
14.6648992225092));
#28563=CARTESIAN_POINT('Ctrl Pts',(-32.6883055651204,-58.7129949703236,
14.5537613319412));
#28564=CARTESIAN_POINT('Ctrl Pts',(-34.6364334330514,-57.4466471822883,
14.4426234413732));
#28565=CARTESIAN_POINT('Ctrl Pts',(-34.6290601547835,-55.1231186965397,
14.3314855508051));
#28566=CARTESIAN_POINT('Ctrl Pts',(-32.9361539945055,-54.0378965296929,
14.2353026435015));
#28567=CARTESIAN_POINT('Ctrl Pts',(-31.8280663212454,-54.3123671657349,
14.1761656997206));
#28568=CARTESIAN_POINT('Ctrl Pts',(-31.4731479817858,-54.5151444612292,
14.1540747194623));
#28569=CARTESIAN_POINT('Origin',(-32.5,-56.2916512459885,23.5459252805377));
#28570=CARTESIAN_POINT('',(-31.4709133736318,-54.5092374781621,15.5540747194623));
#28571=CARTESIAN_POINT('',(-31.4738352212016,-54.5152196643081,15.4959252805377));
#28572=CARTESIAN_POINT('',(-31.4726249999999,-54.5121855475625,23.5459252805377));
#28573=CARTESIAN_POINT('Ctrl Pts',(-31.4738352212016,-54.515219664308,15.4959252805377));
#28574=CARTESIAN_POINT('Ctrl Pts',(-31.201543391866,-54.6716871554888,15.4789613845241));
#28575=CARTESIAN_POINT('Ctrl Pts',(-30.4440567807226,-55.3577373025941,
15.4249515249878));
#28576=CARTESIAN_POINT('Ctrl Pts',(-30.269905357807,-57.2534431023133,15.3338957019289));
#28577=CARTESIAN_POINT('Ctrl Pts',(-32.0985763090804,-58.6869016992398,
15.2227578113608));
#28578=CARTESIAN_POINT('Ctrl Pts',(-34.2946749356979,-57.9279603862777,
15.1116199207928));
#28579=CARTESIAN_POINT('Ctrl Pts',(-34.848087203459,-55.6712867722916,15.0004820302248));
#28580=CARTESIAN_POINT('Ctrl Pts',(-33.3370773338915,-54.0721923398817,
14.895250483473));
#28581=CARTESIAN_POINT('Ctrl Pts',(-31.9692358342251,-54.229443076332,14.827064900244));
#28582=CARTESIAN_POINT('Ctrl Pts',(-31.4704412404259,-54.5116709695925,
14.7959252805377));
#28583=CARTESIAN_POINT('Ctrl Pts',(-31.4709133820845,-54.5092374927209,
15.5540747194623));
#28584=CARTESIAN_POINT('Ctrl Pts',(-31.4705297975013,-54.5094589248369,
15.5540505953261));
#28585=CARTESIAN_POINT('Ctrl Pts',(-30.8812194784826,-54.8499291446222,
15.5169805076671));
#28586=CARTESIAN_POINT('Ctrl Pts',(-30.074257404191,-56.1727516226364,15.4428644564856));
#28587=CARTESIAN_POINT('Ctrl Pts',(-31.0845179881232,-58.2651696619898,
15.3317265659175));
#28588=CARTESIAN_POINT('Ctrl Pts',(-33.3903853125313,-58.551203914661,15.2205886753495));
#28589=CARTESIAN_POINT('Ctrl Pts',(-34.8812728580259,-56.7690439832156,
15.1094507847814));
#28590=CARTESIAN_POINT('Ctrl Pts',(-34.192554360499,-54.5499210682071,14.9983128942134));
#28591=CARTESIAN_POINT('Ctrl Pts',(-32.4784241363503,-54.0712848045823,
14.913187539107));
#28592=CARTESIAN_POINT('Ctrl Pts',(-31.6504081122452,-54.4090598663806,
14.8651081475233));
#28593=CARTESIAN_POINT('Ctrl Pts',(-31.4747795225871,-54.5123867379958,
14.8540747194623));
#28594=CARTESIAN_POINT('Origin',(-32.5,-56.2916512459885,23.5459252805377));
#28595=CARTESIAN_POINT('',(-31.4717385551609,-54.5141703251839,16.2540747194623));
#28596=CARTESIAN_POINT('',(-31.4743433646119,-54.5114040111285,16.1959252805377));
#28597=CARTESIAN_POINT('',(-31.4726249999999,-54.5121855475625,23.5459252805377));
#28598=CARTESIAN_POINT('Ctrl Pts',(-31.4743433646119,-54.5114040111285,
16.1959252805377));
#28599=CARTESIAN_POINT('Ctrl Pts',(-31.0291266592638,-54.7738828820724,
16.1679038323268));
#28600=CARTESIAN_POINT('Ctrl Pts',(-30.2132159159802,-55.7757147456513,
16.1028364205933));
#28601=CARTESIAN_POINT('Ctrl Pts',(-30.6502037274999,-57.8653791294726,
16.0007230453371));
#28602=CARTESIAN_POINT('Ctrl Pts',(-32.8189508948268,-58.6992716537698,
15.8895851547691));
#28603=CARTESIAN_POINT('Ctrl Pts',(-34.6957586912586,-57.3294419144583,
15.778447264201));
#28604=CARTESIAN_POINT('Ctrl Pts',(-34.5627636554057,-55.0097106071377,
15.667309373633));
#28605=CARTESIAN_POINT('Ctrl Pts',(-32.8501896837687,-54.0383319846292,
15.5731353790785));
#28606=CARTESIAN_POINT('Ctrl Pts',(-31.7961776179314,-54.3299915352064,
15.5160073480468));
#28607=CARTESIAN_POINT('Ctrl Pts',(-31.4738352212016,-54.515219664308,15.4959252805377));
#28608=CARTESIAN_POINT('Ctrl Pts',(-31.4717385551609,-54.5141703251839,
16.2540747194623));
#28609=CARTESIAN_POINT('Ctrl Pts',(-31.2936631692288,-54.6150534746527,
16.2429930431288));
#28610=CARTESIAN_POINT('Ctrl Pts',(-30.586678710615,-55.1642906384242,16.1948654032726));
#28611=CARTESIAN_POINT('Ctrl Pts',(-30.1461151763816,-56.8896399584928,
16.1096917998938));
#28612=CARTESIAN_POINT('Ctrl Pts',(-31.7257879044833,-58.5935982250311,
15.9985539093258));
#28613=CARTESIAN_POINT('Ctrl Pts',(-34.0141057438103,-58.1905583158083,
15.8874160187577));
#28614=CARTESIAN_POINT('Ctrl Pts',(-34.9165454246277,-56.0494272304867,
15.7762781281897));
#28615=CARTESIAN_POINT('Ctrl Pts',(-33.6073779089676,-54.1304231724864,
15.6651643617579));
#28616=CARTESIAN_POINT('Ctrl Pts',(-32.0595772284103,-54.1694191401902,
15.5910965588487));
#28617=CARTESIAN_POINT('Ctrl Pts',(-31.4709133820845,-54.5092374927209,
15.5540747194623));
#28618=CARTESIAN_POINT('Origin',(-32.5,-56.2916512459885,23.5459252805377));
#28619=CARTESIAN_POINT('',(-31.4749299874422,-54.5140996860483,16.9540747194623));
#28620=CARTESIAN_POINT('',(-31.4704693279511,-54.5098093620654,16.8959252805377));
#28621=CARTESIAN_POINT('',(-31.4726249999999,-54.5121855475625,23.5459252805377));
#28622=CARTESIAN_POINT('Ctrl Pts',(-31.4704693279511,-54.5098093620654,
16.8959252805377));
#28623=CARTESIAN_POINT('Ctrl Pts',(-31.4380523744923,-54.528339714304,16.8938922436523));
#28624=CARTESIAN_POINT('Ctrl Pts',(-30.8255360958299,-54.9025793613845,
16.8548132432442));
#28625=CARTESIAN_POINT('Ctrl Pts',(-30.0713767023175,-56.3040842326063,
16.7786882793134));
#28626=CARTESIAN_POINT('Ctrl Pts',(-31.1932955779139,-58.3388173981362,
16.6675503887454));
#28627=CARTESIAN_POINT('Ctrl Pts',(-33.5112558300796,-58.4997561681628,
16.5564124981773));
#28628=CARTESIAN_POINT('Ctrl Pts',(-34.9036021525567,-56.6395914613089,
16.4452746076093));
#28629=CARTESIAN_POINT('Ctrl Pts',(-34.0959041660875,-54.4609531294646,
16.3341367170413));
#28630=CARTESIAN_POINT('Ctrl Pts',(-32.3994057229947,-54.0847909276367,
16.251020274684));
#28631=CARTESIAN_POINT('Ctrl Pts',(-31.61772870802,-54.4268707431815,16.2049497958495));
#28632=CARTESIAN_POINT('Ctrl Pts',(-31.4743433646119,-54.5114040111285,
16.1959252805377));
#28633=CARTESIAN_POINT('Ctrl Pts',(-31.4749299874422,-54.5140996860483,
16.9540747194623));
#28634=CARTESIAN_POINT('Ctrl Pts',(-31.1211066997161,-54.7205458521634,
16.9319354909316));
#28635=CARTESIAN_POINT('Ctrl Pts',(-30.3290943933324,-55.5443071105387,
16.8727502988781));
#28636=CARTESIAN_POINT('Ctrl Pts',(-30.4251293279102,-57.5539016004218,
16.776519143302));
#28637=CARTESIAN_POINT('Ctrl Pts',(-32.4351932585659,-58.7194412594432,
16.665381252734));
#28638=CARTESIAN_POINT('Ctrl Pts',(-34.5045755346153,-57.6627971861383,
16.554243362166));
#28639=CARTESIAN_POINT('Ctrl Pts',(-34.7391470903974,-55.3511276839614,
16.4431054715979));
#28640=CARTESIAN_POINT('Ctrl Pts',(-33.1051720185616,-54.0449906258011,
16.3430492573634));
#28641=CARTESIAN_POINT('Ctrl Pts',(-31.8889678914565,-54.277801838456,16.2800390066515));
#28642=CARTESIAN_POINT('Ctrl Pts',(-31.4717385551609,-54.5141703251839,
16.2540747194623));
#28643=CARTESIAN_POINT('Origin',(-32.5,-56.2916512459885,23.5459252805377));
#28644=CARTESIAN_POINT('',(-31.4724078687478,-54.5094050924838,17.6540747194623));
#28645=CARTESIAN_POINT('',(-31.4724615607262,-54.5148044353696,17.5959252805377));
#28646=CARTESIAN_POINT('',(-31.4726249999999,-54.5121855475625,23.5459252805377));
#28647=CARTESIAN_POINT('Ctrl Pts',(-31.4724615607262,-54.5148044353696,
17.5959252805377));
#28648=CARTESIAN_POINT('Ctrl Pts',(-31.2620673353104,-54.6344533407431,
17.582834691455));
#28649=CARTESIAN_POINT('Ctrl Pts',(-30.5366971614125,-55.2281953867951,
17.5326981388497));
#28650=CARTESIAN_POINT('Ctrl Pts',(-30.1818911638421,-57.0160386595509,
17.4455156227217));
#28651=CARTESIAN_POINT('Ctrl Pts',(-31.8513854749211,-58.6320924221469,
17.3343777321536));
#28652=CARTESIAN_POINT('Ctrl Pts',(-34.1145640165938,-58.1059138337969,
17.2232398415856));
#28653=CARTESIAN_POINT('Ctrl Pts',(-34.899913803477,-55.9191201236888,17.1121019510176));
#28654=CARTESIAN_POINT('Ctrl Pts',(-33.5144124105785,-54.1070736669905,
17.0029970973349));
#28655=CARTESIAN_POINT('Ctrl Pts',(-32.0287535486679,-54.190679951206,16.930938207175));
#28656=CARTESIAN_POINT('Ctrl Pts',(-31.4704693279511,-54.5098093620654,
16.8959252805377));
#28657=CARTESIAN_POINT('Ctrl Pts',(-31.4724078687478,-54.5094050924838,
17.6540747194623));
#28658=CARTESIAN_POINT('Ctrl Pts',(-30.946094870988,-54.8181696162505,17.6208779387343));
#28659=CARTESIAN_POINT('Ctrl Pts',(-30.1270731190027,-55.9965693019247,
17.5506351944836));
#28660=CARTESIAN_POINT('Ctrl Pts',(-30.8867448926705,-58.1070774278645,
17.4433464867103));
#28661=CARTESIAN_POINT('Ctrl Pts',(-33.1503020054966,-58.6316238024116,
17.3322085961423));
#28662=CARTESIAN_POINT('Ctrl Pts',(-34.8186303177654,-57.0143667589707,
17.2210707055742));
#28663=CARTESIAN_POINT('Ctrl Pts',(-34.3646900051272,-54.7356000103461,
17.1099328150062));
#28664=CARTESIAN_POINT('Ctrl Pts',(-32.6344025598171,-54.051324400594,17.0209341529689));
#28665=CARTESIAN_POINT('Ctrl Pts',(-31.7131654786556,-54.375095823104,16.9689814544542));
#28666=CARTESIAN_POINT('Ctrl Pts',(-31.4749299874422,-54.5140996860483,
16.9540747194623));
#28667=CARTESIAN_POINT('Origin',(-32.5,-56.2916512459885,23.5459252805377));
#28668=CARTESIAN_POINT('',(-31.470650904959,-54.5123645943458,18.3540747194623));
#28669=CARTESIAN_POINT('',(-31.4749676053556,-54.5132671274454,18.2959252805377));
#28670=CARTESIAN_POINT('',(-31.4726249999999,-54.5121855475625,23.5459252805377));
#28671=CARTESIAN_POINT('Ctrl Pts',(-31.4749676053556,-54.5132671274454,
18.2959252805377));
#28672=CARTESIAN_POINT('Ctrl Pts',(-31.0898434852659,-54.7390742900299,
18.2717771392578));
#28673=CARTESIAN_POINT('Ctrl Pts',(-30.2875910450901,-55.6209976925707,
18.2105830344552));
#28674=CARTESIAN_POINT('Ctrl Pts',(-30.4964134968882,-57.664242527379,18.1123429661299));
#28675=CARTESIAN_POINT('Ctrl Pts',(-32.5665574496276,-58.7193941910097,
18.0012050755619));
#28676=CARTESIAN_POINT('Ctrl Pts',(-34.57578061391,-57.5524052045849,17.8900671849938));
#28677=CARTESIAN_POINT('Ctrl Pts',(-34.6850182413274,-55.2314338219344,
17.7789292944258));
#28678=CARTESIAN_POINT('Ctrl Pts',(-33.0169876554982,-54.0399676860015,
17.6808819929404));
#28679=CARTESIAN_POINT('Ctrl Pts',(-31.8574765068094,-54.295850627297,17.6198806549777));
#28680=CARTESIAN_POINT('Ctrl Pts',(-31.4724615607262,-54.5148044353696,
17.5959252805377));
#28681=CARTESIAN_POINT('Ctrl Pts',(-31.470650904959,-54.5123645943458,18.3540747194623));
#28682=CARTESIAN_POINT('Ctrl Pts',(-31.3550533194394,-54.5776997670471,
18.3468663500598));
#28683=CARTESIAN_POINT('Ctrl Pts',(-30.6863525478934,-55.0471677720896,
18.3026120171345));
#28684=CARTESIAN_POINT('Ctrl Pts',(-30.0966496704334,-56.6413246029078,
18.2213117206866));
#28685=CARTESIAN_POINT('Ctrl Pts',(-31.4903368545418,-58.5004845570078,
18.1101738301185));
#28686=CARTESIAN_POINT('Ctrl Pts',(-33.8081801660464,-58.3378743316584,
17.9990359395505));
#28687=CARTESIAN_POINT('Ctrl Pts',(-34.928631335797,-56.3023329102471,17.8878980489824));
#28688=CARTESIAN_POINT('Ctrl Pts',(-33.8261287013397,-54.2570144404017,
17.7767601584144));
#28689=CARTESIAN_POINT('Ctrl Pts',(-32.2016889552716,-54.1286817447541,
17.6988190485744));
#28690=CARTESIAN_POINT('Ctrl Pts',(-31.5334341156058,-54.4736036964922,
17.657923902257));
#28691=CARTESIAN_POINT('Ctrl Pts',(-31.4724078687478,-54.5094050924838,
17.6540747194623));
#28692=CARTESIAN_POINT('Origin',(-32.5,-56.2916512459885,23.5459252805377));
#28693=CARTESIAN_POINT('',(-31.4742218141004,-54.5151075144861,19.0540747194623));
#28694=CARTESIAN_POINT('',(-31.4715682025536,-54.5091203612935,18.9959252805377));
#28695=CARTESIAN_POINT('',(-31.4726249999999,-54.5121855475625,23.5459252805377));
#28696=CARTESIAN_POINT('Ctrl Pts',(-31.4715682025536,-54.5091203612935,
18.9959252805377));
#28697=CARTESIAN_POINT('Ctrl Pts',(-30.9129158471523,-54.834613753627,18.9607195870605));
#28698=CARTESIAN_POINT('Ctrl Pts',(-30.0982487947042,-56.0866128816227,
18.8884679300607));
#28699=CARTESIAN_POINT('Ctrl Pts',(-30.9872637967358,-58.1916498987633,
18.7791703095382));
#28700=CARTESIAN_POINT('Ctrl Pts',(-33.2758719583609,-58.5930396107435,
18.6680324189701));
#28701=CARTESIAN_POINT('Ctrl Pts',(-34.8543157175077,-56.8879424529461,
18.5568945284021));
#28702=CARTESIAN_POINT('Ctrl Pts',(-34.2778276006655,-54.6370531910174,
18.445756637834));
#28703=CARTESIAN_POINT('Ctrl Pts',(-32.5529073535807,-54.0606456221556,
18.3587668885459));
#28704=CARTESIAN_POINT('Ctrl Pts',(-31.6806671821781,-54.3926607167737,
18.3088231027804));
#28705=CARTESIAN_POINT('Ctrl Pts',(-31.4749676053556,-54.5132671274454,
18.2959252805377));
#28706=CARTESIAN_POINT('Ctrl Pts',(-31.4742218141004,-54.5151075144861,
19.0540747194623));
#28707=CARTESIAN_POINT('Ctrl Pts',(-31.1812845288231,-54.6841025371816,
19.0358087978625));
#28708=CARTESIAN_POINT('Ctrl Pts',(-30.4141219270718,-55.4032020294196,
18.98049691274));
#28709=CARTESIAN_POINT('Ctrl Pts',(-30.3049905142645,-57.3310249135316,
18.8881390640948));
#28710=CARTESIAN_POINT('Ctrl Pts',(-32.182785399016,-58.6995007346588,18.7770011735268));
#28711=CARTESIAN_POINT('Ctrl Pts',(-34.3509304054687,-57.8640446119295,
18.6658632829587));
#28712=CARTESIAN_POINT('Ctrl Pts',(-34.8248978208363,-55.5893590092039,
18.5547253923907));
#28713=CARTESIAN_POINT('Ctrl Pts',(-33.2781402858533,-54.0633320127348,
18.4507958712252));
#28714=CARTESIAN_POINT('Ctrl Pts',(-31.9491438407914,-54.2419227987111,
18.3839123135824));
#28715=CARTESIAN_POINT('Ctrl Pts',(-31.470650904959,-54.5123645943458,18.3540747194623));
#28716=CARTESIAN_POINT('Origin',(-32.5,-56.2916512459885,23.5459252805377));
#28717=CARTESIAN_POINT('',(-31.4739455702221,-54.5107934605777,19.7540747194623));
#28718=CARTESIAN_POINT('',(-31.471143914755,-54.5133742931914,19.6959252805377));
#28719=CARTESIAN_POINT('',(-31.4726249999999,-54.5121855475625,23.5459252805377));
#28720=CARTESIAN_POINT('Ctrl Pts',(-31.471143914755,-54.5133742931914,19.6959252805377));
#28721=CARTESIAN_POINT('Ctrl Pts',(-31.3231329415045,-54.5970512593892,
19.6867079983859));
#28722=CARTESIAN_POINT('Ctrl Pts',(-30.6341370241162,-55.106929574873,19.6404447527115));
#28723=CARTESIAN_POINT('Ctrl Pts',(-30.1190717238489,-56.77076109083,19.5571355435145));
#28724=CARTESIAN_POINT('Ctrl Pts',(-31.611244210167,-58.5518456729879,19.4459976529464));
#28725=CARTESIAN_POINT('Ctrl Pts',(-33.9169049506455,-58.2641486635056,
19.3348597623784));
#28726=CARTESIAN_POINT('Ctrl Pts',(-34.9256565207284,-56.1710023982575,
19.2237218718104));
#28727=CARTESIAN_POINT('Ctrl Pts',(-33.71417716871,-54.1882873915237,19.1125839812423));
#28728=CARTESIAN_POINT('Ctrl Pts',(-32.1271617475077,-54.1490140977469,
19.0366517841514));
#28729=CARTESIAN_POINT('Ctrl Pts',(-31.5007700473113,-54.4921061888467,
18.9977655505832));
#28730=CARTESIAN_POINT('Ctrl Pts',(-31.4715682025536,-54.5091203612935,
18.9959252805377));
#28731=CARTESIAN_POINT('Ctrl Pts',(-31.4739455702221,-54.5107934605777,
19.7540747194623));
#28732=CARTESIAN_POINT('Ctrl Pts',(-31.0084978875972,-54.7852778310984,
19.7247512456653));
#28733=CARTESIAN_POINT('Ctrl Pts',(-30.1900336005111,-55.8297589120183,
19.6583818083455));
#28734=CARTESIAN_POINT('Ctrl Pts',(-30.7065057264145,-57.9292539322017,
19.5549664075031));
#28735=CARTESIAN_POINT('Ctrl Pts',(-32.9031507850421,-58.6866113101154,
19.443828516935));
#28736=CARTESIAN_POINT('Ctrl Pts',(-34.730787355662,-57.2518345802401,19.332690626367));
#28737=CARTESIAN_POINT('Ctrl Pts',(-34.5165589620033,-54.9381911555042,
19.2215527357989));
#28738=CARTESIAN_POINT('Ctrl Pts',(-32.7951211292858,-54.0400334340293,
19.1286807668307));
#28739=CARTESIAN_POINT('Ctrl Pts',(-31.7754042355958,-54.3413558867002,
19.0728547613852));
#28740=CARTESIAN_POINT('Ctrl Pts',(-31.4742218141004,-54.5151075144861,
19.0540747194623));
#28741=CARTESIAN_POINT('Origin',(-32.5,-56.2916512459885,23.5459252805377));
#28742=CARTESIAN_POINT('',(-31.4703419245392,-54.5103623955759,20.4540747194623));
#28743=CARTESIAN_POINT('',(-31.4746836284317,-54.5147000883656,20.3959252805377));
#28744=CARTESIAN_POINT('',(-31.4726249999999,-54.5121855475625,23.5459252805377));
#28745=CARTESIAN_POINT('Ctrl Pts',(-31.4746836284317,-54.5147000883656,
20.3959252805377));
#28746=CARTESIAN_POINT('Ctrl Pts',(-31.1500699868132,-54.7031080152175,
20.3756504461887));
#28747=CARTESIAN_POINT('Ctrl Pts',(-30.3692379110719,-55.4752841065875,
20.318329648317));
#28748=CARTESIAN_POINT('Ctrl Pts',(-30.3643995989091,-57.4481876795404,
20.2239628869227));
#28749=CARTESIAN_POINT('Ctrl Pts',(-32.3134406037768,-58.7131304053242,
20.1128249963547));
#28750=CARTESIAN_POINT('Ctrl Pts',(-34.4332415751289,-57.7616657784424,
20.0016871057866));
#28751=CARTESIAN_POINT('Ctrl Pts',(-34.7835245906331,-55.4646801872418,
19.8905492152186));
#28752=CARTESIAN_POINT('Ctrl Pts',(-33.1879673210569,-54.052355442598,19.7886286068023));
#28753=CARTESIAN_POINT('Ctrl Pts',(-31.9180164468303,-54.2607380396757,
19.7237539619086));
#28754=CARTESIAN_POINT('Ctrl Pts',(-31.471143914755,-54.5133742931914,19.6959252805377));
#28755=CARTESIAN_POINT('Ctrl Pts',(-31.4703419245392,-54.5103623955759,
20.4540747194623));
#28756=CARTESIAN_POINT('Ctrl Pts',(-31.4170740978156,-54.5406699166123,
20.4507396569907));
#28757=CARTESIAN_POINT('Ctrl Pts',(-30.7899238920755,-54.9377208245812,
20.4103586309964));
#28758=CARTESIAN_POINT('Ctrl Pts',(-30.073305550394,-56.3892087930031,20.3329316414794));
#28759=CARTESIAN_POINT('Ctrl Pts',(-31.2658594095642,-58.3833638027876,
20.2217937509113));
#28760=CARTESIAN_POINT('Ctrl Pts',(-33.588036458114,-58.4629506390538,20.1106558603433));
#28761=CARTESIAN_POINT('Ctrl Pts',(-34.914321242052,-56.5551224909764,19.9995179697752));
#28762=CARTESIAN_POINT('Ctrl Pts',(-34.0307504904903,-54.406136137217,19.8883800792072));
#28763=CARTESIAN_POINT('Ctrl Pts',(-32.3488749925859,-54.0946310730832,
19.8065656624362));
#28764=CARTESIAN_POINT('Ctrl Pts',(-31.5965236444216,-54.4385065703594,
19.7617972091879));
#28765=CARTESIAN_POINT('Ctrl Pts',(-31.4739455702221,-54.5107934605777,
19.7540747194623));
#28766=CARTESIAN_POINT('Origin',(-32.5,-56.2916512459885,23.5459252805377));
#28767=CARTESIAN_POINT('',(-31.4729484072307,-54.5150696468519,21.1540747194623));
#28768=CARTESIAN_POINT('',(-31.4731950477465,-54.5099653993635,21.0959252805377));
#28769=CARTESIAN_POINT('',(-31.4726249999999,-54.5121855475625,23.5459252805377));
#28770=CARTESIAN_POINT('Ctrl Pts',(-31.4731950477465,-54.5099653993635,
21.0959252805377));
#28771=CARTESIAN_POINT('Ctrl Pts',(-30.9763557896561,-54.8025287224184,
21.0645928939914));
#28772=CARTESIAN_POINT('Ctrl Pts',(-30.1562124434263,-55.91515240492,20.9962145439225));
#28773=CARTESIAN_POINT('Ctrl Pts',(-30.7976747113088,-58.0238313492005,
20.890790230331));
#28774=CARTESIAN_POINT('Ctrl Pts',(-33.0320547584019,-58.6613103307746,
20.7796523397629));
#28775=CARTESIAN_POINT('Ctrl Pts',(-34.779441328077,-57.1298124049937,20.6685144491949));
#28776=CARTESIAN_POINT('Ctrl Pts',(-34.4404282620852,-54.8311366011663,
20.5573765586268));
#28777=CARTESIAN_POINT('Ctrl Pts',(-32.711178041167,-54.0447560839335,20.4665135024078));
#28778=CARTESIAN_POINT('Ctrl Pts',(-31.7432006097017,-54.3588510380505,
20.4126964097114));
#28779=CARTESIAN_POINT('Ctrl Pts',(-31.4746836284317,-54.5147000883656,
20.3959252805377));
#28780=CARTESIAN_POINT('Ctrl Pts',(-31.4729484072307,-54.5150696468519,
21.1540747194623));
#28781=CARTESIAN_POINT('Ctrl Pts',(-31.2416713093181,-54.6470066065867,
21.1396821047934));
#28782=CARTESIAN_POINT('Ctrl Pts',(-30.5049700979161,-55.27079766484,21.0882435266019));
#28783=CARTESIAN_POINT('Ctrl Pts',(-30.2087196709518,-57.0968534624393,
20.9997589848876));
#28784=CARTESIAN_POINT('Ctrl Pts',(-31.9338196700205,-58.6533891775714,
20.8886210943196));
#28785=CARTESIAN_POINT('Ctrl Pts',(-34.1771709144469,-58.0482026788782,
20.7774832037515));
#28786=CARTESIAN_POINT('Ctrl Pts',(-34.8853786224564,-55.8352230845946,
20.6663453131835));
#28787=CARTESIAN_POINT('Ctrl Pts',(-33.4544940412401,-54.0938892869953,
20.5585424850871));
#28788=CARTESIAN_POINT('Ctrl Pts',(-32.0087745479626,-54.2040131588077,
20.4877856205134));
#28789=CARTESIAN_POINT('Ctrl Pts',(-31.4703419245392,-54.5103623955759,
20.4540747194623));
#28790=CARTESIAN_POINT('Origin',(-32.5,-56.2916512459885,23.5459252805377));
#28791=CARTESIAN_POINT('',(-31.4756555660462,-54.5128362942924,21.8540747194623));
#28792=CARTESIAN_POINT('',(-31.4704151231923,-54.5113563798656,21.7959252805377));
#28793=CARTESIAN_POINT('',(-31.4726249999999,-54.5121855475625,23.5459252805377));
#28794=CARTESIAN_POINT('',(-33.9541262883781,-54.8399232067374,22.));
#28795=CARTESIAN_POINT('Ctrl Pts',(-33.9541262883781,-54.8399232067375,
22.));
#28796=CARTESIAN_POINT('Ctrl Pts',(-33.4713921772736,-54.3563916207415,
21.9629540364773));
#28797=CARTESIAN_POINT('Ctrl Pts',(-32.5011748783928,-54.0682382375653,
21.9143122762981));
#28798=CARTESIAN_POINT('Ctrl Pts',(-31.6603808354702,-54.4043184181514,
21.8656705161189));
#28799=CARTESIAN_POINT('Ctrl Pts',(-31.4756555660462,-54.5128362942924,
21.8540747194623));
#28800=CARTESIAN_POINT('',(-34.4879501863793,-55.7574173922323,22.));
#28801=CARTESIAN_POINT('Origin',(-32.5,-56.2916512459885,22.));
#28802=CARTESIAN_POINT('Ctrl Pts',(-34.4879524958972,-55.7574168944053,
22.));
#28803=CARTESIAN_POINT('Ctrl Pts',(-34.3140194691063,-55.1135181402384,
21.9636770818144));
#28804=CARTESIAN_POINT('Ctrl Pts',(-33.3475254337068,-54.0782693974496,
21.895652175327));
#28805=CARTESIAN_POINT('Ctrl Pts',(-31.9778124788844,-54.224015012867,21.8276272688396));
#28806=CARTESIAN_POINT('Ctrl Pts',(-31.4704151231923,-54.5113563798656,
21.7959252805377));
#28807=CARTESIAN_POINT('Origin',(32.5,-56.2916512459885,17.));
#28808=CARTESIAN_POINT('',(31.665169034441,-54.8481104542883,13.8714803633902));
#28809=CARTESIAN_POINT('',(31.6668355785527,-54.8466294620446,13.6785196366098));
#28810=CARTESIAN_POINT('',(31.667,-54.8488529232837,17.));
#28811=CARTESIAN_POINT('',(31.4059736530044,-55.03520293743,13.));
#28812=CARTESIAN_POINT('Ctrl Pts',(31.6668355785527,-54.8466294620446,13.6785196366098));
#28813=CARTESIAN_POINT('Ctrl Pts',(31.7169359983484,-54.8172333383902,13.6746222055426));
#28814=CARTESIAN_POINT('Ctrl Pts',(31.7685916060498,-54.790608714332,13.6707247744754));
#28815=CARTESIAN_POINT('Ctrl Pts',(31.8215990010622,-54.7670212268678,13.6668273434082));
#28816=CARTESIAN_POINT('Ctrl Pts',(32.3254462758994,-54.5428168252686,13.6297813798856));
#28817=CARTESIAN_POINT('Ctrl Pts',(32.9514266195489,-54.5930156597359,13.5927354163629));
#28818=CARTESIAN_POINT('Ctrl Pts',(33.4130263160919,-54.8947720750738,13.5556894528402));
#28819=CARTESIAN_POINT('Ctrl Pts',(33.8746260126349,-55.1965284904116,13.5186434893175));
#28820=CARTESIAN_POINT('Ctrl Pts',(34.1718450620713,-55.74984248662,13.4815975257948));
#28821=CARTESIAN_POINT('Ctrl Pts',(34.1687200176701,-56.3012302340885,13.4445515622722));
#28822=CARTESIAN_POINT('Ctrl Pts',(34.165594973269,-56.852617981557,13.4075055987495));
#28823=CARTESIAN_POINT('Ctrl Pts',(33.8621258350302,-57.4020794802856,13.3704596352268));
#28824=CARTESIAN_POINT('Ctrl Pts',(33.397076207884,-57.6986656733008,13.3334136717041));
#28825=CARTESIAN_POINT('Ctrl Pts',(32.9320265807378,-57.9952518663159,13.2963677081814));
#28826=CARTESIAN_POINT('Ctrl Pts',(32.3053964646841,-58.0389627536177,13.2593217446588));
#28827=CARTESIAN_POINT('Ctrl Pts',(31.8042046430419,-57.8087421867188,13.2222757811361));
#28828=CARTESIAN_POINT('Ctrl Pts',(31.3030128213997,-57.5785216198199,13.1852298176134));
#28829=CARTESIAN_POINT('Ctrl Pts',(30.927259294169,-57.0743695987204,13.1481838540907));
#28830=CARTESIAN_POINT('Ctrl Pts',(30.8485497633826,-56.5294873752106,13.111137890568));
#28831=CARTESIAN_POINT('Ctrl Pts',(30.7698402325962,-55.9846051517008,13.0740919270453));
#28832=CARTESIAN_POINT('Ctrl Pts',(30.9881746982541,-55.3989927257807,13.0370459635227));
#28833=CARTESIAN_POINT('Ctrl Pts',(31.4059736530044,-55.03520293743,13.));
#28834=CARTESIAN_POINT('',(33.9184188470958,-55.4120275291385,13.));
#28835=CARTESIAN_POINT('Origin',(32.5,-56.2916512459885,13.));
#28836=CARTESIAN_POINT('',(31.6677099856842,-54.8513822049942,13.1714803633902));
#28837=CARTESIAN_POINT('Ctrl Pts',(33.9184205240577,-55.4120266023846,13.));
#28838=CARTESIAN_POINT('Ctrl Pts',(33.6328154176795,-54.952808667466,13.0363229181856));
#28839=CARTESIAN_POINT('Ctrl Pts',(33.102895030897,-54.644333384024,13.0726458363711));
#28840=CARTESIAN_POINT('Ctrl Pts',(32.5624622032656,-54.6241575874771,13.1089687545567));
#28841=CARTESIAN_POINT('Ctrl Pts',(32.2524345659016,-54.6125834302173,13.1298059575012));
#28842=CARTESIAN_POINT('Ctrl Pts',(31.9389473679306,-54.6958863393048,13.1506431604457));
#28843=CARTESIAN_POINT('Ctrl Pts',(31.6677099856842,-54.8513822049942,13.1714803633902));
#28844=CARTESIAN_POINT('',(31.667,-54.8488529232837,12.));
#28845=CARTESIAN_POINT('',(31.667,-54.8488529232837,17.));
#28846=CARTESIAN_POINT('Origin',(32.5,-56.2916512459885,12.));
#28847=CARTESIAN_POINT('Ctrl Pts',(31.6677099856842,-54.8513822049942,13.1714803633902));
#28848=CARTESIAN_POINT('Ctrl Pts',(31.4567209292169,-54.9723387107482,13.1876891239684));
#28849=CARTESIAN_POINT('Ctrl Pts',(31.2712968605907,-55.1369785326559,13.2038978845465));
#28850=CARTESIAN_POINT('Ctrl Pts',(31.1329525371814,-55.334624580881,13.2201066451247));
#28851=CARTESIAN_POINT('Ctrl Pts',(30.8167594060732,-55.7863548817662,13.2571526086474));
#28852=CARTESIAN_POINT('Ctrl Pts',(30.7464989755799,-56.4105013743272,13.2941985721701));
#28853=CARTESIAN_POINT('Ctrl Pts',(30.9545219587097,-56.9212436588756,13.3312445356927));
#28854=CARTESIAN_POINT('Ctrl Pts',(31.1625449418395,-57.4319859434239,13.3682904992154));
#28855=CARTESIAN_POINT('Ctrl Pts',(31.6488513385922,-57.8293240199595,13.4053364627381));
#28856=CARTESIAN_POINT('Ctrl Pts',(32.1907825642961,-57.9315018386831,13.4423824262608));
#28857=CARTESIAN_POINT('Ctrl Pts',(32.7327137899999,-58.0336796574068,13.4794283897835));
#28858=CARTESIAN_POINT('Ctrl Pts',(33.3302698446549,-57.8406972183184,13.5164743533061));
#28859=CARTESIAN_POINT('Ctrl Pts',(33.7100246193121,-57.4408300847799,13.5535203168288));
#28860=CARTESIAN_POINT('Ctrl Pts',(34.0897793939693,-57.0409629512413,13.5905662803515));
#28861=CARTESIAN_POINT('Ctrl Pts',(34.2517328886288,-56.4342111232524,13.6276122438742));
#28862=CARTESIAN_POINT('Ctrl Pts',(34.1217417856583,-55.8982799679713,13.6646582073969));
#28863=CARTESIAN_POINT('Ctrl Pts',(33.9917506826877,-55.3623488126902,13.7017041709196));
#28864=CARTESIAN_POINT('Ctrl Pts',(33.5698149820871,-54.8972383301169,13.7387501344422));
#28865=CARTESIAN_POINT('Ctrl Pts',(33.0490481303447,-54.7157980032898,13.7757960979649));
#28866=CARTESIAN_POINT('Ctrl Pts',(32.6006934475977,-54.5595867930335,13.8076908531067));
#28867=CARTESIAN_POINT('Ctrl Pts',(32.0790815152818,-54.6136422361013,13.8395856082484));
#28868=CARTESIAN_POINT('Ctrl Pts',(31.665169034441,-54.8481104542883,13.8714803633902));
#28869=CARTESIAN_POINT('Origin',(32.5,-56.2916512459885,17.));
#28870=CARTESIAN_POINT('',(31.667523968133,-54.8471109129233,14.5714803633902));
#28871=CARTESIAN_POINT('',(31.668865652917,-54.8504196807178,14.3785196366098));
#28872=CARTESIAN_POINT('',(31.667,-54.8488529232837,17.));
#28873=CARTESIAN_POINT('Ctrl Pts',(31.668865652917,-54.8504196807178,14.3785196366098));
#28874=CARTESIAN_POINT('Ctrl Pts',(31.8626626794392,-54.7373590837469,14.3635646533453));
#28875=CARTESIAN_POINT('Ctrl Pts',(32.0777548846389,-54.6619147081679,14.3486096700809));
#28876=CARTESIAN_POINT('Ctrl Pts',(32.2987508779934,-54.6350670487033,14.3336546868165));
#28877=CARTESIAN_POINT('Ctrl Pts',(32.8461944534029,-54.5685609620293,14.2966087232938));
#28878=CARTESIAN_POINT('Ctrl Pts',(33.4298657229247,-54.8002611998549,14.2595627597711));
#28879=CARTESIAN_POINT('Ctrl Pts',(33.7826437493636,-55.2241308285784,14.2225167962484));
#28880=CARTESIAN_POINT('Ctrl Pts',(34.1354217758025,-55.648000457302,14.1854708327258));
#28881=CARTESIAN_POINT('Ctrl Pts',(34.2573065591586,-56.2640394769235,14.1484248692031));
#28882=CARTESIAN_POINT('Ctrl Pts',(34.0925177799173,-56.7903101462248,14.1113789056804));
#28883=CARTESIAN_POINT('Ctrl Pts',(33.9277290006759,-57.3165808155261,14.0743329421577));
#28884=CARTESIAN_POINT('Ctrl Pts',(33.4762666588371,-57.7530831345071,14.037286978635));
#28885=CARTESIAN_POINT('Ctrl Pts',(32.9447431684491,-57.9000573283161,14.0002410151124));
#28886=CARTESIAN_POINT('Ctrl Pts',(32.4132196780611,-58.0470315221252,13.9631950515897));
#28887=CARTESIAN_POINT('Ctrl Pts',(31.8016350391239,-57.9044775907623,13.926149088067));
#28888=CARTESIAN_POINT('Ctrl Pts',(31.38988820532,-57.537620165814,13.8891031245443));
#28889=CARTESIAN_POINT('Ctrl Pts',(30.9781413715162,-57.1707627408657,13.8520571610216));
#28890=CARTESIAN_POINT('Ctrl Pts',(30.7662323428457,-56.5796018223321,13.815011197499));
#28891=CARTESIAN_POINT('Ctrl Pts',(30.8511349315229,-56.0347175442324,13.7779652339763));
#28892=CARTESIAN_POINT('Ctrl Pts',(30.9271053193521,-55.5471579706766,13.7448167015208));
#28893=CARTESIAN_POINT('Ctrl Pts',(31.2407201802287,-55.0966501403397,13.7116681690653));
#28894=CARTESIAN_POINT('Ctrl Pts',(31.6668355785527,-54.8466294620446,13.6785196366098));
#28895=CARTESIAN_POINT('Ctrl Pts',(31.665169034441,-54.8481104542883,13.8714803633902));
#28896=CARTESIAN_POINT('Ctrl Pts',(31.5983195028865,-54.8859785816721,13.8766315717711));
#28897=CARTESIAN_POINT('Ctrl Pts',(31.5342792394079,-54.92855265549,13.881782780152));
#28898=CARTESIAN_POINT('Ctrl Pts',(31.4738105761082,-54.9757069077013,13.886933988533));
#28899=CARTESIAN_POINT('Ctrl Pts',(31.0389378764983,-55.3148263100205,13.9239799520556));
#28900=CARTESIAN_POINT('Ctrl Pts',(30.7887904801626,-55.8908352857396,13.9610259155783));
#28901=CARTESIAN_POINT('Ctrl Pts',(30.83785280129,-56.4401173240505,13.998071879101));
#28902=CARTESIAN_POINT('Ctrl Pts',(30.8869151224174,-56.9893993623615,14.0351178426237));
#28903=CARTESIAN_POINT('Ctrl Pts',(31.2351871610079,-57.5119544632642,14.0721638061464));
#28904=CARTESIAN_POINT('Ctrl Pts',(31.7232787251799,-57.7686336889847,14.109209769669));
#28905=CARTESIAN_POINT('Ctrl Pts',(32.2113702893519,-58.0253129147052,14.1462557331917));
#28906=CARTESIAN_POINT('Ctrl Pts',(32.8392813791053,-58.0161162652435,14.1833016967144));
#28907=CARTESIAN_POINT('Ctrl Pts',(33.3196456823451,-57.74525195635,14.2203476602371));
#28908=CARTESIAN_POINT('Ctrl Pts',(33.8000099855849,-57.4743876474564,14.2573936237598));
#28909=CARTESIAN_POINT('Ctrl Pts',(34.1328275023111,-56.9418556791311,14.2944395872824));
#28910=CARTESIAN_POINT('Ctrl Pts',(34.1657820298073,-56.3913726675535,14.3314855508051));
#28911=CARTESIAN_POINT('Ctrl Pts',(34.1987365573035,-55.8408896559759,14.3685315143278));
#28912=CARTESIAN_POINT('Ctrl Pts',(33.9318280955697,-55.272455601146,14.4055774778505));
#28913=CARTESIAN_POINT('Ctrl Pts',(33.4872090049183,-54.9462174010392,14.4426234413732));
#28914=CARTESIAN_POINT('Ctrl Pts',(33.0425899142668,-54.6199792009323,14.4796694048958));
#28915=CARTESIAN_POINT('Ctrl Pts',(32.4202601946977,-54.5359368555486,14.5167153684185));
#28916=CARTESIAN_POINT('Ctrl Pts',(31.905032476641,-54.7325529059598,14.5537613319412));
#28917=CARTESIAN_POINT('Ctrl Pts',(31.8228882493844,-54.7638999646704,14.5596676757575));
#28918=CARTESIAN_POINT('Ctrl Pts',(31.7434664303385,-54.8023810331132,14.5655740195739));
#28919=CARTESIAN_POINT('Ctrl Pts',(31.667523968133,-54.8471109129233,14.5714803633902));
#28920=CARTESIAN_POINT('Origin',(32.5,-56.2916512459885,17.));
#28921=CARTESIAN_POINT('',(31.6686398531931,-54.8509327367609,15.2714803633902));
#28922=CARTESIAN_POINT('',(31.6662678127889,-54.8504473245041,15.0785196366098));
#28923=CARTESIAN_POINT('',(31.667,-54.8488529232837,17.));
#28924=CARTESIAN_POINT('Ctrl Pts',(31.6662678127889,-54.8504473245041,15.0785196366098));
#28925=CARTESIAN_POINT('Ctrl Pts',(32.0051837911952,-54.6584589297703,15.0525071011481));
#28926=CARTESIAN_POINT('Ctrl Pts',(32.4124263355195,-54.5807898609867,15.0264945656864));
#28927=CARTESIAN_POINT('Ctrl Pts',(32.7936098272491,-54.6489198132192,15.0004820302247));
#28928=CARTESIAN_POINT('Ctrl Pts',(33.3364753910795,-54.745947637705,14.9634360667021));
#28929=CARTESIAN_POINT('Ctrl Pts',(33.8264872979809,-55.138688877304,14.9263901031794));
#28930=CARTESIAN_POINT('Ctrl Pts',(34.0393888128715,-55.6474033077565,14.8893441396567));
#28931=CARTESIAN_POINT('Ctrl Pts',(34.2522903277622,-56.156117738209,14.852298176134));
#28932=CARTESIAN_POINT('Ctrl Pts',(34.1880814506421,-56.7808053595149,14.8152522126113));
#28933=CARTESIAN_POINT('Ctrl Pts',(33.8761477528874,-57.2355742774498,14.7782062490887));
#28934=CARTESIAN_POINT('Ctrl Pts',(33.5642140551328,-57.6903431953847,14.741160285566));
#28935=CARTESIAN_POINT('Ctrl Pts',(33.0045555367437,-57.9751934099486,14.7041143220433));
#28936=CARTESIAN_POINT('Ctrl Pts',(32.4533030627753,-57.959761729544,14.6670683585206));
#28937=CARTESIAN_POINT('Ctrl Pts',(31.9020505888069,-57.9443300491395,14.6300223949979));
#28938=CARTESIAN_POINT('Ctrl Pts',(31.3592041592591,-57.6286164737664,14.5929764314753));
#28939=CARTESIAN_POINT('Ctrl Pts',(31.0732005795316,-57.1571088626351,14.5559304679526));
#28940=CARTESIAN_POINT('Ctrl Pts',(30.787196999804,-56.6856012515039,14.5188845044299));
#28941=CARTESIAN_POINT('Ctrl Pts',(30.7580362698966,-56.0582996046144,14.4818385409072));
#28942=CARTESIAN_POINT('Ctrl Pts',(30.9990638455916,-55.5622925755828,14.4447925773845));
#28943=CARTESIAN_POINT('Ctrl Pts',(31.142791661258,-55.2665172617734,14.4227015971263));
#28944=CARTESIAN_POINT('Ctrl Pts',(31.3825954370759,-55.0174288556201,14.400610616868));
#28945=CARTESIAN_POINT('Ctrl Pts',(31.668865652917,-54.8504196807178,14.3785196366098));
#28946=CARTESIAN_POINT('Ctrl Pts',(31.667523968133,-54.8471109129233,14.5714803633902));
#28947=CARTESIAN_POINT('Ctrl Pts',(31.2671376265686,-55.0829372532297,14.6026199830965));
#28948=CARTESIAN_POINT('Ctrl Pts',(30.9634650148059,-55.4924582968625,14.6337596028029));
#28949=CARTESIAN_POINT('Ctrl Pts',(30.8674364226636,-55.9459488454016,14.6648992225092));
#28950=CARTESIAN_POINT('Ctrl Pts',(30.7531938032872,-56.4854542882262,14.7019451860319));
#28951=CARTESIAN_POINT('Ctrl Pts',(30.9328342810787,-57.0871907276693,14.7389911495546));
#28952=CARTESIAN_POINT('Ctrl Pts',(31.3241443491424,-57.4757700913936,14.7760371130773));
#28953=CARTESIAN_POINT('Ctrl Pts',(31.715454417206,-57.8643494551178,14.8130830766));
#28954=CARTESIAN_POINT('Ctrl Pts',(32.3184340755416,-58.0397717431231,14.8501290401227));
#28955=CARTESIAN_POINT('Ctrl Pts',(32.8571262761764,-57.9217539399754,14.8871750036453));
#28956=CARTESIAN_POINT('Ctrl Pts',(33.3958184768112,-57.8037361368278,14.924220967168));
#28957=CARTESIAN_POINT('Ctrl Pts',(33.8702232197451,-57.3922782425271,14.9612669306907));
#28958=CARTESIAN_POINT('Ctrl Pts',(34.063226478426,-56.8756863008287,14.9983128942134));
#28959=CARTESIAN_POINT('Ctrl Pts',(34.2562297371068,-56.3590943591303,15.0353588577361));
#28960=CARTESIAN_POINT('Ctrl Pts',(34.1678315115345,-55.7373683700341,15.0724048212587));
#28961=CARTESIAN_POINT('Ctrl Pts',(33.8384877538371,-55.2950447552267,15.1094507847814));
#28962=CARTESIAN_POINT('Ctrl Pts',(33.5091439961397,-54.8527211404193,15.1464967483041));
#28963=CARTESIAN_POINT('Ctrl Pts',(32.9388547063171,-54.5897998999006,15.1835427118268));
#28964=CARTESIAN_POINT('Ctrl Pts',(32.3886160101468,-54.6266084315825,15.2205886753495));
#28965=CARTESIAN_POINT('Ctrl Pts',(32.1366535522459,-54.6434636040356,15.237552571363));
#28966=CARTESIAN_POINT('Ctrl Pts',(31.8888954229186,-54.7231679104083,15.2545164673766));
#28967=CARTESIAN_POINT('Ctrl Pts',(31.6686398531931,-54.8509327367609,15.2714803633902));
#28968=CARTESIAN_POINT('Origin',(32.5,-56.2916512459885,17.));
#28969=CARTESIAN_POINT('',(31.6657545866042,-54.8497426695209,15.9714803633902));
#28970=CARTESIAN_POINT('',(31.6656238197277,-54.8464558867275,15.7785196366098));
#28971=CARTESIAN_POINT('',(31.667,-54.8488529232837,17.));
#28972=CARTESIAN_POINT('Ctrl Pts',(31.6656238265237,-54.8464558985647,15.7785196366098));
#28973=CARTESIAN_POINT('Ctrl Pts',(32.1435040363299,-54.5705135726953,15.7414495489508));
#28974=CARTESIAN_POINT('Ctrl Pts',(32.7717977196734,-54.5551568083656,15.7043794612919));
#28975=CARTESIAN_POINT('Ctrl Pts',(33.2626292375688,-54.8073433428058,15.667309373633));
#28976=CARTESIAN_POINT('Ctrl Pts',(33.7531413365699,-55.0593657615749,15.6302634101103));
#28977=CARTESIAN_POINT('Ctrl Pts',(34.1063700665184,-55.5785832727215,15.5932174465876));
#28978=CARTESIAN_POINT('Ctrl Pts',(34.1606582960961,-56.1273730385891,15.5561714830649));
#28979=CARTESIAN_POINT('Ctrl Pts',(34.2149465256738,-56.6761628044566,15.5191255195423));
#28980=CARTESIAN_POINT('Ctrl Pts',(33.9702942548808,-57.254524825045,15.4820795560196));
#28981=CARTESIAN_POINT('Ctrl Pts',(33.5386679829465,-57.5977684411295,15.4450335924969));
#28982=CARTESIAN_POINT('Ctrl Pts',(33.1070417110123,-57.941012057214,15.4079876289742));
#28983=CARTESIAN_POINT('Ctrl Pts',(32.4884414379368,-58.0491372687946,15.3709416654515));
#28984=CARTESIAN_POINT('Ctrl Pts',(31.9659730859382,-57.8726599616146,15.3338957019289));
#28985=CARTESIAN_POINT('Ctrl Pts',(31.4435047339395,-57.6961826544346,15.2968497384062));
#28986=CARTESIAN_POINT('Ctrl Pts',(31.0171683030177,-57.235102828494,15.2598037748835));
#28987=CARTESIAN_POINT('Ctrl Pts',(30.8820790791908,-56.7004362767628,15.2227578113608));
#28988=CARTESIAN_POINT('Ctrl Pts',(30.7469898553639,-56.1657697250317,15.1857118478381));
#28989=CARTESIAN_POINT('Ctrl Pts',(30.9031478386319,-55.5575164475099,15.1486658843155));
#28990=CARTESIAN_POINT('Ctrl Pts',(31.2790864406456,-55.1540470134354,15.1116199207928));
#28991=CARTESIAN_POINT('Ctrl Pts',(31.391052526185,-55.0338813988213,15.1005864927318));
#28992=CARTESIAN_POINT('Ctrl Pts',(31.5225138495514,-54.931880760509,15.0895530646708));
#28993=CARTESIAN_POINT('Ctrl Pts',(31.6662678127889,-54.8504473245041,15.0785196366098));
#28994=CARTESIAN_POINT('Ctrl Pts',(31.6686398531931,-54.8509327367609,15.2714803633902));
#28995=CARTESIAN_POINT('Ctrl Pts',(31.4078986168085,-55.0021823003073,15.2915624308993));
#28996=CARTESIAN_POINT('Ctrl Pts',(31.185699780635,-55.2207844238422,15.3116444984084));
#28997=CARTESIAN_POINT('Ctrl Pts',(31.0406952948155,-55.4822046794948,15.3317265659175));
#28998=CARTESIAN_POINT('Ctrl Pts',(30.7732013781725,-55.9644540918428,15.3687725294402));
#28999=CARTESIAN_POINT('Ctrl Pts',(30.7684016474046,-56.5924146126563,15.4058184929629));
#29000=CARTESIAN_POINT('Ctrl Pts',(31.0284927261471,-57.0786965491371,15.4428644564855));
#29001=CARTESIAN_POINT('Ctrl Pts',(31.2885838048897,-57.5649784856179,15.4799104200082));
#29002=CARTESIAN_POINT('Ctrl Pts',(31.8135656931426,-57.9095818377658,15.5169563835309));
#29003=CARTESIAN_POINT('Ctrl Pts',(32.3631774530806,-57.9547969272716,15.5540023470536));
#29004=CARTESIAN_POINT('Ctrl Pts',(32.9127892130185,-58.0000120167774,15.5910483105763));
#29005=CARTESIAN_POINT('Ctrl Pts',(33.4870308446415,-57.7458388436409,15.6280942740989));
#29006=CARTESIAN_POINT('Ctrl Pts',(33.8230974089741,-57.3086012018905,15.6651402376216));
#29007=CARTESIAN_POINT('Ctrl Pts',(34.1591639733067,-56.8713635601401,15.7021862011443));
#29008=CARTESIAN_POINT('Ctrl Pts',(34.2570554703489,-56.2510614497756,15.739232164667));
#29009=CARTESIAN_POINT('Ctrl Pts',(34.0719713014427,-55.7315796489166,15.7762781281897));
#29010=CARTESIAN_POINT('Ctrl Pts',(33.8868871325364,-55.2120978480575,15.8133240917123));
#29011=CARTESIAN_POINT('Ctrl Pts',(33.4188272976816,-54.7934363567037,15.850370055235));
#29012=CARTESIAN_POINT('Ctrl Pts',(32.8820020343565,-54.667197980366,15.8874160187577));
#29013=CARTESIAN_POINT('Ctrl Pts',(32.475949123752,-54.5717116766395,15.9154374669685));
#29014=CARTESIAN_POINT('Ctrl Pts',(32.03055302792,-54.6435311984541,15.9434589151794));
#29015=CARTESIAN_POINT('Ctrl Pts',(31.6657545866042,-54.8497426695209,15.9714803633902));
#29016=CARTESIAN_POINT('Origin',(32.5,-56.2916512459885,17.));
#29017=CARTESIAN_POINT('',(31.6662054032747,-54.8463759356941,16.6714803633902));
#29018=CARTESIAN_POINT('',(31.6687530214682,-54.849035096929,16.4785196366098));
#29019=CARTESIAN_POINT('',(31.667,-54.8488529232837,17.));
#29020=CARTESIAN_POINT('Ctrl Pts',(31.6687530214682,-54.849035096929,16.4785196366098));
#29021=CARTESIAN_POINT('Ctrl Pts',(31.8117829954435,-54.7648928865345,16.4674379602763));
#29022=CARTESIAN_POINT('Ctrl Pts',(31.966578267799,-54.7018565467284,16.4563562839428));
#29023=CARTESIAN_POINT('Ctrl Pts',(32.127375662283,-54.6650214760003,16.4452746076093));
#29024=CARTESIAN_POINT('Ctrl Pts',(32.6649201845491,-54.5418821020028,16.4082286440866));
#29025=CARTESIAN_POINT('Ctrl Pts',(33.2695420256081,-54.7115576426435,16.3711826805639));
#29026=CARTESIAN_POINT('Ctrl Pts',(33.6645325714613,-55.0963951246187,16.3341367170412));
#29027=CARTESIAN_POINT('Ctrl Pts',(34.0595231173144,-55.4812326065939,16.2970907535186));
#29028=CARTESIAN_POINT('Ctrl Pts',(34.2448823679617,-56.0812320299036,16.2600447899959));
#29029=CARTESIAN_POINT('Ctrl Pts',(34.1357796112842,-56.6218002562495,16.2229988264732));
#29030=CARTESIAN_POINT('Ctrl Pts',(34.0266768546067,-57.1623684825954,16.1859528629505));
#29031=CARTESIAN_POINT('Ctrl Pts',(33.6231120906044,-57.6435055119775,16.1489068994278));
#29032=CARTESIAN_POINT('Ctrl Pts',(33.1097790218944,-57.8450162546516,16.1118609359052));
#29033=CARTESIAN_POINT('Ctrl Pts',(32.5964459531844,-58.0465269973256,16.0748149723825));
#29034=CARTESIAN_POINT('Ctrl Pts',(31.9733445797666,-57.9684114532915,16.0377690088598));
#29035=CARTESIAN_POINT('Ctrl Pts',(31.5256407784037,-57.646419644252,16.0007230453371));
#29036=CARTESIAN_POINT('Ctrl Pts',(31.0779369770408,-57.3244278352124,15.9636770818144));
#29037=CARTESIAN_POINT('Ctrl Pts',(30.8056307477328,-56.7585597611673,15.9266311182918));
#29038=CARTESIAN_POINT('Ctrl Pts',(30.833344580418,-56.2077881548333,15.8895851547691));
#29039=CARTESIAN_POINT('Ctrl Pts',(30.8610403660015,-55.6573752080674,15.8525633153826));
#29040=CARTESIAN_POINT('Ctrl Pts',(31.188365597836,-55.1220390739338,15.8155414759962));
#29041=CARTESIAN_POINT('Ctrl Pts',(31.6656238265237,-54.8464558985647,15.7785196366098));
#29042=CARTESIAN_POINT('Ctrl Pts',(31.6657545866042,-54.8497426695209,15.9714803633902));
#29043=CARTESIAN_POINT('Ctrl Pts',(31.5482685418209,-54.9161546038406,15.9805048787021));
#29044=CARTESIAN_POINT('Ctrl Pts',(31.4391421648863,-54.9965058030685,15.9895293940139));
#29045=CARTESIAN_POINT('Ctrl Pts',(31.3423819730146,-55.089696808403,15.9985539093258));
#29046=CARTESIAN_POINT('Ctrl Pts',(30.9451778667933,-55.4722492740994,16.0355998728484));
#29047=CARTESIAN_POINT('Ctrl Pts',(30.756360346146,-56.0711694668139,16.0726458363711));
#29048=CARTESIAN_POINT('Ctrl Pts',(30.8623428200595,-56.6123581642474,16.1096917998938));
#29049=CARTESIAN_POINT('Ctrl Pts',(30.9683252939729,-57.1535468616808,16.1467377634165));
#29050=CARTESIAN_POINT('Ctrl Pts',(31.3691077624471,-57.6370040638332,16.1837837269392));
#29051=CARTESIAN_POINT('Ctrl Pts',(31.8812698561966,-57.8414728407482,16.2208296904618));
#29052=CARTESIAN_POINT('Ctrl Pts',(32.393431949946,-58.0459416176631,16.2578756539845));
#29053=CARTESIAN_POINT('Ctrl Pts',(33.0169736689706,-57.9714219693406,16.2949216175072));
#29054=CARTESIAN_POINT('Ctrl Pts',(33.4665276098354,-57.6520182353919,16.3319675810299));
#29055=CARTESIAN_POINT('Ctrl Pts',(33.9160815507002,-57.3326145014432,16.3690135445526));
#29056=CARTESIAN_POINT('Ctrl Pts',(34.1916477134051,-56.7683266818682,16.4060595080752));
#29057=CARTESIAN_POINT('Ctrl Pts',(34.1671116810225,-56.2174042970244,16.4431054715979));
#29058=CARTESIAN_POINT('Ctrl Pts',(34.14257564864,-55.6664819121806,16.4801514351206));
#29059=CARTESIAN_POINT('Ctrl Pts',(33.8179374211699,-55.128924962068,16.5171973986433));
#29060=CARTESIAN_POINT('Ctrl Pts',(33.3417695242377,-54.8507494330611,16.554243362166));
#29061=CARTESIAN_POINT('Ctrl Pts',(32.8656016273054,-54.5725739040543,16.5912893256886));
#29062=CARTESIAN_POINT('Ctrl Pts',(32.237904060911,-54.5537797961531,16.6283352892113));
#29063=CARTESIAN_POINT('Ctrl Pts',(31.7459461756022,-54.8029683394084,16.665381252734));
#29064=CARTESIAN_POINT('Ctrl Pts',(31.7189481323124,-54.8166434999842,16.6674142896194));
#29065=CARTESIAN_POINT('Ctrl Pts',(31.6923588934129,-54.8311257383684,16.6694473265048));
#29066=CARTESIAN_POINT('Ctrl Pts',(31.6662054032747,-54.8463759356941,16.6714803633902));
#29067=CARTESIAN_POINT('Origin',(32.5,-56.2916512459885,17.));
#29068=CARTESIAN_POINT('',(31.6689051738235,-54.8497998491797,17.3714803633902));
#29069=CARTESIAN_POINT('',(31.6674096068672,-54.8512474102517,17.1785196366098));
#29070=CARTESIAN_POINT('',(31.667,-54.8488529232837,17.));
#29071=CARTESIAN_POINT('Ctrl Pts',(31.6674096068672,-54.8512474102517,17.1785196366098));
#29072=CARTESIAN_POINT('Ctrl Pts',(31.9558120832459,-54.6864945235477,17.156380408079));
#29073=CARTESIAN_POINT('Ctrl Pts',(32.2922890124972,-54.603384940747,17.1342411795483));
#29074=CARTESIAN_POINT('Ctrl Pts',(32.6209875748239,-54.6272788981025,17.1121019510175));
#29075=CARTESIAN_POINT('Ctrl Pts',(33.1710047054117,-54.6672610804705,17.0750559874949));
#29076=CARTESIAN_POINT('Ctrl Pts',(33.6992424692083,-55.0068523416602,17.0380100239722));
#29077=CARTESIAN_POINT('Ctrl Pts',(33.9639498583003,-55.4906368153746,17.0009640604495));
#29078=CARTESIAN_POINT('Ctrl Pts',(34.2286572473923,-55.974421289089,16.9639180969268));
#29079=CARTESIAN_POINT('Ctrl Pts',(34.2298342617796,-56.6023989753281,16.9268721334041));
#29080=CARTESIAN_POINT('Ctrl Pts',(33.9669422341538,-57.087172325109,16.8898261698815));
#29081=CARTESIAN_POINT('Ctrl Pts',(33.704050206528,-57.57194567489,16.8527802063588));
#29082=CARTESIAN_POINT('Ctrl Pts',(33.1770891368891,-57.9135146882128,16.8157342428361));
#29083=CARTESIAN_POINT('Ctrl Pts',(32.6272257468299,-57.955558369302,16.7786882793134));
#29084=CARTESIAN_POINT('Ctrl Pts',(32.0773623567706,-57.9976020503912,16.7416423157907));
#29085=CARTESIAN_POINT('Ctrl Pts',(31.504596646291,-57.7401203992468,16.704596352268));
#29086=CARTESIAN_POINT('Ctrl Pts',(31.1710580905944,-57.3009513535357,16.6675503887454));
#29087=CARTESIAN_POINT('Ctrl Pts',(30.8375195348978,-56.8617823078247,16.6305044252227));
#29088=CARTESIAN_POINT('Ctrl Pts',(30.7432081339843,-56.240925867547,16.5934584617));
#29089=CARTESIAN_POINT('Ctrl Pts',(30.9312860352641,-55.7225205030903,16.5564124981773));
#29090=CARTESIAN_POINT('Ctrl Pts',(31.0631035985939,-55.3591873762591,16.5304482109881));
#29091=CARTESIAN_POINT('Ctrl Pts',(31.333634830935,-55.0461796849558,16.504483923799));
#29092=CARTESIAN_POINT('Ctrl Pts',(31.6687530214682,-54.849035096929,16.4785196366098));
#29093=CARTESIAN_POINT('Ctrl Pts',(31.6662054032747,-54.8463759356941,16.6714803633902));
#29094=CARTESIAN_POINT('Ctrl Pts',(31.215790441256,-55.1090145744741,16.7064932900275));
#29095=CARTESIAN_POINT('Ctrl Pts',(30.894617122853,-55.5994272993444,16.7415062166648));
#29096=CARTESIAN_POINT('Ctrl Pts',(30.84031684399,-56.1177955929609,16.776519143302));
#29097=CARTESIAN_POINT('Ctrl Pts',(30.7828636019098,-56.6662631088463,16.8135651068247));
#29098=CARTESIAN_POINT('Ctrl Pts',(31.0241753219725,-57.2460269462057,16.8506110703474));
#29099=CARTESIAN_POINT('Ctrl Pts',(31.4538143271609,-57.5917548973867,16.8876570338701));
#29100=CARTESIAN_POINT('Ctrl Pts',(31.8834533323493,-57.9374828485678,16.9247029973928));
#29101=CARTESIAN_POINT('Ctrl Pts',(32.5014196226634,-58.0491749135707,16.9617489609154));
#29102=CARTESIAN_POINT('Ctrl Pts',(33.0248974212338,-57.8757145855097,16.9987949244381));
#29103=CARTESIAN_POINT('Ctrl Pts',(33.5483752198042,-57.7022542574486,17.0358408879608));
#29104=CARTESIAN_POINT('Ctrl Pts',(33.9773645266309,-57.2436415363237,17.0728868514835));
#29105=CARTESIAN_POINT('Ctrl Pts',(34.1155359529098,-56.7097631344687,17.1099328150062));
#29106=CARTESIAN_POINT('Ctrl Pts',(34.2537073791887,-56.1758847326138,17.1469787785289));
#29107=CARTESIAN_POINT('Ctrl Pts',(34.1010609249198,-55.5667406500288,17.1840247420515));
#29108=CARTESIAN_POINT('Ctrl Pts',(33.7274561054635,-55.1611091301907,17.2210707055742));
#29109=CARTESIAN_POINT('Ctrl Pts',(33.3538512860073,-54.7554776103525,17.2581166690969));
#29110=CARTESIAN_POINT('Ctrl Pts',(32.7592881013637,-54.5533586532611,17.2951626326196));
#29111=CARTESIAN_POINT('Ctrl Pts',(32.2158717643875,-54.6472531457219,17.3322085961422));
#29112=CARTESIAN_POINT('Ctrl Pts',(32.0238497654509,-54.6804317730554,17.3452991852249));
#29113=CARTESIAN_POINT('Ctrl Pts',(31.8382141569135,-54.7505717682631,17.3583897743076));
#29114=CARTESIAN_POINT('Ctrl Pts',(31.6689051738235,-54.8497998491797,17.3714803633902));
#29115=CARTESIAN_POINT('Origin',(32.5,-56.2916512459885,17.));
#29116=CARTESIAN_POINT('',(31.6668097556407,-54.850936308364,18.0714803633902));
#29117=CARTESIAN_POINT('',(31.6651356431699,-54.8475732381353,17.8785196366098));
#29118=CARTESIAN_POINT('',(31.667,-54.8488529232837,17.));
#29119=CARTESIAN_POINT('Ctrl Pts',(31.6651356431699,-54.8475732381353,17.8785196366098));
#29120=CARTESIAN_POINT('Ctrl Pts',(32.0953114189421,-54.6031821110332,17.8453228558818));
#29121=CARTESIAN_POINT('Ctrl Pts',(32.6432818971092,-54.5571637547426,17.8121260751538));
#29122=CARTESIAN_POINT('Ctrl Pts',(33.1039518347459,-54.7360113496833,17.7789292944258));
#29123=CARTESIAN_POINT('Ctrl Pts',(33.6180366746439,-54.9355964098306,17.7418833309031));
#29124=CARTESIAN_POINT('Ctrl Pts',(34.0234021807399,-55.4152172665964,17.7048373673804));
#29125=CARTESIAN_POINT('Ctrl Pts',(34.1345305305902,-55.9553727152466,17.6677914038577));
#29126=CARTESIAN_POINT('Ctrl Pts',(34.2456588804404,-56.4955281638969,17.6307454403351));
#29127=CARTESIAN_POINT('Ctrl Pts',(34.062550074045,-57.0962182044316,17.5936994768124));
#29128=CARTESIAN_POINT('Ctrl Pts',(33.6690048949483,-57.4825336336559,17.5566535132897));
#29129=CARTESIAN_POINT('Ctrl Pts',(33.2754597158515,-57.8688490628802,17.519607549767));
#29130=CARTESIAN_POINT('Ctrl Pts',(32.6714781640536,-58.0407898807941,17.4825615862443));
#29131=CARTESIAN_POINT('Ctrl Pts',(32.133475821543,-57.9196663971084,17.4455156227217));
#29132=CARTESIAN_POINT('Ctrl Pts',(31.5954734790324,-57.7985429134228,17.408469659199));
#29133=CARTESIAN_POINT('Ctrl Pts',(31.1234503458092,-57.3843551281377,17.3714236956763));
#29134=CARTESIAN_POINT('Ctrl Pts',(30.9334304853463,-56.8666584297933,17.3343777321536));
#29135=CARTESIAN_POINT('Ctrl Pts',(30.7434106248833,-56.348961731449,17.2973317686309));
#29136=CARTESIAN_POINT('Ctrl Pts',(30.8353940371805,-55.7277561200454,17.2602858051083));
#29137=CARTESIAN_POINT('Ctrl Pts',(31.1672839920187,-55.2873398661168,17.2232398415856));
#29138=CARTESIAN_POINT('Ctrl Pts',(31.3008314863423,-55.1101230316988,17.2083331065936));
#29139=CARTESIAN_POINT('Ctrl Pts',(31.4732231075307,-54.9621784491468,17.1934263716017));
#29140=CARTESIAN_POINT('Ctrl Pts',(31.6674096068672,-54.8512474102517,17.1785196366098));
#29141=CARTESIAN_POINT('Ctrl Pts',(31.6689051738235,-54.8497998491797,17.3714803633902));
#29142=CARTESIAN_POINT('Ctrl Pts',(31.3590749545435,-55.0313841780677,17.3954357378302));
#29143=CARTESIAN_POINT('Ctrl Pts',(31.1039191289866,-55.3103783149914,17.4193911122703));
#29144=CARTESIAN_POINT('Ctrl Pts',(30.9643532196009,-55.6385333911701,17.4433464867103));
#29145=CARTESIAN_POINT('Ctrl Pts',(30.7485205010994,-56.1460112021445,17.480392450233));
#29146=CARTESIAN_POINT('Ctrl Pts',(30.8091245534053,-56.7710588820805,17.5174384137557));
#29147=CARTESIAN_POINT('Ctrl Pts',(31.1184295883325,-57.2276198159938,17.5544843772783));
#29148=CARTESIAN_POINT('Ctrl Pts',(31.4277346232597,-57.6841807499072,17.591530340801));
#29149=CARTESIAN_POINT('Ctrl Pts',(31.9857406408081,-57.9722549377979,17.6285763043237));
#29150=CARTESIAN_POINT('Ctrl Pts',(32.5370730229374,-57.9600035940862,17.6656222678464));
#29151=CARTESIAN_POINT('Ctrl Pts',(33.0884054050668,-57.9477522503744,17.7026682313691));
#29152=CARTESIAN_POINT('Ctrl Pts',(33.633064151777,-57.6351753750602,17.7397141948917));
#29153=CARTESIAN_POINT('Ctrl Pts',(33.921783099211,-57.1653255475623,17.7767601584144));
#29154=CARTESIAN_POINT('Ctrl Pts',(34.2105020466451,-56.6954757200645,17.8138061219371));
#29155=CARTESIAN_POINT('Ctrl Pts',(34.2432811948029,-56.0683529403831,17.8508520854598));
#29156=CARTESIAN_POINT('Ctrl Pts',(34.0051189806597,-55.5709635046674,17.8878980489825));
#29157=CARTESIAN_POINT('Ctrl Pts',(33.7669567665165,-55.0735740689518,17.9249440125051));
#29158=CARTESIAN_POINT('Ctrl Pts',(33.2578531900722,-54.7059179772018,17.9619899760278));
#29159=CARTESIAN_POINT('Ctrl Pts',(32.7108023899003,-54.6362551245587,17.9990359395505));
#29160=CARTESIAN_POINT('Ctrl Pts',(32.3542113134731,-54.5908459018628,18.0231840808304));
#29161=CARTESIAN_POINT('Ctrl Pts',(31.9814965026905,-54.6720536844457,18.0473322221103));
#29162=CARTESIAN_POINT('Ctrl Pts',(31.6668097556407,-54.850936308364,18.0714803633902));
#29163=CARTESIAN_POINT('Origin',(32.5,-56.2916512459885,17.));
#29164=CARTESIAN_POINT('',(31.6652761166364,-54.8468682178695,18.7714803633902));
#29165=CARTESIAN_POINT('',(31.6679260143736,-54.8475393267799,18.5785196366098));
#29166=CARTESIAN_POINT('',(31.667,-54.8488529232837,17.));
#29167=CARTESIAN_POINT('Ctrl Pts',(31.6679260143736,-54.8475393267799,18.5785196366098));
#29168=CARTESIAN_POINT('Ctrl Pts',(31.7606663811943,-54.7928563701909,18.5713112672072));
#29169=CARTESIAN_POINT('Ctrl Pts',(31.8585183363754,-54.7473751127228,18.5641028978046));
#29170=CARTESIAN_POINT('Ctrl Pts',(31.9600503104883,-54.7126554770058,18.5568945284021));
#29171=CARTESIAN_POINT('Ctrl Pts',(32.4818534533783,-54.5342208981906,18.5198485648794));
#29172=CARTESIAN_POINT('Ctrl Pts',(33.1008546957744,-54.6400264825866,18.4828026013567));
#29173=CARTESIAN_POINT('Ctrl Pts',(33.533764609118,-54.9816497045372,18.445756637834));
#29174=CARTESIAN_POINT('Ctrl Pts',(33.9666745224615,-55.3232729264878,18.4087106743114));
#29175=CARTESIAN_POINT('Ctrl Pts',(34.2134931067525,-55.9007137859928,18.3716647107887));
#29176=CARTESIAN_POINT('Ctrl Pts',(34.1612624373338,-56.4497031993872,18.334618747266));
#29177=CARTESIAN_POINT('Ctrl Pts',(34.109031767915,-56.9986926127816,18.2975727837433));
#29178=CARTESIAN_POINT('Ctrl Pts',(33.7577518447865,-57.5192305800653,18.2605268202206));
#29179=CARTESIAN_POINT('Ctrl Pts',(33.2681879166606,-57.7730899488602,18.223480856698));
#29180=CARTESIAN_POINT('Ctrl Pts',(32.7786239885346,-58.026949317655,18.1864348931753));
#29181=CARTESIAN_POINT('Ctrl Pts',(32.1507760554113,-58.0141300879609,18.1493889296526));
#29182=CARTESIAN_POINT('Ctrl Pts',(31.6719822840244,-57.7404990529372,18.1123429661299));
#29183=CARTESIAN_POINT('Ctrl Pts',(31.1931885126375,-57.4668680179136,18.0752970026072));
#29184=CARTESIAN_POINT('Ctrl Pts',(30.863448902987,-56.9324251775604,18.0382510390845));
#29185=CARTESIAN_POINT('Ctrl Pts',(30.8336706571802,-56.3817613282625,18.0012050755619));
#29186=CARTESIAN_POINT('Ctrl Pts',(30.8038924113734,-55.8310974789645,17.9641591120392));
#29187=CARTESIAN_POINT('Ctrl Pts',(31.0740755294104,-55.2642126207216,17.9271131485165));
#29188=CARTESIAN_POINT('Ctrl Pts',(31.520569175279,-54.9405448233645,17.8900671849938));
#29189=CARTESIAN_POINT('Ctrl Pts',(31.5669611569199,-54.9069148027547,17.8862180021991));
#29190=CARTESIAN_POINT('Ctrl Pts',(31.6152565537377,-54.875910507623,17.8823688194045));
#29191=CARTESIAN_POINT('Ctrl Pts',(31.6651356431699,-54.8475732381353,17.8785196366098));
#29192=CARTESIAN_POINT('Ctrl Pts',(31.6668097556407,-54.850936308364,18.0714803633902));
#29193=CARTESIAN_POINT('Ctrl Pts',(31.4987316547814,-54.9464797400044,18.084378185633));
#29194=CARTESIAN_POINT('Ctrl Pts',(31.3472075724787,-55.0698874675039,18.0972760078758));
#29195=CARTESIAN_POINT('Ctrl Pts',(31.2235359810034,-55.2167495878635,18.1101738301185));
#29196=CARTESIAN_POINT('Ctrl Pts',(30.8683183961781,-55.6385765173477,18.1472197936412));
#29197=CARTESIAN_POINT('Ctrl Pts',(30.7428812504271,-56.2538999898523,18.1842657571639));
#29198=CARTESIAN_POINT('Ctrl Pts',(30.9046315647805,-56.7811137290641,18.2213117206866));
#29199=CARTESIAN_POINT('Ctrl Pts',(31.066381879134,-57.3083274682759,18.2583576842093));
#29200=CARTESIAN_POINT('Ctrl Pts',(31.5153196535918,-57.7474314741949,18.2954036477319));
#29201=CARTESIAN_POINT('Ctrl Pts',(32.0459859700228,-57.8974673086234,18.3324496112546));
#29202=CARTESIAN_POINT('Ctrl Pts',(32.5766522864537,-58.0475031430519,18.3694955747773));
#29203=CARTESIAN_POINT('Ctrl Pts',(33.1890471448577,-57.9084708059901,18.4065415383));
#29204=CARTESIAN_POINT('Ctrl Pts',(33.602904565772,-57.5439992348605,18.4435875018227));
#29205=CARTESIAN_POINT('Ctrl Pts',(34.0167619866863,-57.179527663731,18.4806334653453));
#29206=CARTESIAN_POINT('Ctrl Pts',(34.2320819701108,-56.5896168585339,18.517679428868));
#29207=CARTESIAN_POINT('Ctrl Pts',(34.1503221046824,-56.0442428442904,18.5547253923907));
#29208=CARTESIAN_POINT('Ctrl Pts',(34.068562239254,-55.4988688300469,18.5917713559134));
#29209=CARTESIAN_POINT('Ctrl Pts',(33.6897225249727,-54.9980316067572,18.6288173194361));
#29210=CARTESIAN_POINT('Ctrl Pts',(33.1871811052497,-54.7709421695978,18.6658632829587));
#29211=CARTESIAN_POINT('Ctrl Pts',(32.7096035907249,-54.5551334726087,18.7010689764359));
#29212=CARTESIAN_POINT('Ctrl Pts',(32.1203089631069,-54.5865510549417,18.7362746699131));
#29213=CARTESIAN_POINT('Ctrl Pts',(31.6652761166364,-54.8468682178695,18.7714803633902));
#29214=CARTESIAN_POINT('Origin',(32.5,-56.2916512459885,17.));
#29215=CARTESIAN_POINT('',(31.6684351372492,-54.8482948457192,19.4714803633902));
#29216=CARTESIAN_POINT('',(31.6684043758654,-54.8511587229547,19.2785196366098));
#29217=CARTESIAN_POINT('',(31.667,-54.8488529232837,17.));
#29218=CARTESIAN_POINT('Ctrl Pts',(31.6684043758654,-54.8511587229547,19.2785196366098));
#29219=CARTESIAN_POINT('Ctrl Pts',(31.9058262033729,-54.7139758182214,19.26025371501));
#29220=CARTESIAN_POINT('Ctrl Pts',(32.1752796610303,-54.6323550853735,19.2419877934101));
#29221=CARTESIAN_POINT('Ctrl Pts',(32.4470503478135,-54.6237274947409,19.2237218718103));
#29222=CARTESIAN_POINT('Ctrl Pts',(32.9982410936013,-54.6062294776757,19.1866759082876));
#29223=CARTESIAN_POINT('Ctrl Pts',(33.5589634784782,-54.8889798390775,19.149629944765));
#29224=CARTESIAN_POINT('Ctrl Pts',(33.8725997234821,-55.3425762727762,19.1125839812423));
#29225=CARTESIAN_POINT('Ctrl Pts',(34.186235968486,-55.7961727064748,19.0755380177196));
#29226=CARTESIAN_POINT('Ctrl Pts',(34.252786073617,-56.4206152124703,19.0384920541969));
#29227=CARTESIAN_POINT('Ctrl Pts',(34.0417930059025,-56.9301241370495,19.0014460906742));
#29228=CARTESIAN_POINT('Ctrl Pts',(33.830799938188,-57.4396330616287,18.9644001271515));
#29229=CARTESIAN_POINT('Ctrl Pts',(33.342263697628,-57.8342084047915,18.9273541636289));
#29230=CARTESIAN_POINT('Ctrl Pts',(32.7997656649011,-57.9332705233524,18.8903082001062));
#29231=CARTESIAN_POINT('Ctrl Pts',(32.2572676321741,-58.0323326419133,18.8532622365835));
#29232=CARTESIAN_POINT('Ctrl Pts',(31.6608078072801,-57.8358815358723,18.8162162730608));
#29233=CARTESIAN_POINT('Ctrl Pts',(31.2833594112405,-57.433824167859,18.7791703095382));
#29234=CARTESIAN_POINT('Ctrl Pts',(30.9059110152008,-57.0317667998456,18.7421243460155));
#29235=CARTESIAN_POINT('Ctrl Pts',(30.7474740480154,-56.4241031698599,18.7050783824928));
#29236=CARTESIAN_POINT('Ctrl Pts',(30.8805580861148,-55.8889339838537,18.6680324189701));
#29237=CARTESIAN_POINT('Ctrl Pts',(30.987746754868,-55.4578975242981,18.63819482485));
#29238=CARTESIAN_POINT('Ctrl Pts',(31.2840459342598,-55.0738884180753,18.6083572307299));
#29239=CARTESIAN_POINT('Ctrl Pts',(31.6679260143736,-54.8475393267799,18.5785196366098));
#29240=CARTESIAN_POINT('Ctrl Pts',(31.6652761166364,-54.8468682178695,18.7714803633902));
#29241=CARTESIAN_POINT('Ctrl Pts',(31.6414906650692,-54.8604755020886,18.7733206334357));
#29242=CARTESIAN_POINT('Ctrl Pts',(31.6180720645057,-54.8747082214849,18.7751609034813));
#29243=CARTESIAN_POINT('Ctrl Pts',(31.5950554470213,-54.8895637585373,18.7770011735268));
#29244=CARTESIAN_POINT('Ctrl Pts',(31.1317143336804,-55.1886164356655,18.8140471370495));
#29245=CARTESIAN_POINT('Ctrl Pts',(30.8312752321632,-55.740063440951,18.8510931005722));
#29246=CARTESIAN_POINT('Ctrl Pts',(30.8312358008972,-56.2915319254989,18.8881390640948));
#29247=CARTESIAN_POINT('Ctrl Pts',(30.8311963696312,-56.8430004100469,18.9251850276175));
#29248=CARTESIAN_POINT('Ctrl Pts',(31.1315566086164,-57.3944903738573,18.9622309911402));
#29249=CARTESIAN_POINT('Ctrl Pts',(31.5948549512976,-57.6936093078491,18.9992769546629));
#29250=CARTESIAN_POINT('Ctrl Pts',(32.0581532939788,-57.9927282418409,19.0363229181856));
#29251=CARTESIAN_POINT('Ctrl Pts',(32.684389740356,-58.0394761460141,19.0733688817082));
#29252=CARTESIAN_POINT('Ctrl Pts',(33.186963629793,-57.81245857691,19.1104148452309));
#29253=CARTESIAN_POINT('Ctrl Pts',(33.6895375192301,-57.585441007806,19.1474608087536));
#29254=CARTESIAN_POINT('Ctrl Pts',(34.068448851727,-57.0846579654248,19.1845067722763));
#29255=CARTESIAN_POINT('Ctrl Pts',(34.150286707292,-56.5392956488153,19.221552735799));
#29256=CARTESIAN_POINT('Ctrl Pts',(34.2321245628569,-55.9939333322058,19.2585986993216));
#29257=CARTESIAN_POINT('Ctrl Pts',(34.01688894149,-55.4039917413682,19.2956446628443));
#29258=CARTESIAN_POINT('Ctrl Pts',(33.6030836459812,-55.0394609904048,19.332690626367));
#29259=CARTESIAN_POINT('Ctrl Pts',(33.1892783504724,-54.6749302394416,19.3697365898897));
#29260=CARTESIAN_POINT('Ctrl Pts',(32.5769033808219,-54.5358103283526,19.4067825534124));
#29261=CARTESIAN_POINT('Ctrl Pts',(32.0462156138869,-54.685770273593,19.443828516935));
#29262=CARTESIAN_POINT('Ctrl Pts',(31.9141769673738,-54.7230813054923,19.4530457990868));
#29263=CARTESIAN_POINT('Ctrl Pts',(31.7871951467268,-54.7782877536412,19.4622630812385));
#29264=CARTESIAN_POINT('Ctrl Pts',(31.6684351372492,-54.8482948457192,19.4714803633902));
#29265=CARTESIAN_POINT('Origin',(32.5,-56.2916512459885,17.));
#29266=CARTESIAN_POINT('',(31.667931072794,-54.8513178316736,20.1714803633902));
#29267=CARTESIAN_POINT('',(31.6654871359731,-54.8492158242279,19.9785196366098));
#29268=CARTESIAN_POINT('',(31.667,-54.8488529232837,17.));
#29269=CARTESIAN_POINT('Ctrl Pts',(31.6654871359731,-54.8492158242279,19.9785196366098));
#29270=CARTESIAN_POINT('Ctrl Pts',(32.0469172461538,-54.6336656790849,19.9491961628127));
#29271=CARTESIAN_POINT('Ctrl Pts',(32.517553856985,-54.5668303852667,19.9198726890156));
#29272=CARTESIAN_POINT('Ctrl Pts',(32.9387102808402,-54.6815870878529,19.8905492152186));
#29273=CARTESIAN_POINT('Ctrl Pts',(33.4707804449503,-54.8265655664402,19.8535032516959));
#29274=CARTESIAN_POINT('Ctrl Pts',(33.9238769452872,-55.2613769285398,19.8164572881732));
#29275=CARTESIAN_POINT('Ctrl Pts',(34.0906375985398,-55.7870272905994,19.7794113246505));
#29276=CARTESIAN_POINT('Ctrl Pts',(34.2573982517924,-56.312677652659,19.7423653611279));
#29277=CARTESIAN_POINT('Ctrl Pts',(34.1378230579607,-56.9291670146787,19.7053193976052));
#29278=CARTESIAN_POINT('Ctrl Pts',(33.786636282889,-57.3543555234679,19.6682734340825));
#29279=CARTESIAN_POINT('Ctrl Pts',(33.4354495078173,-57.779544032257,19.6312274705598));
#29280=CARTESIAN_POINT('Ctrl Pts',(32.8526511515056,-58.0134316878157,19.5941815070371));
#29281=CARTESIAN_POINT('Ctrl Pts',(32.3049621862366,-57.9489784788088,19.5571355435145));
#29282=CARTESIAN_POINT('Ctrl Pts',(31.7572732209677,-57.884525269802,19.5200895799918));
#29283=CARTESIAN_POINT('Ctrl Pts',(31.2446936467415,-57.5217311962297,19.4830436164691));
#29284=CARTESIAN_POINT('Ctrl Pts',(31.0018084123138,-57.0266310228124,19.4459976529464));
#29285=CARTESIAN_POINT('Ctrl Pts',(30.7589231778862,-56.531530849395,19.4089516894237));
#29286=CARTESIAN_POINT('Ctrl Pts',(30.7857322832571,-55.9041245761327,19.3719057259011));
#29287=CARTESIAN_POINT('Ctrl Pts',(31.0699663892919,-55.4315482417354,19.3348597623784));
#29288=CARTESIAN_POINT('Ctrl Pts',(31.214055729119,-55.1919808900508,19.3160797204555));
#29289=CARTESIAN_POINT('Ctrl Pts',(31.4242999735977,-54.9922028355067,19.2972996785326));
#29290=CARTESIAN_POINT('Ctrl Pts',(31.6684043758654,-54.8511587229547,19.2785196366098));
#29291=CARTESIAN_POINT('Ctrl Pts',(31.6684351372492,-54.8482948457192,19.4714803633902));
#29292=CARTESIAN_POINT('Ctrl Pts',(31.3098766805411,-55.0596592183269,19.4993090447612));
#29293=CARTESIAN_POINT('Ctrl Pts',(31.0262639705086,-55.405938549172,19.5271377261321));
#29294=CARTESIAN_POINT('Ctrl Pts',(30.9047015762615,-55.801960623025,19.5549664075031));
#29295=CARTESIAN_POINT('Ctrl Pts',(30.7428758697907,-56.3291512256471,19.5920123710258));
#29296=CARTESIAN_POINT('Ctrl Pts',(30.8682250210686,-56.9444926293215,19.6290583345485));
#29297=CARTESIAN_POINT('Ctrl Pts',(31.2233822786099,-57.3663703525617,19.6661042980711));
#29298=CARTESIAN_POINT('Ctrl Pts',(31.5785395361512,-57.7882480758019,19.7031502615938));
#29299=CARTESIAN_POINT('Ctrl Pts',(32.1635048999558,-58.0166621186079,19.7401962251165));
#29300=CARTESIAN_POINT('Ctrl Pts',(32.7105656575522,-57.9470774968357,19.7772421886392));
#29301=CARTESIAN_POINT('Ctrl Pts',(33.2576264151486,-57.8774928750636,19.8142881521619));
#29302=CARTESIAN_POINT('Ctrl Pts',(33.7667825665369,-57.5099095887134,19.8513341156845));
#29303=CARTESIAN_POINT('Ctrl Pts',(34.0050159054109,-57.0125542176421,19.8883800792072));
#29304=CARTESIAN_POINT('Ctrl Pts',(34.243249244285,-56.5151988465708,19.9254260427299));
#29305=CARTESIAN_POINT('Ctrl Pts',(34.2105597706447,-55.8880713907783,19.9624720062526));
#29306=CARTESIAN_POINT('Ctrl Pts',(33.9219080204981,-55.4181802774153,19.9995179697753));
#29307=CARTESIAN_POINT('Ctrl Pts',(33.6332562703514,-54.9482891640523,20.0365639332979));
#29308=CARTESIAN_POINT('Ctrl Pts',(33.0886422436983,-54.6356343931188,20.0736098968206));
#29309=CARTESIAN_POINT('Ctrl Pts',(32.5373116119164,-54.6233042115161,20.1106558603433));
#29310=CARTESIAN_POINT('Ctrl Pts',(32.235574629855,-54.6165560434104,20.1309306946923));
#29311=CARTESIAN_POINT('Ctrl Pts',(31.9318258577411,-54.6997625487969,20.1512055290412));
#29312=CARTESIAN_POINT('Ctrl Pts',(31.667931072794,-54.8513178316736,20.1714803633902));
#29313=CARTESIAN_POINT('Origin',(32.5,-56.2916512459885,17.));
#29314=CARTESIAN_POINT('',(31.6652099567911,-54.8483531313949,20.8714803633902));
#29315=CARTESIAN_POINT('',(31.6666453776089,-54.8465106722,20.6785196366098));
#29316=CARTESIAN_POINT('',(31.667,-54.8488529232837,17.));
#29317=CARTESIAN_POINT('Ctrl Pts',(31.6666453776089,-54.8465106722,20.6785196366098));
#29318=CARTESIAN_POINT('Ctrl Pts',(31.7095215140163,-54.8213939588907,20.6751845741381));
#29319=CARTESIAN_POINT('Ctrl Pts',(31.7535458686671,-54.7983179269086,20.6718495116665));
#29320=CARTESIAN_POINT('Ctrl Pts',(31.7985935167041,-54.7774509892024,20.6685144491949));
#29321=CARTESIAN_POINT('Ctrl Pts',(32.2989840011863,-54.5456604846271,20.6314684856722));
#29322=CARTESIAN_POINT('Ctrl Pts',(32.9256368768596,-54.5864462806581,20.5944225221495));
#29323=CARTESIAN_POINT('Ctrl Pts',(33.3917609918081,-54.881142287214,20.5573765586268));
#29324=CARTESIAN_POINT('Ctrl Pts',(33.8578851067565,-55.1758382937699,20.5203305951041));
#29325=CARTESIAN_POINT('Ctrl Pts',(34.16348046098,-55.7244445108506,20.4832846315815));
#29326=CARTESIAN_POINT('Ctrl Pts',(34.1686895628039,-56.2758883119516,20.4462386680588));
#29327=CARTESIAN_POINT('Ctrl Pts',(34.1738986646279,-56.8273321130526,20.4091927045361));
#29328=CARTESIAN_POINT('Ctrl Pts',(33.8787215140524,-57.3816134981739,20.3721467410134));
#29329=CARTESIAN_POINT('Ctrl Pts',(33.4182476302774,-57.6850623886885,20.3351007774907));
#29330=CARTESIAN_POINT('Ctrl Pts',(32.9577737465024,-57.988511279203,20.2980548139681));
#29331=CARTESIAN_POINT('Ctrl Pts',(32.3320031295279,-58.0411276751107,20.2610088504454));
#29332=CARTESIAN_POINT('Ctrl Pts',(31.8273232393449,-57.8188314143185,20.2239628869227));
#29333=CARTESIAN_POINT('Ctrl Pts',(31.3226433491619,-57.5965351535263,20.1869169234));
#29334=CARTESIAN_POINT('Ctrl Pts',(30.9390541857702,-57.0993262360342,20.1498709598773));
#29335=CARTESIAN_POINT('Ctrl Pts',(30.8521075105052,-56.5547551273837,20.1128249963547));
#29336=CARTESIAN_POINT('Ctrl Pts',(30.7651608352402,-56.0101840187332,20.075779032832));
#29337=CARTESIAN_POINT('Ctrl Pts',(30.9748566481017,-55.4182507189243,20.0387330693093));
#29338=CARTESIAN_POINT('Ctrl Pts',(31.3852264684742,-55.0498568665574,20.0016871057866));
#29339=CARTESIAN_POINT('Ctrl Pts',(31.4707709224493,-54.9730625961603,19.993964616061));
#29340=CARTESIAN_POINT('Ctrl Pts',(31.565035527569,-54.9059820788928,19.9862421263354));
#29341=CARTESIAN_POINT('Ctrl Pts',(31.6654871359731,-54.8492158242279,19.9785196366098));
#29342=CARTESIAN_POINT('Ctrl Pts',(31.667931072794,-54.8513178316736,20.1714803633902));
#29343=CARTESIAN_POINT('Ctrl Pts',(31.4496400894775,-54.9766827635065,20.1882514925639));
#29344=CARTESIAN_POINT('Ctrl Pts',(31.2586188937636,-55.1488148264988,20.2050226217376));
#29345=CARTESIAN_POINT('Ctrl Pts',(31.1185634357287,-55.3554851247115,20.2217937509113));
#29346=CARTESIAN_POINT('Ctrl Pts',(30.8091931282335,-55.8120018117817,20.258839714434));
#29347=CARTESIAN_POINT('Ctrl Pts',(30.7484997501537,-56.4370407781941,20.2958856779567));
#29348=CARTESIAN_POINT('Ctrl Pts',(30.9642598655731,-56.9445494693264,20.3329316414794));
#29349=CARTESIAN_POINT('Ctrl Pts',(31.1800199809926,-57.4520581604587,20.3699776050021));
#29350=CARTESIAN_POINT('Ctrl Pts',(31.6722335899113,-57.842036576311,20.4070235685247));
#29351=CARTESIAN_POINT('Ctrl Pts',(32.2156365524479,-57.9360087382767,20.4440695320474));
#29352=CARTESIAN_POINT('Ctrl Pts',(32.7590395149845,-58.0299809002424,20.4811154955701));
#29353=CARTESIAN_POINT('Ctrl Pts',(33.353631831139,-57.8279468083216,20.5181614590928));
#29354=CARTESIAN_POINT('Ctrl Pts',(33.727294536927,-57.4223688010744,20.5552074226155));
#29355=CARTESIAN_POINT('Ctrl Pts',(34.1009572427151,-57.0167907938273,20.5922533861381));
#29356=CARTESIAN_POINT('Ctrl Pts',(34.2536903381367,-56.4076688712538,20.6292993496608));
#29357=CARTESIAN_POINT('Ctrl Pts',(34.1155954946061,-55.8737705531045,20.6663453131835));
#29358=CARTESIAN_POINT('Ctrl Pts',(33.9775006510756,-55.3398722349553,20.7033912767062));
#29359=CARTESIAN_POINT('Ctrl Pts',(33.5485778685929,-54.8811975212302,20.7404372402289));
#29360=CARTESIAN_POINT('Ctrl Pts',(33.0251244120732,-54.707662660689,20.7774832037515));
#29361=CARTESIAN_POINT('Ctrl Pts',(32.5824028716121,-54.560891978739,20.8088155902978));
#29362=CARTESIAN_POINT('Ctrl Pts',(32.0720609029457,-54.6180897881502,20.840147976844));
#29363=CARTESIAN_POINT('Ctrl Pts',(31.6652099567911,-54.8483531313949,20.8714803633902));
#29364=CARTESIAN_POINT('Origin',(32.5,-56.2916512459885,17.));
#29365=CARTESIAN_POINT('',(31.6673136634551,-54.8469650373412,21.5714803633902));
#29366=CARTESIAN_POINT('',(31.6688940285232,-54.8502492137287,21.3785196366098));
#29367=CARTESIAN_POINT('',(31.667,-54.8488529232837,17.));
#29368=CARTESIAN_POINT('',(34.0692874532607,-56.8510195406194,22.));
#29369=CARTESIAN_POINT('Ctrl Pts',(31.6673136634551,-54.8469650373412,21.5714803633902));
#29370=CARTESIAN_POINT('Ctrl Pts',(31.2598491701086,-55.0867590255674,21.6031823516921));
#29371=CARTESIAN_POINT('Ctrl Pts',(30.9533734485754,-55.5074467114501,21.634884339994));
#29372=CARTESIAN_POINT('Ctrl Pts',(30.8625080737328,-55.9706266060895,21.6665863282959));
#29373=CARTESIAN_POINT('Ctrl Pts',(30.7563256056225,-56.5118843126361,21.7036322918186));
#29374=CARTESIAN_POINT('Ctrl Pts',(30.9445706465322,-57.1111674125324,21.7406782553412));
#29375=CARTESIAN_POINT('Ctrl Pts',(31.341982566131,-57.4936046161573,21.7777242188639));
#29376=CARTESIAN_POINT('Ctrl Pts',(31.7393944857297,-57.8760418197823,21.8147701823866));
#29377=CARTESIAN_POINT('Ctrl Pts',(32.3459732840176,-58.0416331271359,21.8518161459093));
#29378=CARTESIAN_POINT('Ctrl Pts',(32.8819457094271,-57.9158339106247,21.888862109432));
#29379=CARTESIAN_POINT('Ctrl Pts',(33.4179181348367,-57.7900346941135,21.9259080729546));
#29380=CARTESIAN_POINT('Ctrl Pts',(33.8832841873681,-57.3728449537375,21.9629540364773));
#29381=CARTESIAN_POINT('Ctrl Pts',(34.0692874532607,-56.8510195406194,22.));
#29382=CARTESIAN_POINT('',(32.8006122403835,-54.6499198220901,22.));
#29383=CARTESIAN_POINT('Origin',(32.5,-56.2916512459885,22.));
#29384=CARTESIAN_POINT('Ctrl Pts',(32.8006124898337,-54.6499179279034,22.));
#29385=CARTESIAN_POINT('Ctrl Pts',(33.3324299245223,-54.7480089912901,21.9636770818144));
#29386=CARTESIAN_POINT('Ctrl Pts',(33.8131824856955,-55.1285995043638,21.9273541636289));
#29387=CARTESIAN_POINT('Ctrl Pts',(34.0294057231265,-55.6243031692819,21.8910312454433));
#29388=CARTESIAN_POINT('Ctrl Pts',(34.2499331082255,-56.1298743294735,21.8539852819206));
#29389=CARTESIAN_POINT('Ctrl Pts',(34.195294888985,-56.7551871483463,21.816939318398));
#29390=CARTESIAN_POINT('Ctrl Pts',(33.8903094432865,-57.2145585578539,21.7798933548753));
#29391=CARTESIAN_POINT('Ctrl Pts',(33.585323997588,-57.6739299673615,21.7428473913526));
#29392=CARTESIAN_POINT('Ctrl Pts',(33.0299913254315,-57.9673599675038,21.7058014278299));
#29393=CARTESIAN_POINT('Ctrl Pts',(32.4785554363758,-57.9603119672567,21.6687554643073));
#29394=CARTESIAN_POINT('Ctrl Pts',(31.9271195473201,-57.9532639670095,21.6317095007846));
#29395=CARTESIAN_POINT('Ctrl Pts',(31.3795804413652,-57.6457379663728,21.5946635372619));
#29396=CARTESIAN_POINT('Ctrl Pts',(31.0864761391558,-57.1785982034714,21.5576175737392));
#29397=CARTESIAN_POINT('Ctrl Pts',(30.7933718369463,-56.7114584405699,21.5205716102165));
#29398=CARTESIAN_POINT('Ctrl Pts',(30.7547023384823,-56.0847049154036,21.4835256466938));
#29399=CARTESIAN_POINT('Ctrl Pts',(30.9881881185804,-55.5851133656589,21.4464796831712));
#29400=CARTESIAN_POINT('Ctrl Pts',(31.1309630480468,-55.2796166101529,21.4238263343174));
#29401=CARTESIAN_POINT('Ctrl Pts',(31.3755032965772,-55.0216687358223,21.4011729854636));
#29402=CARTESIAN_POINT('Ctrl Pts',(31.6688940285232,-54.8502492137287,21.3785196366098));
#29403=CARTESIAN_POINT('Origin',(32.5,-56.2916512459885,23.5459252805377));
#29404=CARTESIAN_POINT('',(31.4724222119036,-54.5094432564574,13.4540747194623));
#29405=CARTESIAN_POINT('',(31.4735006561133,-54.5153050203084,13.3959252805377));
#29406=CARTESIAN_POINT('',(31.4726250000001,-54.5121855475624,23.5459252805377));
#29407=CARTESIAN_POINT('',(32.7283737736498,-58.3336705852723,13.));
#29408=CARTESIAN_POINT('Ctrl Pts',(31.4735006561133,-54.5153050203084,13.3959252805377));
#29409=CARTESIAN_POINT('Ctrl Pts',(31.808029474343,-54.3235252303773,13.3750880775931));
#29410=CARTESIAN_POINT('Ctrl Pts',(32.8820600904465,-54.0381232256079,13.3172049111259));
#29411=CARTESIAN_POINT('Ctrl Pts',(34.5894859509232,-55.0509345423224,13.2222757811361));
#29412=CARTESIAN_POINT('Ctrl Pts',(34.6719801790384,-57.3759588223509,13.111137890568));
#29413=CARTESIAN_POINT('Ctrl Pts',(33.4073937856322,-58.2577308722946,13.0370459635227));
#29414=CARTESIAN_POINT('Ctrl Pts',(32.7283737736498,-58.3336705852723,13.));
#29415=CARTESIAN_POINT('',(31.6782144221994,-58.178982708051,13.));
#29416=CARTESIAN_POINT('Origin',(32.5,-56.2916512459885,13.));
#29417=CARTESIAN_POINT('Ctrl Pts',(31.4724222119036,-54.5094432564574,13.4540747194623));
#29418=CARTESIAN_POINT('Ctrl Pts',(31.5342132308562,-54.4731877432048,13.4501772883951));
#29419=CARTESIAN_POINT('Ctrl Pts',(32.2034917270506,-54.1282244537509,13.4092338938053));
#29420=CARTESIAN_POINT('Ctrl Pts',(33.8288126996591,-54.2585627611561,13.3312445356927));
#29421=CARTESIAN_POINT('Ctrl Pts',(34.9285321027134,-56.3058411531895,13.2201066451247));
#29422=CARTESIAN_POINT('Ctrl Pts',(33.8129922329338,-58.325638659776,13.1096917998938));
#29423=CARTESIAN_POINT('Ctrl Pts',(32.2900793461072,-58.4444630460461,13.0363229181856));
#29424=CARTESIAN_POINT('Ctrl Pts',(31.6782133743559,-58.1789848186021,13.));
#29425=CARTESIAN_POINT('Origin',(32.5,-56.2916512459885,23.5459252805377));
#29426=CARTESIAN_POINT('',(31.4749259905951,-54.514117897405,14.1540747194623));
#29427=CARTESIAN_POINT('',(31.470366790827,-54.5112698283738,14.0959252805377));
#29428=CARTESIAN_POINT('',(31.4726250000001,-54.5121855475624,23.5459252805377));
#29429=CARTESIAN_POINT('Ctrl Pts',(31.470366790827,-54.5112698283738,14.0959252805377));
#29430=CARTESIAN_POINT('Ctrl Pts',(31.9808629913117,-54.2220900136561,14.0640305253959));
#29431=CARTESIAN_POINT('Ctrl Pts',(33.3714175837229,-54.0779847124815,13.9950898067314));
#29432=CARTESIAN_POINT('Ctrl Pts',(34.8602323505772,-55.7191431963173,13.8891031245444));
#29433=CARTESIAN_POINT('Ctrl Pts',(34.2609995597881,-57.9641431697149,13.7779652339763));
#29434=CARTESIAN_POINT('Ctrl Pts',(32.0500242237095,-58.6781839861316,13.6668273434083));
#29435=CARTESIAN_POINT('Ctrl Pts',(30.2506759606945,-57.2080211780376,13.5556894528402));
#29436=CARTESIAN_POINT('Ctrl Pts',(30.4619007867399,-55.3316416370552,13.4653887652167));
#29437=CARTESIAN_POINT('Ctrl Pts',(31.2132787090688,-54.6644859207873,13.4121340411158));
#29438=CARTESIAN_POINT('Ctrl Pts',(31.4735006561133,-54.5153050203084,13.3959252805377));
#29439=CARTESIAN_POINT('Ctrl Pts',(31.4749259905951,-54.514117897405,14.1540747194623));
#29440=CARTESIAN_POINT('Ctrl Pts',(31.7139442620515,-54.3746753634159,14.1391197361979));
#29441=CARTESIAN_POINT('Ctrl Pts',(32.6363754616288,-54.0511292553545,14.0871187894108));
#29442=CARTESIAN_POINT('Ctrl Pts',(34.3667107654437,-54.7380212138032,13.998071879101));
#29443=CARTESIAN_POINT('Ctrl Pts',(34.817688121868,-57.0173840749687,13.886933988533));
#29444=CARTESIAN_POINT('Ctrl Pts',(33.1472639077745,-58.6324557555082,13.7757960979649));
#29445=CARTESIAN_POINT('Ctrl Pts',(30.8843823888257,-58.1050019311361,13.6646582073969));
#29446=CARTESIAN_POINT('Ctrl Pts',(30.1278087167359,-55.9943944231075,13.557417747896));
#29447=CARTESIAN_POINT('Ctrl Pts',(30.9468756244448,-54.8178045942286,13.4872232519178));
#29448=CARTESIAN_POINT('Ctrl Pts',(31.4724222119036,-54.5094432564574,13.4540747194623));
#29449=CARTESIAN_POINT('Origin',(32.5,-56.2916512459885,23.5459252805377));
#29450=CARTESIAN_POINT('',(31.4717219617816,-54.5141519916847,14.8540747194623));
#29451=CARTESIAN_POINT('',(31.4732712326059,-54.510037050691,14.7959252805377));
#29452=CARTESIAN_POINT('',(31.4726250000001,-54.5121855475624,23.5459252805377));
#29453=CARTESIAN_POINT('Ctrl Pts',(31.4732712326059,-54.510037050691,14.7959252805377));
#29454=CARTESIAN_POINT('Ctrl Pts',(31.5669343623879,-54.4548697514475,14.7900189367213));
#29455=CARTESIAN_POINT('Ctrl Pts',(32.2792813565109,-54.1097268956779,14.7470666293823));
#29456=CARTESIAN_POINT('Ctrl Pts',(33.9367458689222,-54.3335587337424,14.6670683585206));
#29457=CARTESIAN_POINT('Ctrl Pts',(34.9243151877952,-56.4367817964588,14.5559304679526));
#29458=CARTESIAN_POINT('Ctrl Pts',(33.6928803873874,-58.4071660616143,14.4447925773845));
#29459=CARTESIAN_POINT('Ctrl Pts',(31.3695905104292,-58.4411939406326,14.3336546868165));
#29460=CARTESIAN_POINT('Ctrl Pts',(30.0809735153021,-56.5077243843663,14.2225167962484));
#29461=CARTESIAN_POINT('Ctrl Pts',(30.7409078667025,-54.9881078888109,14.1432736608222));
#29462=CARTESIAN_POINT('Ctrl Pts',(31.3879183664802,-54.55797423098,14.1010764889186));
#29463=CARTESIAN_POINT('Ctrl Pts',(31.470366790827,-54.5112698283738,14.0959252805377));
#29464=CARTESIAN_POINT('Ctrl Pts',(31.4717219617816,-54.5141519916847,14.8540747194623));
#29465=CARTESIAN_POINT('Ctrl Pts',(31.8897217256654,-54.2773643841942,14.8280621840006));
#29466=CARTESIAN_POINT('Ctrl Pts',(33.1073033291158,-54.0451479062597,14.7650036850163));
#29467=CARTESIAN_POINT('Ctrl Pts',(34.7403671916158,-55.3540375815297,14.6648992225092));
#29468=CARTESIAN_POINT('Ctrl Pts',(34.5027924192342,-57.6654005284896,14.5537613319412));
#29469=CARTESIAN_POINT('Ctrl Pts',(32.4320391047204,-58.7193548713018,14.4426234413732));
#29470=CARTESIAN_POINT('Ctrl Pts',(30.423491023484,-57.5512051672244,14.3314855508051));
#29471=CARTESIAN_POINT('Ctrl Pts',(30.3301141372088,-55.5424943178045,14.2353026435015));
#29472=CARTESIAN_POINT('Ctrl Pts',(31.12185652721,-54.7200975505446,14.1761656997206));
#29473=CARTESIAN_POINT('Ctrl Pts',(31.4749259905951,-54.514117897405,14.1540747194623));
#29474=CARTESIAN_POINT('Origin',(32.5,-56.2916512459885,23.5459252805377));
#29475=CARTESIAN_POINT('',(31.4709276972304,-54.5092291784965,15.5540747194623));
#29476=CARTESIAN_POINT('',(31.4746475020099,-54.5147506716575,15.4959252805377));
#29477=CARTESIAN_POINT('',(31.4726250000001,-54.5121855475624,23.5459252805377));
#29478=CARTESIAN_POINT('Ctrl Pts',(31.4746475020099,-54.5147506716575,15.4959252805377));
#29479=CARTESIAN_POINT('Ctrl Pts',(31.7462982414417,-54.3571727743297,15.4789613845241));
#29480=CARTESIAN_POINT('Ctrl Pts',(32.7191784117559,-54.0441951966849,15.4249515249878));
#29481=CARTESIAN_POINT('Ctrl Pts',(34.4479835200066,-54.8412285476316,15.3338957019289));
#29482=CARTESIAN_POINT('Ctrl Pts',(34.7750596076319,-57.1416333665308,15.2227578113608));
#29483=CARTESIAN_POINT('Ctrl Pts',(33.019747820939,-58.6640399241195,15.1116199207928));
#29484=CARTESIAN_POINT('Ctrl Pts',(30.7887049884687,-58.0149721937253,15.0004820302248));
#29485=CARTESIAN_POINT('Ctrl Pts',(30.1593535158744,-55.9068520254157,14.895250483473));
#29486=CARTESIAN_POINT('Ctrl Pts',(30.9794574058775,-54.800891896276,14.827064900244));
#29487=CARTESIAN_POINT('Ctrl Pts',(31.4732712326059,-54.510037050691,14.7959252805377));
#29488=CARTESIAN_POINT('Ctrl Pts',(31.4709277056121,-54.5092291930959,15.5540747194623));
#29489=CARTESIAN_POINT('Ctrl Pts',(31.4713112637463,-54.5090077151575,15.5540505953261));
#29490=CARTESIAN_POINT('Ctrl Pts',(32.0608222902465,-54.1688851137838,15.5169805076671));
#29491=CARTESIAN_POINT('Ctrl Pts',(33.6099012175602,-54.1314466960922,15.4428644564855));
#29492=CARTESIAN_POINT('Ctrl Pts',(34.9168581194719,-56.052567070093,15.3317265659175));
#29493=CARTESIAN_POINT('Ctrl Pts',(34.0116373750326,-58.1925239040739,15.2205886753494));
#29494=CARTESIAN_POINT('Ctrl Pts',(31.722797799219,-58.5925904319764,15.1094507847814));
#29495=CARTESIAN_POINT('Ctrl Pts',(30.1453402095973,-56.8865812380664,14.9983128942134));
#29496=CARTESIAN_POINT('Ctrl Pts',(30.5878941637736,-55.1627827650417,14.913187539107));
#29497=CARTESIAN_POINT('Ctrl Pts',(31.2944239690072,-54.6145873774176,14.8651081475233));
#29498=CARTESIAN_POINT('Ctrl Pts',(31.4717219617816,-54.5141519916847,14.8540747194623));
#29499=CARTESIAN_POINT('Origin',(32.5,-56.2916512459885,23.5459252805377));
#29500=CARTESIAN_POINT('',(31.4747870773481,-54.5124102302141,16.2540747194623));
#29501=CARTESIAN_POINT('',(31.4710889776862,-54.513282910156,16.1959252805377));
#29502=CARTESIAN_POINT('',(31.4726250000001,-54.5121855475624,23.5459252805377));
#29503=CARTESIAN_POINT('Ctrl Pts',(31.4710889776862,-54.513282910156,16.1959252805377));
#29504=CARTESIAN_POINT('Ctrl Pts',(31.9210107047531,-54.2589533662338,16.1679038323268));
#29505=CARTESIAN_POINT('Ctrl Pts',(33.1965779324789,-54.0532698651996,16.1028364205933));
#29506=CARTESIAN_POINT('Ctrl Pts',(34.7877864833415,-55.4765446163129,16.0007230453371));
#29507=CARTESIAN_POINT('Ctrl Pts',(34.4255850063652,-57.7716810411711,15.8895851547691));
#29508=CARTESIAN_POINT('Ctrl Pts',(32.3008737352177,-58.7121294100224,15.778447264201));
#29509=CARTESIAN_POINT('Ctrl Pts',(30.3584249929227,-57.4370866648374,15.667309373633));
#29510=CARTESIAN_POINT('Ctrl Pts',(30.3734734150964,-55.4682647699115,15.5731353790785));
#29511=CARTESIAN_POINT('Ctrl Pts',(31.1530640353465,-54.7012933131323,15.5160073480468));
#29512=CARTESIAN_POINT('Ctrl Pts',(31.4746475020099,-54.5147506716575,15.4959252805377));
#29513=CARTESIAN_POINT('Ctrl Pts',(31.4747870773481,-54.5124102302141,16.2540747194623));
#29514=CARTESIAN_POINT('Ctrl Pts',(31.6511921427898,-54.4086339956355,16.2429930431288));
#29515=CARTESIAN_POINT('Ctrl Pts',(32.4803377190682,-54.0709860720283,16.1948654032727));
#29516=CARTESIAN_POINT('Ctrl Pts',(34.1948158493603,-54.5521215254954,16.1096917998938));
#29517=CARTESIAN_POINT('Ctrl Pts',(34.880650639758,-56.7721373989267,15.9985539093257));
#29518=CARTESIAN_POINT('Ctrl Pts',(33.387448901162,-58.5523588475275,15.8874160187577));
#29519=CARTESIAN_POINT('Ctrl Pts',(31.0819551189947,-58.2633289901972,15.7762781281897));
#29520=CARTESIAN_POINT('Ctrl Pts',(30.074632599944,-56.1700546084616,15.6651643617579));
#29521=CARTESIAN_POINT('Ctrl Pts',(30.8823044490718,-54.849117866319,15.5910965588487));
#29522=CARTESIAN_POINT('Ctrl Pts',(31.4709277056121,-54.5092291930959,15.5540747194623));
#29523=CARTESIAN_POINT('Origin',(32.5,-56.2916512459885,23.5459252805377));
#29524=CARTESIAN_POINT('',(31.4731301859007,-54.5151387721108,16.9540747194623));
#29525=CARTESIAN_POINT('',(31.471644989423,-54.5091305714223,16.8959252805377));
#29526=CARTESIAN_POINT('',(31.4726250000001,-54.5121855475624,23.5459252805377));
#29527=CARTESIAN_POINT('Ctrl Pts',(31.471644989423,-54.5091305714223,16.8959252805377));
#29528=CARTESIAN_POINT('Ctrl Pts',(31.5039012222331,-54.4903218421575,16.8938922436523));
#29529=CARTESIAN_POINT('Ctrl Pts',(32.1342604089221,-54.1469870049404,16.8548132432442));
#29530=CARTESIAN_POINT('Ctrl Pts',(33.7250789425299,-54.1946182477115,16.7786882793134));
#29531=CARTESIAN_POINT('Ctrl Pts',(34.9262501272131,-56.1835950962899,16.6675503887454));
#29532=CARTESIAN_POINT('Ctrl Pts',(33.9066470549119,-58.2714769641261,16.5564124981774));
#29533=CARTESIAN_POINT('Ctrl Pts',(31.5995239807838,-58.5472018994033,16.4452746076093));
#29534=CARTESIAN_POINT('Ctrl Pts',(30.1166168191438,-56.7583957419196,16.3341367170413));
#29535=CARTESIAN_POINT('Ctrl Pts',(30.6391000228397,-55.1011038763401,16.251020274684));
#29536=CARTESIAN_POINT('Ctrl Pts',(31.3261883471228,-54.5951916268688,16.2049497958495));
#29537=CARTESIAN_POINT('Ctrl Pts',(31.4710889776862,-54.513282910156,16.1959252805377));
#29538=CARTESIAN_POINT('Ctrl Pts',(31.4731301859007,-54.5151387721108,16.9540747194623));
#29539=CARTESIAN_POINT('Ctrl Pts',(31.8288294586133,-54.3119418969878,16.9319354909316));
#29540=CARTESIAN_POINT('Ctrl Pts',(32.9382338021843,-54.037919745286,16.8727502988781));
#29541=CARTESIAN_POINT('Ctrl Pts',(34.6305762357544,-55.1258856969254,16.776519143302));
#29542=CARTESIAN_POINT('Ctrl Pts',(34.6349312243122,-57.4494219828794,16.665381252734));
#29543=CARTESIAN_POINT('Ctrl Pts',(32.68515945149,-58.7132375833447,16.5542433621659));
#29544=CARTESIAN_POINT('Ctrl Pts',(30.5659091328683,-57.7605477465697,16.4431054715979));
#29545=CARTESIAN_POINT('Ctrl Pts',(30.2517487916383,-55.6924152700814,16.3430492573634));
#29546=CARTESIAN_POINT('Ctrl Pts',(31.0614712898342,-54.7555571943486,16.2800390066515));
#29547=CARTESIAN_POINT('Ctrl Pts',(31.4747870773481,-54.5124102302141,16.2540747194623));
#29548=CARTESIAN_POINT('Origin',(32.5,-56.2916512459885,23.5459252805377));
#29549=CARTESIAN_POINT('',(31.4703256079253,-54.5106072564107,17.6540747194623));
#29550=CARTESIAN_POINT('',(31.4749747334417,-54.5133534323073,17.5959252805377));
#29551=CARTESIAN_POINT('',(31.4726250000001,-54.5121855475624,23.5459252805377));
#29552=CARTESIAN_POINT('Ctrl Pts',(31.4749747334417,-54.5133534323073,17.5959252805377));
#29553=CARTESIAN_POINT('Ctrl Pts',(31.6837908396868,-54.3909711398323,17.582834691455));
#29554=CARTESIAN_POINT('Ctrl Pts',(32.560671629995,-54.0596531620232,17.5326981388497));
#29555=CARTESIAN_POINT('Ctrl Pts',(34.2863923370768,-54.6463037965649,17.4455156227217));
#29556=CARTESIAN_POINT('Ctrl Pts',(34.8511887990977,-56.9001551837646,17.3343777321536));
#29557=CARTESIAN_POINT('Ctrl Pts',(33.26391548901,-58.5970360158138,17.2232398415856));
#29558=CARTESIAN_POINT('Ctrl Pts',(30.9774216684404,-58.1837720232006,17.1121019510175));
#29559=CARTESIAN_POINT('Ctrl Pts',(30.1008940923714,-56.0778693719696,17.0029970973349));
#29560=CARTESIAN_POINT('Ctrl Pts',(30.9161286969814,-54.8330541866883,16.9309382071749));
#29561=CARTESIAN_POINT('Ctrl Pts',(31.471644989423,-54.5091305714223,16.8959252805377));
#29562=CARTESIAN_POINT('Ctrl Pts',(31.4703256079253,-54.5106072564107,17.6540747194623));
#29563=CARTESIAN_POINT('Ctrl Pts',(32.0008800348568,-54.2091890880958,17.6208779387343));
#29564=CARTESIAN_POINT('Ctrl Pts',(33.430914992466,-54.089095285949,17.5506351944836));
#29565=CARTESIAN_POINT('Ctrl Pts',(34.8788327758259,-55.8022444250302,17.4433464867103));
#29566=CARTESIAN_POINT('Ctrl Pts',(34.2013246967004,-58.0248156029211,17.3322085961422));
#29567=CARTESIAN_POINT('Ctrl Pts',(31.9665748283507,-58.6610017894909,17.2210707055742));
#29568=CARTESIAN_POINT('Ctrl Pts',(30.2200750690644,-57.1284945533304,17.1099328150062));
#29569=CARTESIAN_POINT('Ctrl Pts',(30.4926187339168,-55.2878838417842,17.0209341529689));
#29570=CARTESIAN_POINT('Ctrl Pts',(31.2336315607436,-54.6519548298357,16.9689814544542));
#29571=CARTESIAN_POINT('Ctrl Pts',(31.4731301859007,-54.5151387721108,16.9540747194623));
#29572=CARTESIAN_POINT('Origin',(32.5,-56.2916512459885,23.5459252805377));
#29573=CARTESIAN_POINT('',(31.4737670936581,-54.5105654320666,18.3540747194623));
#29574=CARTESIAN_POINT('',(31.472390363387,-54.5147550766704,18.2959252805377));
#29575=CARTESIAN_POINT('',(31.4726250000001,-54.5121855475624,23.5459252805377));
#29576=CARTESIAN_POINT('Ctrl Pts',(31.472390363387,-54.5147550766704,18.2959252805377));
#29577=CARTESIAN_POINT('Ctrl Pts',(31.8605071662086,-54.2941313842958,18.2717771392578));
#29578=CARTESIAN_POINT('Ctrl Pts',(33.02540146796,-54.0403220897573,18.2105830344552));
#29579=CARTESIAN_POINT('Ctrl Pts',(34.6904921906955,-55.242790066521,18.1123429661299));
#29580=CARTESIAN_POINT('Ctrl Pts',(34.5692083587434,-57.5631631725538,18.0012050755619));
#29581=CARTESIAN_POINT('Ctrl Pts',(32.5539546496148,-58.7197069922754,17.8900671849938));
#29582=CARTESIAN_POINT('Ctrl Pts',(30.4893156378063,-57.6538238513956,17.7789292944258));
#29583=CARTESIAN_POINT('Ctrl Pts',(30.2914909874078,-55.613533902771,17.6808819929404));
#29584=CARTESIAN_POINT('Ctrl Pts',(31.0928476967877,-54.7373092545057,17.6198806549777));
#29585=CARTESIAN_POINT('Ctrl Pts',(31.4749747334417,-54.5133534323073,17.5959252805377));
#29586=CARTESIAN_POINT('Ctrl Pts',(31.4737670936581,-54.5105654320666,18.3540747194623));
#29587=CARTESIAN_POINT('Ctrl Pts',(31.5881478071784,-54.4431225718917,18.3468663500598));
#29588=CARTESIAN_POINT('Ctrl Pts',(32.3290694209141,-54.0987447143864,18.3026120171345));
#29589=CARTESIAN_POINT('Ctrl Pts',(34.004501193851,-54.3851254608373,18.2213117206866));
#29590=CARTESIAN_POINT('Ctrl Pts',(34.9177373632483,-56.5216739711635,18.1101738301186));
#29591=CARTESIAN_POINT('Ctrl Pts',(33.6179911050581,-58.4476800725016,17.9990359395505));
#29592=CARTESIAN_POINT('Ctrl Pts',(31.2949349095266,-58.4002485379024,17.8878980489825));
#29593=CARTESIAN_POINT('Ctrl Pts',(30.074888457673,-56.4227939888948,17.7767601584144));
#29594=CARTESIAN_POINT('Ctrl Pts',(30.7759689649702,-54.951821535532,17.6988190485744));
#29595=CARTESIAN_POINT('Ctrl Pts',(31.4088075653018,-54.5455568389317,17.657923902257));
#29596=CARTESIAN_POINT('Ctrl Pts',(31.4703256079253,-54.5106072564107,17.6540747194623));
#29597=CARTESIAN_POINT('Origin',(32.5,-56.2916512459885,23.5459252805377));
#29598=CARTESIAN_POINT('',(31.4743570776169,-54.515029390224,19.0540747194623));
#29599=CARTESIAN_POINT('',(31.4704988599393,-54.5097377243633,18.9959252805377));
#29600=CARTESIAN_POINT('',(31.4726250000001,-54.5121855475624,23.5459252805377));
#29601=CARTESIAN_POINT('Ctrl Pts',(31.4704988599393,-54.5097377243633,18.9959252805377));
#29602=CARTESIAN_POINT('Ctrl Pts',(32.0317105894022,-54.1886772858723,18.9607195870605));
#29603=CARTESIAN_POINT('Ctrl Pts',(33.5233071799065,-54.1091544860817,18.8884679300607));
#29604=CARTESIAN_POINT('Ctrl Pts',(34.9018152245058,-55.9315825877644,18.7791703095382));
#29605=CARTESIAN_POINT('Ctrl Pts',(34.1051248236507,-58.1142702713998,18.6680324189701));
#29606=CARTESIAN_POINT('Ctrl Pts',(31.8392454683584,-58.628694091168,18.5568945284021));
#29607=CARTESIAN_POINT('Ctrl Pts',(30.1781622293417,-57.0039960908763,18.445756637834));
#29608=CARTESIAN_POINT('Ctrl Pts',(30.5414387587065,-55.2219675363374,18.3587668885459));
#29609=CARTESIAN_POINT('Ctrl Pts',(31.2650923575403,-54.6325929315102,18.3088231027804));
#29610=CARTESIAN_POINT('Ctrl Pts',(31.472390363387,-54.5147550766704,18.2959252805377));
#29611=CARTESIAN_POINT('Ctrl Pts',(31.4743570776169,-54.515029390224,19.0540747194623));
#29612=CARTESIAN_POINT('Ctrl Pts',(31.767179706711,-54.345835768675,19.0358087978625));
#29613=CARTESIAN_POINT('Ctrl Pts',(32.773519448388,-54.0410032090046,18.98049691274));
#29614=CARTESIAN_POINT('Ctrl Pts',(34.4976287681445,-54.9104040861686,18.8881390640948));
#29615=CARTESIAN_POINT('Ctrl Pts',(34.7438661544311,-57.2208600991234,18.7770011735268));
#29616=CARTESIAN_POINT('Ctrl Pts',(32.9362674024074,-58.680800710823,18.6658632829587));
#29617=CARTESIAN_POINT('Ctrl Pts',(30.7293481493445,-57.9539257225797,18.5547253923907));
#29618=CARTESIAN_POINT('Ctrl Pts',(30.1811487641285,-55.8513808790736,18.4507958712252));
#29619=CARTESIAN_POINT('Ctrl Pts',(31.0003111545141,-54.7897315757275,18.3839123135824));
#29620=CARTESIAN_POINT('Ctrl Pts',(31.4737670936581,-54.5105654320666,18.3540747194623));
#29621=CARTESIAN_POINT('Origin',(32.5,-56.2916512459885,23.5459252805377));
#29622=CARTESIAN_POINT('',(31.4707591192322,-54.5126331290242,19.7540747194623));
#29623=CARTESIAN_POINT('',(31.4743950169645,-54.5114972463166,19.6959252805377));
#29624=CARTESIAN_POINT('',(31.4726250000001,-54.5121855475624,23.5459252805377));
#29625=CARTESIAN_POINT('Ctrl Pts',(31.4743950169645,-54.5114972463166,19.6959252805377));
#29626=CARTESIAN_POINT('Ctrl Pts',(31.6208668833956,-54.425154465736,19.686707998386));
#29627=CARTESIAN_POINT('Ctrl Pts',(32.4069324234732,-54.0834056527267,19.6404447527116));
#29628=CARTESIAN_POINT('Ctrl Pts',(34.1053854498936,-54.4692617796666,19.5571355435145));
#29629=CARTESIAN_POINT('Ctrl Pts',(34.9017637086038,-56.6520633710957,19.4459976529464));
#29630=CARTESIAN_POINT('Ctrl Pts',(33.4997804064766,-58.5049756574095,19.3348597623784));
#29631=CARTESIAN_POINT('Ctrl Pts',(31.1826867602698,-58.3320070089704,19.2237218718103));
#29632=CARTESIAN_POINT('Ctrl Pts',(30.0713448616115,-56.2914775915524,19.1125839812423));
#29633=CARTESIAN_POINT('Ctrl Pts',(30.8308409091996,-54.8974452606956,19.0366517841514));
#29634=CARTESIAN_POINT('Ctrl Pts',(31.4411632317234,-54.5265201776941,18.9977655505832));
#29635=CARTESIAN_POINT('Ctrl Pts',(31.4704988599393,-54.5097377243633,18.9959252805377));
#29636=CARTESIAN_POINT('Ctrl Pts',(31.4707591192322,-54.5126331290242,19.7540747194623));
#29637=CARTESIAN_POINT('Ctrl Pts',(31.9411934042825,-54.2467857936504,19.7247512456653));
#29638=CARTESIAN_POINT('Ctrl Pts',(33.2549727142225,-54.0602154670517,19.6583818083455));
#29639=CARTESIAN_POINT('Ctrl Pts',(34.8149526935151,-55.5572409773789,19.5549664075031));
#29640=CARTESIAN_POINT('Ctrl Pts',(34.3725208876465,-57.8382701189333,19.443828516935));
#29641=CARTESIAN_POINT('Ctrl Pts',(32.2161494783462,-58.7036614639378,19.332690626367));
#29642=CARTESIAN_POINT('Ctrl Pts',(30.3195896701685,-57.3613125035426,19.221552735799));
#29643=CARTESIAN_POINT('Ctrl Pts',(30.4024811841689,-55.4214247242036,19.1286807668307));
#29644=CARTESIAN_POINT('Ctrl Pts',(31.1732925394658,-54.6889852067103,19.0728547613852));
#29645=CARTESIAN_POINT('Ctrl Pts',(31.4743570776169,-54.515029390224,19.0540747194623));
#29646=CARTESIAN_POINT('Origin',(32.5,-56.2916512459885,23.5459252805377));
#29647=CARTESIAN_POINT('',(31.4721876288368,-54.5092967477939,20.4540747194623));
#29648=CARTESIAN_POINT('',(31.4737733324271,-54.5152256259023,20.3959252805377));
#29649=CARTESIAN_POINT('',(31.4726250000001,-54.5121855475624,23.5459252805377));
#29650=CARTESIAN_POINT('Ctrl Pts',(31.4737733324271,-54.5152256259023,20.3959252805377));
#29651=CARTESIAN_POINT('Ctrl Pts',(31.799246207199,-54.3283059275285,20.3756504461887));
#29652=CARTESIAN_POINT('Ctrl Pts',(32.8583863662623,-54.0381735568299,20.318329648317));
#29653=CARTESIAN_POINT('Ctrl Pts',(34.5693901517228,-55.0204352512209,20.2239628869227));
#29654=CARTESIAN_POINT('Ctrl Pts',(34.6903421852681,-57.3408256590054,20.1128249963547));
#29655=CARTESIAN_POINT('Ctrl Pts',(32.8064491443347,-58.7008948504122,20.0016871057866));
#29656=CARTESIAN_POINT('Ctrl Pts',(30.6420597422744,-57.8557560368671,19.8905492152186));
#29657=CARTESIAN_POINT('Ctrl Pts',(30.2167292658396,-55.7678005164131,19.7886286068023));
#29658=CARTESIAN_POINT('Ctrl Pts',(31.0321693333385,-54.7721820870222,19.7237539619086));
#29659=CARTESIAN_POINT('Ctrl Pts',(31.4743950169645,-54.5114972463166,19.6959252805377));
#29660=CARTESIAN_POINT('Ctrl Pts',(31.4721876288368,-54.5092967477939,20.4540747194623));
#29661=CARTESIAN_POINT('Ctrl Pts',(31.5250686260056,-54.4783192167782,20.4507396569907));
#29662=CARTESIAN_POINT('Ctrl Pts',(32.1824999100289,-54.133716656297,20.4103586309964));
#29663=CARTESIAN_POINT('Ctrl Pts',(33.7978345552324,-54.2388509530007,20.3329316414794));
#29664=CARTESIAN_POINT('Ctrl Pts',(34.9285465373885,-56.2687104209716,20.2217937509113));
#29665=CARTESIAN_POINT('Ctrl Pts',(33.836382221401,-58.3195681810162,20.1106558603433));
#29666=CARTESIAN_POINT('Ctrl Pts',(31.5210121579647,-58.5142504249981,19.9995179697753));
#29667=CARTESIAN_POINT('Ctrl Pts',(30.101720741136,-56.674562508041,19.8883800792072));
#29668=CARTESIAN_POINT('Ctrl Pts',(30.6728871983315,-55.0622630484847,19.8065656624362));
#29669=CARTESIAN_POINT('Ctrl Pts',(31.3468677972824,-54.5826454110005,19.7617972091879));
#29670=CARTESIAN_POINT('Ctrl Pts',(31.4707591192322,-54.5126331290242,19.7540747194623));
#29671=CARTESIAN_POINT('Origin',(32.5,-56.2916512459885,23.5459252805377));
#29672=CARTESIAN_POINT('',(31.4749609874599,-54.5139076530798,21.1540747194623));
#29673=CARTESIAN_POINT('',(31.4704172621348,-54.5115691325664,21.0959252805377));
#29674=CARTESIAN_POINT('',(31.4726250000001,-54.5121855475624,23.5459252805377));
#29675=CARTESIAN_POINT('Ctrl Pts',(31.4704172621348,-54.5115691325664,21.0959252805377));
#29676=CARTESIAN_POINT('Ctrl Pts',(31.9722041658629,-54.227575372343,21.0645928939914));
#29677=CARTESIAN_POINT('Ctrl Pts',(33.3458362247711,-54.0736222398741,20.9962145439225));
#29678=CARTESIAN_POINT('Ctrl Pts',(34.8512746399183,-55.6834843462923,20.890790230331));
#29679=CARTESIAN_POINT('Ctrl Pts',(34.2861576030319,-57.9372537407841,20.7796523397629));
#29680=CARTESIAN_POINT('Ctrl Pts',(32.086148188353,-58.6847859443394,20.6685144491949));
#29681=CARTESIAN_POINT('Ctrl Pts',(30.2649430630364,-57.2418541016519,20.5573765586268));
#29682=CARTESIAN_POINT('Ctrl Pts',(30.4485426703034,-55.3510892045502,20.4665135024078));
#29683=CARTESIAN_POINT('Ctrl Pts',(31.2045456025534,-54.6698436293139,20.4126964097114));
#29684=CARTESIAN_POINT('Ctrl Pts',(31.4737733324271,-54.5152256259023,20.3959252805377));
#29685=CARTESIAN_POINT('Ctrl Pts',(31.4749609874599,-54.5139076530798,21.1540747194623));
#29686=CARTESIAN_POINT('Ctrl Pts',(31.70486029749,-54.3795842898515,21.1396821047934));
#29687=CARTESIAN_POINT('Ctrl Pts',(32.6134298152417,-54.053477853398,21.0882435266019));
#29688=CARTESIAN_POINT('Ctrl Pts',(34.3429657642116,-54.7099453599153,20.9997589848876));
#29689=CARTESIAN_POINT('Ctrl Pts',(34.8284152391772,-56.982193672835,20.8886210943196));
#29690=CARTESIAN_POINT('Ctrl Pts',(33.18263271582,-58.6223996095028,20.7774832037515));
#29691=CARTESIAN_POINT('Ctrl Pts',(30.9120322857351,-58.1292356735021,20.6663453131835));
#29692=CARTESIAN_POINT('Ctrl Pts',(30.1194352615649,-56.0193863503516,20.5585424850871));
#29693=CARTESIAN_POINT('Ctrl Pts',(30.9376650889446,-54.8224184634311,20.4877856205134));
#29694=CARTESIAN_POINT('Ctrl Pts',(31.4721876288368,-54.5092967477939,20.4540747194623));
#29695=CARTESIAN_POINT('Origin',(32.5,-56.2916512459885,23.5459252805377));
#29696=CARTESIAN_POINT('',(31.4716734168817,-54.5151354051885,21.8540747194623));
#29697=CARTESIAN_POINT('',(31.4730118547325,-54.5098571360138,21.7959252805377));
#29698=CARTESIAN_POINT('',(31.4726250000001,-54.5121855475624,23.5459252805377));
#29699=CARTESIAN_POINT('',(30.5157034944333,-56.8250975324092,22.));
#29700=CARTESIAN_POINT('Ctrl Pts',(30.5157034944333,-56.8250975324092,22.));
#29701=CARTESIAN_POINT('Ctrl Pts',(30.3383199129809,-56.1652717359215,21.9629540364773));
#29702=CARTESIAN_POINT('Ctrl Pts',(30.5738806361657,-55.1809621297242,21.9143122762981));
#29703=CARTESIAN_POINT('Ctrl Pts',(31.2853315674047,-54.6208532363719,21.8656705161189));
#29704=CARTESIAN_POINT('Ctrl Pts',(31.4716734168817,-54.5151354051885,21.8540747194623));
#29705=CARTESIAN_POINT('',(31.043364830276,-57.7461496994443,22.));
#29706=CARTESIAN_POINT('Origin',(32.5,-56.2916512459885,22.));
#29707=CARTESIAN_POINT('Ctrl Pts',(31.0433632440414,-57.7461514510325,22.));
#29708=CARTESIAN_POINT('Ctrl Pts',(30.5726971034827,-57.2735716615612,21.9636770818144));
#29709=CARTESIAN_POINT('Ctrl Pts',(30.1593922934378,-55.9189388685996,21.895652175327));
#29710=CARTESIAN_POINT('Ctrl Pts',(30.9704682366631,-54.8056054537255,21.8276272688396));
#29711=CARTESIAN_POINT('Ctrl Pts',(31.4730118547325,-54.5098571360138,21.7959252805377));
#29712=CARTESIAN_POINT('Origin',(32.5,56.2916512459885,3.));
#29713=CARTESIAN_POINT('',(33.334828594439,57.735188017533,6.12851963660981));
#29714=CARTESIAN_POINT('',(33.3331620889267,57.736668395617,6.3214803633902));
#29715=CARTESIAN_POINT('',(33.333,57.7344495686934,3.));
#29716=CARTESIAN_POINT('',(33.5940263469955,57.5480995545471,7.));
#29717=CARTESIAN_POINT('Ctrl Pts',(33.3331620889267,57.736668395617,6.3214803633902));
#29718=CARTESIAN_POINT('Ctrl Pts',(33.2830618082469,57.7660644611829,6.32537779445737));
#29719=CARTESIAN_POINT('Ctrl Pts',(33.2314063486239,57.7926890534068,6.32927522552456));
#29720=CARTESIAN_POINT('Ctrl Pts',(33.1783991110197,57.816276539757,6.33317265659174));
#29721=CARTESIAN_POINT('Ctrl Pts',(32.6745533323838,58.0404809307674,6.37021862011442));
#29722=CARTESIAN_POINT('Ctrl Pts',(32.0485753278831,57.9902848612727,6.4072645836371));
#29723=CARTESIAN_POINT('Ctrl Pts',(31.5869763637319,57.6885282775577,6.44431054715978));
#29724=CARTESIAN_POINT('Ctrl Pts',(31.1253773995808,57.3867716938426,6.48135651068246));
#29725=CARTESIAN_POINT('Ctrl Pts',(30.8281574757791,56.8334545959073,6.51840247420514));
#29726=CARTESIAN_POINT('Ctrl Pts',(30.8312835014825,56.2820697925607,6.55544843772782));
#29727=CARTESIAN_POINT('Ctrl Pts',(30.8344095271858,55.730684989214,6.5924944012505));
#29728=CARTESIAN_POINT('Ctrl Pts',(31.1378815023941,55.181232480456,6.62954036477319));
#29729=CARTESIAN_POINT('Ctrl Pts',(31.6029277671501,54.8846445462125,6.66658632829587));
#29730=CARTESIAN_POINT('Ctrl Pts',(32.0679740319062,54.5880566119689,6.70363229181855));
#29731=CARTESIAN_POINT('Ctrl Pts',(32.6945945862099,54.5443332522399,6.74067825534123));
#29732=CARTESIAN_POINT('Ctrl Pts',(33.1957905862086,54.7745591362764,6.77772421886391));
#29733=CARTESIAN_POINT('Ctrl Pts',(33.6969865862073,55.0047850203128,6.81477018238659));
#29734=CARTESIAN_POINT('Ctrl Pts',(34.072758031901,55.5089601481147,6.85181614590928));
#29735=CARTESIAN_POINT('Ctrl Pts',(34.1514677107856,56.0538413345857,6.88886210943196));
#29736=CARTESIAN_POINT('Ctrl Pts',(34.2301773896702,56.5987225210566,6.92590807295464));
#29737=CARTESIAN_POINT('Ctrl Pts',(34.0118253017458,57.1843097661965,6.96295403647732));
#29738=CARTESIAN_POINT('Ctrl Pts',(33.5940263469955,57.5480995545471,7.));
#29739=CARTESIAN_POINT('',(31.0815846268763,57.1712794637625,6.99999999999998));
#29740=CARTESIAN_POINT('Origin',(32.5,56.2916512459885,7.));
#29741=CARTESIAN_POINT('',(33.3322874886545,57.7319139206534,6.8285196366098));
#29742=CARTESIAN_POINT('Ctrl Pts',(31.0815830733445,57.1712803260698,6.99999999999998));
#29743=CARTESIAN_POINT('Ctrl Pts',(31.3671885733958,57.6305045882043,6.96367708181444));
#29744=CARTESIAN_POINT('Ctrl Pts',(31.8971081113246,57.9389632567025,6.92735416362889));
#29745=CARTESIAN_POINT('Ctrl Pts',(32.4375390310397,57.9591354579207,6.89103124544335));
#29746=CARTESIAN_POINT('Ctrl Pts',(32.7475655738981,57.9707075526647,6.87019404249883));
#29747=CARTESIAN_POINT('Ctrl Pts',(33.0610513288344,57.8874068657131,6.84935683955432));
#29748=CARTESIAN_POINT('Ctrl Pts',(33.3322874886545,57.7319139206534,6.8285196366098));
#29749=CARTESIAN_POINT('',(33.333,57.7344495686934,8.));
#29750=CARTESIAN_POINT('',(33.333,57.7344495686934,3.));
#29751=CARTESIAN_POINT('Origin',(32.5,56.2916512459885,8.));
#29752=CARTESIAN_POINT('Ctrl Pts',(33.3322874886545,57.7319139206534,6.8285196366098));
#29753=CARTESIAN_POINT('Ctrl Pts',(33.5432755942256,57.6109596867872,6.81231087603164));
#29754=CARTESIAN_POINT('Ctrl Pts',(33.7286988454439,57.4463225594197,6.79610211545347));
#29755=CARTESIAN_POINT('Ctrl Pts',(33.8670427528185,57.2486779404332,6.77989335487531));
#29756=CARTESIAN_POINT('Ctrl Pts',(34.1832349330579,56.7969509061471,6.74284739135263));
#29757=CARTESIAN_POINT('Ctrl Pts',(34.2534965093545,56.1728010705694,6.70580142782995));
#29758=CARTESIAN_POINT('Ctrl Pts',(34.0454742915244,55.6620590905692,6.66875546430727));
#29759=CARTESIAN_POINT('Ctrl Pts',(33.8374520736943,55.1513171105689,6.63170950078459));
#29760=CARTESIAN_POINT('Ctrl Pts',(33.3511460617374,54.7539829861461,6.59466353726191));
#29761=CARTESIAN_POINT('Ctrl Pts',(32.8092161915406,54.6518060909041,6.55761757373923));
#29762=CARTESIAN_POINT('Ctrl Pts',(32.2672863213437,54.549629195662,6.52057161021655));
#29763=CARTESIAN_POINT('Ctrl Pts',(31.6697325929069,54.7426095296009,6.48352564669386));
#29764=CARTESIAN_POINT('Ctrl Pts',(31.2899790079621,55.1424751852064,6.44647968317118));
#29765=CARTESIAN_POINT('Ctrl Pts',(30.9102254230173,55.542340840812,6.4094337196485));
#29766=CARTESIAN_POINT('Ctrl Pts',(30.7482719815646,56.1490918180843,6.37238775612583));
#29767=CARTESIAN_POINT('Ctrl Pts',(30.8782626384457,56.6850216626073,6.33534179260315));
#29768=CARTESIAN_POINT('Ctrl Pts',(31.0082532953267,57.2209515071302,6.29829582908047));
#29769=CARTESIAN_POINT('Ctrl Pts',(31.4301880505415,57.6860602189039,6.26124986555778));
#29770=CARTESIAN_POINT('Ctrl Pts',(31.9509534890593,57.8674999291041,6.2242039020351));
#29771=CARTESIAN_POINT('Ctrl Pts',(32.3993069550895,58.023710608475,6.19230914689333));
#29772=CARTESIAN_POINT('Ctrl Pts',(32.9209173239095,57.9696554900369,6.16041439175157));
#29773=CARTESIAN_POINT('Ctrl Pts',(33.334828594439,57.735188017533,6.12851963660981));
#29774=CARTESIAN_POINT('Origin',(32.5,56.2916512459885,3.));
#29775=CARTESIAN_POINT('',(33.3324736911222,57.73618752158,5.4285196366098));
#29776=CARTESIAN_POINT('',(33.3311322154952,57.7328790961699,5.6214803633902));
#29777=CARTESIAN_POINT('',(33.333,57.7344495686934,3.));
#29778=CARTESIAN_POINT('Ctrl Pts',(33.3311322154952,57.7328790961699,5.6214803633902));
#29779=CARTESIAN_POINT('Ctrl Pts',(33.1373356857267,57.8459393971242,5.63643534665463));
#29780=CARTESIAN_POINT('Ctrl Pts',(32.9222440320564,57.9213835767879,5.65139032991906));
#29781=CARTESIAN_POINT('Ctrl Pts',(32.7012486057465,57.9482311745983,5.66634531318349));
#29782=CARTESIAN_POINT('Ctrl Pts',(32.1538064350001,58.0147371085448,5.70339127670617));
#29783=CARTESIAN_POINT('Ctrl Pts',(31.5701366653479,57.7830375418651,5.74043724022885));
#29784=CARTESIAN_POINT('Ctrl Pts',(31.2173595401895,57.3591689672607,5.77748320375153));
#29785=CARTESIAN_POINT('Ctrl Pts',(30.8645824150311,56.9353003926564,5.81452916727421));
#29786=CARTESIAN_POINT('Ctrl Pts',(30.7426979343665,56.3192628101275,5.85157513079689));
#29787=CARTESIAN_POINT('Ctrl Pts',(30.9074862986933,55.7929935490273,5.88862109431957));
#29788=CARTESIAN_POINT('Ctrl Pts',(31.0722746630201,55.266724287927,5.92566705784225));
#29789=CARTESIAN_POINT('Ctrl Pts',(31.5237358723383,54.8302233482555,5.96271302136494));
#29790=CARTESIAN_POINT('Ctrl Pts',(32.0552579823815,54.6832494251182,5.99975898488761));
#29791=CARTESIAN_POINT('Ctrl Pts',(32.5867800924248,54.5362755019809,6.0368049484103));
#29792=CARTESIAN_POINT('Ctrl Pts',(33.1983631031929,54.6788285953779,6.07385091193297));
#29793=CARTESIAN_POINT('Ctrl Pts',(33.6101089221164,55.0456852682332,6.11089687545565));
#29794=CARTESIAN_POINT('Ctrl Pts',(34.02185474104,55.4125419410885,6.14794283897833));
#29795=CARTESIAN_POINT('Ctrl Pts',(34.2337633681189,56.003702193402,6.18498880250102));
#29796=CARTESIAN_POINT('Ctrl Pts',(34.1488609052729,56.5485847453165,6.2220347660237));
#29797=CARTESIAN_POINT('Ctrl Pts',(34.0728906300367,57.036142774291,6.2551832984792));
#29798=CARTESIAN_POINT('Ctrl Pts',(33.7592763040381,57.4866482113774,6.2883318309347));
#29799=CARTESIAN_POINT('Ctrl Pts',(33.3331620889267,57.736668395617,6.3214803633902));
#29800=CARTESIAN_POINT('Ctrl Pts',(33.334828594439,57.735188017533,6.12851963660981));
#29801=CARTESIAN_POINT('Ctrl Pts',(33.4016779305205,57.6973200105818,6.12336842822889));
#29802=CARTESIAN_POINT('Ctrl Pts',(33.4657180077386,57.6547460681795,6.11821721984798));
#29803=CARTESIAN_POINT('Ctrl Pts',(33.5261864969391,57.6075919565364,6.11306601146706));
#29804=CARTESIAN_POINT('Ctrl Pts',(33.96105794448,57.2684735651416,6.07602004794438));
#29805=CARTESIAN_POINT('Ctrl Pts',(34.2112047177408,56.6924660737253,6.0389740844217));
#29806=CARTESIAN_POINT('Ctrl Pts',(34.1621425519641,56.1431855476953,6.00192812089902));
#29807=CARTESIAN_POINT('Ctrl Pts',(34.1130803861875,55.5939050216654,5.96488215737634));
#29808=CARTESIAN_POINT('Ctrl Pts',(33.7648092813734,55.0713514610218,5.92783619385366));
#29809=CARTESIAN_POINT('Ctrl Pts',(33.2767190788242,54.8146729733941,5.89079023033098));
#29810=CARTESIAN_POINT('Ctrl Pts',(32.7886288762749,54.5579944857664,5.8537442668083));
#29811=CARTESIAN_POINT('Ctrl Pts',(32.1607195759905,54.5671910711545,5.81669830328562));
#29812=CARTESIAN_POINT('Ctrl Pts',(31.6803566282497,54.8380546099094,5.77965233976293));
#29813=CARTESIAN_POINT('Ctrl Pts',(31.199993680509,55.1089181486644,5.74260637624025));
#29814=CARTESIAN_POINT('Ctrl Pts',(30.8671770853118,55.6414486407862,5.70556041271757));
#29815=CARTESIAN_POINT('Ctrl Pts',(30.8342226473039,56.1919301102113,5.66851444919489));
#29816=CARTESIAN_POINT('Ctrl Pts',(30.801268209296,56.7424115796364,5.63146848567221));
#29817=CARTESIAN_POINT('Ctrl Pts',(31.0681759284774,57.3108440263648,5.59442252214954));
#29818=CARTESIAN_POINT('Ctrl Pts',(31.5127937714062,57.6370813071645,5.55737655862686));
#29819=CARTESIAN_POINT('Ctrl Pts',(31.9574116143351,57.9633185879642,5.52033059510418));
#29820=CARTESIAN_POINT('Ctrl Pts',(32.5797395810114,58.0473607028353,5.48328463158149));
#29821=CARTESIAN_POINT('Ctrl Pts',(33.0949658502734,57.8507452062818,5.44623866805881));
#29822=CARTESIAN_POINT('Ctrl Pts',(33.1771098465446,57.8193982358743,5.44033232424248));
#29823=CARTESIAN_POINT('Ctrl Pts',(33.2565314423349,57.7809172756723,5.43442598042614));
#29824=CARTESIAN_POINT('Ctrl Pts',(33.3324736911222,57.73618752158,5.4285196366098));
#29825=CARTESIAN_POINT('Origin',(32.5,56.2916512459885,3.));
#29826=CARTESIAN_POINT('',(33.3313578105535,57.7323657066332,4.7285196366098));
#29827=CARTESIAN_POINT('',(33.3337300498339,57.7328514726872,4.9214803633902));
#29828=CARTESIAN_POINT('',(33.333,57.7344495686934,3.));
#29829=CARTESIAN_POINT('Ctrl Pts',(33.3337300498339,57.7328514726872,4.9214803633902));
#29830=CARTESIAN_POINT('Ctrl Pts',(32.9948149402967,57.9248393749082,4.94749289885188));
#29831=CARTESIAN_POINT('Ctrl Pts',(32.5875734400098,58.0025082442025,4.97350543431356));
#29832=CARTESIAN_POINT('Ctrl Pts',(32.2063909254829,57.9343784669252,4.99951796977524));
#29833=CARTESIAN_POINT('Ctrl Pts',(31.6635267533437,57.8373508916032,5.03656393329792));
#29834=CARTESIAN_POINT('Ctrl Pts',(31.1735161025779,57.4446106606262,5.0736098968206));
#29835=CARTESIAN_POINT('Ctrl Pts',(30.9606151335011,56.935897533533,5.11065586034328));
#29836=CARTESIAN_POINT('Ctrl Pts',(30.7477141644243,56.4271844064398,5.14770182386596));
#29837=CARTESIAN_POINT('Ctrl Pts',(30.8119228770365,55.8024983832305,5.18474778738864));
#29838=CARTESIAN_POINT('Ctrl Pts',(31.1238557751029,55.3477306326436,5.22179375091132));
#29839=CARTESIAN_POINT('Ctrl Pts',(31.4357886731693,54.8929628820567,5.258839714434));
#29840=CARTESIAN_POINT('Ctrl Pts',(31.9954457566899,54.6081134040922,5.29588567795668));
#29841=CARTESIAN_POINT('Ctrl Pts',(32.5466968174263,54.6235450421449,5.33293164147937));
#29842=CARTESIAN_POINT('Ctrl Pts',(33.0979478781627,54.6389766801977,5.36997760500205));
#29843=CARTESIAN_POINT('Ctrl Pts',(33.6407929161149,54.9546894342676,5.40702356852472));
#29844=CARTESIAN_POINT('Ctrl Pts',(33.9267957627755,55.4261958418307,5.44406953204741));
#29845=CARTESIAN_POINT('Ctrl Pts',(34.2127986094361,55.8977022493938,5.48111549557009));
#29846=CARTESIAN_POINT('Ctrl Pts',(34.2419592648052,56.52500231045,5.51816145909277));
#29847=CARTESIAN_POINT('Ctrl Pts',(34.0009323065694,57.0210080582645,5.55520742261545));
#29848=CARTESIAN_POINT('Ctrl Pts',(33.8572048591017,57.3167826080678,5.5772984028737));
#29849=CARTESIAN_POINT('Ctrl Pts',(33.6174016975492,57.565870358533,5.59938938313195));
#29850=CARTESIAN_POINT('Ctrl Pts',(33.3311322154952,57.7328790961699,5.6214803633902));
#29851=CARTESIAN_POINT('Ctrl Pts',(33.3324736911222,57.73618752158,5.4285196366098));
#29852=CARTESIAN_POINT('Ctrl Pts',(33.7328589074961,57.5003618440874,5.39738001690346));
#29853=CARTESIAN_POINT('Ctrl Pts',(34.0365306675145,57.0908419490654,5.36624039719712));
#29854=CARTESIAN_POINT('Ctrl Pts',(34.1325589902306,56.6373526743003,5.33510077749077));
#29855=CARTESIAN_POINT('Ctrl Pts',(34.246801289078,56.0978487468504,5.29805481396809));
#29856=CARTESIAN_POINT('Ctrl Pts',(34.0671613149251,55.4961139999285,5.26100885044541));
#29857=CARTESIAN_POINT('Ctrl Pts',(33.6758523462208,55.1075357285356,5.22396288692273));
#29858=CARTESIAN_POINT('Ctrl Pts',(33.2845433775165,54.7189574571428,5.18691692340005));
#29859=CARTESIAN_POINT('Ctrl Pts',(32.6815654142609,54.543535661279,5.14987095987737));
#29860=CARTESIAN_POINT('Ctrl Pts',(32.1428747275693,54.6615531325857,5.11282499635469));
#29861=CARTESIAN_POINT('Ctrl Pts',(31.6041840408777,54.7795706038924,5.07577903283201));
#29862=CARTESIAN_POINT('Ctrl Pts',(31.12978063075,55.1910273423697,5.03873306930933));
#29863=CARTESIAN_POINT('Ctrl Pts',(30.9367779143554,55.7076178324787,5.00168710578665));
#29864=CARTESIAN_POINT('Ctrl Pts',(30.7437751979608,56.2242083225877,4.96464114226396));
#29865=CARTESIAN_POINT('Ctrl Pts',(30.8321731752993,56.8459325643283,4.92759517874128));
#29866=CARTESIAN_POINT('Ctrl Pts',(31.1615160075389,57.2882549360944,4.8905492152186));
#29867=CARTESIAN_POINT('Ctrl Pts',(31.4908588397784,57.7305773078605,4.85350325169592));
#29868=CARTESIAN_POINT('Ctrl Pts',(32.0611465269191,57.9934978096521,4.81645728817324));
#29869=CARTESIAN_POINT('Ctrl Pts',(32.6113836768238,57.956689381435,4.77941132465056));
#29870=CARTESIAN_POINT('Ctrl Pts',(32.8633454266668,57.93983425636,4.76244742863697));
#29871=CARTESIAN_POINT('Ctrl Pts',(33.1111028597659,57.8601301739612,4.74548353262339));
#29872=CARTESIAN_POINT('Ctrl Pts',(33.3313578105535,57.7323657066332,4.7285196366098));
#29873=CARTESIAN_POINT('Origin',(32.5,56.2916512459885,3.));
#29874=CARTESIAN_POINT('',(33.3342430690557,57.7335557705024,4.0285196366098));
#29875=CARTESIAN_POINT('',(33.3343740412804,57.7368429003791,4.2214803633902));
#29876=CARTESIAN_POINT('',(33.333,57.7344495686934,3.));
#29877=CARTESIAN_POINT('Ctrl Pts',(33.3343740344483,57.7368428884789,4.2214803633902));
#29878=CARTESIAN_POINT('Ctrl Pts',(32.8564950497481,58.0127845069312,4.25855045104913));
#29879=CARTESIAN_POINT('Ctrl Pts',(32.2282029771155,58.0281412318725,4.29562053870805));
#29880=CARTESIAN_POINT('Ctrl Pts',(31.7373727175272,57.7759553439527,4.33269062636698));
#29881=CARTESIAN_POINT('Ctrl Pts',(31.2468618760144,57.5239335712834,4.36973658988966));
#29882=CARTESIAN_POINT('Ctrl Pts',(30.8936340516087,57.0047173912526,4.40678255341235));
#29883=CARTESIAN_POINT('Ctrl Pts',(30.8393459612069,56.4559290322592,4.44382851693503));
#29884=CARTESIAN_POINT('Ctrl Pts',(30.7850578708051,55.9071406732657,4.48087448045771));
#29885=CARTESIAN_POINT('Ctrl Pts',(31.0297095144071,55.3287801353096,4.51792044398039));
#29886=CARTESIAN_POINT('Ctrl Pts',(31.4613346798115,54.9855373992054,4.55496640750307));
#29887=CARTESIAN_POINT('Ctrl Pts',(31.8929598452158,54.6422946631012,4.59201237102575));
#29888=CARTESIAN_POINT('Ctrl Pts',(32.5115585324225,54.5341697288488,4.62905833454843));
#29889=CARTESIAN_POINT('Ctrl Pts',(33.0340255450119,54.7106465835455,4.66610429807111));
#29890=CARTESIAN_POINT('Ctrl Pts',(33.5564925576013,54.8871234382422,4.70315026159379));
#29891=CARTESIAN_POINT('Ctrl Pts',(33.9828278955733,55.348202081888,4.74019622511647));
#29892=CARTESIAN_POINT('Ctrl Pts',(34.1179167730764,55.8828672630521,4.77724218863915));
#29893=CARTESIAN_POINT('Ctrl Pts',(34.2530056505794,56.4175324442162,4.81428815216183));
#29894=CARTESIAN_POINT('Ctrl Pts',(34.0968480676134,57.0257841628987,4.85133411568452));
#29895=CARTESIAN_POINT('Ctrl Pts',(33.7209104293741,57.4292525624064,4.8883800792072));
#29896=CARTESIAN_POINT('Ctrl Pts',(33.6089446308763,57.5494178688947,4.8994135072682));
#29897=CARTESIAN_POINT('Ctrl Pts',(33.4774836445333,57.6514182455857,4.9104469353292));
#29898=CARTESIAN_POINT('Ctrl Pts',(33.3337300498339,57.7328514726872,4.9214803633902));
#29899=CARTESIAN_POINT('Ctrl Pts',(33.3313578105535,57.7323657066332,4.7285196366098));
#29900=CARTESIAN_POINT('Ctrl Pts',(33.5920983142318,57.5811165681046,4.70843756910071));
#29901=CARTESIAN_POINT('Ctrl Pts',(33.8142965260144,57.3625150588492,4.68835550159161));
#29902=CARTESIAN_POINT('Ctrl Pts',(33.9593006043585,57.1010955378143,4.66827343408252));
#29903=CARTESIAN_POINT('Ctrl Pts',(34.2267937693199,56.6188474806365,4.63122747055984));
#29904=CARTESIAN_POINT('Ctrl Pts',(34.2315934865741,55.9908887245065,4.59418150703716));
#29905=CARTESIAN_POINT('Ctrl Pts',(33.9715031387158,55.5046081545499,4.55713554351448));
#29906=CARTESIAN_POINT('Ctrl Pts',(33.7114127908575,55.0183275845932,4.5200895799918));
#29907=CARTESIAN_POINT('Ctrl Pts',(33.1864323778867,54.6737252008098,4.48304361646911));
#29908=CARTESIAN_POINT('Ctrl Pts',(32.6368221624337,54.6285102383604,4.44599765294643));
#29909=CARTESIAN_POINT('Ctrl Pts',(32.0872119469807,54.5832952759111,4.40895168942375));
#29910=CARTESIAN_POINT('Ctrl Pts',(31.5129719290456,54.8374677347958,4.37190572590108));
#29911=CARTESIAN_POINT('Ctrl Pts',(31.1769063091028,55.2747041478526,4.3348597623784));
#29912=CARTESIAN_POINT('Ctrl Pts',(30.84084068916,55.7119405609094,4.29781379885572));
#29913=CARTESIAN_POINT('Ctrl Pts',(30.7429494672094,56.3322409281384,4.26076783533303));
#29914=CARTESIAN_POINT('Ctrl Pts',(30.9280331160056,56.8517212691839,4.22372187181035));
#29915=CARTESIAN_POINT('Ctrl Pts',(31.1131167648017,57.3712016102294,4.18667590828767));
#29916=CARTESIAN_POINT('Ctrl Pts',(31.5811752843444,57.7898619250913,4.14962994476499));
#29917=CARTESIAN_POINT('Ctrl Pts',(32.117999039119,57.9160999466831,4.11258398124231));
#29918=CARTESIAN_POINT('Ctrl Pts',(32.5240508086608,58.0115859820809,4.08456253303148));
#29919=CARTESIAN_POINT('Ctrl Pts',(32.9694456528715,57.939766662088,4.05654108482064));
#29920=CARTESIAN_POINT('Ctrl Pts',(33.3342430690557,57.7335557705024,4.0285196366098));
#29921=CARTESIAN_POINT('Origin',(32.5,56.2916512459885,3.));
#29922=CARTESIAN_POINT('',(33.3337922536522,57.7369224948681,3.3285196366098));
#29923=CARTESIAN_POINT('',(33.3312448475263,57.7342636967217,3.5214803633902));
#29924=CARTESIAN_POINT('',(33.333,57.7344495686934,3.));
#29925=CARTESIAN_POINT('Ctrl Pts',(33.3312448475263,57.7342636967217,3.5214803633902));
#29926=CARTESIAN_POINT('Ctrl Pts',(33.1882152402262,57.8184056914071,3.5325620397237));
#29927=CARTESIAN_POINT('Ctrl Pts',(33.0334203647077,57.8814418696117,3.5436437160572));
#29928=CARTESIAN_POINT('Ctrl Pts',(32.8726233824478,57.9182768459085,3.5547253923907));
#29929=CARTESIAN_POINT('Ctrl Pts',(32.3350802382442,58.0414159042228,3.59177135591338));
#29930=CARTESIAN_POINT('Ctrl Pts',(31.7304599472088,57.8717407985661,3.62881731943606));
#29931=CARTESIAN_POINT('Ctrl Pts',(31.3354704139632,57.4869043031699,3.66586328295874));
#29932=CARTESIAN_POINT('Ctrl Pts',(30.9404808807176,57.1020678077737,3.70290924648142));
#29933=CARTESIAN_POINT('Ctrl Pts',(30.7551221052618,56.5020699226381,3.7399552100041));
#29934=CARTESIAN_POINT('Ctrl Pts',(30.8642245822408,55.961503082106,3.77700117352678));
#29935=CARTESIAN_POINT('Ctrl Pts',(30.9733270592199,55.4209362415738,3.81404713704946));
#29936=CARTESIAN_POINT('Ctrl Pts',(31.3768907886337,54.9398004456451,3.85109310057214));
#29937=CARTESIAN_POINT('Ctrl Pts',(31.8902225413503,54.7382902195697,3.88813906409482));
#29938=CARTESIAN_POINT('Ctrl Pts',(32.4035542940669,54.5367799934943,3.9251850276175));
#29939=CARTESIAN_POINT('Ctrl Pts',(33.0266540700863,54.6148953372722,3.96223099114018));
#29940=CARTESIAN_POINT('Ctrl Pts',(33.4743567237047,54.9368863208444,3.99927695466286));
#29941=CARTESIAN_POINT('Ctrl Pts',(33.9220593773232,55.2588773044166,4.03632291818554));
#29942=CARTESIAN_POINT('Ctrl Pts',(34.1943649085407,55.824743927783,4.07336888170822));
#29943=CARTESIAN_POINT('Ctrl Pts',(34.1666511469031,56.3755141221476,4.1104148452309));
#29944=CARTESIAN_POINT('Ctrl Pts',(34.138955432321,56.9259256578637,4.14743668461733));
#29945=CARTESIAN_POINT('Ctrl Pts',(33.8116310396246,57.4612604196062,4.18445852400377));
#29946=CARTESIAN_POINT('Ctrl Pts',(33.3343740344483,57.7368428884789,4.2214803633902));
#29947=CARTESIAN_POINT('Ctrl Pts',(33.3342430690557,57.7335557705024,4.0285196366098));
#29948=CARTESIAN_POINT('Ctrl Pts',(33.4517287836878,57.6671440228089,4.01949512129796));
#29949=CARTESIAN_POINT('Ctrl Pts',(33.560854853963,57.5867930493783,4.01047060598611));
#29950=CARTESIAN_POINT('Ctrl Pts',(33.6576147739257,57.4936023059229,4.00144609067427));
#29951=CARTESIAN_POINT('Ctrl Pts',(34.0548177639512,57.1110509152493,3.96440012715159));
#29952=CARTESIAN_POINT('Ctrl Pts',(34.2436347539958,56.5121324055803,3.92735416362891));
#29953=CARTESIAN_POINT('Ctrl Pts',(34.137652577907,55.9709452289588,3.89030820010623));
#29954=CARTESIAN_POINT('Ctrl Pts',(34.0316704018183,55.4297580523373,3.85326223658355));
#29955=CARTESIAN_POINT('Ctrl Pts',(33.6308890595961,54.9463022087633,3.81621627306086));
#29956=CARTESIAN_POINT('Ctrl Pts',(33.11872840509,54.7418340064325,3.77917030953818));
#29957=CARTESIAN_POINT('Ctrl Pts',(32.6065677505839,54.5373658041018,3.7421243460155));
#29958=CARTESIAN_POINT('Ctrl Pts',(31.9830277837939,54.6118852430143,3.70507838249282));
#29959=CARTESIAN_POINT('Ctrl Pts',(31.5334751062351,54.9312880793963,3.66803241897014));
#29960=CARTESIAN_POINT('Ctrl Pts',(31.0839224286763,55.2506909157783,3.63098645544746));
#29961=CARTESIAN_POINT('Ctrl Pts',(30.8083570403488,55.8149771496297,3.59394049192478));
#29962=CARTESIAN_POINT('Ctrl Pts',(30.8328930037818,56.3658979863088,3.5568945284021));
#29963=CARTESIAN_POINT('Ctrl Pts',(30.8574289672149,56.9168188229878,3.51984856487942));
#29964=CARTESIAN_POINT('Ctrl Pts',(31.1820662824084,57.4543742624943,3.48280260135674));
#29965=CARTESIAN_POINT('Ctrl Pts',(31.6582328412459,57.7325490097912,3.44575663783406));
#29966=CARTESIAN_POINT('Ctrl Pts',(32.1343994000833,58.010723757088,3.40871067431137));
#29967=CARTESIAN_POINT('Ctrl Pts',(32.7620952025646,58.0295178121752,3.3716647107887));
#29968=CARTESIAN_POINT('Ctrl Pts',(33.2540517054067,57.7803299691728,3.33461874726602));
#29969=CARTESIAN_POINT('Ctrl Pts',(33.2810496728284,57.7666548470259,3.33258571038061));
#29970=CARTESIAN_POINT('Ctrl Pts',(33.3076388370087,57.7521726493388,3.33055267349521));
#29971=CARTESIAN_POINT('Ctrl Pts',(33.3337922536522,57.7369224948681,3.3285196366098));
#29972=CARTESIAN_POINT('Origin',(32.5,56.2916512459885,3.));
#29973=CARTESIAN_POINT('',(33.3310924906901,57.7334985910042,2.6285196366098));
#29974=CARTESIAN_POINT('',(33.3325882586834,57.7320513890704,2.8214803633902));
#29975=CARTESIAN_POINT('',(33.333,57.7344495686934,3.));
#29976=CARTESIAN_POINT('Ctrl Pts',(33.3325882586834,57.7320513890704,2.8214803633902));
#29977=CARTESIAN_POINT('Ctrl Pts',(33.0441865216604,57.8968038534098,2.84361959192095));
#29978=CARTESIAN_POINT('Ctrl Pts',(32.7077104550097,57.9799132231487,2.8657588204517));
#29979=CARTESIAN_POINT('Ctrl Pts',(32.3790127353428,57.9560193270484,2.88789804898244));
#29980=CARTESIAN_POINT('Ctrl Pts',(31.8289970147924,57.9160372471796,2.92494401250512));
#29981=CARTESIAN_POINT('Ctrl Pts',(31.3007606051993,57.5764468565745,2.9619899760278));
#29982=CARTESIAN_POINT('Ctrl Pts',(31.0360538947178,57.092663623102,2.99903593955048));
#29983=CARTESIAN_POINT('Ctrl Pts',(30.7713471842362,56.6088803896294,3.03608190307317));
#29984=CARTESIAN_POINT('Ctrl Pts',(30.7701701728664,55.9809043132895,3.07312786659585));
#29985=CARTESIAN_POINT('Ctrl Pts',(31.0330615265356,55.4961322062855,3.11017383011853));
#29986=CARTESIAN_POINT('Ctrl Pts',(31.2959528802049,55.0113600992815,3.14721979364121));
#29987=CARTESIAN_POINT('Ctrl Pts',(31.8229125989134,54.6697919616135,3.18426575716389));
#29988=CARTESIAN_POINT('Ctrl Pts',(32.3727745793293,54.6277483883085,3.22131172068657));
#29989=CARTESIAN_POINT('Ctrl Pts',(32.9226365597451,54.5857048150036,3.25835768420925));
#29990=CARTESIAN_POINT('Ctrl Pts',(33.4954008018683,54.8431858060618,3.29540364773193));
#29991=CARTESIAN_POINT('Ctrl Pts',(33.8289385024972,55.2823537259082,3.33244961125461));
#29992=CARTESIAN_POINT('Ctrl Pts',(34.162476203126,55.7215216457546,3.3694955747773));
#29993=CARTESIAN_POINT('Ctrl Pts',(34.2567873622605,56.3423764943892,3.40654153829998));
#29994=CARTESIAN_POINT('Ctrl Pts',(34.0687099431419,56.8607805298492,3.44358750182266));
#29995=CARTESIAN_POINT('Ctrl Pts',(33.9368927177428,57.2241127252305,3.46955178901184));
#29996=CARTESIAN_POINT('Ctrl Pts',(33.6663621789423,57.5371196140996,3.49551607620102));
#29997=CARTESIAN_POINT('Ctrl Pts',(33.3312448475263,57.7342636967217,3.5214803633902));
#29998=CARTESIAN_POINT('Ctrl Pts',(33.3337922536522,57.7369224948681,3.3285196366098));
#29999=CARTESIAN_POINT('Ctrl Pts',(33.7842059499452,57.4742845941374,3.29350670997253));
#30000=CARTESIAN_POINT('Ctrl Pts',(34.1053783658086,56.9838732473919,3.25849378333525));
#30001=CARTESIAN_POINT('Ctrl Pts',(34.1596784920807,56.465506410459,3.22348085669797));
#30002=CARTESIAN_POINT('Ctrl Pts',(34.2171315727097,55.9170404358397,3.18643489317529));
#30003=CARTESIAN_POINT('Ctrl Pts',(33.975820530765,55.3372782276934,3.14938892965261));
#30004=CARTESIAN_POINT('Ctrl Pts',(33.546182732919,54.9915512480536,3.11234296612993));
#30005=CARTESIAN_POINT('Ctrl Pts',(33.1165449350731,54.6458242684137,3.07529700260725));
#30006=CARTESIAN_POINT('Ctrl Pts',(32.498580381326,54.5341325172804,3.03825103908457));
#30007=CARTESIAN_POINT('Ctrl Pts',(31.9751040537975,54.7075923578949,3.00120507556189));
#30008=CARTESIAN_POINT('Ctrl Pts',(31.4516277262689,54.8810521985095,2.96415911203921));
#30009=CARTESIAN_POINT('Ctrl Pts',(31.0226396249589,55.3396636308718,2.92711314851653));
#30010=CARTESIAN_POINT('Ctrl Pts',(30.88446858696,55.8735405324579,2.89006718499385));
#30011=CARTESIAN_POINT('Ctrl Pts',(30.746297548961,56.4074174340438,2.85302122147117));
#30012=CARTESIAN_POINT('Ctrl Pts',(30.8989435742731,57.0165598048535,2.81597525794848));
#30013=CARTESIAN_POINT('Ctrl Pts',(31.2725473438504,57.4221901848135,2.7789292944258));
#30014=CARTESIAN_POINT('Ctrl Pts',(31.6461511134276,57.8278205647734,2.74188333090312));
#30015=CARTESIAN_POINT('Ctrl Pts',(32.24071262727,58.0299389538838,2.70483736738045));
#30016=CARTESIAN_POINT('Ctrl Pts',(32.7841274371744,57.9360447252789,2.66779140385776));
#30017=CARTESIAN_POINT('Ctrl Pts',(32.9761488965038,57.9028661911818,2.65470081477511));
#30018=CARTESIAN_POINT('Ctrl Pts',(33.1617839833806,57.8327263930767,2.64161022569246));
#30019=CARTESIAN_POINT('Ctrl Pts',(33.3310924906901,57.7334985910042,2.6285196366098));
#30020=CARTESIAN_POINT('Origin',(32.5,56.2916512459885,3.));
#30021=CARTESIAN_POINT('',(33.3331879029845,57.7323621350135,1.9285196366098));
#30022=CARTESIAN_POINT('',(33.3348622165511,57.7357255517677,2.12148036339019));
#30023=CARTESIAN_POINT('',(33.333,57.7344495686934,3.));
#30024=CARTESIAN_POINT('Ctrl Pts',(33.3348622165511,57.7357255517677,2.12148036339019));
#30025=CARTESIAN_POINT('Ctrl Pts',(32.9046875435881,57.9801160523425,2.15467714411819));
#30026=CARTESIAN_POINT('Ctrl Pts',(32.3567184702118,58.0261342906593,2.18787392484619));
#30027=CARTESIAN_POINT('Ctrl Pts',(31.8960497135599,57.8472871542167,2.22107070557419));
#30028=CARTESIAN_POINT('Ctrl Pts',(31.3819661915825,57.6477026057306,2.25811666909687));
#30029=CARTESIAN_POINT('Ctrl Pts',(30.9766017246916,57.1680829785327,2.29516263261955));
#30030=CARTESIAN_POINT('Ctrl Pts',(30.8654736597327,56.6279289146384,2.33220859614223));
#30031=CARTESIAN_POINT('Ctrl Pts',(30.7543455947739,56.087774850744,2.36925455966492));
#30032=CARTESIAN_POINT('Ctrl Pts',(30.9374539317471,55.4870863501531,2.4063005231876));
#30033=CARTESIAN_POINT('Ctrl Pts',(31.3309981019417,55.1007719112967,2.44334648671028));
#30034=CARTESIAN_POINT('Ctrl Pts',(31.7245422721362,54.7144574724402,2.48039245023296));
#30035=CARTESIAN_POINT('Ctrl Pts',(32.3285222755522,54.5425170953181,2.51743841375564));
#30036=CARTESIAN_POINT('Ctrl Pts',(32.8665232388266,54.6636402684886,2.55448437727832));
#30037=CARTESIAN_POINT('Ctrl Pts',(33.404524202101,54.7847634416591,2.591530340801));
#30038=CARTESIAN_POINT('Ctrl Pts',(33.876546125234,55.1989501651222,2.62857630432368));
#30039=CARTESIAN_POINT('Ctrl Pts',(34.0665654985573,55.7166455362864,2.66562226784636));
#30040=CARTESIAN_POINT('Ctrl Pts',(34.2565848718806,56.2343409074507,2.70266823136904));
#30041=CARTESIAN_POINT('Ctrl Pts',(34.1646016953943,56.8555449263162,2.73971419489172));
#30042=CARTESIAN_POINT('Ctrl Pts',(33.8327125913974,57.2959600511828,2.7767601584144));
#30043=CARTESIAN_POINT('Ctrl Pts',(33.6991654394395,57.4731764312833,2.79166689340633));
#30044=CARTESIAN_POINT('Ctrl Pts',(33.5267742601986,57.6211206345609,2.80657362839827));
#30045=CARTESIAN_POINT('Ctrl Pts',(33.3325882586834,57.7320513890704,2.8214803633902));
#30046=CARTESIAN_POINT('Ctrl Pts',(33.3310924906901,57.7334985910042,2.6285196366098));
#30047=CARTESIAN_POINT('Ctrl Pts',(33.6409218393061,57.5519147723922,2.60456426216977));
#30048=CARTESIAN_POINT('Ctrl Pts',(33.8960769478414,57.272921419479,2.58060888772975));
#30049=CARTESIAN_POINT('Ctrl Pts',(34.0356424650284,56.9447672654595,2.55665351328972));
#30050=CARTESIAN_POINT('Ctrl Pts',(34.2514745770115,56.4372908805649,2.51960754976704));
#30051=CARTESIAN_POINT('Ctrl Pts',(34.190870695011,55.8122449570956,2.48256158624436));
#30052=CARTESIAN_POINT('Ctrl Pts',(33.8815665292719,55.3556853061788,2.44551562272168));
#30053=CARTESIAN_POINT('Ctrl Pts',(33.5722623635328,54.899125655262,2.408469659199));
#30054=CARTESIAN_POINT('Ctrl Pts',(33.0142579140551,54.6110522768978,2.37142369567632));
#30055=CARTESIAN_POINT('Ctrl Pts',(32.4629270812427,54.6233035861816,2.33437773215364));
#30056=CARTESIAN_POINT('Ctrl Pts',(31.9115962484303,54.6355548954655,2.29733176863096));
#30057=CARTESIAN_POINT('Ctrl Pts',(31.3669390322832,54.9481308923974,2.26028580510828));
#30058=CARTESIAN_POINT('Ctrl Pts',(31.0782208961876,55.417979399555,2.2232398415856));
#30059=CARTESIAN_POINT('Ctrl Pts',(30.789502760092,55.8878279067126,2.18619387806292));
#30060=CARTESIAN_POINT('Ctrl Pts',(30.7567237040478,56.514948924096,2.14914791454024));
#30061=CARTESIAN_POINT('Ctrl Pts',(30.9948852489236,57.0123369620816,2.11210195101756));
#30062=CARTESIAN_POINT('Ctrl Pts',(31.2330467937995,57.5097250000671,2.07505598749488));
#30063=CARTESIAN_POINT('Ctrl Pts',(31.7421489395953,57.8773800586549,2.0380100239722));
#30064=CARTESIAN_POINT('Ctrl Pts',(32.2891982024821,57.9470427155363,2.00096406044951));
#30065=CARTESIAN_POINT('Ctrl Pts',(32.6457882768413,57.9924518106263,1.97681591916961));
#30066=CARTESIAN_POINT('Ctrl Pts',(33.0185020402459,57.9112442562479,1.95266777788971));
#30067=CARTESIAN_POINT('Ctrl Pts',(33.3331879029845,57.7323621350135,1.9285196366098));
#30068=CARTESIAN_POINT('Origin',(32.5,56.2916512459885,3.));
#30069=CARTESIAN_POINT('',(33.3347215376785,57.7364302140763,1.2285196366098));
#30070=CARTESIAN_POINT('',(33.3320718525009,57.735759463036,1.4214803633902));
#30071=CARTESIAN_POINT('',(33.333,57.7344495686934,3.));
#30072=CARTESIAN_POINT('Ctrl Pts',(33.3320718525009,57.735759463036,1.4214803633902));
#30073=CARTESIAN_POINT('Ctrl Pts',(33.2393317234316,57.7904422794385,1.42868873279277));
#30074=CARTESIAN_POINT('Ctrl Pts',(33.1414800191062,57.8359234203097,1.43589710219533));
#30075=CARTESIAN_POINT('Ctrl Pts',(33.0399483052832,57.8706429670186,1.4431054715979));
#30076=CARTESIAN_POINT('Ctrl Pts',(32.5181465001006,58.0490770883944,1.48015143512058));
#30077=CARTESIAN_POINT('Ctrl Pts',(31.8991468445915,57.9432717752442,1.51719739864326));
#30078=CARTESIAN_POINT('Ctrl Pts',(31.4662380410665,57.6016494290874,1.55424336216595));
#30079=CARTESIAN_POINT('Ctrl Pts',(31.0333292375416,57.2600270829306,1.59128932568863));
#30080=CARTESIAN_POINT('Ctrl Pts',(30.7865112860008,56.6825877037672,1.62833528921131));
#30081=CARTESIAN_POINT('Ctrl Pts',(30.8387418215197,56.1335996977757,1.66538125273399));
#30082=CARTESIAN_POINT('Ctrl Pts',(30.8909723570387,55.5846116917841,1.70242721625667));
#30083=CARTESIAN_POINT('Ctrl Pts',(31.2422513796173,55.0640750589644,1.73947317977935));
#30084=CARTESIAN_POINT('Ctrl Pts',(31.731814052685,54.8102163409698,1.77651914330203));
#30085=CARTESIAN_POINT('Ctrl Pts',(32.2213767257528,54.5563576229752,1.81356510682471));
#30086=CARTESIAN_POINT('Ctrl Pts',(32.8492230493096,54.5691768198056,1.85061107034739));
#30087=CARTESIAN_POINT('Ctrl Pts',(33.3280155932489,54.842807153342,1.88765703387007));
#30088=CARTESIAN_POINT('Ctrl Pts',(33.8068081371882,55.1164374868783,1.92470299739275));
#30089=CARTESIAN_POINT('Ctrl Pts',(34.1365469015101,55.6508789571206,1.96174896091543));
#30090=CARTESIAN_POINT('Ctrl Pts',(34.1663250709766,56.2015413947231,1.99879492443811));
#30091=CARTESIAN_POINT('Ctrl Pts',(34.1961032404431,56.7522038323256,2.03584088796079));
#30092=CARTESIAN_POINT('Ctrl Pts',(33.9259208150542,57.3190872372884,2.07288685148347));
#30093=CARTESIAN_POINT('Ctrl Pts',(33.4794283138278,57.6427542048827,2.10993281500615));
#30094=CARTESIAN_POINT('Ctrl Pts',(33.4330364511186,57.6763841392778,2.11378199780083));
#30095=CARTESIAN_POINT('Ctrl Pts',(33.384741178112,57.7073883549261,2.11763118059551));
#30096=CARTESIAN_POINT('Ctrl Pts',(33.3348622165511,57.7357255517677,2.12148036339019));
#30097=CARTESIAN_POINT('Ctrl Pts',(33.3331879029845,57.7323621350135,1.9285196366098));
#30098=CARTESIAN_POINT('Ctrl Pts',(33.501265531522,57.6368189718628,1.91562181436702));
#30099=CARTESIAN_POINT('Ctrl Pts',(33.6527891880219,57.5134115911553,1.90272399212425));
#30100=CARTESIAN_POINT('Ctrl Pts',(33.7764604319637,57.3665498834978,1.88982616988147));
#30101=CARTESIAN_POINT('Ctrl Pts',(34.1316770185806,56.9447241394031,1.85278020635879));
#30102=CARTESIAN_POINT('Ctrl Pts',(34.2571138118367,56.3294023960388,1.81573424283611));
#30103=CARTESIAN_POINT('Ctrl Pts',(34.0953639520231,55.8021901383674,1.77868827931343));
#30104=CARTESIAN_POINT('Ctrl Pts',(33.9336140922095,55.2749778806959,1.74164231579075));
#30105=CARTESIAN_POINT('Ctrl Pts',(33.4846775793261,54.8358751087172,1.70459635226807));
#30106=CARTESIAN_POINT('Ctrl Pts',(32.9540127541378,54.6858396959092,1.66755038874539));
#30107=CARTESIAN_POINT('Ctrl Pts',(32.4233479289494,54.5358042831012,1.63050442522271));
#30108=CARTESIAN_POINT('Ctrl Pts',(31.8109547914561,54.6748362294637,1.59345846170003));
#30109=CARTESIAN_POINT('Ctrl Pts',(31.3970985335358,55.0393067763799,1.55641249817735));
#30110=CARTESIAN_POINT('Ctrl Pts',(30.9832422756156,55.4037773232961,1.51936653465467));
#30111=CARTESIAN_POINT('Ctrl Pts',(30.7679228972685,55.993686470766,1.48232057113199));
#30112=CARTESIAN_POINT('Ctrl Pts',(30.8496825329409,56.5390589524362,1.44527460760931));
#30113=CARTESIAN_POINT('Ctrl Pts',(30.9314421686133,57.0844314341065,1.40822864408663));
#30114=CARTESIAN_POINT('Ctrl Pts',(31.3102808183052,57.5852672499772,1.37118268056395));
#30115=CARTESIAN_POINT('Ctrl Pts',(31.8128208258201,57.8123560489854,1.33413671704127));
#30116=CARTESIAN_POINT('Ctrl Pts',(32.2903969982888,58.0281641395237,1.29893102356411));
#30117=CARTESIAN_POINT('Ctrl Pts',(32.8796899699103,57.9967466454787,1.26372533008696));
#30118=CARTESIAN_POINT('Ctrl Pts',(33.3347215376785,57.7364302140763,1.2285196366098));
#30119=CARTESIAN_POINT('Origin',(32.5,56.2916512459885,3.));
#30120=CARTESIAN_POINT('',(33.3315625259448,57.7350035902351,0.5285196366098));
#30121=CARTESIAN_POINT('',(33.3315934922344,57.7321400761417,0.721480363390196));
#30122=CARTESIAN_POINT('',(33.333,57.7344495686934,3.));
#30123=CARTESIAN_POINT('Ctrl Pts',(33.3315934922344,57.7321400761417,0.721480363390196));
#30124=CARTESIAN_POINT('Ctrl Pts',(33.094172273388,57.8693226291885,0.739746284990015));
#30125=CARTESIAN_POINT('Ctrl Pts',(32.8247195065089,57.9509431527901,0.758012206589833));
#30126=CARTESIAN_POINT('Ctrl Pts',(32.552949516444,57.9595707213043,0.776278128189651));
#30127=CARTESIAN_POINT('Ctrl Pts',(32.001760183703,57.97706869351,0.813324091712332));
#30128=CARTESIAN_POINT('Ctrl Pts',(31.4410392363067,57.6943190569764,0.850370055235013));
#30129=CARTESIAN_POINT('Ctrl Pts',(31.1274037953482,57.2407237861293,0.887416018757693));
#30130=CARTESIAN_POINT('Ctrl Pts',(30.8137683543896,56.7871285152823,0.924461982280374));
#30131=CARTESIAN_POINT('Ctrl Pts',(30.7472184198688,56.1626876101218,0.961507945803055));
#30132=CARTESIAN_POINT('Ctrl Pts',(30.9582109466764,55.6531799917321,0.998553909325736));
#30133=CARTESIAN_POINT('Ctrl Pts',(31.169203473484,55.1436723733423,1.03559987284842));
#30134=CARTESIAN_POINT('Ctrl Pts',(31.6577384616201,54.7490980417232,1.0726458363711));
#30135=CARTESIAN_POINT('Ctrl Pts',(32.2002351035856,54.6500361771206,1.10969179989378));
#30136=CARTESIAN_POINT('Ctrl Pts',(32.742731745551,54.550974312518,1.14673776341646));
#30137=CARTESIAN_POINT('Ctrl Pts',(33.339190041346,54.7474249149318,1.18378372693914));
#30138=CARTESIAN_POINT('Ctrl Pts',(33.7166374697496,55.1494812522208,1.22082969046182));
#30139=CARTESIAN_POINT('Ctrl Pts',(34.0940848981533,55.5515375895099,1.2578756539845));
#30140=CARTESIAN_POINT('Ctrl Pts',(34.2525214591656,56.1591996616742,1.29492161750718));
#30141=CARTESIAN_POINT('Ctrl Pts',(34.1194377622437,56.6943674757074,1.33196758102986));
#30142=CARTESIAN_POINT('Ctrl Pts',(34.0122493682821,57.1254028302473,1.36180517514997));
#30143=CARTESIAN_POINT('Ctrl Pts',(33.7159509484902,57.5094109520148,1.39164276927008));
#30144=CARTESIAN_POINT('Ctrl Pts',(33.3320718525009,57.735759463036,1.4214803633902));
#30145=CARTESIAN_POINT('Ctrl Pts',(33.3347215376785,57.7364302140763,1.2285196366098));
#30146=CARTESIAN_POINT('Ctrl Pts',(33.3585069224055,57.7228229680956,1.22667936656428));
#30147=CARTESIAN_POINT('Ctrl Pts',(33.3819254571596,57.7085902886951,1.22483909651875));
#30148=CARTESIAN_POINT('Ctrl Pts',(33.4049420099642,57.6937347933887,1.22299882647322));
#30149=CARTESIAN_POINT('Ctrl Pts',(33.8682818212557,57.394682956638,1.18595286295054));
#30150=CARTESIAN_POINT('Ctrl Pts',(34.1687200785007,56.8432375009908,1.14890689942786));
#30151=CARTESIAN_POINT('Ctrl Pts',(34.1687595096553,56.2917705661426,1.11186093590518));
#30152=CARTESIAN_POINT('Ctrl Pts',(34.1687989408099,55.7403036312943,1.0748149723825));
#30153=CARTESIAN_POINT('Ctrl Pts',(33.8684395458741,55.188815217245,1.03776900885982));
#30154=CARTESIAN_POINT('Ctrl Pts',(33.4051425051238,54.8896971238163,1.00072304533714));
#30155=CARTESIAN_POINT('Ctrl Pts',(32.9418454643735,54.5905790303876,0.963677081814459));
#30156=CARTESIAN_POINT('Ctrl Pts',(32.3156107778087,54.5438312575796,0.926631118291778));
#30157=CARTESIAN_POINT('Ctrl Pts',(31.8130383006683,54.7708481887354,0.889585154769097));
#30158=CARTESIAN_POINT('Ctrl Pts',(31.310465823528,54.9978651198912,0.852539191246416));
#30159=CARTESIAN_POINT('Ctrl Pts',(30.9315555558121,55.4986467550108,0.815493227723736));
#30160=CARTESIAN_POINT('Ctrl Pts',(30.8497179302269,56.0440075390777,0.778447264201056));
#30161=CARTESIAN_POINT('Ctrl Pts',(30.7678803046417,56.5893683231447,0.741401300678375));
#30162=CARTESIAN_POINT('Ctrl Pts',(30.9831153211871,57.179308256159,0.704355337155694));
#30163=CARTESIAN_POINT('Ctrl Pts',(31.3969194538394,57.543837982747,0.667309373633013));
#30164=CARTESIAN_POINT('Ctrl Pts',(31.8107235864917,57.9083677093349,0.630263410110333));
#30165=CARTESIAN_POINT('Ctrl Pts',(32.423096835251,58.0474872294965,0.593217446587652));
#30166=CARTESIAN_POINT('Ctrl Pts',(32.9537831109001,57.8975277056554,0.556171483064972));
#30167=CARTESIAN_POINT('Ctrl Pts',(33.0858213863713,57.860216778603,0.546954200913248));
#30168=CARTESIAN_POINT('Ctrl Pts',(33.2128028501901,57.805010485588,0.537736918761524));
#30169=CARTESIAN_POINT('Ctrl Pts',(33.3315625259448,57.7350035902351,0.5285196366098));
#30170=CARTESIAN_POINT('Origin',(32.5,56.2916512459885,3.));
#30171=CARTESIAN_POINT('',(33.332066590478,57.7319806121586,-0.171480363390199));
#30172=CARTESIAN_POINT('',(33.3345107245665,57.7340829700271,0.0214803633901963));
#30173=CARTESIAN_POINT('',(33.333,57.7344495686934,3.));
#30174=CARTESIAN_POINT('Ctrl Pts',(33.3345107245665,57.7340829700271,0.0214803633901963));
#30175=CARTESIAN_POINT('Ctrl Pts',(32.9530815922346,57.9496325625699,0.0508038371872645));
#30176=CARTESIAN_POINT('Ctrl Pts',(32.482446188026,58.016467684898,0.0801273109843327));
#30177=CARTESIAN_POINT('Ctrl Pts',(32.0612908438827,57.9017112764627,0.109450784781401));
#30178=CARTESIAN_POINT('Ctrl Pts',(31.5292220438323,57.7567331694926,0.146496748304082));
#30179=CARTESIAN_POINT('Ctrl Pts',(31.0761267049973,57.3219229222043,0.183542711826762));
#30180=CARTESIAN_POINT('Ctrl Pts',(30.9093664792402,56.796273907743,0.220588675349443));
#30181=CARTESIAN_POINT('Ctrl Pts',(30.7426062534831,56.2706248932818,0.257634638872123));
#30182=CARTESIAN_POINT('Ctrl Pts',(30.8621811408039,55.6541371116476,0.294680602394804));
#30183=CARTESIAN_POINT('Ctrl Pts',(31.2133670155729,55.2289496928674,0.331726565917484));
#30184=CARTESIAN_POINT('Ctrl Pts',(31.5645528903419,54.8037622740873,0.368772529440165));
#30185=CARTESIAN_POINT('Ctrl Pts',(32.1473497525593,54.5698752181613,0.405818492962845));
#30186=CARTESIAN_POINT('Ctrl Pts',(32.6950373137549,54.6343282619421,0.442864456485526));
#30187=CARTESIAN_POINT('Ctrl Pts',(33.2427248749505,54.6987813057228,0.479910420008206));
#30188=CARTESIAN_POINT('Ctrl Pts',(33.7553031351243,55.0615744492104,0.516956383530887));
#30189=CARTESIAN_POINT('Ctrl Pts',(33.9981877468876,55.5566733533726,0.554002347053568));
#30190=CARTESIAN_POINT('Ctrl Pts',(34.2410723586509,56.0517722575349,0.591048310576249));
#30191=CARTESIAN_POINT('Ctrl Pts',(34.2142633220036,56.6791769223718,0.628094274098929));
#30192=CARTESIAN_POINT('Ctrl Pts',(33.9300299446371,57.1517520452627,0.66514023762161));
#30193=CARTESIAN_POINT('Ctrl Pts',(33.7859409742004,57.3913187827875,0.683920279544472));
#30194=CARTESIAN_POINT('Ctrl Pts',(33.5756972687095,57.591096325175,0.702700321467334));
#30195=CARTESIAN_POINT('Ctrl Pts',(33.3315934922344,57.7321400761417,0.721480363390196));
#30196=CARTESIAN_POINT('Ctrl Pts',(33.3315625259448,57.7350035902351,0.5285196366098));
#30197=CARTESIAN_POINT('Ctrl Pts',(33.6901199750815,57.523639811577,0.500690955238843));
#30198=CARTESIAN_POINT('Ctrl Pts',(33.9737318881584,57.1773614538062,0.472862273867886));
#30199=CARTESIAN_POINT('Ctrl Pts',(34.0952939407749,56.781340492839,0.44503359249693));
#30200=CARTESIAN_POINT('Ctrl Pts',(34.2571191924618,56.2541513717075,0.407987628974249));
#30201=CARTESIAN_POINT('Ctrl Pts',(34.1317703932969,55.6388116972881,0.370941665451569));
#30202=CARTESIAN_POINT('Ctrl Pts',(33.7766141338562,55.2169351595517,0.333895701928889));
#30203=CARTESIAN_POINT('Ctrl Pts',(33.4214578744154,54.7950586218153,0.296849738406208));
#30204=CARTESIAN_POINT('Ctrl Pts',(32.8364941546988,54.566645220762,0.259803774883528));
#30205=CARTESIAN_POINT('Ctrl Pts',(32.289434934298,54.636229647045,0.222757811360847));
#30206=CARTESIAN_POINT('Ctrl Pts',(31.7423757138972,54.705814073328,0.185711847838166));
#30207=CARTESIAN_POINT('Ctrl Pts',(31.2332209928121,55.0733963269474,0.148665884315486));
#30208=CARTESIAN_POINT('Ctrl Pts',(30.9949883236289,55.5707503002861,0.111619920792805));
#30209=CARTESIAN_POINT('Ctrl Pts',(30.7567556544457,56.0681042736248,0.0745739572701246));
#30210=CARTESIAN_POINT('Ctrl Pts',(30.7894450371643,56.6952299666827,0.0375279937474443));
#30211=CARTESIAN_POINT('Ctrl Pts',(31.0780959757366,57.1651197597709,0.000482030224763866));
#30212=CARTESIAN_POINT('Ctrl Pts',(31.3667469143089,57.635009552859,-0.0365639332979165));
#30213=CARTESIAN_POINT('Ctrl Pts',(31.9113594087348,57.9476634459773,-0.073609896820597));
#30214=CARTESIAN_POINT('Ctrl Pts',(32.4626884920092,57.9599935925982,-0.110655860343278));
#30215=CARTESIAN_POINT('Ctrl Pts',(32.7644246265901,57.9667417415587,-0.130930694692251));
#30216=CARTESIAN_POINT('Ctrl Pts',(33.0681725463472,57.8835354694765,-0.151205529041225));
#30217=CARTESIAN_POINT('Ctrl Pts',(33.332066590478,57.7319806121586,-0.171480363390199));
#30218=CARTESIAN_POINT('Origin',(32.5,56.2916512459885,3.));
#30219=CARTESIAN_POINT('',(33.3347877909358,57.7349452754743,-0.871480363390197));
#30220=CARTESIAN_POINT('',(33.3333524836119,57.7367881187288,-0.678519636609802));
#30221=CARTESIAN_POINT('',(33.333,57.7344495686934,3.));
#30222=CARTESIAN_POINT('Ctrl Pts',(33.3333524836119,57.7367881187288,-0.678519636609802));
#30223=CARTESIAN_POINT('Ctrl Pts',(33.2904764567157,57.7619047682301,-0.675184574138165));
#30224=CARTESIAN_POINT('Ctrl Pts',(33.2464522145773,57.7849807415505,-0.671849511666528));
#30225=CARTESIAN_POINT('Ctrl Pts',(33.201404681754,57.8058476261432,-0.66851444919489));
#30226=CARTESIAN_POINT('Ctrl Pts',(32.701015477069,58.0376375407333,-0.631468485672209));
#30227=CARTESIAN_POINT('Ctrl Pts',(32.0743642145054,57.9968518393257,-0.594422522149529));
#30228=CARTESIAN_POINT('Ctrl Pts',(31.608241296104,57.7021565859588,-0.557376558626848));
#30229=CARTESIAN_POINT('Ctrl Pts',(31.1421183777026,57.407461332592,-0.520330595104168));
#30230=CARTESIAN_POINT('Ctrl Pts',(30.8365238034633,56.8588565272658,-0.483284631581487));
#30231=CARTESIAN_POINT('Ctrl Pts',(30.8313147141678,56.3074141411014,-0.446238668058807));
#30232=CARTESIAN_POINT('Ctrl Pts',(30.8261056248723,55.7559717549371,-0.409192704536126));
#30233=CARTESIAN_POINT('Ctrl Pts',(31.1212820205206,55.2016917879345,-0.372146741013446));
#30234=CARTESIAN_POINT('Ctrl Pts',(31.5817547242443,54.8982436746825,-0.335100777490766));
#30235=CARTESIAN_POINT('Ctrl Pts',(32.0422274279679,54.5947955614305,-0.298054813968085));
#30236=CARTESIAN_POINT('Ctrl Pts',(32.6679964397669,54.5421793019291,-0.261008850445404));
#30237=CARTESIAN_POINT('Ctrl Pts',(33.1726750359156,54.7644749931934,-0.223962886922724));
#30238=CARTESIAN_POINT('Ctrl Pts',(33.6773536320643,54.9867706844577,-0.186916923400043));
#30239=CARTESIAN_POINT('Ctrl Pts',(34.0609418125626,55.4839783264877,-0.149870959877363));
#30240=CARTESIAN_POINT('Ctrl Pts',(34.1478882650457,56.0285480388725,-0.112824996354682));
#30241=CARTESIAN_POINT('Ctrl Pts',(34.2348347175289,56.5731177512574,-0.0757790328320021));
#30242=CARTESIAN_POINT('Ctrl Pts',(34.0251394419968,57.1650495339971,-0.0387330693093216));
#30243=CARTESIAN_POINT('Ctrl Pts',(33.6147706735978,57.5334424420409,-0.00168710578664105));
#30244=CARTESIAN_POINT('Ctrl Pts',(33.529226438914,57.6102365155873,0.00603538393897141));
#30245=CARTESIAN_POINT('Ctrl Pts',(33.434962075449,57.6773168608924,0.0137578736645838));
#30246=CARTESIAN_POINT('Ctrl Pts',(33.3345107245665,57.7340829700271,0.0214803633901963));
#30247=CARTESIAN_POINT('Ctrl Pts',(33.332066590478,57.7319806121586,-0.171480363390199));
#30248=CARTESIAN_POINT('Ctrl Pts',(33.550356960999,57.6066160323434,-0.188251492563906));
#30249=CARTESIAN_POINT('Ctrl Pts',(33.7413776202381,57.4344844529175,-0.205022621737613));
#30250=CARTESIAN_POINT('Ctrl Pts',(33.8814326840108,57.2278147357495,-0.22179375091132));
#30251=CARTESIAN_POINT('Ctrl Pts',(34.1908021206151,56.7712993321564,-0.258839714434));
#30252=CARTESIAN_POINT('Ctrl Pts',(34.251495321701,56.1462621248467,-0.29588567795668));
#30253=CARTESIAN_POINT('Ctrl Pts',(34.0357358154562,55.638754858791,-0.33293164147936));
#30254=CARTESIAN_POINT('Ctrl Pts',(33.8199763092115,55.1312475927353,-0.369977605002041));
#30255=CARTESIAN_POINT('Ctrl Pts',(33.3277640956362,54.7412702679337,-0.407023568524722));
#30256=CARTESIAN_POINT('Ctrl Pts',(32.7843626547691,54.6472983719835,-0.444069532047402));
#30257=CARTESIAN_POINT('Ctrl Pts',(32.2409612139021,54.5533264760334,-0.481115495570083));
#30258=CARTESIAN_POINT('Ctrl Pts',(31.6463705457434,54.7553600089348,-0.518161459092763));
#30259=CARTESIAN_POINT('Ctrl Pts',(31.2727089000175,55.1609368730463,-0.555207422615444));
#30260=CARTESIAN_POINT('Ctrl Pts',(30.8990472542916,55.5665137371577,-0.592253386138124));
#30261=CARTESIAN_POINT('Ctrl Pts',(30.7463146309986,56.1756339324792,-0.629299349660805));
#30262=CARTESIAN_POINT('Ctrl Pts',(30.8844090678351,56.7095307561729,-0.666345313183486));
#30263=CARTESIAN_POINT('Ctrl Pts',(31.0225035046717,57.2434275798666,-0.703391276706166));
#30264=CARTESIAN_POINT('Ctrl Pts',(31.4514250016378,57.7021010319325,-0.740437240228847));
#30265=CARTESIAN_POINT('Ctrl Pts',(31.9748770216296,57.8756353949644,-0.777483203751527));
#30266=CARTESIAN_POINT('Ctrl Pts',(32.4175973471179,58.0224056561357,-0.80881559029775));
#30267=CARTESIAN_POINT('Ctrl Pts',(32.9279379927888,57.9652079725634,-0.840147976843973));
#30268=CARTESIAN_POINT('Ctrl Pts',(33.3347877909358,57.7349452754743,-0.871480363390197));
#30269=CARTESIAN_POINT('Origin',(32.5,56.2916512459885,3.));
#30270=CARTESIAN_POINT('',(33.332685602761,57.7363329907929,-1.5714803633902));
#30271=CARTESIAN_POINT('',(33.3311039683456,57.7330494773494,-1.3785196366098));
#30272=CARTESIAN_POINT('',(33.333,57.7344495686934,3.));
#30273=CARTESIAN_POINT('',(30.9307125467392,55.7322829513575,-2.));
#30274=CARTESIAN_POINT('Ctrl Pts',(33.332685602761,57.7363329907929,-1.5714803633902));
#30275=CARTESIAN_POINT('Ctrl Pts',(33.7401458440335,57.4965393115171,-1.60318235169209));
#30276=CARTESIAN_POINT('Ctrl Pts',(34.046614399938,57.0758524794489,-1.63488433999398));
#30277=CARTESIAN_POINT('Ctrl Pts',(34.1374824480444,56.6126749242948,-1.66658632829587));
#30278=CARTESIAN_POINT('Ctrl Pts',(34.2436680400479,56.0714199515982,-1.70363229181855));
#30279=CARTESIAN_POINT('Ctrl Pts',(34.0554395585675,55.472141614315,-1.74067825534123));
#30280=CARTESIAN_POINT('Ctrl Pts',(33.6580205398159,55.0897022763625,-1.77772421886391));
#30281=CARTESIAN_POINT('Ctrl Pts',(33.2606015210643,54.70726293841,-1.81477018238659));
#30282=CARTESIAN_POINT('Ctrl Pts',(32.6539919650415,54.5416625997882,-1.85181614590927));
#30283=CARTESIAN_POINT('Ctrl Pts',(32.1180205379334,54.6674612497455,-1.88886210943196));
#30284=CARTESIAN_POINT('Ctrl Pts',(31.5820491108253,54.7932598997029,-1.92590807295464));
#30285=CARTESIAN_POINT('Ctrl Pts',(31.116715812632,55.2104575382394,-1.96295403647732));
#30286=CARTESIAN_POINT('Ctrl Pts',(30.9307125467392,55.7322829513575,-2.));
#30287=CARTESIAN_POINT('',(32.1993827818326,57.933381219007,-1.99999999999999));
#30288=CARTESIAN_POINT('Origin',(32.5,56.2916512459885,-2.));
#30289=CARTESIAN_POINT('Ctrl Pts',(32.1993825459686,57.9333829869217,-1.99999999999999));
#30290=CARTESIAN_POINT('Ctrl Pts',(31.6675596070896,57.835293698039,-1.96367708181444));
#30291=CARTESIAN_POINT('Ctrl Pts',(31.1868214355218,57.4546983693859,-1.92735416362889));
#30292=CARTESIAN_POINT('Ctrl Pts',(30.9706018866112,56.9589951265537,-1.89103124544334));
#30293=CARTESIAN_POINT('Ctrl Pts',(30.7500782634565,56.4534243968501,-1.85398528192066));
#30294=CARTESIAN_POINT('Ctrl Pts',(30.8047091132838,55.8281174567283,-1.81693931839798));
#30295=CARTESIAN_POINT('Ctrl Pts',(31.1096921022323,55.3687479433185,-1.7798933548753));
#30296=CARTESIAN_POINT('Ctrl Pts',(31.4146750911809,54.9093784299087,-1.74284739135262));
#30297=CARTESIAN_POINT('Ctrl Pts',(31.9700102192507,54.6159463432109,-1.70580142782994));
#30298=CARTESIAN_POINT('Ctrl Pts',(32.521445594378,54.6229937951642,-1.66875546430726));
#30299=CARTESIAN_POINT('Ctrl Pts',(33.0728809695053,54.6300412471175,-1.63170950078458));
#30300=CARTESIAN_POINT('Ctrl Pts',(33.62041659169,54.9375682377219,-1.5946635372619));
#30301=CARTESIAN_POINT('Ctrl Pts',(33.9135196580232,55.4047071572134,-1.55761757373922));
#30302=CARTESIAN_POINT('Ctrl Pts',(34.2066227243565,55.8718460767048,-1.52057161021654));
#30303=CARTESIAN_POINT('Ctrl Pts',(34.2452932348383,56.4985969250833,-1.48352564669386));
#30304=CARTESIAN_POINT('Ctrl Pts',(34.0118083132187,56.9981869719763,-1.44647968317118));
#30305=CARTESIAN_POINT('Ctrl Pts',(33.869033908706,57.3036828084989,-1.42382633431739));
#30306=CARTESIAN_POINT('Ctrl Pts',(33.6244941277173,57.5616302028089,-1.4011729854636));
#30307=CARTESIAN_POINT('Ctrl Pts',(33.3311039683456,57.7330494773494,-1.3785196366098));
#30308=CARTESIAN_POINT('Origin',(32.5,56.2916512459885,-3.54592528053767));
#30309=CARTESIAN_POINT('',(33.5275749112977,58.0738535198176,6.54592528053768));
#30310=CARTESIAN_POINT('',(33.5264962288793,58.0679896197986,6.60407471946233));
#30311=CARTESIAN_POINT('',(33.5273749999999,58.0711169444147,-3.54592528053767));
#30312=CARTESIAN_POINT('',(32.2716262263503,54.2496319067047,7.));
#30313=CARTESIAN_POINT('Ctrl Pts',(33.5264962288793,58.0679896197986,6.60407471946233));
#30314=CARTESIAN_POINT('Ctrl Pts',(33.1919689183208,58.2597658075907,6.62491192240684));
#30315=CARTESIAN_POINT('Ctrl Pts',(32.1179432461623,58.5451601991561,6.68279508887403));
#30316=CARTESIAN_POINT('Ctrl Pts',(30.4105200538552,57.5324032730233,6.77772421886391));
#30317=CARTESIAN_POINT('Ctrl Pts',(30.3280193568976,55.2072605605051,6.88886210943196));
#30318=CARTESIAN_POINT('Ctrl Pts',(31.592606214368,54.3255716196824,6.96295403647732));
#30319=CARTESIAN_POINT('Ctrl Pts',(32.2716262263503,54.2496319067047,7.));
#30320=CARTESIAN_POINT('',(33.3217794842373,54.4043178444011,6.99999999999999));
#30321=CARTESIAN_POINT('Origin',(32.5,56.2916512459885,7.));
#30322=CARTESIAN_POINT('Ctrl Pts',(33.5275749112977,58.0738535198176,6.54592528053768));
#30323=CARTESIAN_POINT('Ctrl Pts',(33.4657840639228,58.1101089614272,6.54982271160486));
#30324=CARTESIAN_POINT('Ctrl Pts',(32.7965074863137,58.4550718384181,6.59076610619471));
#30325=CARTESIAN_POINT('Ctrl Pts',(31.1711925871668,58.3247407101007,6.66875546430726));
#30326=CARTESIAN_POINT('Ctrl Pts',(30.0714699489351,56.2774508415846,6.77989335487529));
#30327=CARTESIAN_POINT('Ctrl Pts',(31.1870202472961,54.2576863817542,6.89030820010621));
#30328=CARTESIAN_POINT('Ctrl Pts',(32.7099100739971,54.1388320417446,6.96367708181444));
#30329=CARTESIAN_POINT('Ctrl Pts',(33.3217804591137,54.4043158724519,7.));
#30330=CARTESIAN_POINT('Origin',(32.5,56.2916512459885,-3.54592528053767));
#30331=CARTESIAN_POINT('',(33.5250713804254,58.0691800125914,5.84592528053768));
#30332=CARTESIAN_POINT('',(33.5296302847681,58.0720277053709,5.90407471946232));
#30333=CARTESIAN_POINT('',(33.5273749999999,58.0711169444147,-3.54592528053767));
#30334=CARTESIAN_POINT('Ctrl Pts',(33.5296302847681,58.0720277053709,5.90407471946233));
#30335=CARTESIAN_POINT('Ctrl Pts',(33.0191355770127,58.3612066004053,5.93596947460409));
#30336=CARTESIAN_POINT('Ctrl Pts',(31.6285851526934,58.5053110361567,6.00491019326853));
#30337=CARTESIAN_POINT('Ctrl Pts',(30.1397737216656,56.8641588006487,6.11089687545567));
#30338=CARTESIAN_POINT('Ctrl Pts',(30.7390063155881,54.6191619749282,6.2220347660237));
#30339=CARTESIAN_POINT('Ctrl Pts',(32.9499730445898,53.9051289476276,6.33317265659175));
#30340=CARTESIAN_POINT('Ctrl Pts',(34.7493198838486,55.375277132786,6.44431054715978));
#30341=CARTESIAN_POINT('Ctrl Pts',(34.5380916131598,57.2516667239214,6.53461123478332));
#30342=CARTESIAN_POINT('Ctrl Pts',(33.7867170031423,57.9188115213373,6.58786595888416));
#30343=CARTESIAN_POINT('Ctrl Pts',(33.5264962288793,58.0679896197986,6.60407471946233));
#30344=CARTESIAN_POINT('Ctrl Pts',(33.5250713804254,58.0691800125914,5.84592528053768));
#30345=CARTESIAN_POINT('Ctrl Pts',(33.2860537216368,58.2086221814904,5.8608802638021));
#30346=CARTESIAN_POINT('Ctrl Pts',(32.3636248873145,58.5321674493612,5.91288121058921));
#30347=CARTESIAN_POINT('Ctrl Pts',(30.6332940299706,57.8452774805726,6.00192812089902));
#30348=CARTESIAN_POINT('Ctrl Pts',(30.1823177935136,55.5659199366929,6.11306601146704));
#30349=CARTESIAN_POINT('Ctrl Pts',(31.8527378172473,53.9508533596396,6.2242039020351));
#30350=CARTESIAN_POINT('Ctrl Pts',(34.1156133119216,54.4783040835128,6.33534179260312));
#30351=CARTESIAN_POINT('Ctrl Pts',(34.8721855502189,56.5889092129518,6.442582252104));
#30352=CARTESIAN_POINT('Ctrl Pts',(34.0531200394492,57.7654927913865,6.51277674808218));
#30353=CARTESIAN_POINT('Ctrl Pts',(33.5275749112977,58.0738535198176,6.54592528053768));
#30354=CARTESIAN_POINT('Origin',(32.5,56.2916512459885,-3.54592528053767));
#30355=CARTESIAN_POINT('',(33.5282754020985,58.069145943353,5.14592528053768));
#30356=CARTESIAN_POINT('',(33.5267258804522,58.073260437028,5.20407471946232));
#30357=CARTESIAN_POINT('',(33.5273749999999,58.0711169444147,-3.54592528053767));
#30358=CARTESIAN_POINT('Ctrl Pts',(33.5267258804522,58.073260437028,5.20407471946232));
#30359=CARTESIAN_POINT('Ctrl Pts',(33.4330630138882,58.1284275812183,5.20998106327866));
#30360=CARTESIAN_POINT('Ctrl Pts',(32.7207180221807,58.4735694661581,5.25293337061768));
#30361=CARTESIAN_POINT('Ctrl Pts',(31.0632581782873,58.2497382420229,5.33293164147937));
#30362=CARTESIAN_POINT('Ctrl Pts',(30.0756916068806,56.1465211293306,5.44406953204742));
#30363=CARTESIAN_POINT('Ctrl Pts',(31.3071229976033,54.1761423261722,5.55520742261545));
#30364=CARTESIAN_POINT('Ctrl Pts',(33.6304062534725,54.1421146842281,5.6663453131835));
#30365=CARTESIAN_POINT('Ctrl Pts',(34.9190197935988,56.0755785414894,5.77748320375153));
#30366=CARTESIAN_POINT('Ctrl Pts',(34.2590870859834,57.5951911211838,5.85672633917782));
#30367=CARTESIAN_POINT('Ctrl Pts',(33.6120784680294,58.0253234512995,5.89892351108141));
#30368=CARTESIAN_POINT('Ctrl Pts',(33.5296302847681,58.0720277053709,5.90407471946233));
#30369=CARTESIAN_POINT('Ctrl Pts',(33.5282754020985,58.069145943353,5.14592528053768));
#30370=CARTESIAN_POINT('Ctrl Pts',(33.1102767098287,58.3059329434062,5.17193781599936));
#30371=CARTESIAN_POINT('Ctrl Pts',(31.892698227861,58.5381488249037,5.23499631498371));
#30372=CARTESIAN_POINT('Ctrl Pts',(30.2596385516873,57.2292625110706,5.33510077749076));
#30373=CARTESIAN_POINT('Ctrl Pts',(30.4972127153845,54.9179054771161,5.44623866805879));
#30374=CARTESIAN_POINT('Ctrl Pts',(32.5679607208418,53.8639538597437,5.55737655862684));
#30375=CARTESIAN_POINT('Ctrl Pts',(34.5765036531329,55.0321005249752,5.66851444919487));
#30376=CARTESIAN_POINT('Ctrl Pts',(34.6698803007257,57.0408062963268,5.7646973564985));
#30377=CARTESIAN_POINT('Ctrl Pts',(33.8781399387991,57.8632008987502,5.82383430027942));
#30378=CARTESIAN_POINT('Ctrl Pts',(33.5250713804254,58.0691800125914,5.84592528053768));
#30379=CARTESIAN_POINT('Origin',(32.5,56.2916512459885,-3.54592528053767));
#30380=CARTESIAN_POINT('',(33.5290696646583,58.0740687441032,4.44592528053768));
#30381=CARTESIAN_POINT('',(33.5253496165875,58.0685468270267,4.50407471946232));
#30382=CARTESIAN_POINT('',(33.5273749999999,58.0711169444147,-3.54592528053767));
#30383=CARTESIAN_POINT('Ctrl Pts',(33.5253496165875,58.0685468270267,4.50407471946232));
#30384=CARTESIAN_POINT('Ctrl Pts',(33.2536996405186,58.2261242815538,4.52103861547591));
#30385=CARTESIAN_POINT('Ctrl Pts',(32.2808222041073,58.539100979713,4.57504847501218));
#30386=CARTESIAN_POINT('Ctrl Pts',(30.5520219543112,57.7420698681825,4.66610429807112));
#30387=CARTESIAN_POINT('Ctrl Pts',(30.2249467851584,55.4416715145514,4.77724218863916));
#30388=CARTESIAN_POINT('Ctrl Pts',(31.980253640428,53.9192692335435,4.8883800792072));
#30389=CARTESIAN_POINT('Ctrl Pts',(34.2112902010514,54.5683351429997,4.99951796977525));
#30390=CARTESIAN_POINT('Ctrl Pts',(34.8406399092008,56.6764493817393,5.10474951652695));
#30391=CARTESIAN_POINT('Ctrl Pts',(34.0205383194344,57.7824064089199,5.17293509975598));
#30392=CARTESIAN_POINT('Ctrl Pts',(33.5267258804522,58.073260437028,5.20407471946232));
#30393=CARTESIAN_POINT('Ctrl Pts',(33.529069656232,58.0740687294262,4.44592528053768));
#30394=CARTESIAN_POINT('Ctrl Pts',(33.5286860990811,58.0742902067968,4.44594940467393));
#30395=CARTESIAN_POINT('Ctrl Pts',(32.9391765838663,58.4144119362181,4.48301949233286));
#30396=CARTESIAN_POINT('Ctrl Pts',(31.390101627814,58.451850257884,4.55713554351446));
#30397=CARTESIAN_POINT('Ctrl Pts',(30.0831480764379,56.5307348090518,4.66827343408251));
#30398=CARTESIAN_POINT('Ctrl Pts',(30.9883665002516,54.3907834608547,4.77941132465054));
#30399=CARTESIAN_POINT('Ctrl Pts',(33.2772002083032,53.9907179590751,4.89054921521859));
#30400=CARTESIAN_POINT('Ctrl Pts',(34.8546537539781,55.6967227784588,5.00168710578663));
#30401=CARTESIAN_POINT('Ctrl Pts',(34.4121009342633,57.4205168337107,5.08681246089299));
#30402=CARTESIAN_POINT('Ctrl Pts',(33.705572940339,57.9687108152697,5.13489185247668));
#30403=CARTESIAN_POINT('Ctrl Pts',(33.5282754020985,58.069145943353,5.14592528053768));
#30404=CARTESIAN_POINT('Origin',(32.5,56.2916512459885,-3.54592528053767));
#30405=CARTESIAN_POINT('',(33.5252102943906,58.0708877004567,3.74592528053768));
#30406=CARTESIAN_POINT('',(33.5289081309378,58.0700145843707,3.80407471946232));
#30407=CARTESIAN_POINT('',(33.5273749999999,58.0711169444147,-3.54592528053767));
#30408=CARTESIAN_POINT('Ctrl Pts',(33.5289081309378,58.0700145843707,3.80407471946232));
#30409=CARTESIAN_POINT('Ctrl Pts',(33.0789876682099,58.3243434135939,3.83209616767316));
#30410=CARTESIAN_POINT('Ctrl Pts',(31.8034240249952,58.5300263366319,3.89716357940668));
#30411=CARTESIAN_POINT('Ctrl Pts',(30.2122199456457,57.1067555851009,3.99927695466286));
#30412=CARTESIAN_POINT('Ctrl Pts',(30.5744204047745,54.811625609896,4.11041484523092));
#30413=CARTESIAN_POINT('Ctrl Pts',(32.6991257052286,53.8711798837977,4.22155273579895));
#30414=CARTESIAN_POINT('Ctrl Pts',(34.6415689889353,55.1462190460046,4.332690626367));
#30415=CARTESIAN_POINT('Ctrl Pts',(34.6265206091308,57.1150354081819,4.42686462092145));
#30416=CARTESIAN_POINT('Ctrl Pts',(33.8469321795725,57.8820047097448,4.48399265195323));
#30417=CARTESIAN_POINT('Ctrl Pts',(33.5253496165875,58.0685468270267,4.50407471946232));
#30418=CARTESIAN_POINT('Ctrl Pts',(33.5252102943906,58.0708877004567,3.74592528053768));
#30419=CARTESIAN_POINT('Ctrl Pts',(33.3488056811853,58.174663668992,3.75700695687117));
#30420=CARTESIAN_POINT('Ctrl Pts',(32.5196622305249,58.5123107269967,3.80513459672736));
#30421=CARTESIAN_POINT('Ctrl Pts',(30.8051884955116,58.0311765069792,3.89030820010621));
#30422=CARTESIAN_POINT('Ctrl Pts',(30.1193554633367,55.8111663248381,4.00144609067426));
#30423=CARTESIAN_POINT('Ctrl Pts',(31.6125533739245,54.0309494400521,4.11258398124229));
#30424=CARTESIAN_POINT('Ctrl Pts',(33.9180412456697,54.3199785564283,4.22372187181034));
#30425=CARTESIAN_POINT('Ctrl Pts',(34.9253611823253,56.4132475717747,4.33483563824213));
#30426=CARTESIAN_POINT('Ctrl Pts',(34.1176914037627,57.7341809275558,4.40890344115124));
#30427=CARTESIAN_POINT('Ctrl Pts',(33.529069656232,58.0740687294262,4.44592528053768));
#30428=CARTESIAN_POINT('Origin',(32.5,56.2916512459885,-3.54592528053767));
#30429=CARTESIAN_POINT('',(33.5268671815904,58.0681591655549,3.04592528053767));
#30430=CARTESIAN_POINT('',(33.5283521207634,58.0741669114358,3.10407471946232));
#30431=CARTESIAN_POINT('',(33.5273749999999,58.0711169444147,-3.54592528053767));
#30432=CARTESIAN_POINT('Ctrl Pts',(33.5283521207634,58.0741669114358,3.10407471946232));
#30433=CARTESIAN_POINT('Ctrl Pts',(33.4960959785976,58.0929755878456,3.10610775634772));
#30434=CARTESIAN_POINT('Ctrl Pts',(32.8657385633012,58.4363094602464,3.14518675675581));
#30435=CARTESIAN_POINT('Ctrl Pts',(31.2749245001037,58.3886783513255,3.22131172068658));
#30436=CARTESIAN_POINT('Ctrl Pts',(30.0737566908708,56.3997070920348,3.33244961125462));
#30437=CARTESIAN_POINT('Ctrl Pts',(31.0933568979523,54.3118310914232,3.44358750182266));
#30438=CARTESIAN_POINT('Ctrl Pts',(33.40047348876,54.0361069309691,3.5547253923907));
#30439=CARTESIAN_POINT('Ctrl Pts',(34.8833764832335,55.8249080616723,3.66586328295875));
#30440=CARTESIAN_POINT('Ctrl Pts',(34.3608947477859,57.4821952700404,3.74897972531595));
#30441=CARTESIAN_POINT('Ctrl Pts',(33.6738083543113,57.9881060978322,3.79505020415047));
#30442=CARTESIAN_POINT('Ctrl Pts',(33.5289081309378,58.0700145843707,3.80407471946232));
#30443=CARTESIAN_POINT('Ctrl Pts',(33.5268671815904,58.0681591655549,3.04592528053768));
#30444=CARTESIAN_POINT('Ctrl Pts',(33.1711688207572,58.2713555197574,3.06806450906842));
#30445=CARTESIAN_POINT('Ctrl Pts',(32.0617673212826,58.5453769689693,3.12724970112185));
#30446=CARTESIAN_POINT('Ctrl Pts',(30.3694292262435,57.4574138064661,3.22348085669796));
#30447=CARTESIAN_POINT('Ctrl Pts',(30.3650742488504,55.1338834771873,3.33461874726601));
#30448=CARTESIAN_POINT('Ctrl Pts',(32.3148410231894,53.870071116671,3.44575663783404));
#30449=CARTESIAN_POINT('Ctrl Pts',(34.4340859088485,54.822758511107,3.55689452840209));
#30450=CARTESIAN_POINT('Ctrl Pts',(34.7482454446892,56.8908856856794,3.65695074263663));
#30451=CARTESIAN_POINT('Ctrl Pts',(33.9385250223179,57.8277413596598,3.71996099334849));
#30452=CARTESIAN_POINT('Ctrl Pts',(33.5252102943906,58.0708877004567,3.74592528053768));
#30453=CARTESIAN_POINT('Origin',(32.5,56.2916512459885,-3.54592528053767));
#30454=CARTESIAN_POINT('',(33.5296717523759,58.0726906696378,2.34592528053768));
#30455=CARTESIAN_POINT('',(33.5250223861017,58.0699440624176,2.40407471946232));
#30456=CARTESIAN_POINT('',(33.5273749999999,58.0711169444147,-3.54592528053767));
#30457=CARTESIAN_POINT('Ctrl Pts',(33.5250223861017,58.0699440624176,2.40407471946232));
#30458=CARTESIAN_POINT('Ctrl Pts',(33.3162068666575,58.1923260109822,2.41716530854498));
#30459=CARTESIAN_POINT('Ctrl Pts',(32.4393285405002,58.523643057744,2.46730186115031));
#30460=CARTESIAN_POINT('Ctrl Pts',(30.7136126829218,57.9369940717681,2.55448437727833));
#30461=CARTESIAN_POINT('Ctrl Pts',(30.1488178080538,55.6831490181888,2.66562226784637));
#30462=CARTESIAN_POINT('Ctrl Pts',(31.7360866576937,53.9862729545993,2.77676015841441));
#30463=CARTESIAN_POINT('Ctrl Pts',(34.0225740529132,54.3995357858862,2.88789804898245));
#30464=CARTESIAN_POINT('Ctrl Pts',(34.8990991658236,56.5054325192522,2.99700290266509));
#30465=CARTESIAN_POINT('Ctrl Pts',(34.0838668521307,57.750244206438,3.06906179282504));
#30466=CARTESIAN_POINT('Ctrl Pts',(33.5283521207634,58.0741669114358,3.10407471946232));
#30467=CARTESIAN_POINT('Ctrl Pts',(33.5296717523759,58.0726906696378,2.34592528053768));
#30468=CARTESIAN_POINT('Ctrl Pts',(32.9991186855868,58.3741080652298,2.37912206126567));
#30469=CARTESIAN_POINT('Ctrl Pts',(31.5690873940506,58.494201559501,2.44936480551635));
#30470=CARTESIAN_POINT('Ctrl Pts',(30.1211733226086,56.7810568122913,2.55665351328971));
#30471=CARTESIAN_POINT('Ctrl Pts',(30.7986796648578,54.558491332239,2.66779140385775));
#30472=CARTESIAN_POINT('Ctrl Pts',(33.0334238041474,53.9223067766118,2.7789292944258));
#30473=CARTESIAN_POINT('Ctrl Pts',(34.7799190860636,55.4548100839991,2.89006718499383));
#30474=CARTESIAN_POINT('Ctrl Pts',(34.5073761199108,57.2954160769099,2.97906584703113));
#30475=CARTESIAN_POINT('Ctrl Pts',(33.7663651927629,57.931343458575,3.03101854554574));
#30476=CARTESIAN_POINT('Ctrl Pts',(33.5268671815904,58.0681591655549,3.04592528053768));
#30477=CARTESIAN_POINT('Origin',(32.5,56.2916512459885,-3.54592528053767));
#30478=CARTESIAN_POINT('',(33.5262302754658,58.0727324938748,1.64592528053768));
#30479=CARTESIAN_POINT('',(33.527606748894,58.0685424219933,1.70407471946232));
#30480=CARTESIAN_POINT('',(33.5273749999999,58.0711169444147,-3.54592528053767));
#30481=CARTESIAN_POINT('Ctrl Pts',(33.527606748894,58.0685424219933,1.70407471946232));
#30482=CARTESIAN_POINT('Ctrl Pts',(33.1394910367319,58.2891654943862,1.72822286074223));
#30483=CARTESIAN_POINT('Ctrl Pts',(31.9746000084876,58.542974075687,1.78941696554481));
#30484=CARTESIAN_POINT('Ctrl Pts',(30.3095139648772,57.3405094780172,1.88765703387008));
#30485=CARTESIAN_POINT('Ctrl Pts',(30.4307974560058,55.0201428925398,1.99879492443812));
#30486=CARTESIAN_POINT('Ctrl Pts',(32.4460455020051,53.8636023228594,2.10993281500616));
#30487=CARTESIAN_POINT('Ctrl Pts',(34.5106787119048,54.9294824684667,2.2210707055742));
#30488=CARTESIAN_POINT('Ctrl Pts',(34.7085028063897,56.9697666836067,2.31911800705959));
#30489=CARTESIAN_POINT('Ctrl Pts',(33.9071483489282,57.8459888695647,2.3801193450223));
#30490=CARTESIAN_POINT('Ctrl Pts',(33.5250223861017,58.0699440624176,2.40407471946232));
#30491=CARTESIAN_POINT('Ctrl Pts',(33.5262302754658,58.0727324938748,1.64592528053767));
#30492=CARTESIAN_POINT('Ctrl Pts',(33.4118498551747,58.1401751811515,1.65313364994024));
#30493=CARTESIAN_POINT('Ctrl Pts',(32.670930140884,58.4845521558011,1.69738798286549));
#30494=CARTESIAN_POINT('Ctrl Pts',(30.9955026631254,58.198172143523,1.77868827931342));
#30495=CARTESIAN_POINT('Ctrl Pts',(30.082268834923,56.0616291105053,1.88982616988146));
#30496=CARTESIAN_POINT('Ctrl Pts',(31.3820117610517,54.1356279467244,2.0009640604495));
#30497=CARTESIAN_POINT('Ctrl Pts',(33.7050620011388,54.1830593597268,2.11210195101754));
#30498=CARTESIAN_POINT('Ctrl Pts',(34.9251053252509,56.1605088392832,2.22323984158559));
#30499=CARTESIAN_POINT('Ctrl Pts',(34.224026615261,57.6314775216245,2.30118095142563));
#30500=CARTESIAN_POINT('Ctrl Pts',(33.5911896372902,58.0377411767145,2.34207609774299));
#30501=CARTESIAN_POINT('Ctrl Pts',(33.5296717523759,58.0726906696378,2.34592528053768));
#30502=CARTESIAN_POINT('Origin',(32.5,56.2916512459885,-3.54592528053767));
#30503=CARTESIAN_POINT('',(33.5256402930184,58.0682685471634,0.945925280537676));
#30504=CARTESIAN_POINT('',(33.5294982470258,58.0735597602013,1.00407471946232));
#30505=CARTESIAN_POINT('',(33.5273749999999,58.0711169444147,-3.54592528053767));
#30506=CARTESIAN_POINT('Ctrl Pts',(33.5294982470258,58.0735597602013,1.00407471946232));
#30507=CARTESIAN_POINT('Ctrl Pts',(32.9682880946418,58.3946192964702,1.03928041293948));
#30508=CARTESIAN_POINT('Ctrl Pts',(31.4766956957228,58.4741418727902,1.11153206993931));
#30509=CARTESIAN_POINT('Ctrl Pts',(30.0981915249122,56.6517188923722,1.22082969046183));
#30510=CARTESIAN_POINT('Ctrl Pts',(30.8948796869627,54.4690373423775,1.33196758102987));
#30511=CARTESIAN_POINT('Ctrl Pts',(33.1607526748339,53.9546149682086,1.44310547159791));
#30512=CARTESIAN_POINT('Ctrl Pts',(34.8218312459871,55.5793084028842,1.55424336216595));
#30513=CARTESIAN_POINT('Ctrl Pts',(34.4585557374772,57.361331949687,1.64123311145409));
#30514=CARTESIAN_POINT('Ctrl Pts',(33.7349041722058,57.9507048982935,1.69117689721955));
#30515=CARTESIAN_POINT('Ctrl Pts',(33.527606748894,58.0685424219933,1.70407471946232));
#30516=CARTESIAN_POINT('Ctrl Pts',(33.5256402930184,58.0682685471634,0.945925280537675));
#30517=CARTESIAN_POINT('Ctrl Pts',(33.2328184146122,58.2374617349622,0.964191202137492));
#30518=CARTESIAN_POINT('Ctrl Pts',(32.2264812528154,58.542293513151,1.01950308725999));
#30519=CARTESIAN_POINT('Ctrl Pts',(30.5023763530244,57.672894864812,1.11186093590517));
#30520=CARTESIAN_POINT('Ctrl Pts',(30.2561395980005,55.3624447749947,1.22299882647321));
#30521=CARTESIAN_POINT('Ctrl Pts',(32.0637337160182,53.9025079060376,1.33413671704125));
#30522=CARTESIAN_POINT('Ctrl Pts',(34.2706473113688,54.6293810308449,1.44527460760929));
#30523=CARTESIAN_POINT('Ctrl Pts',(34.8188452912069,56.7319204842157,1.54920412877477));
#30524=CARTESIAN_POINT('Ctrl Pts',(33.9996850008464,57.7935670658911,1.61608768641756));
#30525=CARTESIAN_POINT('Ctrl Pts',(33.5262302754658,58.0727324938748,1.64592528053767));
#30526=CARTESIAN_POINT('Origin',(32.5,56.2916512459885,-3.54592528053767));
#30527=CARTESIAN_POINT('',(33.5292382420787,58.0706648023921,0.245925280537672));
#30528=CARTESIAN_POINT('',(33.5256021009515,58.0718002431918,0.30407471946232));
#30529=CARTESIAN_POINT('',(33.5273749999999,58.0711169444147,-3.54592528053767));
#30530=CARTESIAN_POINT('Ctrl Pts',(33.5256021009515,58.0718002431918,0.304074719462319));
#30531=CARTESIAN_POINT('Ctrl Pts',(33.3791306461153,58.1581427811428,0.313292001614043));
#30532=CARTESIAN_POINT('Ctrl Pts',(32.5930673149394,58.4998906338152,0.359555247288449));
#30533=CARTESIAN_POINT('Ctrl Pts',(30.894619061498,58.1140355911319,0.442864456485535));
#30534=CARTESIAN_POINT('Ctrl Pts',(30.0982430406458,55.931240133699,0.554002347053577));
#30535=CARTESIAN_POINT('Ctrl Pts',(31.5002224030512,54.0783330542954,0.665140237621618));
#30536=CARTESIAN_POINT('Ctrl Pts',(33.8173095378994,54.2513012166796,0.776278128189661));
#30537=CARTESIAN_POINT('Ctrl Pts',(34.9286483135496,56.2918248999351,0.887416018757702));
#30538=CARTESIAN_POINT('Ctrl Pts',(34.1691544002424,57.6858533133783,0.963348215848589));
#30539=CARTESIAN_POINT('Ctrl Pts',(33.5588337928047,58.0567773540314,1.00223444941679));
#30540=CARTESIAN_POINT('Ctrl Pts',(33.5294982470258,58.0735597602013,1.00407471946232));
#30541=CARTESIAN_POINT('Ctrl Pts',(33.5292382420787,58.0706648023921,0.245925280537674));
#30542=CARTESIAN_POINT('Ctrl Pts',(33.0588051630517,58.33651145622,0.275248754334741));
#30543=CARTESIAN_POINT('Ctrl Pts',(31.7450292213916,58.5230813041052,0.34161819165449));
#30544=CARTESIAN_POINT('Ctrl Pts',(30.1850532410697,57.0260596319961,0.445033592496918));
#30545=CARTESIAN_POINT('Ctrl Pts',(30.6274839128385,54.7450363379153,0.55617148306496));
#30546=CARTESIAN_POINT('Ctrl Pts',(32.783849793945,53.8796472115696,0.667309373633002));
#30547=CARTESIAN_POINT('Ctrl Pts',(34.6804047400893,55.2219927306231,0.778447264201043));
#30548=CARTESIAN_POINT('Ctrl Pts',(34.5975134385768,57.1618755368451,0.871319233169269));
#30549=CARTESIAN_POINT('Ctrl Pts',(33.8267040593522,57.8943131766358,0.927145238614812));
#30550=CARTESIAN_POINT('Ctrl Pts',(33.5256402930184,58.0682685471634,0.945925280537675));
#30551=CARTESIAN_POINT('Origin',(32.5,56.2916512459885,-3.54592528053767));
#30552=CARTESIAN_POINT('',(33.5278097333143,58.0740011795199,-0.454074719462328));
#30553=CARTESIAN_POINT('',(33.5262237855851,58.0680718733222,-0.395925280537679));
#30554=CARTESIAN_POINT('',(33.5273749999999,58.0711169444147,-3.54592528053767));
#30555=CARTESIAN_POINT('Ctrl Pts',(33.5262237855851,58.0680718733222,-0.395925280537681));
#30556=CARTESIAN_POINT('Ctrl Pts',(33.2007518244939,58.254991046836,-0.375650446188706));
#30557=CARTESIAN_POINT('Ctrl Pts',(32.1416146375096,58.5451226040269,-0.318329648317051));
#30558=CARTESIAN_POINT('Ctrl Pts',(30.4306156658191,57.5628636674516,-0.223962886922716));
#30559=CARTESIAN_POINT('Ctrl Pts',(30.309663968686,55.2424797818377,-0.112824996354674));
#30560=CARTESIAN_POINT('Ctrl Pts',(32.1935517174548,53.8824144115655,-0.00168710578663204));
#30561=CARTESIAN_POINT('Ctrl Pts',(34.3579350363403,54.7275508506072,0.10945078478141));
#30562=CARTESIAN_POINT('Ctrl Pts',(34.7832643179971,56.8155005034113,0.211371393197726));
#30563=CARTESIAN_POINT('Ctrl Pts',(33.9678265418961,57.8111161350299,0.276246038091363));
#30564=CARTESIAN_POINT('Ctrl Pts',(33.5256021009515,58.0718002431918,0.304074719462319));
#30565=CARTESIAN_POINT('Ctrl Pts',(33.5278097333143,58.0740011795199,-0.454074719462326));
#30566=CARTESIAN_POINT('Ctrl Pts',(33.4749288712104,58.1049786318385,-0.450739656990689));
#30567=CARTESIAN_POINT('Ctrl Pts',(32.8174992673745,58.4495803163018,-0.410358630996372));
#30568=CARTESIAN_POINT('Ctrl Pts',(31.2021687803137,58.344446263511,-0.332931641479374));
#30569=CARTESIAN_POINT('Ctrl Pts',(30.0714596841225,56.3145920190741,-0.221793750911332));
#30570=CARTESIAN_POINT('Ctrl Pts',(31.1636212068566,54.2637395061115,-0.110655860343291));
#30571=CARTESIAN_POINT('Ctrl Pts',(33.4789853310955,54.0690577668369,0.000482030224751639));
#30572=CARTESIAN_POINT('Ctrl Pts',(34.8982731111897,55.908740964546,0.111619920792793));
#30573=CARTESIAN_POINT('Ctrl Pts',(34.3271081175644,57.521036291931,0.193434337563767));
#30574=CARTESIAN_POINT('Ctrl Pts',(33.6531292464159,58.0006526999044,0.238202790812061));
#30575=CARTESIAN_POINT('Ctrl Pts',(33.5292382420787,58.0706648023921,0.245925280537674));
#30576=CARTESIAN_POINT('Origin',(32.5,56.2916512459885,-3.54592528053767));
#30577=CARTESIAN_POINT('',(33.5250365419916,58.0693901510839,-1.15407471946233));
#30578=CARTESIAN_POINT('',(33.5295799600394,58.0717283210701,-1.09592528053768));
#30579=CARTESIAN_POINT('',(33.5273749999999,58.0711169444147,-3.54592528053767));
#30580=CARTESIAN_POINT('Ctrl Pts',(33.5295799600394,58.0717283210701,-1.09592528053768));
#30581=CARTESIAN_POINT('Ctrl Pts',(33.0277944721986,58.3557212843618,-1.06459289399146));
#30582=CARTESIAN_POINT('Ctrl Pts',(31.6541659742537,58.5096740781238,-0.996214543922551));
#30583=CARTESIAN_POINT('Ctrl Pts',(30.1487320710281,56.8998163998922,-0.890790230330966));
#30584=CARTESIAN_POINT('Ctrl Pts',(30.7138473610246,54.6460533962845,-0.779652339762924));
#30585=CARTESIAN_POINT('Ctrl Pts',(32.9138506780699,53.8985232611178,-0.668514449194883));
#30586=CARTESIAN_POINT('Ctrl Pts',(34.7350506405739,55.3414510668855,-0.55737655862684));
#30587=CARTESIAN_POINT('Ctrl Pts',(34.5514515687201,57.2322106426396,-0.466513502407774));
#30588=CARTESIAN_POINT('Ctrl Pts',(33.7954507596715,57.9134543040694,-0.412696409711387));
#30589=CARTESIAN_POINT('Ctrl Pts',(33.5262237855851,58.0680718733222,-0.395925280537681));
#30590=CARTESIAN_POINT('Ctrl Pts',(33.5250365419916,58.0693901510839,-1.15407471946233));
#30591=CARTESIAN_POINT('Ctrl Pts',(33.2951376806275,58.2037133203311,-1.13968210479344));
#30592=CARTESIAN_POINT('Ctrl Pts',(32.3865699532721,58.5298194771329,-1.08824352660187));
#30593=CARTESIAN_POINT('Ctrl Pts',(30.6570393620672,57.873352597378,-0.999758984887625));
#30594=CARTESIAN_POINT('Ctrl Pts',(30.1715905180572,55.6011108576298,-0.888621094319582));
#30595=CARTESIAN_POINT('Ctrl Pts',(31.817369145763,53.960908709333,-0.777483203751541));
#30596=CARTESIAN_POINT('Ctrl Pts',(34.087963584719,54.4540716106361,-0.666345313183499));
#30597=CARTESIAN_POINT('Ctrl Pts',(34.8805586635865,56.5639154031852,-0.558542485087094));
#30598=CARTESIAN_POINT('Ctrl Pts',(34.0623309079662,57.7608802593548,-0.48778562051337));
#30599=CARTESIAN_POINT('Ctrl Pts',(33.5278097333143,58.0740011795199,-0.454074719462326));
#30600=CARTESIAN_POINT('Origin',(32.5,56.2916512459885,-3.54592528053767));
#30601=CARTESIAN_POINT('',(33.5283546803393,58.0681541983481,-1.85407471946233));
#30602=CARTESIAN_POINT('',(33.5269872402601,58.0734398505124,-1.79592528053768));
#30603=CARTESIAN_POINT('',(33.5273749999999,58.0711169444147,-3.54592528053767));
#30604=CARTESIAN_POINT('',(34.4842965055667,55.7582049595679,-2.));
#30605=CARTESIAN_POINT('Ctrl Pts',(34.4842965055667,55.7582049595679,-2.));
#30606=CARTESIAN_POINT('Ctrl Pts',(34.6616800870191,56.4180307560557,-1.96295403647732));
#30607=CARTESIAN_POINT('Ctrl Pts',(34.426165795488,57.4023224375313,-1.91431227629809));
#30608=CARTESIAN_POINT('Ctrl Pts',(33.7147012993046,57.9624349357751,-1.86567051611887));
#30609=CARTESIAN_POINT('Ctrl Pts',(33.5283546803393,58.0681541983481,-1.85407471946233));
#30610=CARTESIAN_POINT('',(33.9566395923166,54.8371582344187,-2.));
#30611=CARTESIAN_POINT('Origin',(32.5,56.2916512459885,-2.));
#30612=CARTESIAN_POINT('Ctrl Pts',(33.9566410663199,54.8371566128168,-2.));
#30613=CARTESIAN_POINT('Ctrl Pts',(34.4273146919907,55.3097386618185,-1.96367708181445));
#30614=CARTESIAN_POINT('Ctrl Pts',(34.8405825937333,56.6643607585548,-1.89565217532701));
#30615=CARTESIAN_POINT('Ctrl Pts',(34.0295256140624,57.7776919138425,-1.82762726883957));
#30616=CARTESIAN_POINT('Ctrl Pts',(33.5269872402601,58.0734398505124,-1.79592528053768));
#30617=CARTESIAN_POINT('Origin',(-32.5,56.2916512459885,3.));
#30618=CARTESIAN_POINT('',(-33.3327252244639,57.7364024133913,6.12851963660979));
#30619=CARTESIAN_POINT('',(-33.3348404573524,57.735699266238,6.32148036339022));
#30620=CARTESIAN_POINT('',(-33.333,57.7344495686934,3.));
#30621=CARTESIAN_POINT('',(-33.041102980256,57.8673300091754,7.));
#30622=CARTESIAN_POINT('Ctrl Pts',(-33.3348404573524,57.735699266238,6.32148036339022));
#30623=CARTESIAN_POINT('Ctrl Pts',(-33.3853483348094,57.7070091850913,6.3253777944574));
#30624=CARTESIAN_POINT('Ctrl Pts',(-33.4342336358034,57.6755865432426,6.32927522552458));
#30625=CARTESIAN_POINT('Ctrl Pts',(-33.4811646154108,57.6414746748817,6.33317265659176));
#30626=CARTESIAN_POINT('Ctrl Pts',(-33.9272541879144,57.3172336532427,6.37021862011444));
#30627=CARTESIAN_POINT('Ctrl Pts',(-34.196772145609,56.7500228359925,6.40726458363712));
#30628=CARTESIAN_POINT('Ctrl Pts',(-34.1662427495344,56.1993881251834,6.44431054715981));
#30629=CARTESIAN_POINT('Ctrl Pts',(-34.1357133534599,55.6487534143743,6.48135651068249));
#30630=CARTESIAN_POINT('Ctrl Pts',(-33.8051366036161,55.1146948100063,6.51840247420516));
#30631=CARTESIAN_POINT('Ctrl Pts',(-33.3260603863118,54.8417096746676,6.55544843772784));
#30632=CARTESIAN_POINT('Ctrl Pts',(-32.8469841690075,54.5687245393289,6.59249440125052));
#30633=CARTESIAN_POINT('Ctrl Pts',(-32.2194084842428,54.5568128730195,6.62954036477321));
#30634=CARTESIAN_POINT('Ctrl Pts',(-31.7300326690206,54.8112607055414,6.66658632829589));
#30635=CARTESIAN_POINT('Ctrl Pts',(-31.2406568537983,55.0657085380633,6.70363229181857));
#30636=CARTESIAN_POINT('Ctrl Pts',(-30.8894809081185,55.5865158694165,6.74067825534124));
#30637=CARTESIAN_POINT('Ctrl Pts',(-30.8382644239114,56.1356774091288,6.77772421886393));
#30638=CARTESIAN_POINT('Ctrl Pts',(-30.7870479397043,56.6848389488411,6.81477018238661));
#30639=CARTESIAN_POINT('Ctrl Pts',(-31.0357909169699,57.2623546969124,6.85181614590929));
#30640=CARTESIAN_POINT('Ctrl Pts',(-31.4683170081768,57.6029598655743,6.88886210943197));
#30641=CARTESIAN_POINT('Ctrl Pts',(-31.9008430993837,57.9435650342361,6.92590807295465));
#30642=CARTESIAN_POINT('Ctrl Pts',(-32.5171523045318,58.0472596234884,6.96295403647733));
#30643=CARTESIAN_POINT('Ctrl Pts',(-33.0411029802559,57.8673300091754,7.00000000000001));
#30644=CARTESIAN_POINT('',(-33.9709880617747,55.5030815934933,7.));
#30645=CARTESIAN_POINT('Origin',(-32.5,56.2916512459885,7.));
#30646=CARTESIAN_POINT('',(-33.3311603318024,57.7325647065031,6.82851963660978));
#30647=CARTESIAN_POINT('Ctrl Pts',(-33.9709895856634,55.5030806790319,7.));
#30648=CARTESIAN_POINT('Ctrl Pts',(-34.2258866982027,55.9800344189509,6.96367708181444));
#30649=CARTESIAN_POINT('Ctrl Pts',(-34.2280600118628,56.5931875605704,6.92735416362888));
#30650=CARTESIAN_POINT('Ctrl Pts',(-33.9753141969146,57.071300576271,6.89103124544333));
#30651=CARTESIAN_POINT('Ctrl Pts',(-33.8303226570678,57.3455774911288,6.87019404249881));
#30652=CARTESIAN_POINT('Ctrl Pts',(-33.6014392610868,57.5754137754314,6.8493568395543));
#30653=CARTESIAN_POINT('Ctrl Pts',(-33.3311603318024,57.7325647065031,6.82851963660978));
#30654=CARTESIAN_POINT('',(-33.333,57.7344495686934,8.));
#30655=CARTESIAN_POINT('',(-33.333,57.7344495686934,3.));
#30656=CARTESIAN_POINT('Origin',(-32.5,56.2916512459885,8.));
#30657=CARTESIAN_POINT('Ctrl Pts',(-33.3311603318024,57.7325647065031,6.82851963660978));
#30658=CARTESIAN_POINT('Ctrl Pts',(-33.1209168329143,57.8548086479361,6.81231087603162));
#30659=CARTESIAN_POINT('Ctrl Pts',(-32.8856252648826,57.9330713283931,6.79610211545345));
#30660=CARTESIAN_POINT('Ctrl Pts',(-32.6452880462139,57.9540583561262,6.77989335487529));
#30661=CARTESIAN_POINT('Ctrl Pts',(-32.0959848596434,58.0020252972197,6.74284739135261));
#30662=CARTESIAN_POINT('Ctrl Pts',(-31.5203244682533,57.7507986915124,6.70580142782992));
#30663=CARTESIAN_POINT('Ctrl Pts',(-31.1820200481675,57.3152751741701,6.66875546430724));
#30664=CARTESIAN_POINT('Ctrl Pts',(-30.8437156280816,56.8797516568278,6.63170950078456));
#30665=CARTESIAN_POINT('Ctrl Pts',(-30.7427671793001,56.2599312278504,6.59466353726189));
#30666=CARTESIAN_POINT('Ctrl Pts',(-30.9252443270204,55.7395177410929,6.55761757373921));
#30667=CARTESIAN_POINT('Ctrl Pts',(-31.1077214747407,55.2191042543355,6.52057161021653));
#30668=CARTESIAN_POINT('Ctrl Pts',(-31.5736242189628,54.7980977097981,6.48352564669384));
#30669=CARTESIAN_POINT('Ctrl Pts',(-32.1097948324389,54.6691542850845,6.44647968317116));
#30670=CARTESIAN_POINT('Ctrl Pts',(-32.645965445915,54.540210860371,6.40943371964848));
#30671=CARTESIAN_POINT('Ctrl Pts',(-33.2524039286451,54.7033305554813,6.37238775612581));
#30672=CARTESIAN_POINT('Ctrl Pts',(-33.6515374626529,55.0838706916793,6.33534179260313));
#30673=CARTESIAN_POINT('Ctrl Pts',(-34.0506709966607,55.4644108278773,6.29829582908045));
#30674=CARTESIAN_POINT('Ctrl Pts',(-34.2424995819463,56.0623714051628,6.26124986555776));
#30675=CARTESIAN_POINT('Ctrl Pts',(-34.1392482605268,56.604087363599,6.22420390203508));
#30676=CARTESIAN_POINT('Ctrl Pts',(-34.0503539438026,57.0704781983288,6.19230914689331));
#30677=CARTESIAN_POINT('Ctrl Pts',(-33.7427356506951,57.4951784726193,6.16041439175155));
#30678=CARTESIAN_POINT('Ctrl Pts',(-33.3327252244639,57.7364024133913,6.12851963660979));
#30679=CARTESIAN_POINT('Origin',(-32.5,56.2916512459885,3.));
#30680=CARTESIAN_POINT('',(-33.3347682721563,57.7348627592985,5.42851963660978));
#30681=CARTESIAN_POINT('',(-33.3325737793451,57.732046708219,5.62148036339022));
#30682=CARTESIAN_POINT('',(-33.333,57.7344495686934,3.));
#30683=CARTESIAN_POINT('Ctrl Pts',(-33.3325737793451,57.732046708219,5.62148036339022));
#30684=CARTESIAN_POINT('Ctrl Pts',(-33.5273851267367,57.6207441464882,5.63643534665465));
#30685=CARTESIAN_POINT('Ctrl Pts',(-33.7002675206604,57.4721914078235,5.65139032991908));
#30686=CARTESIAN_POINT('Ctrl Pts',(-33.8340159287013,57.2942275627961,5.66634531318351));
#30687=CARTESIAN_POINT('Ctrl Pts',(-34.1653328254098,56.853381726016,5.70339127670619));
#30688=CARTESIAN_POINT('Ctrl Pts',(-34.2565099960996,56.2320591280652,5.74043724022887));
#30689=CARTESIAN_POINT('Ctrl Pts',(-34.0658176145799,55.7146109150825,5.77748320375155));
#30690=CARTESIAN_POINT('Ctrl Pts',(-33.8751252330602,55.1971627020998,5.81452916727423));
#30691=CARTESIAN_POINT('Ctrl Pts',(-33.4025632993311,54.7835888740851,5.85157513079691));
#30692=CARTESIAN_POINT('Ctrl Pts',(-32.8644065969169,54.6631651603563,5.88862109431959));
#30693=CARTESIAN_POINT('Ctrl Pts',(-32.3262498945026,54.5427414466275,5.92566705784227));
#30694=CARTESIAN_POINT('Ctrl Pts',(-31.7224984234031,54.7154678471845,5.96271302136495));
#30695=CARTESIAN_POINT('Ctrl Pts',(-31.3294542359752,55.1022925139247,5.99975898488763));
#30696=CARTESIAN_POINT('Ctrl Pts',(-30.9364100485472,55.4891171806648,6.03680494841031));
#30697=CARTESIAN_POINT('Ctrl Pts',(-30.7540731447909,56.0900401135881,6.073850911933));
#30698=CARTESIAN_POINT('Ctrl Pts',(-30.8659074307874,56.6300507637272,6.11089687545568));
#30699=CARTESIAN_POINT('Ctrl Pts',(-30.9777417167839,57.1700614138663,6.14794283897836));
#30700=CARTESIAN_POINT('Ctrl Pts',(-31.3837471925331,57.6491597812212,6.18498880250104));
#30701=CARTESIAN_POINT('Ctrl Pts',(-31.898080524064,57.8480733518848,6.22203476602372));
#30702=CARTESIAN_POINT('Ctrl Pts',(-32.358303272023,58.0260601641038,6.25518329847922));
#30703=CARTESIAN_POINT('Ctrl Pts',(-32.9052595394904,57.9797148933651,6.28833183093472));
#30704=CARTESIAN_POINT('Ctrl Pts',(-33.3348404573524,57.735699266238,6.32148036339022));
#30705=CARTESIAN_POINT('Ctrl Pts',(-33.3327252244639,57.7364024133913,6.12851963660979));
#30706=CARTESIAN_POINT('Ctrl Pts',(-33.2665058998609,57.7753616334844,6.12336842822888));
#30707=CARTESIAN_POINT('Ctrl Pts',(-33.1976157450274,57.8095349962739,6.11821721984796));
#30708=CARTESIAN_POINT('Ctrl Pts',(-33.1265448412825,57.8383251884469,6.11306601146705));
#30709=CARTESIAN_POINT('Ctrl Pts',(-32.6154239715823,58.0453757152716,6.07602004794436));
#30710=CARTESIAN_POINT('Ctrl Pts',(-31.9915134603068,57.9740054293342,6.03897408442168));
#30711=CARTESIAN_POINT('Ctrl Pts',(-31.5403536505083,57.6568760819726,6.001928120899));
#30712=CARTESIAN_POINT('Ctrl Pts',(-31.0891938407098,57.3397467346111,5.96488215737631));
#30713=CARTESIAN_POINT('Ctrl Pts',(-30.8107847323884,56.7768583258254,5.92783619385363));
#30714=CARTESIAN_POINT('Ctrl Pts',(-30.8325397428817,56.2258205630586,5.89079023033096));
#30715=CARTESIAN_POINT('Ctrl Pts',(-30.854294753375,55.6747828002917,5.85374426680828));
#30716=CARTESIAN_POINT('Ctrl Pts',(-31.1762138826829,55.1355956835436,5.81669830328559));
#30717=CARTESIAN_POINT('Ctrl Pts',(-31.6509700657299,54.8550209349976,5.77965233976292));
#30718=CARTESIAN_POINT('Ctrl Pts',(-32.1257262487769,54.5744461864516,5.74260637624023));
#30719=CARTESIAN_POINT('Ctrl Pts',(-32.7533194855629,54.5524838061077,5.70556041271756));
#30720=CARTESIAN_POINT('Ctrl Pts',(-33.2465276451507,54.7991851622225,5.66851444919487));
#30721=CARTESIAN_POINT('Ctrl Pts',(-33.7397358047386,55.0458865183372,5.63146848567219));
#30722=CARTESIAN_POINT('Ctrl Pts',(-34.0985588871282,55.5612516109106,5.59442252214951));
#30723=CARTESIAN_POINT('Ctrl Pts',(-34.1587797389667,56.1094206024476,5.55737655862683));
#30724=CARTESIAN_POINT('Ctrl Pts',(-34.2190005908052,56.6575895939846,5.52033059510415));
#30725=CARTESIAN_POINT('Ctrl Pts',(-33.9806192120925,57.2385624844852,5.48328463158147));
#30726=CARTESIAN_POINT('Ctrl Pts',(-33.5527320593966,57.5864537767431,5.44623866805879));
#30727=CARTESIAN_POINT('Ctrl Pts',(-33.4845127880347,57.6419190795021,5.44033232424245));
#30728=CARTESIAN_POINT('Ctrl Pts',(-33.4114765004847,57.6914597193429,5.43442598042612));
#30729=CARTESIAN_POINT('Ctrl Pts',(-33.3347682721563,57.7348627592985,5.42851963660978));
#30730=CARTESIAN_POINT('Origin',(-32.5,56.2916512459885,3.));
#30731=CARTESIAN_POINT('',(-33.3320164235939,57.7319854708823,4.72851963660978));
#30732=CARTESIAN_POINT('',(-33.3312509399777,57.7342826871321,4.92148036339022));
#30733=CARTESIAN_POINT('',(-33.333,57.7344495686934,3.));
#30734=CARTESIAN_POINT('Ctrl Pts',(-33.3312509399777,57.7342826871321,4.92148036339022));
#30735=CARTESIAN_POINT('Ctrl Pts',(-33.6669748777684,57.5367675539577,4.9474928988519));
#30736=CARTESIAN_POINT('Ctrl Pts',(-33.937858827665,57.2229205202501,4.97350543431358));
#30737=CARTESIAN_POINT('Ctrl Pts',(-34.0694479601931,56.8587419095544,4.99951796977526));
#30738=CARTESIAN_POINT('Ctrl Pts',(-34.2568516913979,56.3400939850778,5.03656393329794));
#30739=CARTESIAN_POINT('Ctrl Pts',(-34.1617340046634,55.7193622303022,5.07360989682062));
#30740=CARTESIAN_POINT('Ctrl Pts',(-33.8276260153151,55.2806280419242,5.1106558603433));
#30741=CARTESIAN_POINT('Ctrl Pts',(-33.4935180259667,54.8418938535461,5.14770182386598));
#30742=CARTESIAN_POINT('Ctrl Pts',(-32.9204197340046,54.5851572315657,5.18474778738866));
#30743=CARTESIAN_POINT('Ctrl Pts',(-32.370612888852,54.6279151680597,5.22179375091134));
#30744=CARTESIAN_POINT('Ctrl Pts',(-31.8208060436993,54.6706731045536,5.25883971443402));
#30745=CARTESIAN_POINT('Ctrl Pts',(-31.2942906453562,55.0129255995219,5.2958856779567));
#30746=CARTESIAN_POINT('Ctrl Pts',(-31.032029319193,55.4980388156703,5.33293164147938));
#30747=CARTESIAN_POINT('Ctrl Pts',(-30.7697679930298,55.9831520318186,5.36997760500206));
#30748=CARTESIAN_POINT('Ctrl Pts',(-30.7717607390465,56.611125969147,5.40702356852474));
#30749=CARTESIAN_POINT('Ctrl Pts',(-31.0370958289673,57.0945648785311,5.44406953204742));
#30750=CARTESIAN_POINT('Ctrl Pts',(-31.3024309188881,57.5780037879153,5.48111549557011));
#30751=CARTESIAN_POINT('Ctrl Pts',(-31.831108352713,57.9169076693552,5.51816145909279));
#30752=CARTESIAN_POINT('Ctrl Pts',(-32.3811753809891,57.9561750722705,5.55520742261547));
#30753=CARTESIAN_POINT('Ctrl Pts',(-32.7091873614286,57.9795907251543,5.57729840287372));
#30754=CARTESIAN_POINT('Ctrl Pts',(-33.0448052440539,57.8964589747132,5.59938938313197));
#30755=CARTESIAN_POINT('Ctrl Pts',(-33.3325737793451,57.732046708219,5.62148036339022));
#30756=CARTESIAN_POINT('Ctrl Pts',(-33.3347682721563,57.7348627592985,5.42851963660978));
#30757=CARTESIAN_POINT('Ctrl Pts',(-32.9303446333077,57.9636936909789,5.39738001690344));
#30758=CARTESIAN_POINT('Ctrl Pts',(-32.4238541169951,58.0219212024995,5.36624039719709));
#30759=CARTESIAN_POINT('Ctrl Pts',(-31.9831067199836,57.8783395309755,5.33510077749075));
#30760=CARTESIAN_POINT('Ctrl Pts',(-31.4587614599457,57.7075242989346,5.29805481396806));
#30761=CARTESIAN_POINT('Ctrl Pts',(-31.0274638665491,57.2510841408376,5.26100885044538));
#30762=CARTESIAN_POINT('Ctrl Pts',(-30.8865996954395,56.7179114934437,5.2239628869227));
#30763=CARTESIAN_POINT('Ctrl Pts',(-30.7457355243299,56.1847388460498,5.18691692340002));
#30764=CARTESIAN_POINT('Ctrl Pts',(-30.8953047755072,55.5748337093591,5.14987095987734));
#30765=CARTESIAN_POINT('Ctrl Pts',(-31.2668562499327,55.1673226224438,5.11282499635466));
#30766=CARTESIAN_POINT('Ctrl Pts',(-31.6384077243582,54.7598115355286,5.07577903283198));
#30767=CARTESIAN_POINT('Ctrl Pts',(-32.231941422032,54.5546944983887,5.0387330693093));
#30768=CARTESIAN_POINT('Ctrl Pts',(-32.7758232721695,54.6458444887421,5.00168710578662));
#30769=CARTESIAN_POINT('Ctrl Pts',(-33.319705122307,54.7369944790955,4.96464114226394));
#30770=CARTESIAN_POINT('Ctrl Pts',(-33.8139351249082,55.1244114969421,4.92759517874126));
#30771=CARTESIAN_POINT('Ctrl Pts',(-34.0323261210678,55.6307919459654,4.89054921521858));
#30772=CARTESIAN_POINT('Ctrl Pts',(-34.2507171172273,56.1371723949886,4.8535032516959));
#30773=CARTESIAN_POINT('Ctrl Pts',(-34.1932691069452,56.7625162751885,4.81645728817321));
#30774=CARTESIAN_POINT('Ctrl Pts',(-33.8862734957393,57.2206314145012,4.77941132465053));
#30775=CARTESIAN_POINT('Ctrl Pts',(-33.7456956532455,57.4304091297115,4.76244742863695));
#30776=CARTESIAN_POINT('Ctrl Pts',(-33.5527911750803,57.6051213208863,4.74548353262336));
#30777=CARTESIAN_POINT('Ctrl Pts',(-33.3320164235939,57.7319854708823,4.72851963660978));
#30778=CARTESIAN_POINT('Origin',(-32.5,56.2916512459885,3.));
#30779=CARTESIAN_POINT('',(-33.3316044198825,57.73507921,4.02851963660978));
#30780=CARTESIAN_POINT('',(-33.3343856218719,57.7368361137997,4.22148036339022));
#30781=CARTESIAN_POINT('',(-33.333,57.7344495686934,3.));
#30782=CARTESIAN_POINT('Ctrl Pts',(-33.3343856149812,57.7368361019314,4.22148036339022));
#30783=CARTESIAN_POINT('Ctrl Pts',(-33.8122975339405,57.4609515848648,4.25855045104915));
#30784=CARTESIAN_POINT('Ctrl Pts',(-34.1397428670923,56.9245130794241,4.29562053870808));
#30785=CARTESIAN_POINT('Ctrl Pts',(-34.1667586100628,56.373348690468,4.33269062636701));
#30786=CARTESIAN_POINT('Ctrl Pts',(-34.1937567719725,55.8225429832862,4.36973658988969));
#30787=CARTESIAN_POINT('Ctrl Pts',(-33.9207162964576,55.2570306535141,4.40678255341237));
#30788=CARTESIAN_POINT('Ctrl Pts',(-33.4725957048463,54.9356216253736,4.44382851693505));
#30789=CARTESIAN_POINT('Ctrl Pts',(-33.024475113235,54.6142125972331,4.48087448045773));
#30790=CARTESIAN_POINT('Ctrl Pts',(-32.4012744055273,54.5369068707243,4.51792044398041));
#30791=CARTESIAN_POINT('Ctrl Pts',(-31.8882049204609,54.7390838502781,4.55496640750309));
#30792=CARTESIAN_POINT('Ctrl Pts',(-31.3751354353946,54.9412608298319,4.59201237102577));
#30793=CARTESIAN_POINT('Ctrl Pts',(-30.9721971729695,55.4229205154484,4.62905833454845));
#30794=CARTESIAN_POINT('Ctrl Pts',(-30.8637971116759,55.9636286201302,4.66610429807113));
#30795=CARTESIAN_POINT('Ctrl Pts',(-30.7553970503824,56.5043367248119,4.70315026159382));
#30796=CARTESIAN_POINT('Ctrl Pts',(-30.9415351902204,57.1040932485588,4.7401962251165));
#30797=CARTESIAN_POINT('Ctrl Pts',(-31.3370243602463,57.488416218779,4.77724218863918));
#30798=CARTESIAN_POINT('Ctrl Pts',(-31.7325135302723,57.8727391889992,4.81428815216186));
#30799=CARTESIAN_POINT('Ctrl Pts',(-32.3373537304862,58.0416286056926,4.85133411568454));
#30800=CARTESIAN_POINT('Ctrl Pts',(-32.8747364051652,57.9177912669505,4.88838007920722));
#30801=CARTESIAN_POINT('Ctrl Pts',(-33.0347855041357,57.880908696264,4.89941350726822));
#30802=CARTESIAN_POINT('Ctrl Pts',(-33.1888509066774,57.8180603341073,4.91044693532922));
#30803=CARTESIAN_POINT('Ctrl Pts',(-33.3312509399777,57.7342826871321,4.92148036339022));
#30804=CARTESIAN_POINT('Ctrl Pts',(-33.3320164235939,57.7319854708823,4.72851963660978));
#30805=CARTESIAN_POINT('Ctrl Pts',(-33.0706605734929,57.8821688027457,4.70843756910068));
#30806=CARTESIAN_POINT('Ctrl Pts',(-32.7702470049871,57.965297344832,4.68835550159159));
#30807=CARTESIAN_POINT('Ctrl Pts',(-32.4713490172715,57.9601647997737,4.6682734340825));
#30808=CARTESIAN_POINT('Ctrl Pts',(-31.919963362139,57.9506966473077,4.63122747055982));
#30809=CARTESIAN_POINT('Ctrl Pts',(-31.3737352640037,57.6408739439502,4.59418150703713));
#30810=CARTESIAN_POINT('Ctrl Pts',(-31.0826491087611,57.1724888068711,4.55713554351445));
#30811=CARTESIAN_POINT('Ctrl Pts',(-30.7915629535184,56.704103669792,4.52008957999177));
#30812=CARTESIAN_POINT('Ctrl Pts',(-30.7556187411683,56.0771560989914,4.48304361646909));
#30813=CARTESIAN_POINT('Ctrl Pts',(-30.9912665445818,55.5785722051981,4.44599765294641));
#30814=CARTESIAN_POINT('Ctrl Pts',(-31.2269143479953,55.0799883114048,4.40895168942373));
#30815=CARTESIAN_POINT('Ctrl Pts',(-31.7341541671722,54.7097680946189,4.37190572590105));
#30816=CARTESIAN_POINT('Ctrl Pts',(-32.2808448224847,54.6373449363853,4.33485976237837));
#30817=CARTESIAN_POINT('Ctrl Pts',(-32.8275354777971,54.5649217781517,4.29781379885569));
#30818=CARTESIAN_POINT('Ctrl Pts',(-33.413676969245,54.7902956784704,4.26076783533301));
#30819=CARTESIAN_POINT('Ctrl Pts',(-33.7710183196873,55.2103229938828,4.22372187181033));
#30820=CARTESIAN_POINT('Ctrl Pts',(-34.1283596701297,55.6303503092951,4.18667590828765));
#30821=CARTESIAN_POINT('Ctrl Pts',(-34.2569008795666,56.2450310398012,4.14962994476497));
#30822=CARTESIAN_POINT('Ctrl Pts',(-34.0978143345866,56.7730530636186,4.11258398124229));
#30823=CARTESIAN_POINT('Ctrl Pts',(-33.9774817812581,57.1724472320418,4.08456253303145));
#30824=CARTESIAN_POINT('Ctrl Pts',(-33.6925870013811,57.5222608245174,4.05654108482062));
#30825=CARTESIAN_POINT('Ctrl Pts',(-33.3316044198825,57.73507921,4.02851963660978));
#30826=CARTESIAN_POINT('Origin',(-32.5,56.2916512459885,3.));
#30827=CARTESIAN_POINT('',(-33.3347454964365,57.7363721546008,3.32851963660978));
#30828=CARTESIAN_POINT('',(-33.333716562894,57.7328365508938,3.52148036339022));
#30829=CARTESIAN_POINT('',(-33.333,57.7344495686934,3.));
#30830=CARTESIAN_POINT('Ctrl Pts',(-33.333716562894,57.7328365508938,3.52148036339022));
#30831=CARTESIAN_POINT('Ctrl Pts',(-33.4781004639345,57.6510402790884,3.53256203972372));
#30832=CARTESIAN_POINT('Ctrl Pts',(-33.6100888264908,57.5485020789653,3.54364371605722));
#30833=CARTESIAN_POINT('Ctrl Pts',(-33.7223873369832,57.4276653019286,3.55472539239072));
#30834=CARTESIAN_POINT('Ctrl Pts',(-34.0978004421986,57.0237088336489,3.5917713559134));
#30835=CARTESIAN_POINT('Ctrl Pts',(-34.2531676277225,56.4152547808823,3.62881731943608));
#30836=CARTESIAN_POINT('Ctrl Pts',(-34.1173842201124,55.8807655910479,3.66586328295876));
#30837=CARTESIAN_POINT('Ctrl Pts',(-33.9816008125024,55.3462764012135,3.70290924648144));
#30838=CARTESIAN_POINT('Ctrl Pts',(-33.5546668117583,54.8857520743114,3.73995521000412));
#30839=CARTESIAN_POINT('Ctrl Pts',(-33.0319709841926,54.709954179896,3.7770011735268));
#30840=CARTESIAN_POINT('Ctrl Pts',(-32.5092751566268,54.5341562854806,3.81404713704948));
#30841=CARTESIAN_POINT('Ctrl Pts',(-31.8908175022394,54.643084823552,3.85109310057216));
#30842=CARTESIAN_POINT('Ctrl Pts',(-31.4596386734712,54.9868880310005,3.88813906409484));
#30843=CARTESIAN_POINT('Ctrl Pts',(-31.0284598447031,55.330691238449,3.92518502761752));
#30844=CARTESIAN_POINT('Ctrl Pts',(-30.7845598415543,55.9093691152746,3.9622309911402));
#30845=CARTESIAN_POINT('Ctrl Pts',(-30.8395608834388,56.4580864498103,3.99927695466289));
#30846=CARTESIAN_POINT('Ctrl Pts',(-30.8945619253233,57.0068037843461,4.03632291818557));
#30847=CARTESIAN_POINT('Ctrl Pts',(-31.2484640122411,57.525560576592,4.07336888170825));
#30848=CARTESIAN_POINT('Ctrl Pts',(-31.7393018474209,57.7769448390475,4.11041484523093));
#30849=CARTESIAN_POINT('Ctrl Pts',(-32.2298200515887,58.0281654013957,4.14743668461736));
#30850=CARTESIAN_POINT('Ctrl Pts',(-32.8570957184112,58.0123615437382,4.18445852400379));
#30851=CARTESIAN_POINT('Ctrl Pts',(-33.3343856149812,57.7368361019314,4.22148036339022));
#30852=CARTESIAN_POINT('Ctrl Pts',(-33.3316044198825,57.73507921,4.02851963660978));
#30853=CARTESIAN_POINT('Ctrl Pts',(-33.2153473010665,57.8036189501297,4.01949512129794));
#30854=CARTESIAN_POINT('Ctrl Pts',(-33.0911982807713,57.8579494129027,4.01047060598609));
#30855=CARTESIAN_POINT('Ctrl Pts',(-32.9621127685743,57.8951505902149,4.00144609067424));
#30856=CARTESIAN_POINT('Ctrl Pts',(-32.4322120469391,58.0478627758654,3.96440012715156));
#30857=CARTESIAN_POINT('Ctrl Pts',(-31.8191249030656,57.9119238300377,3.92735416362888));
#30858=CARTESIAN_POINT('Ctrl Pts',(-31.4034341447795,57.5495469821188,3.8903082001062));
#30859=CARTESIAN_POINT('Ctrl Pts',(-30.9877433864933,57.1871701341999,3.85326223658352));
#30860=CARTESIAN_POINT('Ctrl Pts',(-30.7694490137945,56.5983553841898,3.81621627306084));
#30861=CARTESIAN_POINT('Ctrl Pts',(-30.8484546841662,56.0525771412361,3.77917030953816));
#30862=CARTESIAN_POINT('Ctrl Pts',(-30.9274603545379,55.5067988982823,3.74212434601548));
#30863=CARTESIAN_POINT('Ctrl Pts',(-31.3037660679802,55.0040571623848,3.7050783824928));
#30864=CARTESIAN_POINT('Ctrl Pts',(-31.8051533809355,54.7744345397173,3.66803241897012));
#30865=CARTESIAN_POINT('Ctrl Pts',(-32.3065406938908,54.5448119170498,3.63098645544744));
#30866=CARTESIAN_POINT('Ctrl Pts',(-32.9330096063591,54.5883084076123,3.59394049192476));
#30867=CARTESIAN_POINT('Ctrl Pts',(-33.3978530682301,54.8850175958567,3.55689452840208));
#30868=CARTESIAN_POINT('Ctrl Pts',(-33.862696530101,55.181726784101,3.5198485648794));
#30869=CARTESIAN_POINT('Ctrl Pts',(-34.1659145413746,55.7316486700272,3.48280260135672));
#30870=CARTESIAN_POINT('Ctrl Pts',(-34.1687376598278,56.2831083842721,3.44575663783404));
#30871=CARTESIAN_POINT('Ctrl Pts',(-34.1715607782811,56.834568098517,3.40871067431136));
#30872=CARTESIAN_POINT('Ctrl Pts',(-33.873989003914,57.3875656410806,3.37166471078867));
#30873=CARTESIAN_POINT('Ctrl Pts',(-33.4122077466127,57.6890185508992,3.33461874726599));
#30874=CARTESIAN_POINT('Ctrl Pts',(-33.3868657595293,57.7055619155899,3.33258571038059));
#30875=CARTESIAN_POINT('Ctrl Pts',(-33.3610292261422,57.7213477085124,3.33055267349519));
#30876=CARTESIAN_POINT('Ctrl Pts',(-33.3347454964365,57.7363721546008,3.32851963660978));
#30877=CARTESIAN_POINT('Origin',(-32.5,56.2916512459885,3.));
#30878=CARTESIAN_POINT('',(-33.333130190179,57.7323221393285,2.62851963660978));
#30879=CARTESIAN_POINT('',(-33.3311289428234,57.7328938252549,2.82148036339022));
#30880=CARTESIAN_POINT('',(-33.333,57.7344495686934,3.));
#30881=CARTESIAN_POINT('Ctrl Pts',(-33.3311289428234,57.7328938252549,2.82148036339022));
#30882=CARTESIAN_POINT('Ctrl Pts',(-33.6180096158229,57.5655068353994,2.84361959192097));
#30883=CARTESIAN_POINT('Ctrl Pts',(-33.8582224621032,57.3156647118177,2.86575882045172));
#30884=CARTESIAN_POINT('Ctrl Pts',(-34.0018785934241,57.0190572038434,2.88789804898247));
#30885=CARTESIAN_POINT('Ctrl Pts',(-34.2422609442965,56.5227386033237,2.92494401250515));
#30886=CARTESIAN_POINT('Ctrl Pts',(-34.2122852455117,55.8954772908327,2.96198997602783));
#30887=CARTESIAN_POINT('Ctrl Pts',(-33.9256700455925,55.4243429628454,2.99903593955051));
#30888=CARTESIAN_POINT('Ctrl Pts',(-33.6390548456733,54.9532086348582,3.03608190307319));
#30889=CARTESIAN_POINT('Ctrl Pts',(-33.0958001446196,54.6382012913747,3.07312786659587));
#30890=CARTESIAN_POINT('Ctrl Pts',(-32.5445295368321,54.6234858293533,3.11017383011855));
#30891=CARTESIAN_POINT('Ctrl Pts',(-31.9932589290447,54.6087703673319,3.14721979364123));
#30892=CARTESIAN_POINT('Ctrl Pts',(-31.4339724145236,54.8943467867725,3.18426575716391));
#30893=CARTESIAN_POINT('Ctrl Pts',(-31.1226306380099,55.3495194199898,3.22131172068659));
#30894=CARTESIAN_POINT('Ctrl Pts',(-30.8112888614961,55.8046920532072,3.25835768420927));
#30895=CARTESIAN_POINT('Ctrl Pts',(-30.7478918229898,56.4294609002012,3.29540364773196));
#30896=CARTESIAN_POINT('Ctrl Pts',(-30.9614535366484,56.9378969554647,3.33244961125464));
#30897=CARTESIAN_POINT('Ctrl Pts',(-31.175015250307,57.4463330107282,3.36949557477732));
#30898=CARTESIAN_POINT('Ctrl Pts',(-31.6655357161305,57.8384362742609,3.40654153829999));
#30899=CARTESIAN_POINT('Ctrl Pts',(-32.2085254614957,57.934758464131,3.44358750182267));
#30900=CARTESIAN_POINT('Ctrl Pts',(-32.5890889655549,58.0022674924478,3.46955178901185));
#30901=CARTESIAN_POINT('Ctrl Pts',(-32.9954261310775,57.9244846218395,3.49551607620104));
#30902=CARTESIAN_POINT('Ctrl Pts',(-33.333716562894,57.7328365508938,3.52148036339022));
#30903=CARTESIAN_POINT('Ctrl Pts',(-33.3347454964365,57.7363721546008,3.32851963660978));
#30904=CARTESIAN_POINT('Ctrl Pts',(-32.8820875508044,57.9951229094133,3.2935067099725));
#30905=CARTESIAN_POINT('Ctrl Pts',(-32.2967926538179,58.0280607074246,3.25849378333523));
#30906=CARTESIAN_POINT('Ctrl Pts',(-31.8207237377836,57.8159025761185,3.22348085669795));
#30907=CARTESIAN_POINT('Ctrl Pts',(-31.3170117264914,57.5914254144454,3.18643489317527));
#30908=CARTESIAN_POINT('Ctrl Pts',(-30.9355784441425,57.0925628140254,3.14938892965259));
#30909=CARTESIAN_POINT('Ctrl Pts',(-30.8509889952779,56.547622072684,3.11234296612991));
#30910=CARTESIAN_POINT('Ctrl Pts',(-30.7663995464132,56.0026813313427,3.07529700260723));
#30911=CARTESIAN_POINT('Ctrl Pts',(-30.9786539310327,55.41166244908,3.03825103908455));
#30912=CARTESIAN_POINT('Ctrl Pts',(-31.390612726451,55.0450485686685,3.00120507556187));
#30913=CARTESIAN_POINT('Ctrl Pts',(-31.8025715218694,54.678434688257,2.96415911203919));
#30914=CARTESIAN_POINT('Ctrl Pts',(-32.4142347280865,54.5362258096967,2.92711314851651));
#30915=CARTESIAN_POINT('Ctrl Pts',(-32.9456712104109,54.6835046326399,2.89006718499383));
#30916=CARTESIAN_POINT('Ctrl Pts',(-33.4771076927354,54.8307834555831,2.85302122147115));
#30917=CARTESIAN_POINT('Ctrl Pts',(-33.9283174511671,55.2675499800297,2.81597525794846));
#30918=CARTESIAN_POINT('Ctrl Pts',(-34.0928017812264,55.7939155294323,2.77892929442578));
#30919=CARTESIAN_POINT('Ctrl Pts',(-34.2572861112858,56.3202810788348,2.7418833309031));
#30920=CARTESIAN_POINT('Ctrl Pts',(-34.1350450129728,56.9362456531931,2.70483736738042));
#30921=CARTESIAN_POINT('Ctrl Pts',(-33.7820228180846,57.3599095722955,2.66779140385774));
#30922=CARTESIAN_POINT('Ctrl Pts',(-33.6572786340789,57.509615768241,2.65470081477509));
#30923=CARTESIAN_POINT('Ctrl Pts',(-33.5037182424927,57.6353105712173,2.64161022569243));
#30924=CARTESIAN_POINT('Ctrl Pts',(-33.333130190179,57.7323221393285,2.62851963660978));
#30925=CARTESIAN_POINT('Origin',(-32.5,56.2916512459885,3.));
#30926=CARTESIAN_POINT('',(-33.3310982842581,57.7335685916211,1.92851963660978));
#30927=CARTESIAN_POINT('',(-33.3331738820164,57.7367002116855,2.12148036339022));
#30928=CARTESIAN_POINT('',(-33.333,57.7344495686934,3.));
#30929=CARTESIAN_POINT('Ctrl Pts',(-33.3331738820164,57.7367002116855,2.12148036339022));
#30930=CARTESIAN_POINT('Ctrl Pts',(-33.7599095781773,57.4863532801825,2.15467714411822));
#30931=CARTESIAN_POINT('Ctrl Pts',(-34.0737470619129,57.0348072848651,2.18787392484622));
#30932=CARTESIAN_POINT('Ctrl Pts',(-34.1491952727494,56.5464328961311,2.22107070557422));
#30933=CARTESIAN_POINT('Ctrl Pts',(-34.233391740154,56.0014312606204,2.2581166690969));
#30934=CARTESIAN_POINT('Ctrl Pts',(-34.0207112033876,55.4105655517268,2.29516263261958));
#30935=CARTESIAN_POINT('Ctrl Pts',(-33.608488116082,55.0442488115619,2.33220859614226));
#30936=CARTESIAN_POINT('Ctrl Pts',(-33.1962650287764,54.6779320713971,2.36925455966494));
#30937=CARTESIAN_POINT('Ctrl Pts',(-32.5844993909317,54.5361642999609,2.40630052318762));
#30938=CARTESIAN_POINT('Ctrl Pts',(-32.0531692156545,54.6838263217292,2.4433464867103));
#30939=CARTESIAN_POINT('Ctrl Pts',(-31.5218390403773,54.8314883434974,2.48039245023298));
#30940=CARTESIAN_POINT('Ctrl Pts',(-31.0709443276677,55.2685801584701,2.51743841375566));
#30941=CARTESIAN_POINT('Ctrl Pts',(-30.9068395995442,55.7950642190458,2.55448437727834));
#30942=CARTESIAN_POINT('Ctrl Pts',(-30.7427348714206,56.3215482796215,2.59153034080102));
#30943=CARTESIAN_POINT('Ctrl Pts',(-30.8654201278831,56.9374245858002,2.6285763043237));
#30944=CARTESIAN_POINT('Ctrl Pts',(-31.2187477656388,57.360833853803,2.66562226784638));
#30945=CARTESIAN_POINT('Ctrl Pts',(-31.5720754033946,57.7842431218059,2.70266823136906));
#30946=CARTESIAN_POINT('Ctrl Pts',(-32.1560454224436,58.0151853516328,2.73971419489175));
#30947=CARTESIAN_POINT('Ctrl Pts',(-32.7034006322329,57.9479685222721,2.77676015841443));
#30948=CARTESIAN_POINT('Ctrl Pts',(-32.9236480838557,57.9209214875348,2.79166689340636));
#30949=CARTESIAN_POINT('Ctrl Pts',(-33.1379671006766,57.845598452492,2.80657362839829));
#30950=CARTESIAN_POINT('Ctrl Pts',(-33.3311289428234,57.7328938252549,2.82148036339022));
#30951=CARTESIAN_POINT('Ctrl Pts',(-33.333130190179,57.7323221393285,2.62851963660978));
#30952=CARTESIAN_POINT('Ctrl Pts',(-33.0209593136532,57.9098503181175,2.60456426216975));
#30953=CARTESIAN_POINT('Ctrl Pts',(-32.6517664254568,57.9913244481799,2.58060888772973));
#30954=CARTESIAN_POINT('Ctrl Pts',(-32.2977938304223,57.9481146542165,2.5566535132897));
#30955=CARTESIAN_POINT('Ctrl Pts',(-31.7503903291117,57.8812925531888,2.51960754976702));
#30956=CARTESIAN_POINT('Ctrl Pts',(-31.2393866179539,57.5162850872868,2.48256158624434));
#30957=CARTESIAN_POINT('Ctrl Pts',(-30.9986464429484,57.0201399930138,2.44551562272166));
#30958=CARTESIAN_POINT('Ctrl Pts',(-30.7579062679429,56.5239948987407,2.40846965919898));
#30959=CARTESIAN_POINT('Ctrl Pts',(-30.7874296290898,55.8967121760965,2.3714236956763));
#30960=CARTESIAN_POINT('Ctrl Pts',(-31.0737049927512,55.4253713200344,2.33437773215362));
#30961=CARTESIAN_POINT('Ctrl Pts',(-31.3599803564127,54.9540304639722,2.29733176863094));
#30962=CARTESIAN_POINT('Ctrl Pts',(-31.9030077225887,54.6386314744921,2.26028580510826));
#30963=CARTESIAN_POINT('Ctrl Pts',(-32.4542675379743,54.6235184875634,2.22323984158558));
#30964=CARTESIAN_POINT('Ctrl Pts',(-33.00552735336,54.6084055006347,2.1861938780629));
#30965=CARTESIAN_POINT('Ctrl Pts',(-33.5650196179551,54.8935785162575,2.14914791454022));
#30966=CARTESIAN_POINT('Ctrl Pts',(-33.8766895243309,55.3485264867911,2.11210195101753));
#30967=CARTESIAN_POINT('Ctrl Pts',(-34.1883594307067,55.8034744573246,2.07505598749485));
#30968=CARTESIAN_POINT('Ctrl Pts',(-34.2522069788632,56.4281973827689,2.03801002397217));
#30969=CARTESIAN_POINT('Ctrl Pts',(-34.0390119763463,56.9367872738744,2.00096406044949));
#30970=CARTESIAN_POINT('Ctrl Pts',(-33.9000423680165,57.2683078870831,1.97681591916959));
#30971=CARTESIAN_POINT('Ctrl Pts',(-33.6433576792834,57.550483699497,1.95266777788969));
#30972=CARTESIAN_POINT('Ctrl Pts',(-33.3310982842581,57.7335685916211,1.92851963660978));
#30973=CARTESIAN_POINT('Origin',(-32.5,56.2916512459885,3.));
#30974=CARTESIAN_POINT('',(-33.3338545267451,57.7369307977834,1.22851963660978));
#30975=CARTESIAN_POINT('',(-33.3345984319871,57.7343006412916,1.42148036339021));
#30976=CARTESIAN_POINT('',(-33.333,57.7344495686934,3.));
#30977=CARTESIAN_POINT('Ctrl Pts',(-33.3345984319871,57.7343006412916,1.42148036339021));
#30978=CARTESIAN_POINT('Ctrl Pts',(-33.4283251997872,57.6813267445322,1.42868873279278));
#30979=CARTESIAN_POINT('Ctrl Pts',(-33.5166388707303,57.6193252564529,1.43589710219535));
#30980=CARTESIAN_POINT('Ctrl Pts',(-33.5974727328826,57.5487559900283,1.44310547159792));
#30981=CARTESIAN_POINT('Ctrl Pts',(-34.0129020958151,57.1860794506077,1.4801514351206));
#30982=CARTESIAN_POINT('Ctrl Pts',(-34.2307718231603,56.5971073981534,1.51719739864329));
#30983=CARTESIAN_POINT('Ctrl Pts',(-34.1513725987927,56.0513862321698,1.55424336216597));
#30984=CARTESIAN_POINT('Ctrl Pts',(-34.071973374425,55.5056650661861,1.59128932568865));
#30985=CARTESIAN_POINT('Ctrl Pts',(-33.6953051983445,55.0031947866731,1.62833528921133));
#30986=CARTESIAN_POINT('Ctrl Pts',(-33.1937523971885,54.7739337662501,1.66538125273401));
#30987=CARTESIAN_POINT('Ctrl Pts',(-32.6921995960325,54.5446727458271,1.70242721625669));
#30988=CARTESIAN_POINT('Ctrl Pts',(-32.0657621698011,54.5886209844942,1.73947317977937));
#30989=CARTESIAN_POINT('Ctrl Pts',(-31.6011327587506,54.8856653216219,1.77651914330205));
#30990=CARTESIAN_POINT('Ctrl Pts',(-31.1365033477001,55.1827096587496,1.81356510682473));
#30991=CARTESIAN_POINT('Ctrl Pts',(-30.8336819518306,55.7328500943379,1.85061107034741));
#30992=CARTESIAN_POINT('Ctrl Pts',(-30.831256500076,56.2843117385313,1.88765703387009));
#30993=CARTESIAN_POINT('Ctrl Pts',(-30.8288310483213,56.8357733827248,1.92470299739277));
#30994=CARTESIAN_POINT('Ctrl Pts',(-31.1268015406815,57.3885562355234,1.96174896091545));
#30995=CARTESIAN_POINT('Ctrl Pts',(-31.5888000917203,57.689676089852,1.99879492443813));
#30996=CARTESIAN_POINT('Ctrl Pts',(-32.050798642759,57.9907959441805,2.03584088796081));
#30997=CARTESIAN_POINT('Ctrl Pts',(-32.6768252524764,58.040252800039,2.07288685148349));
#30998=CARTESIAN_POINT('Ctrl Pts',(-33.1803752931228,57.8154124469043,2.10993281500617));
#30999=CARTESIAN_POINT('Ctrl Pts',(-33.2326955992617,57.7920508836856,2.11378199780085));
#31000=CARTESIAN_POINT('Ctrl Pts',(-33.2836936714804,57.7657280595765,2.11763118059554));
#31001=CARTESIAN_POINT('Ctrl Pts',(-33.3331738820164,57.7367002116855,2.12148036339022));
#31002=CARTESIAN_POINT('Ctrl Pts',(-33.3310982842581,57.7335685916211,1.92851963660978));
#31003=CARTESIAN_POINT('Ctrl Pts',(-33.1643166622694,57.8313565069137,1.91562181436701));
#31004=CARTESIAN_POINT('Ctrl Pts',(-32.9816809059178,57.900876152894,1.90272399212423));
#31005=CARTESIAN_POINT('Ctrl Pts',(-32.792659312829,57.9345477382935,1.88982616988145));
#31006=CARTESIAN_POINT('Ctrl Pts',(-32.2497392050189,58.0312614548405,1.85278020635877));
#31007=CARTESIAN_POINT('Ctrl Pts',(-31.6541365425887,57.8322320311677,1.81573424283609));
#31008=CARTESIAN_POINT('Ctrl Pts',(-31.2784322612969,57.4285464115925,1.77868827931341));
#31009=CARTESIAN_POINT('Ctrl Pts',(-30.902727980005,57.0248607920173,1.74164231579073));
#31010=CARTESIAN_POINT('Ctrl Pts',(-30.7469220798514,56.4165189765397,1.70459635226805));
#31011=CARTESIAN_POINT('Ctrl Pts',(-30.8823200145203,55.8819320465459,1.66755038874537));
#31012=CARTESIAN_POINT('Ctrl Pts',(-31.0177179491892,55.3473451165522,1.63050442522269));
#31013=CARTESIAN_POINT('Ctrl Pts',(-31.4443197186808,54.8865130720423,1.59345846170001));
#31014=CARTESIAN_POINT('Ctrl Pts',(-31.9668886041916,54.7103383112811,1.55641249817733));
#31015=CARTESIAN_POINT('Ctrl Pts',(-32.4894574897024,54.53416355052,1.51936653465465));
#31016=CARTESIAN_POINT('Ctrl Pts',(-33.1079934912324,54.6426460735076,1.48232057113197));
#31017=CARTESIAN_POINT('Ctrl Pts',(-33.5394201003418,54.9861382384619,1.44527460760928));
#31018=CARTESIAN_POINT('Ctrl Pts',(-33.9708467094511,55.3296304034162,1.4082286440866));
#31019=CARTESIAN_POINT('Ctrl Pts',(-34.2151639261398,55.9081322103372,1.37118268056392));
#31020=CARTESIAN_POINT('Ctrl Pts',(-34.1605585908214,56.4568890269572,1.33413671704124));
#31021=CARTESIAN_POINT('Ctrl Pts',(-34.1086657929391,56.9783861738082,1.29893102356409));
#31022=CARTESIAN_POINT('Ctrl Pts',(-33.7868109567046,57.4730201142583,1.26372533008693));
#31023=CARTESIAN_POINT('Ctrl Pts',(-33.3338545267451,57.7369307977834,1.22851963660978));
#31024=CARTESIAN_POINT('Origin',(-32.5,56.2916512459885,3.));
#31025=CARTESIAN_POINT('',(-33.3341985401264,57.7334817014241,0.528519636609781));
#31026=CARTESIAN_POINT('',(-33.3317031312748,57.7320766758176,0.721480363390217));
#31027=CARTESIAN_POINT('',(-33.333,57.7344495686934,3.));
#31028=CARTESIAN_POINT('Ctrl Pts',(-33.3317031312748,57.7320766758176,0.721480363390217));
#31029=CARTESIAN_POINT('Ctrl Pts',(-33.5692173042018,57.5950551525707,0.739746284990036));
#31030=CARTESIAN_POINT('Ctrl Pts',(-33.7746291238346,57.4025124831788,0.758012206589854));
#31031=CARTESIAN_POINT('Ctrl Pts',(-33.9179858048945,57.1714665641067,0.776278128189673));
#31032=CARTESIAN_POINT('Ctrl Pts',(-34.208734144542,56.7028716102066,0.813324091712354));
#31033=CARTESIAN_POINT('Ctrl Pts',(-34.2442262482397,56.0758982397685,0.850370055235033));
#31034=CARTESIAN_POINT('Ctrl Pts',(-34.0082189534411,55.5774843709491,0.887416018757714));
#31035=CARTESIAN_POINT('Ctrl Pts',(-33.7722116586424,55.0790705021297,0.924461982280394));
#31036=CARTESIAN_POINT('Ctrl Pts',(-33.2647049653473,54.7092161349289,0.961507945803076));
#31037=CARTESIAN_POINT('Ctrl Pts',(-32.7179621895189,54.6371872177157,0.998553909325756));
#31038=CARTESIAN_POINT('Ctrl Pts',(-32.1712194136904,54.5651583005025,1.03559987284844));
#31039=CARTESIAN_POINT('Ctrl Pts',(-31.5852405553285,54.7909548332769,1.07264583637112));
#31040=CARTESIAN_POINT('Ctrl Pts',(-31.2282021616797,55.21123975246,1.1096917998938));
#31041=CARTESIAN_POINT('Ctrl Pts',(-30.8711637680309,55.631524671643,1.14673776341648));
#31042=CARTESIAN_POINT('Ctrl Pts',(-30.7430658390951,56.2462979772347,1.18378372693916));
#31043=CARTESIAN_POINT('Ctrl Pts',(-30.902533118419,56.7742051799299,1.22082969046184));
#31044=CARTESIAN_POINT('Ctrl Pts',(-31.0620003977429,57.3021123826251,1.25787565398452));
#31045=CARTESIAN_POINT('Ctrl Pts',(-31.5090328853265,57.7431534824239,1.2949216175072));
#31046=CARTESIAN_POINT('Ctrl Pts',(-32.0390436283783,57.8954835191298,1.33196758102988));
#31047=CARTESIAN_POINT('Ctrl Pts',(-32.4659253700502,58.0181733178376,1.36180517514999));
#31048=CARTESIAN_POINT('Ctrl Pts',(-32.9466353435787,57.9535754234504,1.3916427692701));
#31049=CARTESIAN_POINT('Ctrl Pts',(-33.3345984319871,57.7343006412916,1.42148036339021));
#31050=CARTESIAN_POINT('Ctrl Pts',(-33.3338545267451,57.7369307977834,1.22851963660978));
#31051=CARTESIAN_POINT('Ctrl Pts',(-33.3101776135059,57.7507259223106,1.22667936656425));
#31052=CARTESIAN_POINT('Ctrl Pts',(-33.2861424840206,57.7638906287274,1.22483909651873));
#31053=CARTESIAN_POINT('Ctrl Pts',(-33.261768971111,57.776395800606,1.2229988264732));
#31054=CARTESIAN_POINT('Ctrl Pts',(-32.7711125740444,58.0281339313158,1.18595286295052));
#31055=CARTESIAN_POINT('Ctrl Pts',(-32.1433276672366,58.0125983664166,1.14890689942784));
#31056=CARTESIAN_POINT('Ctrl Pts',(-31.6657235730869,57.7368990452689,1.11186093590516));
#31057=CARTESIAN_POINT('Ctrl Pts',(-31.1881194789371,57.4611997241213,1.07481497238248));
#31058=CARTESIAN_POINT('Ctrl Pts',(-30.8606961974455,56.9253366467254,1.0377690088598));
#31059=CARTESIAN_POINT('Ctrl Pts',(-30.8333008499707,56.3745505890176,1.00072304533712));
#31060=CARTESIAN_POINT('Ctrl Pts',(-30.8059055024959,55.8237645313099,0.963677081814436));
#31061=CARTESIAN_POINT('Ctrl Pts',(-31.0785380890379,55.2580554932903,0.926631118291755));
#31062=CARTESIAN_POINT('Ctrl Pts',(-31.526426760498,54.9363234239653,0.889585154769075));
#31063=CARTESIAN_POINT('Ctrl Pts',(-31.9743154319581,54.6145913546402,0.852539191246395));
#31064=CARTESIAN_POINT('Ctrl Pts',(-32.5974601883362,54.5368362540097,0.815493227723714));
#31065=CARTESIAN_POINT('Ctrl Pts',(-33.1106752982773,54.7386431848418,0.778447264201034));
#31066=CARTESIAN_POINT('Ctrl Pts',(-33.6238904082183,54.940450115674,0.741401300678353));
#31067=CARTESIAN_POINT('Ctrl Pts',(-34.0271758717221,55.4218190779688,0.704355337155672));
#31068=CARTESIAN_POINT('Ctrl Pts',(-34.1359658098863,55.9624488364586,0.667309373632992));
#31069=CARTESIAN_POINT('Ctrl Pts',(-34.2447557480506,56.5030785949484,0.630263410110312));
#31070=CARTESIAN_POINT('Ctrl Pts',(-34.0590501608752,57.1029691496333,0.593217446587631));
#31071=CARTESIAN_POINT('Ctrl Pts',(-33.6638382628473,57.4875771868012,0.556171483064951));
#31072=CARTESIAN_POINT('Ctrl Pts',(-33.5655069136947,57.5832702248356,0.546954200913227));
#31073=CARTESIAN_POINT('Ctrl Pts',(-33.4542061287358,57.6656362524338,0.537736918761504));
#31074=CARTESIAN_POINT('Ctrl Pts',(-33.3341985401264,57.7334817014241,0.528519636609781));
#31075=CARTESIAN_POINT('Origin',(-32.5,56.2916512459885,3.));
#31076=CARTESIAN_POINT('',(-33.3313285320323,57.7324067450656,-0.171480363390219));
#31077=CARTESIAN_POINT('',(-33.3319271105623,57.7355745198861,0.0214803633902191));
#31078=CARTESIAN_POINT('',(-33.333,57.7344495686934,3.));
#31079=CARTESIAN_POINT('Ctrl Pts',(-33.3319271105623,57.7355745198861,0.0214803633902191));
#31080=CARTESIAN_POINT('Ctrl Pts',(-33.7093130799579,57.5130220094248,0.0508038371872872));
#31081=CARTESIAN_POINT('Ctrl Pts',(-34.0025116805638,57.1388573741433,0.0801273109843555));
#31082=CARTESIAN_POINT('Ctrl Pts',(-34.1137073818815,56.7167479649787,0.109450784781424));
#31083=CARTESIAN_POINT('Ctrl Pts',(-34.254187050948,56.1834738419088,0.146496748304104));
#31084=CARTESIAN_POINT('Ctrl Pts',(-34.1041780082168,55.5736766763093,0.183542711826784));
#31085=CARTESIAN_POINT('Ctrl Pts',(-33.7323327404969,55.1664335984773,0.220588675349465));
#31086=CARTESIAN_POINT('Ctrl Pts',(-33.360487472777,54.7591905206453,0.257634638872145));
#31087=CARTESIAN_POINT('Ctrl Pts',(-32.7668059800683,54.5545015305809,0.294680602394826));
#31088=CARTESIAN_POINT('Ctrl Pts',(-32.2229899650202,54.6460437054155,0.331726565917507));
#31089=CARTESIAN_POINT('Ctrl Pts',(-31.6791739499721,54.7375858802501,0.368772529440187));
#31090=CARTESIAN_POINT('Ctrl Pts',(-31.1852234125845,55.1253592199837,0.405818492962867));
#31091=CARTESIAN_POINT('Ctrl Pts',(-30.9671976166263,55.6318970567811,0.442864456485548));
#31092=CARTESIAN_POINT('Ctrl Pts',(-30.7491718206681,56.1384348935784,0.479910420008228));
#31093=CARTESIAN_POINT('Ctrl Pts',(-30.8070707661393,56.7637372274395,0.516956383530909));
#31094=CARTESIAN_POINT('Ctrl Pts',(-31.1143966726152,57.2216308996084,0.55400234705359));
#31095=CARTESIAN_POINT('Ctrl Pts',(-31.4217225790911,57.6795245717774,0.59104831057627));
#31096=CARTESIAN_POINT('Ctrl Pts',(-31.9784754465718,57.9700095822542,0.62809427409895));
#31097=CARTESIAN_POINT('Ctrl Pts',(-32.5298541681108,57.9601438188116,0.665140237621631));
#31098=CARTESIAN_POINT('Ctrl Pts',(-32.8093695193456,57.9551424790316,0.683920279544493));
#31099=CARTESIAN_POINT('Ctrl Pts',(-33.0875037843945,57.8729548645719,0.702700321467355));
#31100=CARTESIAN_POINT('Ctrl Pts',(-33.3317031312748,57.7320766758176,0.721480363390217));
#31101=CARTESIAN_POINT('Ctrl Pts',(-33.3341985401264,57.7334817014241,0.528519636609781));
#31102=CARTESIAN_POINT('Ctrl Pts',(-32.9718734110338,57.9383196733276,0.500690955238824));
#31103=CARTESIAN_POINT('Ctrl Pts',(-32.5301815965127,58.010795616536,0.472862273867866));
#31104=CARTESIAN_POINT('Ctrl Pts',(-32.1264363544929,57.9180609610464,0.445033592496909));
#31105=CARTESIAN_POINT('Ctrl Pts',(-31.5889645530468,57.7946111784728,0.407987628974228));
#31106=CARTESIAN_POINT('Ctrl Pts',(-31.1187391590349,57.3783860936747,0.370941665451548));
#31107=CARTESIAN_POINT('Ctrl Pts',(-30.9309614883814,56.8598734778586,0.333895701928867));
#31108=CARTESIAN_POINT('Ctrl Pts',(-30.7431838177278,56.3413608620425,0.296849738406187));
#31109=CARTESIAN_POINT('Ctrl Pts',(-30.8378538704327,55.7205607152083,0.259803774883506));
#31110=CARTESIAN_POINT('Ctrl Pts',(-31.1716453640503,55.2815857427567,0.222757811360826));
#31111=CARTESIAN_POINT('Ctrl Pts',(-31.5054368576679,54.842610770305,0.185711847838145));
#31112=CARTESIAN_POINT('Ctrl Pts',(-32.0783497921982,54.5854609722358,0.148665884315465));
#31113=CARTESIAN_POINT('Ctrl Pts',(-32.6281873065731,54.6278224157042,0.111619920792784));
#31114=CARTESIAN_POINT('Ctrl Pts',(-33.178024820948,54.6701838591725,0.0745739572701037));
#31115=CARTESIAN_POINT('Ctrl Pts',(-33.7047869151673,55.0120565441784,0.0375279937474228));
#31116=CARTESIAN_POINT('Ctrl Pts',(-33.9673979456785,55.4969804900557,0.000482030224742209));
#31117=CARTESIAN_POINT('Ctrl Pts',(-34.2300089761898,55.981904435933,-0.0365639332979384));
#31118=CARTESIAN_POINT('Ctrl Pts',(-34.2284689429929,56.6098796426817,-0.0736098968206187));
#31119=CARTESIAN_POINT('Ctrl Pts',(-33.9634826195406,57.0935097116441,-0.110655860343299));
#31120=CARTESIAN_POINT('Ctrl Pts',(-33.8184586195722,57.3581949459313,-0.130930694692273));
#31121=CARTESIAN_POINT('Ctrl Pts',(-33.5945259126096,57.5796452264349,-0.151205529041246));
#31122=CARTESIAN_POINT('Ctrl Pts',(-33.3313285320323,57.7324067450656,-0.171480363390219));
#31123=CARTESIAN_POINT('Origin',(-32.5,56.2916512459885,3.));
#31124=CARTESIAN_POINT('',(-33.3325354057627,57.7362457052863,-0.87148036339022));
#31125=CARTESIAN_POINT('',(-33.3348489584778,57.7359240281238,-0.678519636609784));
#31126=CARTESIAN_POINT('',(-33.333,57.7344495686934,3.));
#31127=CARTESIAN_POINT('Ctrl Pts',(-33.3348489584778,57.7359240281238,-0.678519636609784));
#31128=CARTESIAN_POINT('Ctrl Pts',(-33.3780386262143,57.7113506256494,-0.675184574138146));
#31129=CARTESIAN_POINT('Ctrl Pts',(-33.4200351242183,57.6847625016212,-0.671849511666509));
#31130=CARTESIAN_POINT('Ctrl Pts',(-33.4606301406774,57.6561836376047,-0.668514449194871));
#31131=CARTESIAN_POINT('Ctrl Pts',(-33.9115606739847,57.3387288484125,-0.631468485672191));
#31132=CARTESIAN_POINT('Ctrl Pts',(-34.1895648369722,56.7756401144087,-0.59442252214951));
#31133=CARTESIAN_POINT('Ctrl Pts',(-34.1674127214773,56.2246182278545,-0.557376558626829));
#31134=CARTESIAN_POINT('Ctrl Pts',(-34.1452606059824,55.6735963413002,-0.520330595104149));
#31135=CARTESIAN_POINT('Ctrl Pts',(-33.8229522120051,55.1346413021956,-0.483284631581468));
#31136=CARTESIAN_POINT('Ctrl Pts',(-33.3479936663214,54.8544089200699,-0.446238668058787));
#31137=CARTESIAN_POINT('Ctrl Pts',(-32.8730351206376,54.5741765379441,-0.409192704536106));
#31138=CARTESIAN_POINT('Ctrl Pts',(-32.2454264232474,54.5526668127973,-0.372146741013426));
#31139=CARTESIAN_POINT('Ctrl Pts',(-31.7523963222819,54.7997238024577,-0.335100777490745));
#31140=CARTESIAN_POINT('Ctrl Pts',(-31.2593662213165,55.0467807921182,-0.298054813968064));
#31141=CARTESIAN_POINT('Ctrl Pts',(-30.9009147167759,55.562404496586,-0.261008850445383));
#31142=CARTESIAN_POINT('Ctrl Pts',(-30.8410891376185,56.1106167986295,-0.223962886922702));
#31143=CARTESIAN_POINT('Ctrl Pts',(-30.7812635584611,56.658829100673,-0.186916923400021));
#31144=CARTESIAN_POINT('Ctrl Pts',(-31.020063904687,57.2396300002921,-0.149870959877341));
#31145=CARTESIAN_POINT('Ctrl Pts',(-31.4482018611622,57.5872126749713,-0.11282499635466));
#31146=CARTESIAN_POINT('Ctrl Pts',(-31.8763398176374,57.9347953496505,-0.0757790328319798));
#31147=CARTESIAN_POINT('Ctrl Pts',(-32.4938153843619,58.0491597993896,-0.0387330693092992));
#31148=CARTESIAN_POINT('Ctrl Pts',(-33.0180373581563,57.8779664839892,-0.00168710578661843));
#31149=CARTESIAN_POINT('Ctrl Pts',(-33.1273150883492,57.8422800422405,0.00603538393899408));
#31150=CARTESIAN_POINT('Ctrl Pts',(-33.2325405477213,57.7941848839699,0.0137578736646066));
#31151=CARTESIAN_POINT('Ctrl Pts',(-33.3319271105623,57.7355745198861,0.0214803633902191));
#31152=CARTESIAN_POINT('Ctrl Pts',(-33.3313285320323,57.7324067450656,-0.171480363390219));
#31153=CARTESIAN_POINT('Ctrl Pts',(-33.1136144342564,57.8587694623943,-0.188251492563927));
#31154=CARTESIAN_POINT('Ctrl Pts',(-32.8690337821938,57.9381324168355,-0.205022621737634));
#31155=CARTESIAN_POINT('Ctrl Pts',(-32.6200250231441,57.9560888015457,-0.221793750911342));
#31156=CARTESIAN_POINT('Ctrl Pts',(-32.0699863639079,57.9957528913089,-0.258839714434022));
#31157=CARTESIAN_POINT('Ctrl Pts',(-31.4983416591433,57.7357961396592,-0.295885677956703));
#31158=CARTESIAN_POINT('Ctrl Pts',(-31.166707224731,57.2951892897454,-0.332931641479383));
#31159=CARTESIAN_POINT('Ctrl Pts',(-30.8350727903188,56.8545824398317,-0.369977605002064));
#31160=CARTESIAN_POINT('Ctrl Pts',(-30.7434486262588,56.233325491654,-0.407023568524745));
#31161=CARTESIAN_POINT('Ctrl Pts',(-30.9337672989981,55.7157400874939,-0.444069532047425));
#31162=CARTESIAN_POINT('Ctrl Pts',(-31.1240859717375,55.1981546833338,-0.481115495570106));
#31163=CARTESIAN_POINT('Ctrl Pts',(-31.5963474812763,54.7842408231913,-0.518161459092787));
#31164=CARTESIAN_POINT('Ctrl Pts',(-32.1344181757785,54.6634287766855,-0.555207422615468));
#31165=CARTESIAN_POINT('Ctrl Pts',(-32.6724888702807,54.5426167301798,-0.592253386138148));
#31166=CARTESIAN_POINT('Ctrl Pts',(-33.2763687497463,54.7149064973108,-0.629299349660829));
#31167=CARTESIAN_POINT('Ctrl Pts',(-33.6696897466081,55.1014482025695,-0.666345313183509));
#31168=CARTESIAN_POINT('Ctrl Pts',(-34.0630107434699,55.4879899078282,-0.70339127670619));
#31169=CARTESIAN_POINT('Ctrl Pts',(-34.2457728577278,56.0887835512146,-0.740437240228871));
#31170=CARTESIAN_POINT('Ctrl Pts',(-34.1343320137705,56.6288734837568,-0.777483203751551));
#31171=CARTESIAN_POINT('Ctrl Pts',(-34.040078625064,57.0856656664133,-0.808815590297774));
#31172=CARTESIAN_POINT('Ctrl Pts',(-33.7353736531391,57.4990347912871,-0.840147976843997));
#31173=CARTESIAN_POINT('Ctrl Pts',(-33.3325354057627,57.7362457052863,-0.87148036339022));
#31174=CARTESIAN_POINT('Origin',(-32.5,56.2916512459885,3.));
#31175=CARTESIAN_POINT('',(-33.3347882996638,57.7351190113229,-1.57148036339022));
#31176=CARTESIAN_POINT('',(-33.3327354544031,57.732107437543,-1.37851963660978));
#31177=CARTESIAN_POINT('',(-33.333,57.7344495686934,3.));
#31178=CARTESIAN_POINT('',(-32.8002165734084,54.652924298309,-2.));
#31179=CARTESIAN_POINT('Ctrl Pts',(-33.3347882996638,57.7351190113229,-1.57148036339022));
#31180=CARTESIAN_POINT('Ctrl Pts',(-32.9233907544682,57.9680931016245,-1.60318235169211));
#31181=CARTESIAN_POINT('Ctrl Pts',(-32.4058309808294,58.0231592569491,-1.634884339994));
#31182=CARTESIAN_POINT('Ctrl Pts',(-31.9592734257388,57.8702645075936,-1.66658632829588));
#31183=CARTESIAN_POINT('Ctrl Pts',(-31.4374400713406,57.6915964299482,-1.70363229181857));
#31184=CARTESIAN_POINT('Ctrl Pts',(-31.0125640599592,57.2289465672061,-1.74067825534125));
#31185=CARTESIAN_POINT('Ctrl Pts',(-30.880071382614,56.6935519519193,-1.77772421886393));
#31186=CARTESIAN_POINT('Ctrl Pts',(-30.7475787052689,56.1581573366325,-1.81477018238661));
#31187=CARTESIAN_POINT('Ctrl Pts',(-30.9074693619599,55.550017968801,-1.85181614590929));
#31188=CARTESIAN_POINT('Ctrl Pts',(-31.2843999047331,55.1487524209429,-1.88886210943197));
#31189=CARTESIAN_POINT('Ctrl Pts',(-31.6613304475062,54.7474868730847,-1.92590807295465));
#31190=CARTESIAN_POINT('Ctrl Pts',(-32.2553008763615,54.5530951451999,-1.96295403647733));
#31191=CARTESIAN_POINT('Ctrl Pts',(-32.8002165734084,54.652924298309,-2.00000000000001));
#31192=CARTESIAN_POINT('',(-34.0720885049226,56.8521739755918,-2.));
#31193=CARTESIAN_POINT('Origin',(-32.5,56.2916512459885,-2.));
#31194=CARTESIAN_POINT('Ctrl Pts',(-34.0720901513885,56.8521746541718,-2.));
#31195=CARTESIAN_POINT('Ctrl Pts',(-34.2530538927521,56.3425577544553,-1.96367708181444));
#31196=CARTESIAN_POINT('Ctrl Pts',(-34.16381751404,55.7359288334825,-1.92735416362889));
#31197=CARTESIAN_POINT('Ctrl Pts',(-33.8426356554965,55.3008256611299,-1.89103124544333));
#31198=CARTESIAN_POINT('Ctrl Pts',(-33.5150603391364,54.857061309124,-1.85398528192065));
#31199=CARTESIAN_POINT('Ctrl Pts',(-32.9462134040812,54.59171946851,-1.81693931839797));
#31200=CARTESIAN_POINT('Ctrl Pts',(-32.3958963008479,54.6261577029506,-1.77989335487529));
#31201=CARTESIAN_POINT('Ctrl Pts',(-31.8455791976147,54.6605959373911,-1.74284739135261));
#31202=CARTESIAN_POINT('Ctrl Pts',(-31.3137919262033,54.9948142468862,-1.70580142782993));
#31203=CARTESIAN_POINT('Ctrl Pts',(-31.0441775058384,55.4758950021693,-1.66875546430725));
#31204=CARTESIAN_POINT('Ctrl Pts',(-30.7745630854735,55.9569757574525,-1.63170950078457));
#31205=CARTESIAN_POINT('Ctrl Pts',(-30.767121516155,56.5849189585236,-1.59466353726188));
#31206=CARTESIAN_POINT('Ctrl Pts',(-31.0251241525943,57.0723230889947,-1.5576175737392));
#31207=CARTESIAN_POINT('Ctrl Pts',(-31.2831267890337,57.5597272194657,-1.52057161021652));
#31208=CARTESIAN_POINT('Ctrl Pts',(-31.8065736312309,57.9065922793366,-1.48352564669384));
#31209=CARTESIAN_POINT('Ctrl Pts',(-32.3559737285805,57.9541834292484,-1.44647968317116));
#31210=CARTESIAN_POINT('Ctrl Pts',(-32.6919280642789,57.9832850861845,-1.42382633431737));
#31211=CARTESIAN_POINT('Ctrl Pts',(-33.0375869381561,57.9004811240364,-1.40117298546358));
#31212=CARTESIAN_POINT('Ctrl Pts',(-33.3327354544031,57.732107437543,-1.37851963660978));
#31213=CARTESIAN_POINT('Origin',(-32.5,56.2916512459885,-3.54592528053767));
#31214=CARTESIAN_POINT('',(-33.5296449158133,58.0726582505548,6.54592528053768));
#31215=CARTESIAN_POINT('',(-33.5251060574855,58.0687922621904,6.60407471946233));
#31216=CARTESIAN_POINT('',(-33.5273750000001,58.0711169444145,-3.54592528053767));
#31217=CARTESIAN_POINT('',(-30.845746263986,55.0728640868079,7.));
#31218=CARTESIAN_POINT('Ctrl Pts',(-33.5251060574855,58.0687922621904,6.60407471946233));
#31219=CARTESIAN_POINT('Ctrl Pts',(-33.8584527741405,57.8749712083971,6.62491192240684));
#31220=CARTESIAN_POINT('Ctrl Pts',(-34.6426244289716,57.0875348868181,6.68279508887404));
#31221=CARTESIAN_POINT('Ctrl Pts',(-34.6192626691618,55.1024844807855,6.77772421886391));
#31222=CARTESIAN_POINT('Ctrl Pts',(-32.6468806392671,53.8684656063832,6.88886210943196));
#31223=CARTESIAN_POINT('Ctrl Pts',(-31.2510219905719,54.522785363242,6.96295403647732));
#31224=CARTESIAN_POINT('Ctrl Pts',(-30.845746263986,55.0728640868079,7.));
#31225=CARTESIAN_POINT('',(-30.4546316093048,56.0596663160167,7.));
#31226=CARTESIAN_POINT('Origin',(-32.5,56.2916512459885,7.));
#31227=CARTESIAN_POINT('Ctrl Pts',(-33.5296449158133,58.0726582505548,6.54592528053768));
#31228=CARTESIAN_POINT('Ctrl Pts',(-33.5919384699578,58.0372735301249,6.54982271160486));
#31229=CARTESIAN_POINT('Ctrl Pts',(-34.225323347054,57.6301444802746,6.59076610619471));
#31230=CARTESIAN_POINT('Ctrl Pts',(-34.9251107981772,56.1574151102239,6.66875546430726));
#31231=CARTESIAN_POINT('Ctrl Pts',(-33.7019669024841,54.1813822458926,6.77989335487529));
#31232=CARTESIAN_POINT('Ctrl Pts',(-31.3950249125263,54.1375954583441,6.89030820010622));
#31233=CARTESIAN_POINT('Ctrl Pts',(-30.5306488143205,55.3970288255657,6.96367708181445));
#31234=CARTESIAN_POINT('Ctrl Pts',(-30.4546294175093,56.0596661744468,7.));
#31235=CARTESIAN_POINT('Origin',(-32.5,56.2916512459885,-3.54592528053767));
#31236=CARTESIAN_POINT('',(-33.5268493235952,58.0681533924579,5.84592528053768));
#31237=CARTESIAN_POINT('',(-33.5270361074232,58.0735254724117,5.90407471946233));
#31238=CARTESIAN_POINT('',(-33.5273750000001,58.0711169444145,-3.54592528053767));
#31239=CARTESIAN_POINT('Ctrl Pts',(-33.5270361074232,58.0735254724117,5.90407471946232));
#31240=CARTESIAN_POINT('Ctrl Pts',(-34.0327197348533,57.7760135322548,5.93596947460409));
#31241=CARTESIAN_POINT('Ctrl Pts',(-34.8527930569705,56.6438137488048,6.00491019326854));
#31242=CARTESIAN_POINT('Ctrl Pts',(-34.1759192345577,54.5338890939528,6.11089687545567));
#31243=CARTESIAN_POINT('Ctrl Pts',(-31.9320786480218,53.9303413264953,6.2220347660237));
#31244=CARTESIAN_POINT('Ctrl Pts',(-30.2082245117245,55.4880781765344,6.33317265659175));
#31245=CARTESIAN_POINT('Ctrl Pts',(-30.5817368018815,57.7814323658043,6.44431054715979));
#31246=CARTESIAN_POINT('Ctrl Pts',(-32.3123519600732,58.5366981066488,6.53461123478332));
#31247=CARTESIAN_POINT('Ctrl Pts',(-33.265803638914,58.2195610128864,6.58786595888416));
#31248=CARTESIAN_POINT('Ctrl Pts',(-33.5251060574855,58.0687922621904,6.60407471946233));
#31249=CARTESIAN_POINT('Ctrl Pts',(-33.5268493235952,58.0681533924579,5.84592528053768));
#31250=CARTESIAN_POINT('Ctrl Pts',(-33.7671186009377,57.9308791195189,5.86088026380211));
#31251=CARTESIAN_POINT('Ctrl Pts',(-34.5085314004615,57.2938049828723,5.91288121058922));
#31252=CARTESIAN_POINT('Ctrl Pts',(-34.7788326566387,55.451849617872,6.00192812089901));
#31253=CARTESIAN_POINT('Ctrl Pts',(-33.0303393193103,53.921614042038,6.11306601146705));
#31254=CARTESIAN_POINT('Ctrl Pts',(-30.79644075645,54.5607069079647,6.22420390203509));
#31255=CARTESIAN_POINT('Ctrl Pts',(-30.1217887402557,56.7841397946825,6.33534179260313));
#31256=CARTESIAN_POINT('Ctrl Pts',(-31.5713402558441,58.4946530906761,6.442582252104));
#31257=CARTESIAN_POINT('Ctrl Pts',(-32.999824152922,58.3736132984777,6.51277674808218));
#31258=CARTESIAN_POINT('Ctrl Pts',(-33.5296449158133,58.0726582505548,6.54592528053768));
#31259=CARTESIAN_POINT('Origin',(-32.5,56.2916512459885,-3.54592528053767));
#31260=CARTESIAN_POINT('',(-33.525217808475,58.0709111221528,5.14592528053768));
#31261=CARTESIAN_POINT('',(-33.5295558866825,58.0716265502945,5.20407471946232));
#31262=CARTESIAN_POINT('',(-33.5273750000001,58.0711169444145,-3.54592528053767));
#31263=CARTESIAN_POINT('Ctrl Pts',(-33.5295558866825,58.0716265502945,5.20407471946232));
#31264=CARTESIAN_POINT('Ctrl Pts',(-33.6241634690101,58.0180957001452,5.20998106327865));
#31265=CARTESIAN_POINT('Ctrl Pts',(-34.2792376101367,57.5737577801449,5.25293337061767));
#31266=CARTESIAN_POINT('Ctrl Pts',(-34.9141240107244,56.0264398256936,5.33293164147938));
#31267=CARTESIAN_POINT('Ctrl Pts',(-33.5864678368826,54.1195735160326,5.44406953204741));
#31268=CARTESIAN_POINT('Ctrl Pts',(-31.2643540254432,54.2008349824401,5.55520742261546));
#31269=CARTESIAN_POINT('Ctrl Pts',(-30.0732435855652,56.1958434964943,5.66634531318349));
#31270=CARTESIAN_POINT('Ctrl Pts',(-31.10336564197,58.2785475024108,5.77748320375154));
#31271=CARTESIAN_POINT('Ctrl Pts',(-32.7493551050699,58.4668353041202,5.85672633917781));
#31272=CARTESIAN_POINT('Ctrl Pts',(-33.4453649446213,58.1215755669412,5.89892351108141));
#31273=CARTESIAN_POINT('Ctrl Pts',(-33.5270361074232,58.0735254724117,5.90407471946232));
#31274=CARTESIAN_POINT('Ctrl Pts',(-33.525217808475,58.0709111221528,5.14592528053768));
#31275=CARTESIAN_POINT('Ctrl Pts',(-33.9392806903329,57.8273071486293,5.17193781599936));
#31276=CARTESIAN_POINT('Ctrl Pts',(-34.7491747415829,56.8889612418332,5.23499631498372));
#31277=CARTESIAN_POINT('Ctrl Pts',(-34.4321757978777,54.8202470274371,5.33510077749076));
#31278=CARTESIAN_POINT('Ctrl Pts',(-32.3116949177892,53.8703138209288,5.44623866805879));
#31279=CARTESIAN_POINT('Ctrl Pts',(-30.3635721421369,55.1366583239951,5.55737655862684));
#31280=CARTESIAN_POINT('Ctrl Pts',(-30.3709453622051,57.4601807388668,5.66851444919488));
#31281=CARTESIAN_POINT('Ctrl Pts',(-32.0638471781548,58.5454001176689,5.76469735649849));
#31282=CARTESIAN_POINT('Ctrl Pts',(-33.1719319178991,58.2709301659147,5.82383430027943));
#31283=CARTESIAN_POINT('Ctrl Pts',(-33.5268493235952,58.0681533924579,5.84592528053768));
#31284=CARTESIAN_POINT('Origin',(-32.5,56.2916512459885,-3.54592528053767));
#31285=CARTESIAN_POINT('',(-33.5290839475038,58.0740603739206,4.44592528053768));
#31286=CARTESIAN_POINT('',(-33.5261619125926,58.0680778657968,4.50407471946232));
#31287=CARTESIAN_POINT('',(-33.5273750000001,58.0711169444145,-3.54592528053767));
#31288=CARTESIAN_POINT('Ctrl Pts',(-33.5261619125926,58.0680778657968,4.50407471946232));
#31289=CARTESIAN_POINT('Ctrl Pts',(-33.7984529813903,57.9116108116526,4.5210386154759));
#31290=CARTESIAN_POINT('Ctrl Pts',(-34.5559374767779,57.225562580793,4.57504847501217));
#31291=CARTESIAN_POINT('Ctrl Pts',(-34.7300884128152,55.3298620761609,4.66610429807112));
#31292=CARTESIAN_POINT('Ctrl Pts',(-32.9014225703573,53.8964074829672,4.77724218863916));
#31293=CARTESIAN_POINT('Ctrl Pts',(-30.7053300758283,54.6553466763578,4.88838007920721));
#31294=CARTESIAN_POINT('Ctrl Pts',(-30.1519193575992,56.9120139865896,4.99951796977524));
#31295=CARTESIAN_POINT('Ctrl Pts',(-31.6629249999102,58.5111039532885,5.10474951652696));
#31296=CARTESIAN_POINT('Ctrl Pts',(-33.0307626862479,58.3538536552586,5.17293509975597));
#31297=CARTESIAN_POINT('Ctrl Pts',(-33.5295558866825,58.0716265502945,5.20407471946232));
#31298=CARTESIAN_POINT('Ctrl Pts',(-33.5290839390052,58.0740603592829,4.44592528053768));
#31299=CARTESIAN_POINT('Ctrl Pts',(-33.5294675225899,58.0738389277433,4.44594940467393));
#31300=CARTESIAN_POINT('Ctrl Pts',(-34.118776307512,57.7333695942669,4.48301949233285));
#31301=CARTESIAN_POINT('Ctrl Pts',(-34.9257362810773,56.410550559801,4.55713554351447));
#31302=CARTESIAN_POINT('Ctrl Pts',(-33.91547832718,54.3181379674856,4.6682734340825));
#31303=CARTESIAN_POINT('Ctrl Pts',(-31.6096170051591,54.0321044593028,4.77941132465055));
#31304=CARTESIAN_POINT('Ctrl Pts',(-30.1187333412011,55.8142597516568,4.89054921521859));
#31305=CARTESIAN_POINT('Ctrl Pts',(-30.8074500449804,58.033376889416,5.00168710578664));
#31306=CARTESIAN_POINT('Ctrl Pts',(-32.5215758081835,58.5120119076972,5.08681246089299));
#31307=CARTESIAN_POINT('Ctrl Pts',(-33.3495896761677,58.1742377248673,5.13489185247668));
#31308=CARTESIAN_POINT('Ctrl Pts',(-33.525217808475,58.0709111221528,5.14592528053768));
#31309=CARTESIAN_POINT('Origin',(-32.5,56.2916512459885,-3.54592528053767));
#31310=CARTESIAN_POINT('',(-33.5282587680712,58.0691275396584,3.74592528053768));
#31311=CARTESIAN_POINT('',(-33.5256537705603,58.0718935083249,3.80407471946232));
#31312=CARTESIAN_POINT('',(-33.5273750000001,58.0711169444145,-3.54592528053767));
#31313=CARTESIAN_POINT('Ctrl Pts',(-33.5256537705603,58.0718935083249,3.80407471946232));
#31314=CARTESIAN_POINT('Ctrl Pts',(-33.9708692323456,57.8094153705276,3.83209616767316));
#31315=CARTESIAN_POINT('Ctrl Pts',(-34.7867776966583,56.8075863052296,3.89716357940667));
#31316=CARTESIAN_POINT('Ctrl Pts',(-34.3497911057075,54.7179277581866,3.99927695466287));
#31317=CARTESIAN_POINT('Ctrl Pts',(-32.1810499960691,53.8840375630848,4.11041484523091));
#31318=CARTESIAN_POINT('Ctrl Pts',(-30.3042474418304,55.2538634762437,4.22155273579896));
#31319=CARTESIAN_POINT('Ctrl Pts',(-30.4372421062834,57.5735883041595,4.332690626367));
#31320=CARTESIAN_POINT('Ctrl Pts',(-32.1498112942942,58.5449642134685,4.42686462092145));
#31321=CARTESIAN_POINT('Ctrl Pts',(-33.2038204161972,58.2533054775292,4.48399265195323));
#31322=CARTESIAN_POINT('Ctrl Pts',(-33.5261619125926,58.0680778657968,4.50407471946232));
#31323=CARTESIAN_POINT('Ctrl Pts',(-33.5282587680712,58.0691275396584,3.74592528053768));
#31324=CARTESIAN_POINT('Ctrl Pts',(-33.7063336904378,57.9682446528084,3.75700695687118));
#31325=CARTESIAN_POINT('Ctrl Pts',(-34.4133163086311,57.41900891881,3.80513459672736));
#31326=CARTESIAN_POINT('Ctrl Pts',(-34.8538786959893,55.6936640901667,3.89030820010621));
#31327=CARTESIAN_POINT('Ctrl Pts',(-33.2742100800909,53.9897102593704,4.00144609067426));
#31328=CARTESIAN_POINT('Ctrl Pts',(-30.9858981977034,54.3927491193984,4.1125839812423));
#31329=CARTESIAN_POINT('Ctrl Pts',(-30.0834608661247,56.5338746309361,4.22372187181034));
#31330=CARTESIAN_POINT('Ctrl Pts',(-31.3926249737446,58.4528736933808,4.33483563824213));
#31331=CARTESIAN_POINT('Ctrl Pts',(-32.9404216250933,58.4138778272017,4.40890344115124));
#31332=CARTESIAN_POINT('Ctrl Pts',(-33.5290839390052,58.0740603592829,4.44592528053768));
#31333=CARTESIAN_POINT('Origin',(-32.5,56.2916512459885,-3.54592528053767));
#31334=CARTESIAN_POINT('',(-33.5250673440976,58.0691981786101,3.04592528053768));
#31335=CARTESIAN_POINT('',(-33.5295277964002,58.073488152934,3.10407471946232));
#31336=CARTESIAN_POINT('',(-33.5273750000001,58.0711169444145,-3.54592528053767));
#31337=CARTESIAN_POINT('Ctrl Pts',(-33.5295277964002,58.073488152934,3.10407471946232));
#31338=CARTESIAN_POINT('Ctrl Pts',(-33.5619446593131,58.0549578524536,3.10610775634773));
#31339=CARTESIAN_POINT('Ctrl Pts',(-34.1744592271169,57.680719250686,3.14518675675581));
#31340=CARTESIAN_POINT('Ctrl Pts',(-34.9286165141379,56.2792182940979,3.22131172068658));
#31341=CARTESIAN_POINT('Ctrl Pts',(-33.8067007722453,54.2444908119128,3.33244961125462));
#31342=CARTESIAN_POINT('Ctrl Pts',(-31.4887469945246,54.0835524914147,3.44358750182266));
#31343=CARTESIAN_POINT('Ctrl Pts',(-30.0964045610992,55.9437120025227,3.5547253923907));
#31344=CARTESIAN_POINT('Ctrl Pts',(-30.9041002915367,58.1223442490711,3.66586328295875));
#31345=CARTESIAN_POINT('Ctrl Pts',(-32.6005939960278,58.4985054002163,3.74897972531595));
#31346=CARTESIAN_POINT('Ctrl Pts',(-33.3822688276508,58.1564265401566,3.79505020415048));
#31347=CARTESIAN_POINT('Ctrl Pts',(-33.5256537705603,58.0718935083249,3.80407471946232));
#31348=CARTESIAN_POINT('Ctrl Pts',(-33.5250673440976,58.0691981786101,3.04592528053768));
#31349=CARTESIAN_POINT('Ctrl Pts',(-33.8788897107517,57.8627525499152,3.06806450906843));
#31350=CARTESIAN_POINT('Ctrl Pts',(-34.6708999553705,57.0389934359535,3.12724970112185));
#31351=CARTESIAN_POINT('Ctrl Pts',(-34.5748652707907,55.0294041774427,3.22348085669796));
#31352=CARTESIAN_POINT('Ctrl Pts',(-32.5648065727292,53.8638675525518,3.334618747266));
#31353=CARTESIAN_POINT('Ctrl Pts',(-30.4954296836916,54.9205088752031,3.44575663783405));
#31354=CARTESIAN_POINT('Ctrl Pts',(-30.2608587385459,57.2321723596468,3.55689452840209));
#31355=CARTESIAN_POINT('Ctrl Pts',(-31.8948295568209,58.5383060176734,3.65695074263663));
#31356=CARTESIAN_POINT('Ctrl Pts',(-33.1110305179062,58.3054954110723,3.71996099334849));
#31357=CARTESIAN_POINT('Ctrl Pts',(-33.5282587680712,58.0691275396584,3.74592528053768));
#31358=CARTESIAN_POINT('Origin',(-32.5,56.2916512459885,-3.54592528053767));
#31359=CARTESIAN_POINT('',(-33.5275894562265,58.0738927599536,2.34592528053768));
#31360=CARTESIAN_POINT('',(-33.5275355691898,58.0684930935818,2.40407471946232));
#31361=CARTESIAN_POINT('',(-33.5273750000001,58.0711169444145,-3.54592528053767));
#31362=CARTESIAN_POINT('Ctrl Pts',(-33.5275355691898,58.0684930935818,2.40407471946232));
#31363=CARTESIAN_POINT('Ctrl Pts',(-33.7379292069399,57.9488445224074,2.41716530854498));
#31364=CARTESIAN_POINT('Ctrl Pts',(-34.4632973547596,57.3551041347746,2.46730186115031));
#31365=CARTESIAN_POINT('Ctrl Pts',(-34.8181023612983,55.5672658557593,2.55448437727833));
#31366=CARTESIAN_POINT('Ctrl Pts',(-33.1486127133916,53.9512166070675,2.66562226784637));
#31367=CARTESIAN_POINT('Ctrl Pts',(-30.8854404931491,54.4773937257141,2.77676015841441));
#31368=CARTESIAN_POINT('Ctrl Pts',(-30.1000928998773,56.6641813277477,2.88789804898245));
#31369=CARTESIAN_POINT('Ctrl Pts',(-31.4855904228425,58.4762227231016,2.99700290266509));
#31370=CARTESIAN_POINT('Ctrl Pts',(-32.9712451350632,58.3926166724123,3.06906179282505));
#31371=CARTESIAN_POINT('Ctrl Pts',(-33.5295277964002,58.073488152934,3.10407471946232));
#31372=CARTESIAN_POINT('Ctrl Pts',(-33.5275894562265,58.0738927599536,2.34592528053768));
#31373=CARTESIAN_POINT('Ctrl Pts',(-34.0539010838894,57.7651290399621,2.37912206126568));
#31374=CARTESIAN_POINT('Ctrl Pts',(-34.8729207037989,56.5867324218955,2.44936480551635));
#31375=CARTESIAN_POINT('Ctrl Pts',(-34.113250907707,54.4762297900261,2.55665351328971));
#31376=CARTESIAN_POINT('Ctrl Pts',(-31.8496996873681,53.9516847809774,2.66779140385775));
#31377=CARTESIAN_POINT('Ctrl Pts',(-30.1813757180884,55.5689376143778,2.7789292944258));
#31378=CARTESIAN_POINT('Ctrl Pts',(-30.6353148490301,57.8476984309217,2.89006718499383));
#31379=CARTESIAN_POINT('Ctrl Pts',(-32.3655977900595,58.5319722593687,2.97906584703113));
#31380=CARTESIAN_POINT('Ctrl Pts',(-33.2868324730584,58.2082016796998,3.03101854554575));
#31381=CARTESIAN_POINT('Ctrl Pts',(-33.5250673440976,58.0691981786101,3.04592528053768));
#31382=CARTESIAN_POINT('Origin',(-32.5,56.2916512459885,-3.54592528053767));
#31383=CARTESIAN_POINT('',(-33.5293464154416,58.0709332657958,1.64592528053768));
#31384=CARTESIAN_POINT('',(-33.5250295315601,58.0700303972121,1.70407471946232));
#31385=CARTESIAN_POINT('',(-33.5273750000001,58.0711169444145,-3.54592528053767));
#31386=CARTESIAN_POINT('Ctrl Pts',(-33.5250295315601,58.0700303972121,1.70407471946232));
#31387=CARTESIAN_POINT('Ctrl Pts',(-33.9101525759349,57.8442238653441,1.72822286074222));
#31388=CARTESIAN_POINT('Ctrl Pts',(-34.7124027752876,56.9623029261605,1.78941696554481));
#31389=CARTESIAN_POINT('Ctrl Pts',(-34.5035809067649,54.9190637984713,1.88765703387008));
#31390=CARTESIAN_POINT('Ctrl Pts',(-32.4334427362781,53.863915082053,1.99879492443812));
#31391=CARTESIAN_POINT('Ctrl Pts',(-30.4242251840869,55.0309008088856,2.10993281500616));
#31392=CARTESIAN_POINT('Ctrl Pts',(-30.3149878617883,57.3518657086808,2.22107070557421));
#31393=CARTESIAN_POINT('Ctrl Pts',(-31.9830137885335,58.5433285166527,2.31911800705959));
#31394=CARTESIAN_POINT('Ctrl Pts',(-33.1425216985167,58.2874462900804,2.3801193450223));
#31395=CARTESIAN_POINT('Ctrl Pts',(-33.5275355691898,58.0684930935818,2.40407471946232));
#31396=CARTESIAN_POINT('Ctrl Pts',(-33.5293464154416,58.0709332657958,1.64592528053768));
#31397=CARTESIAN_POINT('Ctrl Pts',(-33.6449437000377,58.0055982631749,1.65313364994024));
#31398=CARTESIAN_POINT('Ctrl Pts',(-34.3136427308233,57.5361314802505,1.69738798286549));
#31399=CARTESIAN_POINT('Ctrl Pts',(-34.90334407317,55.9419787993381,1.77868827931342));
#31400=CARTESIAN_POINT('Ctrl Pts',(-33.5096605171051,54.0828236849994,1.88982616988146));
#31401=CARTESIAN_POINT('Ctrl Pts',(-31.1918232394055,54.2454334870425,2.0009640604495));
#31402=CARTESIAN_POINT('Ctrl Pts',(-30.0713749864112,56.2809696095364,2.11210195101755));
#31403=CARTESIAN_POINT('Ctrl Pts',(-31.1738747508359,58.326282755013,2.22323984158559));
#31404=CARTESIAN_POINT('Ctrl Pts',(-32.7983102681658,58.4546151165851,2.30118095142563));
#31405=CARTESIAN_POINT('Ctrl Pts',(-33.4665633682319,58.1096940627471,2.342076097743));
#31406=CARTESIAN_POINT('Ctrl Pts',(-33.5275894562265,58.0738927599536,2.34592528053768));
#31407=CARTESIAN_POINT('Origin',(-32.5,56.2916512459885,-3.54592528053767));
#31408=CARTESIAN_POINT('',(-33.5257755155985,58.0681903527959,0.945925280537675));
#31409=CARTESIAN_POINT('',(-33.5284289248676,58.0741771517811,1.00407471946232));
#31410=CARTESIAN_POINT('',(-33.5273750000001,58.0711169444145,-3.54592528053767));
#31411=CARTESIAN_POINT('Ctrl Pts',(-33.5284289248676,58.0741771517811,1.00407471946232));
#31412=CARTESIAN_POINT('Ctrl Pts',(-34.0870797198612,57.7486846686039,1.03928041293948));
#31413=CARTESIAN_POINT('Ctrl Pts',(-34.9017444968086,56.4966890376489,1.11153206993931));
#31414=CARTESIAN_POINT('Ctrl Pts',(-34.0127319779434,54.3916579002222,1.22082969046183));
#31415=CARTESIAN_POINT('Ctrl Pts',(-31.7241302087768,53.9902693093903,1.33196758102987));
#31416=CARTESIAN_POINT('Ctrl Pts',(-30.1456908584837,55.6953617045703,1.44310547159791));
#31417=CARTESIAN_POINT('Ctrl Pts',(-30.7221773650996,57.9462446793952,1.55424336216595));
#31418=CARTESIAN_POINT('Ctrl Pts',(-32.4470927941984,58.5226506382554,1.64123311145409));
#31419=CARTESIAN_POINT('Ctrl Pts',(-33.3193305292905,58.1906364710101,1.69117689721954));
#31420=CARTESIAN_POINT('Ctrl Pts',(-33.5250295315601,58.0700303972121,1.70407471946232));
#31421=CARTESIAN_POINT('Ctrl Pts',(-33.5257755155985,58.0681903527959,0.945925280537676));
#31422=CARTESIAN_POINT('Ctrl Pts',(-33.8187120383006,57.8991957700279,0.964191202137494));
#31423=CARTESIAN_POINT('Ctrl Pts',(-34.5858726429697,57.180098149748,1.01950308725999));
#31424=CARTESIAN_POINT('Ctrl Pts',(-34.6950037716947,55.2522802841409,1.11186093590517));
#31425=CARTESIAN_POINT('Ctrl Pts',(-32.8172137752098,53.883808025427,1.22299882647321));
#31426=CARTESIAN_POINT('Ctrl Pts',(-30.6490744128705,54.7192619732989,1.33413671704125));
#31427=CARTESIAN_POINT('Ctrl Pts',(-30.1751082313325,56.9939416545675,1.44527460760929));
#31428=CARTESIAN_POINT('Ctrl Pts',(-31.7218617398002,58.5199646784861,1.54920412877477));
#31429=CARTESIAN_POINT('Ctrl Pts',(-33.0508547252211,58.3413743574169,1.61608768641756));
#31430=CARTESIAN_POINT('Ctrl Pts',(-33.5293464154416,58.0709332657958,1.64592528053768));
#31431=CARTESIAN_POINT('Origin',(-32.5,56.2916512459885,-3.54592528053767));
#31432=CARTESIAN_POINT('',(-33.5260517589603,58.0725043954729,0.245925280537674));
#31433=CARTESIAN_POINT('',(-33.5288532114794,58.0699232317666,0.304074719462319));
#31434=CARTESIAN_POINT('',(-33.5273750000001,58.0711169444145,-3.54592528053767));
#31435=CARTESIAN_POINT('Ctrl Pts',(-33.5288532114794,58.0699232317666,0.304074719462319));
#31436=CARTESIAN_POINT('Ctrl Pts',(-33.6768637713204,57.9862464992859,0.313292001614044));
#31437=CARTESIAN_POINT('Ctrl Pts',(-34.3658577642721,57.4763696079473,0.359555247288449));
#31438=CARTESIAN_POINT('Ctrl Pts',(-34.8809216257836,55.8125427394079,0.442864456485535));
#31439=CARTESIAN_POINT('Ctrl Pts',(-33.3887533074142,54.0314631320695,0.554002347053576));
#31440=CARTESIAN_POINT('Ctrl Pts',(-31.0830990069914,54.3191593379889,0.665140237621618));
#31441=CARTESIAN_POINT('Ctrl Pts',(-30.0743502545356,56.4122997567237,0.77627812818966));
#31442=CARTESIAN_POINT('Ctrl Pts',(-31.2858262226837,58.3950092254139,0.887416018757703));
#31443=CARTESIAN_POINT('Ctrl Pts',(-32.8728372110939,58.4342824094917,0.963348215848589));
#31444=CARTESIAN_POINT('Ctrl Pts',(-33.4992271616754,58.0911912767045,1.00223444941679));
#31445=CARTESIAN_POINT('Ctrl Pts',(-33.5284289248676,58.0741771517811,1.00407471946232));
#31446=CARTESIAN_POINT('Ctrl Pts',(-33.5260517589603,58.0725043954729,0.245925280537675));
#31447=CARTESIAN_POINT('Ctrl Pts',(-33.991498229918,57.7980207394882,0.275248754334742));
#31448=CARTESIAN_POINT('Ctrl Pts',(-34.8099603858883,56.7535423775609,0.34161819165449));
#31449=CARTESIAN_POINT('Ctrl Pts',(-34.2934896049409,54.6540528227808,0.445033592496919));
#31450=CARTESIAN_POINT('Ctrl Pts',(-32.0968502643471,53.8966974164155,0.55617148306496));
#31451=CARTESIAN_POINT('Ctrl Pts',(-30.2692184515671,55.3314704112852,0.667309373633001));
#31452=CARTESIAN_POINT('Ctrl Pts',(-30.4834462874739,57.6451078131478,0.778447264201044));
#31453=CARTESIAN_POINT('Ctrl Pts',(-32.2048796389798,58.5432631965409,0.871319233169268));
#31454=CARTESIAN_POINT('Ctrl Pts',(-33.224593878142,58.2419415282719,0.927145238614813));
#31455=CARTESIAN_POINT('Ctrl Pts',(-33.5257755155985,58.0681903527959,0.945925280537676));
#31456=CARTESIAN_POINT('Origin',(-32.5,56.2916512459885,-3.54592528053767));
#31457=CARTESIAN_POINT('',(-33.5296554006197,58.0729354591291,-0.454074719462322));
#31458=CARTESIAN_POINT('',(-33.5253135061185,58.0685974415039,-0.395925280537681));
#31459=CARTESIAN_POINT('',(-33.5273750000001,58.0711169444145,-3.54592528053767));
#31460=CARTESIAN_POINT('Ctrl Pts',(-33.5253135061185,58.0685974415039,-0.395925280537681));
#31461=CARTESIAN_POINT('Ctrl Pts',(-33.8499262418575,57.8801900402997,-0.375650446188706));
#31462=CARTESIAN_POINT('Ctrl Pts',(-34.6307561402676,57.1080161029863,-0.318329648317051));
#31463=CARTESIAN_POINT('Ctrl Pts',(-34.6355944339958,55.1351180442908,-0.223962886922716));
#31464=CARTESIAN_POINT('Ctrl Pts',(-32.6865588761979,53.8701788494842,-0.112824996354674));
#31465=CARTESIAN_POINT('Ctrl Pts',(-30.5667638241697,54.8216408199214,-0.00168710578663194));
#31466=CARTESIAN_POINT('Ctrl Pts',(-30.2164817879238,57.1186199946645,0.109450784781409));
#31467=CARTESIAN_POINT('Ctrl Pts',(-31.8120346004306,58.5309407947375,0.211371393197727));
#31468=CARTESIAN_POINT('Ctrl Pts',(-33.081981927564,58.322558779647,0.276246038091363));
#31469=CARTESIAN_POINT('Ctrl Pts',(-33.5288532114794,58.0699232317666,0.304074719462319));
#31470=CARTESIAN_POINT('Ctrl Pts',(-33.5296554006197,58.0729354591291,-0.454074719462324));
#31471=CARTESIAN_POINT('Ctrl Pts',(-33.5829230895642,58.0426280169118,-0.450739656990688));
#31472=CARTESIAN_POINT('Ctrl Pts',(-34.2100716718942,57.6455781417159,-0.410358630996371));
#31473=CARTESIAN_POINT('Ctrl Pts',(-34.926688116847,56.1940939537868,-0.332931641479374));
#31474=CARTESIAN_POINT('Ctrl Pts',(-33.7341373860101,54.1999441339785,-0.221793750911332));
#31475=CARTESIAN_POINT('Ctrl Pts',(-31.4119663698709,54.1203575053851,-0.110655860343291));
#31476=CARTESIAN_POINT('Ctrl Pts',(-30.0856850452223,56.0281806868171,0.000482030224751779));
#31477=CARTESIAN_POINT('Ctrl Pts',(-30.9692534931352,58.1771614464074,0.111619920792793));
#31478=CARTESIAN_POINT('Ctrl Pts',(-32.6511246141561,58.4886656996171,0.193434337563768));
#31479=CARTESIAN_POINT('Ctrl Pts',(-33.4034740038598,58.1447910975144,0.238202790812062));
#31480=CARTESIAN_POINT('Ctrl Pts',(-33.5260517589603,58.0725043954729,0.245925280537675));
#31481=CARTESIAN_POINT('Origin',(-32.5,56.2916512459885,-3.54592528053767));
#31482=CARTESIAN_POINT('',(-33.5270487244507,58.0682282925651,-1.15407471946232));
#31483=CARTESIAN_POINT('',(-33.5268019957928,58.0733321975144,-1.09592528053768));
#31484=CARTESIAN_POINT('',(-33.5273750000001,58.0711169444145,-3.54592528053767));
#31485=CARTESIAN_POINT('Ctrl Pts',(-33.5268019957928,58.0733321975144,-1.09592528053768));
#31486=CARTESIAN_POINT('Ctrl Pts',(-34.0236398642182,57.7807696971903,-1.06459289399146));
#31487=CARTESIAN_POINT('Ctrl Pts',(-34.8437811491657,56.6681489116154,-0.996214543922552));
#31488=CARTESIAN_POINT('Ctrl Pts',(-34.2023204507042,54.559476051911,-0.890790230330966));
#31489=CARTESIAN_POINT('Ctrl Pts',(-31.9679467730355,53.921998742765,-0.779652339762925));
#31490=CARTESIAN_POINT('Ctrl Pts',(-30.2205650142274,55.453492447677,-0.668514449194883));
#31491=CARTESIAN_POINT('Ctrl Pts',(-30.5595771710743,57.752161801101,-0.557376558626841));
#31492=CARTESIAN_POINT('Ctrl Pts',(-32.2888225453055,58.5385401346074,-0.466513502407774));
#31493=CARTESIAN_POINT('Ctrl Pts',(-33.2567972741826,58.2244460570088,-0.412696409711387));
#31494=CARTESIAN_POINT('Ctrl Pts',(-33.5253135061185,58.0685974415039,-0.395925280537681));
#31495=CARTESIAN_POINT('Ctrl Pts',(-33.5270487244507,58.0682282925651,-1.15407471946232));
#31496=CARTESIAN_POINT('Ctrl Pts',(-33.7583254242685,57.9362916288017,-1.13968210479344));
#31497=CARTESIAN_POINT('Ctrl Pts',(-34.4950254817816,57.3125020026611,-1.08824352660187));
#31498=CARTESIAN_POINT('Ctrl Pts',(-34.7912737376158,55.4864512354733,-0.999758984887624));
#31499=CARTESIAN_POINT('Ctrl Pts',(-33.0661792001092,53.929919412126,-0.888621094319583));
#31500=CARTESIAN_POINT('Ctrl Pts',(-30.822833264184,54.5351044086333,-0.77748320375154));
#31501=CARTESIAN_POINT('Ctrl Pts',(-30.114627688562,56.7480782089187,-0.666345313183499));
#31502=CARTESIAN_POINT('Ctrl Pts',(-31.5455083936009,58.4894074878942,-0.558542485087094));
#31503=CARTESIAN_POINT('Ctrl Pts',(-32.9912241698708,58.3792838991923,-0.487785620513369));
#31504=CARTESIAN_POINT('Ctrl Pts',(-33.5296554006197,58.0729354591291,-0.454074719462324));
#31505=CARTESIAN_POINT('Origin',(-32.5,56.2916512459885,-3.54592528053767));
#31506=CARTESIAN_POINT('',(-33.5243188290626,58.0704843676251,-1.85407471946232));
#31507=CARTESIAN_POINT('',(-33.5295805874755,58.0719425970214,-1.79592528053768));
#31508=CARTESIAN_POINT('',(-33.5273750000001,58.0711169444145,-3.54592528053767));
#31509=CARTESIAN_POINT('',(-31.045873711622,57.7433792852396,-2.));
#31510=CARTESIAN_POINT('Ctrl Pts',(-31.045873711622,57.7433792852396,-2.));
#31511=CARTESIAN_POINT('Ctrl Pts',(-31.5286078227265,58.2269108712356,-1.96295403647732));
#31512=CARTESIAN_POINT('Ctrl Pts',(-32.4987857659729,58.5150960016802,-1.91431227629809));
#31513=CARTESIAN_POINT('Ctrl Pts',(-33.339589876325,58.1790057138553,-1.86567051611887));
#31514=CARTESIAN_POINT('Ctrl Pts',(-33.5243188290626,58.0704843676251,-1.85407471946232));
#31515=CARTESIAN_POINT('',(-30.5120522999331,56.8258916115681,-2.));
#31516=CARTESIAN_POINT('Origin',(-32.5,56.2916512459885,-2.));
#31517=CARTESIAN_POINT('Ctrl Pts',(-30.5120501580915,56.825892077386,-2.));
#31518=CARTESIAN_POINT('Ctrl Pts',(-30.6859814099171,57.4697983977034,-1.96367708181445));
#31519=CARTESIAN_POINT('Ctrl Pts',(-31.6524845810095,58.5050100533592,-1.89565217532701));
#31520=CARTESIAN_POINT('Ctrl Pts',(-33.0221861661125,58.3592796390666,-1.82762726883957));
#31521=CARTESIAN_POINT('Ctrl Pts',(-33.5295805874755,58.0719425970214,-1.79592528053768));
#31522=CARTESIAN_POINT('Origin',(-65.,8.88178419700125E-15,3.));
#31523=CARTESIAN_POINT('',(-66.6675465985015,0.00121430446292491,6.12851963660979));
#31524=CARTESIAN_POINT('',(-66.6679935094968,-0.00096847687650235,6.32148036339021));
#31525=CARTESIAN_POINT('',(-66.666,8.90896198514149E-15,3.));
#31526=CARTESIAN_POINT('',(-66.6351293272515,0.319230454628283,7.));
#31527=CARTESIAN_POINT('Ctrl Pts',(-66.6679935094968,-0.00096847687650235,
6.32148036339021));
#31528=CARTESIAN_POINT('Ctrl Pts',(-66.6684011451999,-0.0590543694261873,
6.32537779445739));
#31529=CARTESIAN_POINT('Ctrl Pts',(-66.6656310767024,-0.117101359876398,
6.32927522552457));
#31530=CARTESIAN_POINT('Ctrl Pts',(-66.6595549679121,-0.174800485042597,
6.33317265659175));
#31531=CARTESIAN_POINT('Ctrl Pts',(-66.6018001800214,-0.723243715815264,
6.37021862011443));
#31532=CARTESIAN_POINT('Ctrl Pts',(-66.2453468888447,-1.24025755357673,
6.40726458363711));
#31533=CARTESIAN_POINT('Ctrl Pts',(-65.7532186868384,-1.48913446656881,
6.44431054715979));
#31534=CARTESIAN_POINT('Ctrl Pts',(-65.2610904848321,-1.73801137956088,
6.48135651068247));
#31535=CARTESIAN_POINT('Ctrl Pts',(-64.6332873719962,-1.71875136778354,
6.51840247420515));
#31536=CARTESIAN_POINT('Ctrl Pts',(-64.1573426907198,-1.44035276658658,
6.55544843772783));
#31537=CARTESIAN_POINT('Ctrl Pts',(-63.6813980094434,-1.16195416538962,
6.59249440125051));
#31538=CARTESIAN_POINT('Ctrl Pts',(-63.3573117597265,-0.624416974773032,
6.6295403647732));
#31539=CARTESIAN_POINT('Ctrl Pts',(-63.3329761432024,-0.0733847413024255,
6.66658632829588));
#31540=CARTESIAN_POINT('Ctrl Pts',(-63.3086405266783,0.477647492168173,
6.70363229181856));
#31541=CARTESIAN_POINT('Ctrl Pts',(-63.5840555433469,1.04217476849279,6.74067825534123));
#31542=CARTESIAN_POINT('Ctrl Pts',(-64.0340468080883,1.36111204342974,6.77772421886391));
#31543=CARTESIAN_POINT('Ctrl Pts',(-64.4840380728297,1.68004931836668,6.81477018238659));
#31544=CARTESIAN_POINT('Ctrl Pts',(-65.1086055856438,1.75339659191594,6.85181614590928));
#31545=CARTESIAN_POINT('Ctrl Pts',(-65.6198404690058,1.54912172664725,6.88886210943196));
#31546=CARTESIAN_POINT('Ctrl Pts',(-66.1310753523678,1.34484686137856,6.92590807295464));
#31547=CARTESIAN_POINT('Ctrl Pts',(-66.5289776062776,0.862949857291932,
6.96295403647732));
#31548=CARTESIAN_POINT('Ctrl Pts',(-66.6351293272514,0.319230454628307,
7.));
#31549=CARTESIAN_POINT('',(-65.0525836066607,-1.66819787866866,7.));
#31550=CARTESIAN_POINT('Origin',(-65.,8.88178419700125E-15,7.));
#31551=CARTESIAN_POINT('',(-66.6634369488939,0.000652451249345126,6.82851963660979));
#31552=CARTESIAN_POINT('Ctrl Pts',(-65.0525835864496,-1.66819940096573,
7.));
#31553=CARTESIAN_POINT('Ctrl Pts',(-65.5930952523355,-1.6504743391327,6.96367708181444));
#31554=CARTESIAN_POINT('Ctrl Pts',(-66.1251624614536,-1.34576660284024,
6.92735416362889));
#31555=CARTESIAN_POINT('Ctrl Pts',(-66.412840678391,-0.887825324655531,
6.89103124544334));
#31556=CARTESIAN_POINT('Ctrl Pts',(-66.5778717300928,-0.625120238531662,
6.87019404249883));
#31557=CARTESIAN_POINT('Ctrl Pts',(-66.6624763097416,-0.311987213470665,
6.84935683955431));
#31558=CARTESIAN_POINT('Ctrl Pts',(-66.6634369488939,0.000652451249345126,
6.82851963660979));
#31559=CARTESIAN_POINT('',(-66.666,9.31701429861739E-15,8.));
#31560=CARTESIAN_POINT('',(-66.666,8.90896198514149E-15,3.));
#31561=CARTESIAN_POINT('Origin',(-65.,8.88178419700125E-15,8.));
#31562=CARTESIAN_POINT('Ctrl Pts',(-66.6634369488939,0.000652451249345126,
6.82851963660979));
#31563=CARTESIAN_POINT('Ctrl Pts',(-66.6641842070583,0.243847350592484,
6.81231087603163));
#31564=CARTESIAN_POINT('Ctrl Pts',(-66.614319260528,0.486743721979884,6.79610211545346));
#31565=CARTESIAN_POINT('Ctrl Pts',(-66.5123276923829,0.705373629571163,
6.7798933548753));
#31566=CARTESIAN_POINT('Ctrl Pts',(-66.2792206701092,1.20506363008265,6.74284739135262));
#31567=CARTESIAN_POINT('Ctrl Pts',(-65.7738173393357,1.577991751398,6.70580142782994));
#31568=CARTESIAN_POINT('Ctrl Pts',(-65.2274915068526,1.65321113835932,6.66875546430726));
#31569=CARTESIAN_POINT('Ctrl Pts',(-64.6811656743696,1.72843052532065,6.63170950078458));
#31570=CARTESIAN_POINT('Ctrl Pts',(-64.0939173401772,1.50594117792797,6.5946635372619));
#31571=CARTESIAN_POINT('Ctrl Pts',(-63.734467017542,1.08770559986529,6.55761757373921));
#31572=CARTESIAN_POINT('Ctrl Pts',(-63.3750166949069,0.669470021802603,
6.52057161021653));
#31573=CARTESIAN_POINT('Ctrl Pts',(-63.2433643838291,0.0554882130699169,
6.48352564669385));
#31574=CARTESIAN_POINT('Ctrl Pts',(-63.3997802821251,-0.473318066669364,
6.44647968317117));
#31575=CARTESIAN_POINT('Ctrl Pts',(-63.556196180421,-1.00212434640863,6.40943371964849));
#31576=CARTESIAN_POINT('Ctrl Pts',(-64.0006802880906,-1.4457550971545,6.37238775612581));
#31577=CARTESIAN_POINT('Ctrl Pts',(-64.5298024116317,-1.60114443125079,
6.33534179260313));
#31578=CARTESIAN_POINT('Ctrl Pts',(-65.0589245351728,-1.75653376534709,
6.29829582908045));
#31579=CARTESIAN_POINT('Ctrl Pts',(-65.6726846745854,-1.62368168279381,
6.26124986555777));
#31580=CARTESIAN_POINT('Ctrl Pts',(-66.0901968514498,-1.26340683134222,
6.22420390203509));
#31581=CARTESIAN_POINT('Ctrl Pts',(-66.4496543303097,-0.9532278785462,6.19230914689332));
#31582=CARTESIAN_POINT('Ctrl Pts',(-66.6636456701669,-0.474474884606722,
6.16041439175156));
#31583=CARTESIAN_POINT('Ctrl Pts',(-66.6675465985015,0.00121430446292491,
6.12851963660979));
#31584=CARTESIAN_POINT('Origin',(-65.,8.88178419700125E-15,3.));
#31585=CARTESIAN_POINT('',(-66.6672347084384,-0.00132477166024408,5.42851963660979));
#31586=CARTESIAN_POINT('',(-66.6636987213601,-0.000832290200039209,5.62148036339021));
#31587=CARTESIAN_POINT('',(-66.666,8.90896198514149E-15,3.));
#31588=CARTESIAN_POINT('Ctrl Pts',(-66.6636987213601,-0.000832290200039209,
5.62148036339021));
#31589=CARTESIAN_POINT('Ctrl Pts',(-66.6647135334695,-0.225194170777286,
5.63643534665464));
#31590=CARTESIAN_POINT('Ctrl Pts',(-66.6225044629126,-0.449190113916426,
5.65139032991907));
#31591=CARTESIAN_POINT('Ctrl Pts',(-66.5352578465541,-0.654000676170921,
5.6663453131835));
#31592=CARTESIAN_POINT('Ctrl Pts',(-66.3191335681149,-1.16135026554736,
5.70339127670618));
#31593=CARTESIAN_POINT('Ctrl Pts',(-65.8266432700797,-1.55097169600334,
5.74043724022886));
#31594=CARTESIAN_POINT('Ctrl Pts',(-65.2831760713864,-1.64455092497835,
5.77748320375154));
#31595=CARTESIAN_POINT('Ctrl Pts',(-64.739708872693,-1.73813015395336,5.81452916727422));
#31596=CARTESIAN_POINT('Ctrl Pts',(-64.1452647733414,-1.53566718144741,
5.8515751307969));
#31597=CARTESIAN_POINT('Ctrl Pts',(-63.771898150977,-1.12982346148107,5.88862109431958));
#31598=CARTESIAN_POINT('Ctrl Pts',(-63.3985315286127,-0.723979741514712,
5.92566705784226));
#31599=CARTESIAN_POINT('Ctrl Pts',(-63.2462423832356,-0.114755274087964,
5.96271302136494));
#31600=CARTESIAN_POINT('Ctrl Pts',(-63.3847194791661,0.419041074004913,
5.99975898488762));
#31601=CARTESIAN_POINT('Ctrl Pts',(-63.5231965750967,0.952837422097797,
6.0368049484103));
#31602=CARTESIAN_POINT('Ctrl Pts',(-63.952439912335,1.4112056508568,6.07385091193298));
#31603=CARTESIAN_POINT('Ctrl Pts',(-64.4760180935273,1.58435878418328,6.11089687545566));
#31604=CARTESIAN_POINT('Ctrl Pts',(-64.9995962747196,1.75751191750977,6.14794283897834));
#31605=CARTESIAN_POINT('Ctrl Pts',(-65.617509299866,1.64544995540375,6.18498880250103));
#31606=CARTESIAN_POINT('Ctrl Pts',(-66.0469376701368,1.29948266245883,6.22203476602371));
#31607=CARTESIAN_POINT('Ctrl Pts',(-66.431187907292,0.989912956390705,6.25518329847921));
#31608=CARTESIAN_POINT('Ctrl Pts',(-66.6645264756734,0.493065172776578,
6.28833183093471));
#31609=CARTESIAN_POINT('Ctrl Pts',(-66.6679935094968,-0.00096847687650235,
6.32148036339021));
#31610=CARTESIAN_POINT('Ctrl Pts',(-66.6675465985015,0.00121430446292491,
6.12851963660979));
#31611=CARTESIAN_POINT('Ctrl Pts',(-66.6681766235524,0.0780411722834916,
6.12336842822888));
#31612=CARTESIAN_POINT('Ctrl Pts',(-66.6633265808958,0.154788122805561,
6.11821721984797));
#31613=CARTESIAN_POINT('Ctrl Pts',(-66.6527242222132,0.230732082280723,
6.11306601146705));
#31614=CARTESIAN_POINT('Ctrl Pts',(-66.5764752017958,0.776898524102178,
6.07602004794437));
#31615=CARTESIAN_POINT('Ctrl Pts',(-66.202712946645,1.28153378739521,6.03897408442169));
#31616=CARTESIAN_POINT('Ctrl Pts',(-65.7024931149025,1.51368401519417,6.00192812089901));
#31617=CARTESIAN_POINT('Ctrl Pts',(-65.20227328316,1.74583424299314,5.96488215737633));
#31618=CARTESIAN_POINT('Ctrl Pts',(-64.5755958748258,1.70549943529802,5.92783619385365));
#31619=CARTESIAN_POINT('Ctrl Pts',(-64.1092627289642,1.41114141304214,5.89079023033097));
#31620=CARTESIAN_POINT('Ctrl Pts',(-63.6429295831026,1.11678339078626,5.85374426680829));
#31621=CARTESIAN_POINT('Ctrl Pts',(-63.3369406997136,0.568402153969617,
5.81669830328561));
#31622=CARTESIAN_POINT('Ctrl Pts',(-63.3313339461091,0.0169662842418741,
5.77965233976292));
#31623=CARTESIAN_POINT('Ctrl Pts',(-63.3257271925045,-0.534469585485869,
5.74260637624024));
#31624=CARTESIAN_POINT('Ctrl Pts',(-63.6205025686844,-1.08896008812472,
5.70556041271756));
#31625=CARTESIAN_POINT('Ctrl Pts',(-64.0807542900534,-1.39273889179927,
5.66851444919488));
#31626=CARTESIAN_POINT('Ctrl Pts',(-64.5410060114225,-1.69651769547382,
5.6314684856722));
#31627=CARTESIAN_POINT('Ctrl Pts',(-65.1667340779808,-1.74958480018409,
5.59442252214952));
#31628=CARTESIAN_POINT('Ctrl Pts',(-65.6715705742232,-1.52765405355123,
5.55737655862684));
#31629=CARTESIAN_POINT('Ctrl Pts',(-66.1764070704656,-1.30572330691838,
5.52033059510416));
#31630=CARTESIAN_POINT('Ctrl Pts',(-66.5603519963922,-0.808794708942411,
5.48328463158148));
#31631=CARTESIAN_POINT('Ctrl Pts',(-66.6476907378026,-0.264290293520927,
5.4462386680588));
#31632=CARTESIAN_POINT('Ctrl Pts',(-66.6616154028998,-0.177478398750709,
5.44033232424247));
#31633=CARTESIAN_POINT('Ctrl Pts',(-66.6680006840388,-0.0894571820797048,
5.43442598042613));
#31634=CARTESIAN_POINT('Ctrl Pts',(-66.6672347084384,-0.00132477166024408,
5.42851963660979));
#31635=CARTESIAN_POINT('Origin',(-65.,8.88178419700125E-15,3.));
#31636=CARTESIAN_POINT('',(-66.663366994258,-0.000380245158974196,4.72851963660979));
#31637=CARTESIAN_POINT('',(-66.664973747664,0.00143128352027648,4.92148036339021));
#31638=CARTESIAN_POINT('',(-66.666,8.90896198514149E-15,3.));
#31639=CARTESIAN_POINT('Ctrl Pts',(-66.664973747664,0.00143128352027648,
4.92148036339021));
#31640=CARTESIAN_POINT('Ctrl Pts',(-66.6617826067969,-0.388070057475542,
4.94749289885189));
#31641=CARTESIAN_POINT('Ctrl Pts',(-66.5254256665028,-0.779584263278036,
4.97350543431356));
#31642=CARTESIAN_POINT('Ctrl Pts',(-66.27583338404,-1.07563182061434,4.99951796977524));
#31643=CARTESIAN_POINT('Ctrl Pts',(-65.9203745090186,-1.49725035242627,
5.03656393329793));
#31644=CARTESIAN_POINT('Ctrl Pts',(-65.3352487301258,-1.72524091300358,
5.07360989682061));
#31645=CARTESIAN_POINT('Ctrl Pts',(-64.7882421463444,-1.65526230253065,
5.11065586034329));
#31646=CARTESIAN_POINT('Ctrl Pts',(-64.2412355625629,-1.58528369205772,
5.14770182386597));
#31647=CARTESIAN_POINT('Ctrl Pts',(-63.7323481738928,-1.21733591053453,
5.18474778738865));
#31648=CARTESIAN_POINT('Ctrl Pts',(-63.4944752416899,-0.719812399768212,
5.22179375091133));
#31649=CARTESIAN_POINT('Ctrl Pts',(-63.256602309487,-0.22228888900191,5.25883971443401));
#31650=CARTESIAN_POINT('Ctrl Pts',(-63.2897438337514,0.404810351007526,
5.29588567795669));
#31651=CARTESIAN_POINT('Ctrl Pts',(-63.5787322850456,0.874489902053361,
5.33293164147937));
#31652=CARTESIAN_POINT('Ctrl Pts',(-63.8677207363397,1.3441694530992,5.36997760500205));
#31653=CARTESIAN_POINT('Ctrl Pts',(-64.4125561146635,1.65642931518146,5.40702356852473));
#31654=CARTESIAN_POINT('Ctrl Pts',(-64.9638916621075,1.66836178497852,5.44406953204741));
#31655=CARTESIAN_POINT('Ctrl Pts',(-65.5152272095514,1.68029425477557,5.48111549557009));
#31656=CARTESIAN_POINT('Ctrl Pts',(-66.0730629261155,1.39189933228744,5.51816145909277));
#31657=CARTESIAN_POINT('Ctrl Pts',(-66.382101654976,0.935162996894921,5.55520742261545));
#31658=CARTESIAN_POINT('Ctrl Pts',(-66.5663853881852,0.662805298269947,
5.57729840287371));
#31659=CARTESIAN_POINT('Ctrl Pts',(-66.6621996762674,0.330587263195571,
5.59938938313196));
#31660=CARTESIAN_POINT('Ctrl Pts',(-66.6636987213601,-0.000832290200039209,
5.62148036339021));
#31661=CARTESIAN_POINT('Ctrl Pts',(-66.6672347084384,-0.00132477166024408,
5.42851963660979));
#31662=CARTESIAN_POINT('Ctrl Pts',(-66.6631963067396,0.463329814934407,
5.39738001690345));
#31663=CARTESIAN_POINT('Ctrl Pts',(-66.4603784340712,0.93107519176336,5.3662403971971));
#31664=CARTESIAN_POINT('Ctrl Pts',(-66.1156608616196,1.24098144967674,5.33510077749075));
#31665=CARTESIAN_POINT('Ctrl Pts',(-65.705559687132,1.60966854458596,5.29805481396807));
#31666=CARTESIAN_POINT('Ctrl Pts',(-65.0946247812625,1.75496250153737,5.2610088504454));
#31667=CARTESIAN_POINT('Ctrl Pts',(-64.5624539571804,1.61036875759038,5.22396288692272));
#31668=CARTESIAN_POINT('Ctrl Pts',(-64.0302831330983,1.4657750136434,5.18691692340004));
#31669=CARTESIAN_POINT('Ctrl Pts',(-63.5768763908035,1.03129356879801,5.14987095987736));
#31670=CARTESIAN_POINT('Ctrl Pts',(-63.4097379023455,0.50576729950702,5.11282499635467));
#31671=CARTESIAN_POINT('Ctrl Pts',(-63.2425994138875,-0.0197589697839626,
5.07577903283199));
#31672=CARTESIAN_POINT('Ctrl Pts',(-63.3617291792663,-0.636330063520541,
5.03873306930931));
#31673=CARTESIAN_POINT('Ctrl Pts',(-63.7126067830815,-1.06176871408085,
5.00168710578663));
#31674=CARTESIAN_POINT('Ctrl Pts',(-64.0634843868967,-1.48720736464116,
4.96464114226395));
#31675=CARTESIAN_POINT('Ctrl Pts',(-64.6461098291483,-1.72151357202521,
4.92759517874127));
#31676=CARTESIAN_POINT('Ctrl Pts',(-65.1938412738805,-1.65745577708111,
4.89054921521859));
#31677=CARTESIAN_POINT('Ctrl Pts',(-65.7415727186126,-1.59339798213701,
4.85350325169591));
#31678=CARTESIAN_POINT('Ctrl Pts',(-66.2544101658253,-1.23097618486477,
4.81645728817322));
#31679=CARTESIAN_POINT('Ctrl Pts',(-66.4976506491046,-0.73605477318721,
4.77941132465054));
#31680=CARTESIAN_POINT('Ctrl Pts',(-66.6090340731616,-0.509422920098683,
4.76244742863696));
#31681=CARTESIAN_POINT('Ctrl Pts',(-66.6638867910221,-0.255007754231674,
4.74548353262337));
#31682=CARTESIAN_POINT('Ctrl Pts',(-66.663366994258,-0.000380245158974196,
4.72851963660979));
#31683=CARTESIAN_POINT('Origin',(-65.,8.88178419700125E-15,3.));
#31684=CARTESIAN_POINT('',(-66.66584023827,0.00152342185142561,4.02851963660979));
#31685=CARTESIAN_POINT('',(-66.668752404953,-6.71116606238314E-6,4.22148036339021));
#31686=CARTESIAN_POINT('',(-66.666,8.90896198514149E-15,3.));
#31687=CARTESIAN_POINT('Ctrl Pts',(-66.6687523910643,-6.71113219753621E-6,
4.22148036339021));
#31688=CARTESIAN_POINT('Ctrl Pts',(-66.6687853501023,-0.551830446441265,
4.25855045104914));
#31689=CARTESIAN_POINT('Ctrl Pts',(-66.3679399440666,-1.10362329032224,
4.29562053870807));
#31690=CARTESIAN_POINT('Ctrl Pts',(-65.9041274583633,-1.40260051189835,
4.332690626367));
#31691=CARTESIAN_POINT('Ctrl Pts',(-65.440616808353,-1.70138316778324,4.36973658988968));
#31692=CARTESIAN_POINT('Ctrl Pts',(-64.8143512345865,-1.74767914449737,
4.40678255341236));
#31693=CARTESIAN_POINT('Ctrl Pts',(-64.3119447275275,-1.52030082532264,
4.44382851693504));
#31694=CARTESIAN_POINT('Ctrl Pts',(-63.8095382204685,-1.2929225061479,4.48087448045772));
#31695=CARTESIAN_POINT('Ctrl Pts',(-63.430990780117,-0.791869891084301,
4.5179204439804));
#31696=CARTESIAN_POINT('Ctrl Pts',(-63.3495467901205,-0.246452551482032,
4.55496640750308));
#31697=CARTESIAN_POINT('Ctrl Pts',(-63.2681028001239,0.298964788120236,
4.59201237102576));
#31698=CARTESIAN_POINT('Ctrl Pts',(-63.4837622604823,0.888746852261173,
4.62905833454844));
#31699=CARTESIAN_POINT('Ctrl Pts',(-63.897827394199,1.25297653677901,4.66610429807112));
#31700=CARTESIAN_POINT('Ctrl Pts',(-64.3118925279157,1.61720622129685,4.7031502615938));
#31701=CARTESIAN_POINT('Ctrl Pts',(-64.9243633349907,1.7558835261916,4.74019622511648));
#31702=CARTESIAN_POINT('Ctrl Pts',(-65.4549390817441,1.60554199300636,4.77724218863916));
#31703=CARTESIAN_POINT('Ctrl Pts',(-65.9855148284976,1.45520045982113,4.81428815216184));
#31704=CARTESIAN_POINT('Ctrl Pts',(-66.4341955149295,1.01584008855591,4.85133411568453));
#31705=CARTESIAN_POINT('Ctrl Pts',(-66.5956398725704,0.488536651400025,
4.88838007920721));
#31706=CARTESIAN_POINT('Ctrl Pts',(-66.643722970876,0.331489459561816,4.89941350726821));
#31707=CARTESIAN_POINT('Ctrl Pts',(-66.6663272959654,0.166641438903683,
4.91044693532921));
#31708=CARTESIAN_POINT('Ctrl Pts',(-66.664973747664,0.00143128352027648,
4.92148036339021));
#31709=CARTESIAN_POINT('Ctrl Pts',(-66.663366994258,-0.000380245158974196,
4.72851963660979));
#31710=CARTESIAN_POINT('Ctrl Pts',(-66.6627516524935,0.301050913271586,
4.7084375691007));
#31711=CARTESIAN_POINT('Ctrl Pts',(-66.5845366381801,0.602779651888659,
4.6883555015916));
#31712=CARTESIAN_POINT('Ctrl Pts',(-66.4306434003258,0.859065513400944,
4.66827343408251));
#31713=CARTESIAN_POINT('Ctrl Pts',(-66.1467521489217,1.33184336222866,4.63122747055983));
#31714=CARTESIAN_POINT('Ctrl Pts',(-65.6053261267676,1.64997803380121,4.59418150703714));
#31715=CARTESIAN_POINT('Ctrl Pts',(-65.0541520228137,1.6678733924142,4.55713554351446));
#31716=CARTESIAN_POINT('Ctrl Pts',(-64.5029779188599,1.68576875102718,4.52008957999178));
#31717=CARTESIAN_POINT('Ctrl Pts',(-63.9420557331062,1.40342479668061,4.4830436164691));
#31718=CARTESIAN_POINT('Ctrl Pts',(-63.6280946846009,0.950057840731767,
4.44599765294642));
#31719=CARTESIAN_POINT('Ctrl Pts',(-63.3141336360955,0.496690884782925,
4.40895168942374));
#31720=CARTESIAN_POINT('Ctrl Pts',(-63.2471337248385,-0.12769907276818,
4.37190572590106));
#31721=CARTESIAN_POINT('Ctrl Pts',(-63.4577578400848,-0.637356427139624,
4.33485976237838));
#31722=CARTESIAN_POINT('Ctrl Pts',(-63.6683819553311,-1.14701378151105,
4.2978137988557));
#31723=CARTESIAN_POINT('Ctrl Pts',(-64.1566300970808,-1.54193853270284,
4.26076783533302));
#31724=CARTESIAN_POINT('Ctrl Pts',(-64.6990527347307,-1.64139112904608,
4.22372187181034));
#31725=CARTESIAN_POINT('Ctrl Pts',(-65.2414753723806,-1.74084372538932,
4.18667590828766));
#31726=CARTESIAN_POINT('Ctrl Pts',(-65.8380725059307,-1.54482416688402,
4.14962994476498));
#31727=CARTESIAN_POINT('Ctrl Pts',(-66.2158080742639,-1.14304191594114,
4.1125839812423));
#31728=CARTESIAN_POINT('Ctrl Pts',(-66.501526048881,-0.839135107580329,
4.08456253303146));
#31729=CARTESIAN_POINT('Ctrl Pts',(-66.6620254174182,-0.417504031348412,
4.05654108482063));
#31730=CARTESIAN_POINT('Ctrl Pts',(-66.66584023827,0.00152342185142561,
4.02851963660979));
#31731=CARTESIAN_POINT('Origin',(-65.,8.88178419700125E-15,3.));
#31732=CARTESIAN_POINT('',(-66.6685304876972,-0.000550348904949371,3.32851963660979));
#31733=CARTESIAN_POINT('',(-66.6649541686305,-0.00142706439963382,3.52148036339021));
#31734=CARTESIAN_POINT('',(-66.666,8.90896198514149E-15,3.));
#31735=CARTESIAN_POINT('Ctrl Pts',(-66.6649541686305,-0.00142706439963382,
3.52148036339021));
#31736=CARTESIAN_POINT('Ctrl Pts',(-66.6663084639771,-0.167364609070321,
3.53256203972371));
#31737=CARTESIAN_POINT('Ctrl Pts',(-66.6435020576938,-0.332938268252238,
3.5436437160572));
#31738=CARTESIAN_POINT('Ctrl Pts',(-66.5950038039968,-0.490609337973565,
3.5547253923907));
#31739=CARTESIAN_POINT('Ctrl Pts',(-66.4328744940168,-1.017702579257,3.59177135591338));
#31740=CARTESIAN_POINT('Ctrl Pts',(-65.9836233623828,-1.45647963816642,
3.62881731943606));
#31741=CARTESIAN_POINT('Ctrl Pts',(-65.4528527369189,-1.60613170566074,
3.66586328295875));
#31742=CARTESIAN_POINT('Ctrl Pts',(-64.9220821114551,-1.75578377315507,
3.70290924648143));
#31743=CARTESIAN_POINT('Ctrl Pts',(-64.3097919921614,-1.6163108492343,3.73995521000411));
#31744=CARTESIAN_POINT('Ctrl Pts',(-63.8962004240445,-1.25154350838823,
3.77700117352679));
#31745=CARTESIAN_POINT('Ctrl Pts',(-63.4826088559277,-0.886776167542167,
3.81404713704947));
#31746=CARTESIAN_POINT('Ctrl Pts',(-63.2677158389876,-0.296714409770812,
3.85109310057215));
#31747=CARTESIAN_POINT('Ctrl Pts',(-63.3498683809715,0.248596655588651,
3.88813906409483));
#31748=CARTESIAN_POINT('Ctrl Pts',(-63.4320209229553,0.793907720948114,
3.92518502761751));
#31749=CARTESIAN_POINT('Ctrl Pts',(-63.8112190238629,1.29446809389569,3.96223099114019));
#31750=CARTESIAN_POINT('Ctrl Pts',(-64.3139205225789,1.52119348141189,3.99927695466287));
#31751=CARTESIAN_POINT('Ctrl Pts',(-64.8166220212948,1.7479188689281,4.03632291818555));
#31752=CARTESIAN_POINT('Ctrl Pts',(-65.4428269178191,1.70080927101295,4.07336888170823));
#31753=CARTESIAN_POINT('Ctrl Pts',(-65.9059489905043,1.40142466222205,4.11041484523092));
#31754=CARTESIAN_POINT('Ctrl Pts',(-66.368769480536,1.10223501111092,4.14743668461735));
#31755=CARTESIAN_POINT('Ctrl Pts',(-66.6687194749238,0.551098802461351,
4.18445852400378));
#31756=CARTESIAN_POINT('Ctrl Pts',(-66.6687523910643,-6.71113219753621E-6,
4.22148036339021));
#31757=CARTESIAN_POINT('Ctrl Pts',(-66.66584023827,0.00152342185142561,
4.02851963660979));
#31758=CARTESIAN_POINT('Ctrl Pts',(-66.6670688296308,0.136474322284305,
4.01949512129795));
#31759=CARTESIAN_POINT('Ctrl Pts',(-66.6520459458893,0.271155172380335,
4.0104706059861));
#31760=CARTESIAN_POINT('Ctrl Pts',(-66.6197204952159,0.401546525825023,
4.00144609067426));
#31761=CARTESIAN_POINT('Ctrl Pts',(-66.4870233447183,0.936807773267803,
3.96440012715158));
#31762=CARTESIAN_POINT('Ctrl Pts',(-66.0627550406069,1.39978532477288,3.92735416362889));
#31763=CARTESIAN_POINT('Ctrl Pts',(-65.54108437802,1.5785948786444,3.89030820010621));
#31764=CARTESIAN_POINT('Ctrl Pts',(-65.0194137154332,1.75740443251591,3.85326223658353));
#31765=CARTESIAN_POINT('Ctrl Pts',(-64.400340694371,1.65204598875386,3.81621627306085));
#31766=CARTESIAN_POINT('Ctrl Pts',(-63.9671875933068,1.31073743656301,3.77917030953817));
#31767=CARTESIAN_POINT('Ctrl Pts',(-63.5340344922426,0.96942888437217,3.74212434601549));
#31768=CARTESIAN_POINT('Ctrl Pts',(-63.2868013111764,0.392170223752536,
3.70507838249281));
#31769=CARTESIAN_POINT('Ctrl Pts',(-63.3386357173299,-0.156852845981067,
3.66803241897013));
#31770=CARTESIAN_POINT('Ctrl Pts',(-63.3904701234834,-0.705875915714671,
3.63098645544745));
#31771=CARTESIAN_POINT('Ctrl Pts',(-63.7413721168566,-1.22666339456225,
3.59394049192477));
#31772=CARTESIAN_POINT('Ctrl Pts',(-64.230749410433,-1.48087393976487,3.55689452840209));
#31773=CARTESIAN_POINT('Ctrl Pts',(-64.7201267040094,-1.73508448496749,
3.51984856487941));
#31774=CARTESIAN_POINT('Ctrl Pts',(-65.347979297789,-1.72271809652517,3.48280260135673));
#31775=CARTESIAN_POINT('Ctrl Pts',(-65.826966892062,-1.44943432222994,3.44575663783405));
#31776=CARTESIAN_POINT('Ctrl Pts',(-66.305954486335,-1.17615054793471,3.40871067431137));
#31777=CARTESIAN_POINT('Ctrl Pts',(-66.6360770811014,-0.641949387786585,
3.37166471078869));
#31778=CARTESIAN_POINT('Ctrl Pts',(-66.6662521989441,-0.0913110318543388,
3.33461874726601));
#31779=CARTESIAN_POINT('Ctrl Pts',(-66.6679081722746,-0.0610926765551588,
3.3325857103806));
#31780=CARTESIAN_POINT('Ctrl Pts',(-66.668660799992,-0.0308248176933715,
3.3305526734952));
#31781=CARTESIAN_POINT('Ctrl Pts',(-66.6685304876972,-0.000550348904949371,
3.32851963660979));
#31782=CARTESIAN_POINT('Origin',(-65.,8.88178419700125E-15,3.));
#31783=CARTESIAN_POINT('',(-66.664215437255,-0.00117645755964804,2.62851963660979));
#31784=CARTESIAN_POINT('',(-66.663709965026,0.000842507685015625,2.82148036339021));
#31785=CARTESIAN_POINT('',(-66.666,8.90896198514149E-15,3.));
#31786=CARTESIAN_POINT('Ctrl Pts',(-66.663709965026,0.000842507685015625,
2.82148036339021));
#31787=CARTESIAN_POINT('Ctrl Pts',(-66.6621889226241,-0.331295501917179,
2.84361959192095));
#31788=CARTESIAN_POINT('Ctrl Pts',(-66.565926135999,-0.664245551393369,
2.8657588204517));
#31789=CARTESIAN_POINT('Ctrl Pts',(-66.3808853648239,-0.936957985442174,
2.88789804898245));
#31790=CARTESIAN_POINT('Ctrl Pts',(-66.0712533625325,-1.39329253521755,
2.92494401250513));
#31791=CARTESIAN_POINT('Ctrl Pts',(-65.5130436951299,-1.68096223107997,
2.96198997602781));
#31792=CARTESIAN_POINT('Ctrl Pts',(-64.9617241821671,-1.66831340551996,
2.9990359395505));
#31793=CARTESIAN_POINT('Ctrl Pts',(-64.4104046692042,-1.65566457995995,
3.03608190307317));
#31794=CARTESIAN_POINT('Ctrl Pts',(-63.8659753106812,-1.34269723297749,
3.07312786659585));
#31795=CARTESIAN_POINT('Ctrl Pts',(-63.5775972896502,-0.872642645564539,
3.11017383011853));
#31796=CARTESIAN_POINT('Ctrl Pts',(-63.2892192686192,-0.402588058151592,
3.14721979364122));
#31797=CARTESIAN_POINT('Ctrl Pts',(-63.2568925850803,0.22455376969184,3.1842657571639));
#31798=CARTESIAN_POINT('Ctrl Pts',(-63.4954117290602,0.721767824316931,
3.22131172068658));
#31799=CARTESIAN_POINT('Ctrl Pts',(-63.73393087304,1.21898187894203,3.25835768420926));
#31800=CARTESIAN_POINT('Ctrl Pts',(-64.2432958445387,1.58626816034878,3.29540364773194));
#31801=CARTESIAN_POINT('Ctrl Pts',(-64.7903928760533,1.65553601919702,3.33244961125462));
#31802=CARTESIAN_POINT('Ctrl Pts',(-65.3374899075679,1.72480387804527,3.3694955747773));
#31803=CARTESIAN_POINT('Ctrl Pts',(-65.9223189990984,1.49605331433501,3.40654153829998));
#31804=CARTESIAN_POINT('Ctrl Pts',(-66.2772298007007,1.07397332065117,3.44358750182266));
#31805=CARTESIAN_POINT('Ctrl Pts',(-66.5259750107882,0.77815145152619,3.46955178901184));
#31806=CARTESIAN_POINT('Ctrl Pts',(-66.6617810644663,0.387363397948813,
3.49551607620103));
#31807=CARTESIAN_POINT('Ctrl Pts',(-66.6649541686305,-0.00142706439963382,
3.52148036339021));
#31808=CARTESIAN_POINT('Ctrl Pts',(-66.6685304876972,-0.000550348904949371,
3.32851963660979));
#31809=CARTESIAN_POINT('Ctrl Pts',(-66.6662862515739,0.520836037284772,
3.29350670997252));
#31810=CARTESIAN_POINT('Ctrl Pts',(-66.4021649235169,1.04418290588671,3.25849378333524));
#31811=CARTESIAN_POINT('Ctrl Pts',(-65.9803979715476,1.35039028151488,3.22348085669796));
#31812=CARTESIAN_POINT('Ctrl Pts',(-65.5341409853895,1.67437768723549,3.18643489317528));
#31813=CARTESIAN_POINT('Ctrl Pts',(-64.9113993721543,1.75527694696034,3.1493889296526));
#31814=CARTESIAN_POINT('Ctrl Pts',(-64.3971743623243,1.55606405574625,3.11234296612992));
#31815=CARTESIAN_POINT('Ctrl Pts',(-63.8829493524943,1.35685116453216,3.07529700260724));
#31816=CARTESIAN_POINT('Ctrl Pts',(-63.4772409460695,0.877526122379138,
3.03825103908456));
#31817=CARTESIAN_POINT('Ctrl Pts',(-63.3657238957733,0.337454752786405,
3.00120507556188));
#31818=CARTESIAN_POINT('Ctrl Pts',(-63.2542068454771,-0.202616616806327,
2.9641591120392));
#31819=CARTESIAN_POINT('Ctrl Pts',(-63.4368811513095,-0.803434313838767,
2.92711314851652));
#31820=CARTESIAN_POINT('Ctrl Pts',(-63.8301448813726,-1.19003071239599,
2.89006718499384));
#31821=CARTESIAN_POINT('Ctrl Pts',(-64.2234086114356,-1.57662711095321,
2.85302122147116));
#31822=CARTESIAN_POINT('Ctrl Pts',(-64.8272617657294,-1.74900221103521,
2.81597525794848));
#31823=CARTESIAN_POINT('Ctrl Pts',(-65.3653475241109,-1.62826757065615,
2.7789292944258));
#31824=CARTESIAN_POINT('Ctrl Pts',(-65.9034332824925,-1.5075329302771,2.74188333090311));
#31825=CARTESIAN_POINT('Ctrl Pts',(-66.3757516449619,-1.09368854943699,
2.70483736738043));
#31826=CARTESIAN_POINT('Ctrl Pts',(-66.5661434347078,-0.576132655684546,
2.66779140385775));
#31827=CARTESIAN_POINT('Ctrl Pts',(-66.6334204184134,-0.393248722101033,
2.6547008147751));
#31828=CARTESIAN_POINT('Ctrl Pts',(-66.6654949753924,-0.197414973610965,
2.64161022569244));
#31829=CARTESIAN_POINT('Ctrl Pts',(-66.664215437255,-0.00117645755964804,
2.62851963660979));
#31830=CARTESIAN_POINT('Origin',(-65.,8.88178419700125E-15,3.));
#31831=CARTESIAN_POINT('',(-66.6642789433678,0.00120644035141754,1.92851963660979));
#31832=CARTESIAN_POINT('',(-66.6680288432953,0.000974731038378531,2.1214803633902));
#31833=CARTESIAN_POINT('',(-66.666,8.90896198514149E-15,3.));
#31834=CARTESIAN_POINT('Ctrl Pts',(-66.6680288432953,0.000974731038378531,
2.1214803633902));
#31835=CARTESIAN_POINT('Ctrl Pts',(-66.6645899038029,-0.49376054930324,
2.1546771441182));
#31836=CARTESIAN_POINT('Ctrl Pts',(-66.4304593550116,-0.99132262932826,
2.1878739248462));
#31837=CARTESIAN_POINT('Ctrl Pts',(-66.0452404987214,-1.30084855271515,
2.2210707055742));
#31838=CARTESIAN_POINT('Ctrl Pts',(-65.6153553295749,-1.64626415674821,
2.25811666909688));
#31839=CARTESIAN_POINT('Ctrl Pts',(-64.9973130191693,-1.75750978249457,
2.29516263261956));
#31840=CARTESIAN_POINT('Ctrl Pts',(-64.4739641353999,-1.58367323852582,
2.33220859614224));
#31841=CARTESIAN_POINT('Ctrl Pts',(-63.9506152516305,-1.40983669455707,
2.36925455966492));
#31842=CARTESIAN_POINT('Ctrl Pts',(-63.5219597944974,-0.950917980873204,
2.40630052318761));
#31843=CARTESIAN_POINT('Ctrl Pts',(-63.3841743645993,-0.41694384903774,
2.44334648671029));
#31844=CARTESIAN_POINT('Ctrl Pts',(-63.2463889347012,0.117030282797723,
2.48039245023297));
#31845=CARTESIAN_POINT('Ctrl Pts',(-63.399473532038,0.726059832784788,2.51743841375565));
#31846=CARTESIAN_POINT('Ctrl Pts',(-63.77336812259,1.13141897393944,2.55448437727833));
#31847=CARTESIAN_POINT('Ctrl Pts',(-64.1472627131419,1.53677811509409,2.59153034080101));
#31848=CARTESIAN_POINT('Ctrl Pts',(-64.741967296909,1.73846684741633,2.62857630432369));
#31849=CARTESIAN_POINT('Ctrl Pts',(-65.2853119489257,1.64418117890599,2.66562226784637));
#31850=CARTESIAN_POINT('Ctrl Pts',(-65.8286566009425,1.54989551039566,2.70266823136905));
#31851=CARTESIAN_POINT('Ctrl Pts',(-66.3206413212089,1.15963544105275,2.73971419489173));
#31852=CARTESIAN_POINT('Ctrl Pts',(-66.5361065127521,0.652005704537134,
2.77676015841441));
#31853=CARTESIAN_POINT('Ctrl Pts',(-66.6228064445369,0.447743182072859,
2.79166689340634));
#31854=CARTESIAN_POINT('Ctrl Pts',(-66.664734109836,0.224476916761689,2.80657362839827));
#31855=CARTESIAN_POINT('Ctrl Pts',(-66.663709965026,0.000842507685015625,
2.82148036339021));
#31856=CARTESIAN_POINT('Ctrl Pts',(-66.664215437255,-0.00117645755964804,
2.62851963660979));
#31857=CARTESIAN_POINT('Ctrl Pts',(-66.6618739219115,0.357933976805246,
2.60456426216976));
#31858=CARTESIAN_POINT('Ctrl Pts',(-66.5478366409886,0.718399891583497,
2.58060888772974));
#31859=CARTESIAN_POINT('Ctrl Pts',(-66.3334304982421,1.00334301282383,2.55665351328971));
#31860=CARTESIAN_POINT('Ctrl Pts',(-66.0018605550081,1.44399538091501,2.51960754976703));
#31861=CARTESIAN_POINT('Ctrl Pts',(-65.4302554515179,1.70403271043259,2.48256158624435));
#31862=CARTESIAN_POINT('Ctrl Pts',(-64.880213504605,1.6644474430109,2.44551562272167));
#31863=CARTESIAN_POINT('Ctrl Pts',(-64.3301715576922,1.62486217558921,2.40846965919899));
#31864=CARTESIAN_POINT('Ctrl Pts',(-63.8016927673567,1.28565431122825,2.37142369567631));
#31865=CARTESIAN_POINT('Ctrl Pts',(-63.5366384486743,0.802064252492247,
2.33437773215363));
#31866=CARTESIAN_POINT('Ctrl Pts',(-63.2715841299918,0.318474193756241,
2.29733176863095));
#31867=CARTESIAN_POINT('Ctrl Pts',(-63.2699542829623,-0.309498059354816,
2.26028580510827));
#31868=CARTESIAN_POINT('Ctrl Pts',(-63.5324948163207,-0.794457444359814,
2.22323984158559));
#31869=CARTESIAN_POINT('Ctrl Pts',(-63.795035349679,-1.27941682936481,2.18619387806291));
#31870=CARTESIAN_POINT('Ctrl Pts',(-64.3217462634253,-1.62136334626375,
2.14914791454023));
#31871=CARTESIAN_POINT('Ctrl Pts',(-64.8715753212295,-1.66380323262915,
2.11210195101754));
#31872=CARTESIAN_POINT('Ctrl Pts',(-65.4214043790337,-1.70624311899455,
2.07505598749486));
#31873=CARTESIAN_POINT('Ctrl Pts',(-65.9943515808958,-1.44917637482641,
2.03801002397218));
#31874=CARTESIAN_POINT('Ctrl Pts',(-66.3282043910519,-1.01025105326097,
2.0009640604495));
#31875=CARTESIAN_POINT('Ctrl Pts',(-66.54582391177,-0.724140781894937,1.9768159191696));
#31876=CARTESIAN_POINT('Ctrl Pts',(-66.6618524838225,-0.360758997512868,
1.95266777788969));
#31877=CARTESIAN_POINT('Ctrl Pts',(-66.6642789433678,0.00120644035141754,
1.92851963660979));
#31878=CARTESIAN_POINT('Origin',(-65.,8.88178419700125E-15,3.));
#31879=CARTESIAN_POINT('',(-66.6685688018723,0.000500570493875176,1.22851963660979));
#31880=CARTESIAN_POINT('',(-66.6666630352664,-0.00145874010107553,1.4214803633902));
#31881=CARTESIAN_POINT('',(-66.666,8.90896198514149E-15,3.));
#31882=CARTESIAN_POINT('Ctrl Pts',(-66.6666630352664,-0.00145874010107553,
1.4214803633902));
#31883=CARTESIAN_POINT('Ctrl Pts',(-66.6676496745696,-0.109114984958735,
1.42868873279277));
#31884=CARTESIAN_POINT('Ctrl Pts',(-66.6581116875295,-0.216597146837632,
1.43589710219534));
#31885=CARTESIAN_POINT('Ctrl Pts',(-66.6374139306422,-0.321885502945873,
1.44310547159791));
#31886=CARTESIAN_POINT('Ctrl Pts',(-66.5310419755125,-0.862993814953153,
1.48015143512059));
#31887=CARTESIAN_POINT('Ctrl Pts',(-66.1299138139174,-1.34615847081563,
1.51719739864327));
#31888=CARTESIAN_POINT('Ctrl Pts',(-65.6176080235618,-1.55025642604728,
1.55424336216595));
#31889=CARTESIAN_POINT('Ctrl Pts',(-65.1053022332063,-1.75435438127892,
1.59128932568863));
#31890=CARTESIAN_POINT('Ctrl Pts',(-64.4818188140901,-1.67938563587972,
1.62833528921131));
#31891=CARTESIAN_POINT('Ctrl Pts',(-64.0324984883637,-1.35966006128364,
1.66538125273399));
#31892=CARTESIAN_POINT('Ctrl Pts',(-63.5831781626372,-1.03993448668757,
1.70242721625667));
#31893=CARTESIAN_POINT('Ctrl Pts',(-63.3080209303004,-0.475452082894621,
1.73947317977936));
#31894=CARTESIAN_POINT('Ctrl Pts',(-63.3329540589798,0.0754485771665916,
1.77651914330204));
#31895=CARTESIAN_POINT('Ctrl Pts',(-63.3578871876591,0.626349237227804,
1.81356510682472));
#31896=CARTESIAN_POINT('Ctrl Pts',(-63.6829106773545,1.16366815355728,1.8506110703474));
#31897=CARTESIAN_POINT('Ctrl Pts',(-64.1592756849985,1.44149827729127,1.88765703387008));
#31898=CARTESIAN_POINT('Ctrl Pts',(-64.6356406926424,1.71932840102527,1.92470299739276));
#31899=CARTESIAN_POINT('Ctrl Pts',(-65.2633472182348,1.73766973216378,1.96174896091544));
#31900=CARTESIAN_POINT('Ctrl Pts',(-65.7551218110002,1.48812825650889,1.99879492443812));
#31901=CARTESIAN_POINT('Ctrl Pts',(-66.2468964037657,1.23858678085399,2.0358408879608));
#31902=CARTESIAN_POINT('Ctrl Pts',(-66.6027390637042,0.721162498405699,
2.07288685148348));
#31903=CARTESIAN_POINT('Ctrl Pts',(-66.6597963797297,0.172657566021677,
2.10993281500616));
#31904=CARTESIAN_POINT('Ctrl Pts',(-66.6657247999481,0.115666316563748,
2.11378199780084));
#31905=CARTESIAN_POINT('Ctrl Pts',(-66.6684275899941,0.0583395262760883,
2.11763118059552));
#31906=CARTESIAN_POINT('Ctrl Pts',(-66.6680288432953,0.000974731038378531,
2.1214803633902));
#31907=CARTESIAN_POINT('Ctrl Pts',(-66.6642789433678,0.00120644035141754,
1.92851963660979));
#31908=CARTESIAN_POINT('Ctrl Pts',(-66.6655749455541,0.194536677303725,
1.91562181436701));
#31909=CARTESIAN_POINT('Ctrl Pts',(-66.634462982395,0.387462864473397,1.90272399212424));
#31910=CARTESIAN_POINT('Ctrl Pts',(-66.5691129188822,0.567995372183053,
1.88982616988146));
#31911=CARTESIAN_POINT('Ctrl Pts',(-66.3814102181061,1.08653257709889,1.85278020635878));
#31912=CARTESIAN_POINT('Ctrl Pts',(-65.9112463981035,1.50282308796782,1.8157342428361));
#31913=CARTESIAN_POINT('Ctrl Pts',(-65.3737945971089,1.62634919196252,1.77868827931342));
#31914=CARTESIAN_POINT('Ctrl Pts',(-64.8363427961142,1.74987529595721,1.74164231579074));
#31915=CARTESIAN_POINT('Ctrl Pts',(-64.2316030141275,1.58063699307768,1.70459635226806));
#31916=CARTESIAN_POINT('Ctrl Pts',(-63.8363378414827,1.19608715228399,1.66755038874538));
#31917=CARTESIAN_POINT('Ctrl Pts',(-63.4410726688379,0.811537311490293,
1.6305044252227));
#31918=CARTESIAN_POINT('Ctrl Pts',(-63.2552821055351,0.211675932782425,
1.59345846170002));
#31919=CARTESIAN_POINT('Ctrl Pts',(-63.3639942563739,-0.328967022430164,
1.55641249817734));
#31920=CARTESIAN_POINT('Ctrl Pts',(-63.4727064072127,-0.869609977642748,
1.51936653465465));
#31921=CARTESIAN_POINT('Ctrl Pts',(-63.8759212721932,-1.35103450936006,
1.48232057113197));
#31922=CARTESIAN_POINT('Ctrl Pts',(-64.3891052819731,-1.55291395077578,
1.44527460760929));
#31923=CARTESIAN_POINT('Ctrl Pts',(-64.9022892917531,-1.75479339219151,
1.40822864408661));
#31924=CARTESIAN_POINT('Ctrl Pts',(-65.5254424463325,-1.67712774330567,
1.37118268056393));
#31925=CARTESIAN_POINT('Ctrl Pts',(-65.9733751709996,-1.35546112873117,
1.33413671704125));
#31926=CARTESIAN_POINT('Ctrl Pts',(-66.3990566948007,-1.0497734057594,1.2989310235641));
#31927=CARTESIAN_POINT('Ctrl Pts',(-66.6664936696292,-0.5237242626975,1.26372533008694));
#31928=CARTESIAN_POINT('Ctrl Pts',(-66.6685688018723,0.000500570493875176,
1.22851963660979));
#31929=CARTESIAN_POINT('Origin',(-65.,8.88178419700125E-15,3.));
#31930=CARTESIAN_POINT('',(-66.6657538157597,-0.00152189319960278,0.528519636609788));
#31931=CARTESIAN_POINT('',(-66.6632893889008,-6.33249066055908E-5,0.721480363390205));
#31932=CARTESIAN_POINT('',(-66.666,8.90896198514149E-15,3.));
#31933=CARTESIAN_POINT('Ctrl Pts',(-66.6632893889008,-6.33249066055908E-5,
0.721480363390205));
#31934=CARTESIAN_POINT('Ctrl Pts',(-66.663382354964,-0.274266208525866,
0.739746284990023));
#31935=CARTESIAN_POINT('Ctrl Pts',(-66.5993416986523,-0.548428211919451,
0.758012206589842));
#31936=CARTESIAN_POINT('Ctrl Pts',(-66.4709289590166,-0.788100662831112,
0.77627812818966));
#31937=CARTESIAN_POINT('Ctrl Pts',(-66.2104891206872,-1.274191486409,0.81332409171234));
#31938=CARTESIAN_POINT('Ctrl Pts',(-65.6852625770594,-1.61841374682522,
0.850370055235021));
#31939=CARTESIAN_POINT('Ctrl Pts',(-65.1356222340335,-1.66323217468976,
0.887416018757702));
#31940=CARTESIAN_POINT('Ctrl Pts',(-64.5859818910076,-1.7080506025543,0.924461982280382));
#31941=CARTESIAN_POINT('Ctrl Pts',(-64.0119277485837,-1.45346519786716,
0.961507945803063));
#31942=CARTESIAN_POINT('Ctrl Pts',(-63.6761789401645,-1.01598841469988,
0.998553909325744));
#31943=CARTESIAN_POINT('Ctrl Pts',(-63.3404301317454,-0.578511631532607,
1.03559987284842));
#31944=CARTESIAN_POINT('Ctrl Pts',(-63.242986657331,0.0418565301148077,
1.0726458363711));
#31945=CARTESIAN_POINT('Ctrl Pts',(-63.4284440755221,0.561201063347344,
1.10969179989379));
#31946=CARTESIAN_POINT('Ctrl Pts',(-63.6139014937132,1.08054559657989,1.14673776341647));
#31947=CARTESIAN_POINT('Ctrl Pts',(-64.0822598045097,1.49886650139754,1.18378372693915));
#31948=CARTESIAN_POINT('Ctrl Pts',(-64.619172171207,1.62471684366477,1.22082969046183));
#31949=CARTESIAN_POINT('Ctrl Pts',(-65.1560845379043,1.75056718593199,1.25787565398451));
#31950=CARTESIAN_POINT('Ctrl Pts',(-65.7615509605024,1.58394696564878,1.29492161750719));
#31951=CARTESIAN_POINT('Ctrl Pts',(-66.1584762974693,1.20111087143114,1.33196758102987));
#31952=CARTESIAN_POINT('Ctrl Pts',(-66.4781682685839,0.892766671210744,
1.36180517514998));
#31953=CARTESIAN_POINT('Ctrl Pts',(-66.6625790404782,0.444162614627713,
1.39164276927009));
#31954=CARTESIAN_POINT('Ctrl Pts',(-66.6666630352664,-0.00145874010107553,
1.4214803633902));
#31955=CARTESIAN_POINT('Ctrl Pts',(-66.6685688018723,0.000500570493875176,
1.22851963660979));
#31956=CARTESIAN_POINT('Ctrl Pts',(-66.6686772730691,0.0279028217311334,
1.22667936656426));
#31957=CARTESIAN_POINT('Ctrl Pts',(-66.6680606812028,0.0553000883040936,
1.22483909651874));
#31958=CARTESIAN_POINT('Ctrl Pts',(-66.6667037271851,0.082660636409592,
1.22299882647321));
#31959=CARTESIAN_POINT('Ctrl Pts',(-66.6393872639487,0.633448206712722,
1.18595286295053));
#31960=CARTESIAN_POINT('Ctrl Pts',(-66.3120420427213,1.16935576705584,1.14890689942785));
#31961=CARTESIAN_POINT('Ctrl Pts',(-65.8344794601719,1.44512218362151,1.11186093590517));
#31962=CARTESIAN_POINT('Ctrl Pts',(-65.3569168776225,1.72088860018718,1.07481497238249));
#31963=CARTESIAN_POINT('Ctrl Pts',(-64.729136933751,1.73651387297539,1.03776900885981));
#31964=CARTESIAN_POINT('Ctrl Pts',(-64.2384466796233,1.48484700734035,1.00072304533713));
#31965=CARTESIAN_POINT('Ctrl Pts',(-63.7477564254956,1.23318014170531,0.963677081814447));
#31966=CARTESIAN_POINT('Ctrl Pts',(-63.3941558611116,0.714221137647021,
0.926631118291766));
#31967=CARTESIAN_POINT('Ctrl Pts',(-63.3394722898162,0.165474525977697,
0.889585154769085));
#31968=CARTESIAN_POINT('Ctrl Pts',(-63.2847887185207,-0.383272085691625,
0.852539191246405));
#31969=CARTESIAN_POINT('Ctrl Pts',(-63.5290221403138,-0.961806304971977,
0.815493227723724));
#31970=CARTESIAN_POINT('Ctrl Pts',(-63.9603977448083,-1.30535866571471,
0.778447264201044));
#31971=CARTESIAN_POINT('Ctrl Pts',(-64.3917733493027,-1.64891102645745,
0.741401300678363));
#31972=CARTESIAN_POINT('Ctrl Pts',(-65.0102911364986,-1.75748152866257,
0.704355337155683));
#31973=CARTESIAN_POINT('Ctrl Pts',(-65.5328829338629,-1.58138226671975,
0.667309373633002));
#31974=CARTESIAN_POINT('Ctrl Pts',(-66.0554747312272,-1.40528300477693,
0.630263410110321));
#31975=CARTESIAN_POINT('Ctrl Pts',(-66.4821405387599,-0.944513978686166,
0.593217446587641));
#31976=CARTESIAN_POINT('Ctrl Pts',(-66.6176143302611,-0.409948745265357,
0.55617148306496));
#31977=CARTESIAN_POINT('Ctrl Pts',(-66.6513211107492,-0.276945359297945,
0.546954200913236));
#31978=CARTESIAN_POINT('Ctrl Pts',(-66.6670017222694,-0.139373637561401,
0.537736918761512));
#31979=CARTESIAN_POINT('Ctrl Pts',(-66.6657538157597,-0.00152189319960278,
0.528519636609788));
#31980=CARTESIAN_POINT('Origin',(-65.,8.88178419700125E-15,3.));
#31981=CARTESIAN_POINT('',(-66.6633878829795,0.000426123154294022,-0.171480363390211));
#31982=CARTESIAN_POINT('',(-66.6664305869533,0.00149161834302873,0.0214803633902054));
#31983=CARTESIAN_POINT('',(-66.666,8.90896198514149E-15,3.));
#31984=CARTESIAN_POINT('Ctrl Pts',(-66.6664305869533,0.00149161834302873,
0.0214803633902054));
#31985=CARTESIAN_POINT('Ctrl Pts',(-66.6623874613811,-0.43660857926759,
0.0508038371872736));
#31986=CARTESIAN_POINT('Ctrl Pts',(-66.484951449296,-0.877606426402566,
0.0801273109843417));
#31987=CARTESIAN_POINT('Ctrl Pts',(-66.1749931684956,-1.18495810418995,
0.10945078478141));
#31988=CARTESIAN_POINT('Ctrl Pts',(-65.7834057582335,-1.57325244894403,
0.146496748304091));
#31989=CARTESIAN_POINT('Ctrl Pts',(-65.1803040079573,-1.74823863365067,
0.183542711826771));
#31990=CARTESIAN_POINT('Ctrl Pts',(-64.641700851863,-1.62983323643182,0.220588675349452));
#31991=CARTESIAN_POINT('Ctrl Pts',(-64.1030976957686,-1.51142783921296,
0.257634638872132));
#31992=CARTESIAN_POINT('Ctrl Pts',(-63.6289931338561,-1.09963086006863,
0.294680602394813));
#31993=CARTESIAN_POINT('Ctrl Pts',(-63.4363638080708,-0.582903522671596,
0.331726565917493));
#31994=CARTESIAN_POINT('Ctrl Pts',(-63.2437344822855,-0.0661761852745638,
0.368772529440174));
#31995=CARTESIAN_POINT('Ctrl Pts',(-63.3325803926274,0.555481510375165,
0.405818492962854));
#31996=CARTESIAN_POINT('Ctrl Pts',(-63.6622407040169,0.997564395392442,
0.442864456485535));
#31997=CARTESIAN_POINT('Ctrl Pts',(-63.9919010154063,1.43964728040972,0.479910420008216));
#31998=CARTESIAN_POINT('Ctrl Pts',(-64.5623757278433,1.70215535479454,0.516956383530896));
#31999=CARTESIAN_POINT('Ctrl Pts',(-65.1125838545831,1.66495030949471,0.554002347053577));
#32000=CARTESIAN_POINT('Ctrl Pts',(-65.6627919813228,1.62774526419488,0.591048310576258));
#32001=CARTESIAN_POINT('Ctrl Pts',(-66.1927335223652,1.29082709921039,0.628094274098938));
#32002=CARTESIAN_POINT('Ctrl Pts',(-66.4598777263709,0.808388323348361,
0.665140237621619));
#32003=CARTESIAN_POINT('Ctrl Pts',(-66.5953035291742,0.563821315923753,
0.683920279544481));
#32004=CARTESIAN_POINT('Ctrl Pts',(-66.6631938061757,0.281857388570598,
0.702700321467343));
#32005=CARTESIAN_POINT('Ctrl Pts',(-66.6632893889008,-6.33249066055908E-5,
0.721480363390205));
#32006=CARTESIAN_POINT('Ctrl Pts',(-66.6657538157597,-0.00152189319960278,
0.528519636609788));
#32007=CARTESIAN_POINT('Ctrl Pts',(-66.6619861549602,0.414678045906911,
0.500690955238832));
#32008=CARTESIAN_POINT('Ctrl Pts',(-66.5039069443419,0.833430525360491,
0.472862273867875));
#32009=CARTESIAN_POINT('Ctrl Pts',(-66.2217249851539,1.13671551258267,0.445033592496918));
#32010=CARTESIAN_POINT('Ctrl Pts',(-65.8460800730759,1.54045309625903,0.407987628974238));
#32011=CARTESIAN_POINT('Ctrl Pts',(-65.2505084734505,1.7395668228609,0.370941665451557));
#32012=CARTESIAN_POINT('Ctrl Pts',(-64.7075769058774,1.64293116911908,0.333895701928877));
#32013=CARTESIAN_POINT('Ctrl Pts',(-64.1646453383043,1.54629551537725,0.296849738406196));
#32014=CARTESIAN_POINT('Ctrl Pts',(-63.6743538027836,1.15391048129173,0.259803774883516));
#32015=CARTESIAN_POINT('Ctrl Pts',(-63.4610870008646,0.645353297241691,
0.222757811360835));
#32016=CARTESIAN_POINT('Ctrl Pts',(-63.2478201989456,0.136796113191647,
0.185711847838155));
#32017=CARTESIAN_POINT('Ctrl Pts',(-63.3115781306282,-0.487933220822921,
0.148665884315474));
#32018=CARTESIAN_POINT('Ctrl Pts',(-63.6231816165986,-0.942923771900624,
0.111619920792793));
#32019=CARTESIAN_POINT('Ctrl Pts',(-63.9347851025691,-1.39791432297833,
0.0745739572701125));
#32020=CARTESIAN_POINT('Ctrl Pts',(-64.4942341428273,-1.68316609111917,
0.0375279937474321));
#32021=CARTESIAN_POINT('Ctrl Pts',(-65.0454937124919,-1.66813200830569,
0.000482030224751638));
#32022=CARTESIAN_POINT('Ctrl Pts',(-65.5967532821565,-1.65309792549221,
-0.0365639332979289));
#32023=CARTESIAN_POINT('Ctrl Pts',(-66.1398233812275,-1.33777799172442,
-0.0736098968206095));
#32024=CARTESIAN_POINT('Ctrl Pts',(-66.4261648980985,-0.866480120962484,
-0.11065586034329));
#32025=CARTESIAN_POINT('Ctrl Pts',(-66.5828763524582,-0.608544158441976,
-0.130930694692264));
#32026=CARTESIAN_POINT('Ctrl Pts',(-66.6626912202299,-0.303888929858138,
-0.151205529041237));
#32027=CARTESIAN_POINT('Ctrl Pts',(-66.6633878829795,0.000426123154294022,
-0.171480363390211));
#32028=CARTESIAN_POINT('Origin',(-65.,8.88178419700125E-15,3.));
#32029=CARTESIAN_POINT('',(-66.6673159824367,0.00130059074132209,-0.871480363390211));
#32030=CARTESIAN_POINT('',(-66.6681941903091,-0.000864019930029195,-0.678519636609795));
#32031=CARTESIAN_POINT('',(-66.666,8.90896198514149E-15,3.));
#32032=CARTESIAN_POINT('Ctrl Pts',(-66.6681941903091,-0.000864019930029195,
-0.678519636609795));
#32033=CARTESIAN_POINT('Ctrl Pts',(-66.6685078326159,-0.0505538571114753,
-0.675184574138157));
#32034=CARTESIAN_POINT('Ctrl Pts',(-66.6664801000417,-0.100217739688416,
-0.67184951166652));
#32035=CARTESIAN_POINT('Ctrl Pts',(-66.6620276056557,-0.149663274321054,
-0.668514449194882));
#32036=CARTESIAN_POINT('Ctrl Pts',(-66.6125691784105,-0.698905601245364,
-0.631468485672201));
#32037=CARTESIAN_POINT('Ctrl Pts',(-66.2639236084022,-1.22120635507833,
-0.594422522149521));
#32038=CARTESIAN_POINT('Ctrl Pts',(-65.7756507075141,-1.47753189011201,
-0.557376558626841));
#32039=CARTESIAN_POINT('Ctrl Pts',(-65.287377806626,-1.73385742514569,-0.52033059510416));
#32040=CARTESIAN_POINT('Ctrl Pts',(-64.659477574858,-1.72420774138009,-0.483284631581479));
#32041=CARTESIAN_POINT('Ctrl Pts',(-64.1793120174543,-1.45299894151709,
-0.446238668058799));
#32042=CARTESIAN_POINT('Ctrl Pts',(-63.6991464600505,-1.18179014165408,
-0.409192704536118));
#32043=CARTESIAN_POINT('Ctrl Pts',(-63.3667155770108,-0.649022225693665,
-0.372146741013438));
#32044=CARTESIAN_POINT('Ctrl Pts',(-63.334158295787,-0.098519517195975,
-0.335100777490757));
#32045=CARTESIAN_POINT('Ctrl Pts',(-63.3016010145631,0.451983191301712,
-0.298054813968077));
#32046=CARTESIAN_POINT('Ctrl Pts',(-63.568917335155,1.02022069233667,-0.261008850445396));
#32047=CARTESIAN_POINT('Ctrl Pts',(-64.0137684029003,1.34613590481466,-0.223962886922715));
#32048=CARTESIAN_POINT('Ctrl Pts',(-64.4586194706456,1.67205111729264,-0.186916923400034));
#32049=CARTESIAN_POINT('Ctrl Pts',(-65.0810052855443,1.75564404121365,-0.149870959877354));
#32050=CARTESIAN_POINT('Ctrl Pts',(-65.5960874627954,1.55865788401291,-0.112824996354674));
#32051=CARTESIAN_POINT('Ctrl Pts',(-66.1111696400466,1.36167172681217,-0.0757790328319931));
#32052=CARTESIAN_POINT('Ctrl Pts',(-66.5189481796502,0.884106488489685,
-0.0387330693093125));
#32053=CARTESIAN_POINT('Ctrl Pts',(-66.632800914328,0.344522616927675,-0.00168710578663189));
#32054=CARTESIAN_POINT('Ctrl Pts',(-66.6565343117127,0.232042591898964,
0.00603538393898058));
#32055=CARTESIAN_POINT('Ctrl Pts',(-66.6674953651548,0.116867589766136,
0.013757873664593));
#32056=CARTESIAN_POINT('Ctrl Pts',(-66.6664305869533,0.00149161834302873,
0.0214803633902054));
#32057=CARTESIAN_POINT('Ctrl Pts',(-66.6633878829795,0.000426123154294022,
-0.171480363390211));
#32058=CARTESIAN_POINT('Ctrl Pts',(-66.6639641550595,0.252152325979392,
-0.188251492563918));
#32059=CARTESIAN_POINT('Ctrl Pts',(-66.6104043971,0.503645766257019,-0.205022621737625));
#32060=CARTESIAN_POINT('Ctrl Pts',(-66.5014511773033,0.728270889754936,
-0.221793750911332));
#32061=CARTESIAN_POINT('Ctrl Pts',(-66.2607830049661,1.22444822195433,-0.258839714434013));
#32062=CARTESIAN_POINT('Ctrl Pts',(-65.7498337256207,1.58952707859705,-0.295885677956694));
#32063=CARTESIAN_POINT('Ctrl Pts',(-65.2024421689935,1.65642721292162,-0.332931641479375));
#32064=CARTESIAN_POINT('Ctrl Pts',(-64.6550506123664,1.72332734724618,-0.369977605002055));
#32065=CARTESIAN_POINT('Ctrl Pts',(-64.0712167784575,1.4920487592526,-0.407023568524736));
#32066=CARTESIAN_POINT('Ctrl Pts',(-63.7181355422591,1.06843708657373,-0.444069532047416));
#32067=CARTESIAN_POINT('Ctrl Pts',(-63.3650543060608,0.644825413894857,
-0.481115495570097));
#32068=CARTESIAN_POINT('Ctrl Pts',(-63.242725667573,0.0288806565306957,
-0.518161459092778));
#32069=CARTESIAN_POINT('Ctrl Pts',(-63.4071340014642,-0.497505944605285,
-0.555207422615458));
#32070=CARTESIAN_POINT('Ctrl Pts',(-63.5715423353554,-1.02389254574127,
-0.592253386138139));
#32071=CARTESIAN_POINT('Ctrl Pts',(-64.0226876416257,-1.46072099064906,
-0.629299349660819));
#32072=CARTESIAN_POINT('Ctrl Pts',(-64.5541007528815,-1.6080755066333,-0.6663453131835));
#32073=CARTESIAN_POINT('Ctrl Pts',(-65.0855138641373,-1.75543002261753,
-0.70339127670618));
#32074=CARTESIAN_POINT('Ctrl Pts',(-65.6971947803788,-1.6133106096782,-0.740437240228861));
#32075=CARTESIAN_POINT('Ctrl Pts',(-66.1092041825925,-1.24675657433953,
-0.777483203751541));
#32076=CARTESIAN_POINT('Ctrl Pts',(-66.4576696191289,-0.936735950411702,
-0.808815590297765));
#32077=CARTESIAN_POINT('Ctrl Pts',(-66.6633044515624,-0.466170980160872,
-0.840147976843988));
#32078=CARTESIAN_POINT('Ctrl Pts',(-66.6673159824367,0.00130059074132209,
-0.871480363390211));
#32079=CARTESIAN_POINT('Origin',(-65.,8.88178419700125E-15,3.));
#32080=CARTESIAN_POINT('',(-66.6674675207825,-0.00121113675535883,-1.57148036339021));
#32081=CARTESIAN_POINT('',(-66.6638321395092,-0.000941642735140673,-1.3785196366098));
#32082=CARTESIAN_POINT('',(-66.666,8.90896198514149E-15,3.));
#32083=CARTESIAN_POINT('',(-63.7309291201476,-1.0793586530485,-2.));
#32084=CARTESIAN_POINT('Ctrl Pts',(-66.6674675207825,-0.00121113675535883,
-1.57148036339021));
#32085=CARTESIAN_POINT('Ctrl Pts',(-66.6635269376583,0.471550204230273,
-1.6031823516921));
#32086=CARTESIAN_POINT('Ctrl Pts',(-66.452430524463,0.947291842680182,-1.63488433999399));
#32087=CARTESIAN_POINT('Ctrl Pts',(-66.0967466510819,1.25757678610754,-1.66658632829587));
#32088=CARTESIAN_POINT('Ctrl Pts',(-65.6811054719418,1.62016617912559,-1.70363229181856));
#32089=CARTESIAN_POINT('Ctrl Pts',(-65.0680223500032,1.75681556827132,-1.74067825534124));
#32090=CARTESIAN_POINT('Ctrl Pts',(-64.5381019768621,1.60385217794779,-1.77772421886392));
#32091=CARTESIAN_POINT('Ctrl Pts',(-64.008181603721,1.45088878762426,-1.8147701823866));
#32092=CARTESIAN_POINT('Ctrl Pts',(-63.5614239793774,1.00831261783146,-1.85181614590928));
#32093=CARTESIAN_POINT('Ctrl Pts',(-63.4023827506955,0.481249822665519,
-1.88886210943196));
#32094=CARTESIAN_POINT('Ctrl Pts',(-63.2433415220136,-0.0458129725004199,
-1.92590807295464));
#32095=CARTESIAN_POINT('Ctrl Pts',(-63.3720166889934,-0.6573623930395,-1.96295403647732));
#32096=CARTESIAN_POINT('Ctrl Pts',(-63.7309291201476,-1.0793586530485,-2.));
#32097=CARTESIAN_POINT('',(-66.2714644419457,-1.08121564890976,-2.));
#32098=CARTESIAN_POINT('Origin',(-65.,8.88178419700125E-15,-2.));
#32099=CARTESIAN_POINT('Ctrl Pts',(-66.2714656498818,-1.08121658606209,
-2.));
#32100=CARTESIAN_POINT('Ctrl Pts',(-65.9206041791687,-1.49275399655514,
-1.96367708181445));
#32101=CARTESIAN_POINT('Ctrl Pts',(-65.350635463119,-1.71875942899392,-1.92735416362889));
#32102=CARTESIAN_POINT('Ctrl Pts',(-64.8132380266976,-1.65815373977101,
-1.89103124544334));
#32103=CARTESIAN_POINT('Ctrl Pts',(-64.2651431372632,-1.59634163148307,
-1.85398528192066));
#32104=CARTESIAN_POINT('Ctrl Pts',(-63.7509291640016,-1.23639424886418,
-1.81693931839798));
#32105=CARTESIAN_POINT('Ctrl Pts',(-63.5055956276972,-0.742592085292541,
-1.7798933548753));
#32106=CARTESIAN_POINT('Ctrl Pts',(-63.2602620913927,-0.248789921720896,
-1.74284739135262));
#32107=CARTESIAN_POINT('Ctrl Pts',(-63.2838089920452,0.378867022803503,
-1.70580142782994));
#32108=CARTESIAN_POINT('Ctrl Pts',(-63.5656287203753,0.852900276652188,
-1.66875546430726));
#32109=CARTESIAN_POINT('Ctrl Pts',(-63.8474484487053,1.32693353050087,-1.63170950078458));
#32110=CARTESIAN_POINT('Ctrl Pts',(-64.387541004713,1.64734309367384,-1.5946635372619));
#32111=CARTESIAN_POINT('Ctrl Pts',(-64.9386444101885,1.66760708582443,-1.55761757373922));
#32112=CARTESIAN_POINT('Ctrl Pts',(-65.4897478156641,1.68787107797503,-1.52057161021654));
#32113=CARTESIAN_POINT('Ctrl Pts',(-66.0518620706076,1.40798949910324,-1.48352564669385));
#32114=CARTESIAN_POINT('Ctrl Pts',(-66.3677757854406,0.955993240532992,
-1.44647968317117));
#32115=CARTESIAN_POINT('Ctrl Pts',(-66.5609548232979,0.67960067431637,-1.42382633431738));
#32116=CARTESIAN_POINT('Ctrl Pts',(-66.6620736349107,0.338850343710045,
-1.40117298546359));
#32117=CARTESIAN_POINT('Ctrl Pts',(-66.6638321395092,-0.000941642735140673,
-1.3785196366098));
#32118=CARTESIAN_POINT('Origin',(-65.,8.88178419700125E-15,-3.54592528053767));
#32119=CARTESIAN_POINT('',(-67.0572086816557,-0.00119446450308647,6.54592528053768));
#32120=CARTESIAN_POINT('',(-67.0515888779951,0.000804696401313844,6.60407471946233));
#32121=CARTESIAN_POINT('',(-67.05475,-9.40612120991423E-14,-3.54592528053767));
#32122=CARTESIAN_POINT('',(-63.1173724903363,0.823232180103149,7.));
#32123=CARTESIAN_POINT('Ctrl Pts',(-67.0515888779951,0.000804696401313851,
6.60407471946233));
#32124=CARTESIAN_POINT('Ctrl Pts',(-67.0504040800969,-0.384787351067738,
6.62491192240684));
#32125=CARTESIAN_POINT('Ctrl Pts',(-66.7605424545076,-1.45760454425863,
6.68279508887404));
#32126=CARTESIAN_POINT('Ctrl Pts',(-65.029841359516,-2.42994159679626,6.77772421886392));
#32127=CARTESIAN_POINT('Ctrl Pts',(-62.9747815436376,-1.33872801408515,
6.88886210943195));
#32128=CARTESIAN_POINT('Ctrl Pts',(-62.8436282049399,0.19721374355959,6.96295403647732));
#32129=CARTESIAN_POINT('Ctrl Pts',(-63.1173724903363,0.823232180103149,
7.));
#32130=CARTESIAN_POINT('',(-63.7764000215903,1.65534094402446,7.));
#32131=CARTESIAN_POINT('Origin',(-65.,8.88178419700125E-15,7.));
#32132=CARTESIAN_POINT('Ctrl Pts',(-67.0572086816557,-0.00119446450308609,
6.54592528053768));
#32133=CARTESIAN_POINT('Ctrl Pts',(-67.0577114364342,-0.0728343130723733,
6.54982271160486));
#32134=CARTESIAN_POINT('Ctrl Pts',(-67.0218209037147,-0.824923083408348,
6.59076610619472));
#32135=CARTESIAN_POINT('Ctrl Pts',(-66.0963109962835,-2.16731896239628,
6.66875546430726));
#32136=CARTESIAN_POINT('Ctrl Pts',(-63.7734206371606,-2.09605634078855,
6.77989335487529));
#32137=CARTESIAN_POINT('Ctrl Pts',(-62.5820931272045,-0.120092092488803,
6.89030820010622));
#32138=CARTESIAN_POINT('Ctrl Pts',(-63.2405356955179,1.25818726815372,6.96367708181444));
#32139=CARTESIAN_POINT('Ctrl Pts',(-63.7763989699203,1.65534250909263,7.));
#32140=CARTESIAN_POINT('Origin',(-65.,8.88178419700125E-15,-3.54592528053767));
#32141=CARTESIAN_POINT('',(-67.0519117333221,-0.00102649957300818,5.84592528053768));
#32142=CARTESIAN_POINT('',(-67.0566574869574,0.00149765431884231,5.90407471946233));
#32143=CARTESIAN_POINT('',(-67.05475,-9.40612120991423E-14,-3.54592528053767));
#32144=CARTESIAN_POINT('Ctrl Pts',(-67.0566574869574,0.00149765431884247,
5.90407471946233));
#32145=CARTESIAN_POINT('Ctrl Pts',(-67.0518463029865,-0.585190437662465,
5.93596947460409));
#32146=CARTESIAN_POINT('Ctrl Pts',(-66.4813711624858,-1.8614882619805,6.00491019326854));
#32147=CARTESIAN_POINT('Ctrl Pts',(-64.3156972041947,-2.33026144716284,
6.11089687545566));
#32148=CARTESIAN_POINT('Ctrl Pts',(-62.6710926659578,-0.688814355154873,
6.22203476602371));
#32149=CARTESIAN_POINT('Ctrl Pts',(-63.1582101680956,1.58293676398102,6.33317265659174));
#32150=CARTESIAN_POINT('Ctrl Pts',(-65.3310466291073,2.40615402668531,6.4443105471598));
#32151=CARTESIAN_POINT('Ctrl Pts',(-66.8504470921567,1.28501547118087,6.53461123478332));
#32152=CARTESIAN_POINT('Ctrl Pts',(-67.0525105038734,0.300747505180014,
6.58786595888416));
#32153=CARTESIAN_POINT('Ctrl Pts',(-67.0515888779951,0.000804696401313851,
6.60407471946233));
#32154=CARTESIAN_POINT('Ctrl Pts',(-67.0519117333221,-0.00102649957300794,
5.84592528053768));
#32155=CARTESIAN_POINT('Ctrl Pts',(-67.0531633450758,-0.277741730134872,
5.86088026380211));
#32156=CARTESIAN_POINT('Ctrl Pts',(-66.8721481216246,-1.2383569525156,5.91288121058921));
#32157=CARTESIAN_POINT('Ctrl Pts',(-65.4121253417219,-2.39341760299656,
6.00192812089901));
#32158=CARTESIAN_POINT('Ctrl Pts',(-63.2126643336617,-1.64429852840487,
6.11306601146705));
#32159=CARTESIAN_POINT('Ctrl Pts',(-62.649189925264,0.60985028512182,6.22420390203509));
#32160=CARTESIAN_POINT('Ctrl Pts',(-64.2374031554986,2.30582648807955,6.33534179260313));
#32161=CARTESIAN_POINT('Ctrl Pts',(-66.4435230617628,1.90573437919649,6.44258225210399));
#32162=CARTESIAN_POINT('Ctrl Pts',(-67.0529326385893,0.608118645715832,
6.51277674808218));
#32163=CARTESIAN_POINT('Ctrl Pts',(-67.0572086816557,-0.00119446450308609,
6.54592528053768));
#32164=CARTESIAN_POINT('Origin',(-65.,8.88178419700125E-15,-3.54592528053767));
#32165=CARTESIAN_POINT('',(-67.0534842785189,0.00176526399348016,5.14592528053768));
#32166=CARTESIAN_POINT('',(-67.0562728194261,-0.00163389830065408,5.20407471946232));
#32167=CARTESIAN_POINT('',(-67.05475,-9.40612120991423E-14,-3.54592528053767));
#32168=CARTESIAN_POINT('Ctrl Pts',(-67.0562728194261,-0.00163389830065397,
5.20407471946232));
#32169=CARTESIAN_POINT('Ctrl Pts',(-67.0572175303294,-0.110331419494764,
5.20998106327866));
#32170=CARTESIAN_POINT('Ctrl Pts',(-66.9999469228229,-0.899807785912462,
5.25293337061767));
#32171=CARTESIAN_POINT('Ctrl Pts',(-65.9773779060574,-2.22328871643558,
5.33293164147938));
#32172=CARTESIAN_POINT('Ctrl Pts',(-63.6621652804381,-2.0269388363574,5.44406953204741));
#32173=CARTESIAN_POINT('Ctrl Pts',(-62.5714875417724,0.0246926647779575,
5.55520742261546));
#32174=CARTESIAN_POINT('Ctrl Pts',(-63.7036555936518,2.05371969901984,5.66634531318349));
#32175=CARTESIAN_POINT('Ctrl Pts',(-66.0223808123334,2.20295969802022,5.77748320375154));
#32176=CARTESIAN_POINT('Ctrl Pts',(-67.0084336557534,0.871640043874873,
5.85672633917782));
#32177=CARTESIAN_POINT('Ctrl Pts',(-67.0574345241562,0.0962515598736501,
5.89892351108141));
#32178=CARTESIAN_POINT('Ctrl Pts',(-67.0566574869574,0.00149765431884247,
5.90407471946233));
#32179=CARTESIAN_POINT('Ctrl Pts',(-67.0534842785189,0.00176526399348016,
5.14592528053768));
#32180=CARTESIAN_POINT('Ctrl Pts',(-67.049548506192,-0.478623619806704,
5.17193781599936));
#32181=CARTESIAN_POINT('Ctrl Pts',(-66.6418658995519,-1.6491803337807,5.23499631498372));
#32182=CARTESIAN_POINT('Ctrl Pts',(-64.6918158067504,-2.40900502421389,
5.33510077749075));
#32183=CARTESIAN_POINT('Ctrl Pts',(-62.80891719594,-1.04758718972751,5.4462386680588));
#32184=CARTESIAN_POINT('Ctrl Pts',(-62.9315418303621,1.27269881881277,5.55737655862684));
#32185=CARTESIAN_POINT('Ctrl Pts',(-64.947449081762,2.42806968006159,5.66851444919488));
#32186=CARTESIAN_POINT('Ctrl Pts',(-66.7337199477999,1.50458731301856,5.7646973564985));
#32187=CARTESIAN_POINT('Ctrl Pts',(-67.0500628960447,0.407727598470006,
5.82383430027943));
#32188=CARTESIAN_POINT('Ctrl Pts',(-67.0519117333221,-0.00102649957300794,
5.84592528053768));
#32189=CARTESIAN_POINT('Origin',(-65.,8.88178419700125E-15,-3.54592528053767));
#32190=CARTESIAN_POINT('',(-67.0581446603105,-8.27717200928135E-6,4.44592528053768));
#32191=CARTESIAN_POINT('',(-67.051502599911,-0.00046897283331893,4.50407471946232));
#32192=CARTESIAN_POINT('',(-67.05475,-9.40612120991423E-14,-3.54592528053767));
#32193=CARTESIAN_POINT('Ctrl Pts',(-67.051502599911,-0.00046897283331862,
4.50407471946232));
#32194=CARTESIAN_POINT('Ctrl Pts',(-67.0521436877867,-0.314512114650342,
4.52103861547591));
#32195=CARTESIAN_POINT('Ctrl Pts',(-66.8367516776872,-1.31353269400002,
4.57504847501217));
#32196=CARTESIAN_POINT('Ctrl Pts',(-65.2821091229946,-2.41219729396228,
4.66610429807113));
#32197=CARTESIAN_POINT('Ctrl Pts',(-63.1263775009061,-1.5452572946423,4.77724218863916));
#32198=CARTESIAN_POINT('Ctrl Pts',(-62.6855937936814,0.736074256717683,
4.88838007920721));
#32199=CARTESIAN_POINT('Ctrl Pts',(-64.3632123478174,2.34366864230481,4.99951796977525));
#32200=CARTESIAN_POINT('Ctrl Pts',(-66.5035583733625,1.83464658396607,5.10474951652696));
#32201=CARTESIAN_POINT('Ctrl Pts',(-67.0512920835974,0.571444740237986,
5.17293509975598));
#32202=CARTESIAN_POINT('Ctrl Pts',(-67.0562728194261,-0.00163389830065397,
5.20407471946232));
#32203=CARTESIAN_POINT('Ctrl Pts',(-67.0581446431809,-8.27713024233776E-6,
4.44592528053768));
#32204=CARTESIAN_POINT('Ctrl Pts',(-67.0581446696346,-0.00045118411400466,
4.44594940467392));
#32205=CARTESIAN_POINT('Ctrl Pts',(-67.0579439709526,-0.681039286739854,
4.48301949233285));
#32206=CARTESIAN_POINT('Ctrl Pts',(-66.315832277707,-2.04129075981347,4.55713554351446));
#32207=CARTESIAN_POINT('Ctrl Pts',(-63.9986308592856,-2.21258726309084,
4.66827343408251));
#32208=CARTESIAN_POINT('Ctrl Pts',(-62.5979939690176,-0.358677549762027,
4.77941132465054));
#32209=CARTESIAN_POINT('Ctrl Pts',(-63.3959404447163,1.82353378810158,4.89054921521859));
#32210=CARTESIAN_POINT('Ctrl Pts',(-65.6621008123707,2.33664397819608,5.00168710578663));
#32211=CARTESIAN_POINT('Ctrl Pts',(-66.9336682838985,1.0914904129242,5.08681246089299));
#32212=CARTESIAN_POINT('Ctrl Pts',(-67.0551536682982,0.205526108395703,
5.13489185247667));
#32213=CARTESIAN_POINT('Ctrl Pts',(-67.0534842785189,0.00176526399348016,
5.14592528053768));
#32214=CARTESIAN_POINT('Origin',(-65.,8.88178419700125E-15,-3.54592528053767));
#32215=CARTESIAN_POINT('',(-67.0534601308484,-0.00176006036929743,3.74592528053768));
#32216=CARTESIAN_POINT('',(-67.0545529589347,0.00187890219046263,3.80407471946232));
#32217=CARTESIAN_POINT('',(-67.05475,-9.40612120991423E-14,-3.54592528053767));
#32218=CARTESIAN_POINT('Ctrl Pts',(-67.0545529589347,0.00187890219046255,
3.80407471946232));
#32219=CARTESIAN_POINT('Ctrl Pts',(-67.049847975054,-0.514925815373994,
3.83209616767316));
#32220=CARTESIAN_POINT('Ctrl Pts',(-66.5901947888396,-1.72243254492318,
3.89716357940667));
#32221=CARTESIAN_POINT('Ctrl Pts',(-64.5620129419189,-2.3888174265201,3.99927695466288));
#32222=CARTESIAN_POINT('Ctrl Pts',(-62.7554801641395,-0.927583994626942,
4.11041484523091));
#32223=CARTESIAN_POINT('Ctrl Pts',(-63.0033818465923,1.3826775875065,4.22155273579896));
#32224=CARTESIAN_POINT('Ctrl Pts',(-65.0788107682801,2.42735869229697,4.33269062636699));
#32225=CARTESIAN_POINT('Ctrl Pts',(-66.7763241812549,1.4299225698547,4.42686462092146));
#32226=CARTESIAN_POINT('Ctrl Pts',(-67.0507436722455,0.371299138082145,
4.48399265195323));
#32227=CARTESIAN_POINT('Ctrl Pts',(-67.051502599911,-0.00046897283331862,
4.50407471946232));
#32228=CARTESIAN_POINT('Ctrl Pts',(-67.0534601308484,-0.0017600603692971,
3.74592528053768));
#32229=CARTESIAN_POINT('Ctrl Pts',(-67.055130441991,-0.206418025502587,
3.75700695687117));
#32230=CARTESIAN_POINT('Ctrl Pts',(-66.9329701809384,-1.09329696547216,
3.80513459672735));
#32231=CARTESIAN_POINT('Ctrl Pts',(-65.6590644304509,-2.3375022198779,3.89030820010621));
#32232=CARTESIAN_POINT('Ctrl Pts',(-63.39357261301,-1.82144821550898,4.00144609067426));
#32233=CARTESIAN_POINT('Ctrl Pts',(-62.5984620009619,0.361797997181342,
4.1125839812423));
#32234=CARTESIAN_POINT('Ctrl Pts',(-64.0015063548152,2.21388639990767,4.22372187181034));
#32235=CARTESIAN_POINT('Ctrl Pts',(-66.3179803312342,2.03961730968541,4.33483563824213));
#32236=CARTESIAN_POINT('Ctrl Pts',(-67.0581040462783,0.679694036228928,
4.40890344115124));
#32237=CARTESIAN_POINT('Ctrl Pts',(-67.0581446431809,-8.27713024233776E-6,
4.44592528053768));
#32238=CARTESIAN_POINT('Origin',(-65.,8.88178419700125E-15,-3.54592528053767));
#32239=CARTESIAN_POINT('',(-67.0519256006226,0.00103910123989234,3.04592528053768));
#32240=CARTESIAN_POINT('',(-67.0578709601416,-0.000678769155100989,3.10407471946232));
#32241=CARTESIAN_POINT('',(-67.05475,-9.40612120991423E-14,-3.54592528053767));
#32242=CARTESIAN_POINT('Ctrl Pts',(-67.0578709601415,-0.000678769155101162,
3.10407471946232));
#32243=CARTESIAN_POINT('Ctrl Pts',(-67.0580316799421,-0.0380175835266657,
3.10610775634773));
#32244=CARTESIAN_POINT('Ctrl Pts',(-67.0401889053665,-0.755586934309652,
3.14518675675581));
#32245=CARTESIAN_POINT('Ctrl Pts',(-66.2035357618251,-2.1094508836634,3.22131172068658));
#32246=CARTESIAN_POINT('Ctrl Pts',(-63.8804623217255,-2.15520689204011,
3.33244961125462));
#32247=CARTESIAN_POINT('Ctrl Pts',(-62.5821144149725,-0.228277590427775,
3.44358750182266));
#32248=CARTESIAN_POINT('Ctrl Pts',(-63.4968846048806,1.90759677855457,3.55472539239071));
#32249=CARTESIAN_POINT('Ctrl Pts',(-65.7874733624335,2.29742618249228,3.66586328295874));
#32250=CARTESIAN_POINT('Ctrl Pts',(-66.9614802130625,1.01630569367124,3.74897972531595));
#32251=CARTESIAN_POINT('Ctrl Pts',(-67.0560682339038,0.168319696106685,
3.79505020415048));
#32252=CARTESIAN_POINT('Ctrl Pts',(-67.0545529589347,0.00187890219046255,
3.80407471946232));
#32253=CARTESIAN_POINT('Ctrl Pts',(-67.0519256006226,0.00103910123989245,
3.04592528053768));
#32254=CARTESIAN_POINT('Ctrl Pts',(-67.0500496331103,-0.408601099978636,
3.06806450906842));
#32255=CARTESIAN_POINT('Ctrl Pts',(-66.7326598083642,-1.50637690262577,
3.12724970112185));
#32256=CARTESIAN_POINT('Ctrl Pts',(-64.9442948490232,-2.42799907075925,
3.22348085669796));
#32257=CARTESIAN_POINT('Ctrl Pts',(-62.9298898830714,-1.27001049414664,
3.334618747266));
#32258=CARTESIAN_POINT('Ctrl Pts',(-62.8102801837888,1.05043309065765,3.44575663783405));
#32259=CARTESIAN_POINT('Ctrl Pts',(-64.6949458653977,2.40940335486023,3.55689452840209));
#32260=CARTESIAN_POINT('Ctrl Pts',(-66.643067780423,1.64741324066797,3.65695074263663));
#32261=CARTESIAN_POINT('Ctrl Pts',(-67.0495466039689,0.477752065987548,
3.71996099334849));
#32262=CARTESIAN_POINT('Ctrl Pts',(-67.0534601308484,-0.0017600603692971,
3.74592528053768));
#32263=CARTESIAN_POINT('Origin',(-65.,8.88178419700125E-15,-3.54592528053767));
#32264=CARTESIAN_POINT('',(-67.0572522603608,0.00120217803180264,2.34592528053767));
#32265=CARTESIAN_POINT('',(-67.0525490214284,-0.00145097609280704,2.40407471946232));
#32266=CARTESIAN_POINT('',(-67.05475,-9.40612120991423E-14,-3.54592528053767));
#32267=CARTESIAN_POINT('Ctrl Pts',(-67.0525490214284,-0.00145097609280675,
2.40407471946232));
#32268=CARTESIAN_POINT('Ctrl Pts',(-67.054127131265,-0.243480442393208,
2.41716530854498));
#32269=CARTESIAN_POINT('Ctrl Pts',(-66.9026176062656,-1.16853384943058,
2.46730186115031));
#32270=CARTESIAN_POINT('Ctrl Pts',(-65.5317127142361,-2.36971790517293,
2.55448437727833));
#32271=CARTESIAN_POINT('Ctrl Pts',(-63.2974379205056,-1.73192486154719,
2.66562226784637));
#32272=CARTESIAN_POINT('Ctrl Pts',(-62.6215375065036,0.491118649216447,
2.77676015841441));
#32273=CARTESIAN_POINT('Ctrl Pts',(-64.122670786398,2.26463569068811,2.88789804898245));
#32274=CARTESIAN_POINT('Ctrl Pts',(-66.3846835747723,1.97078161673767,2.99700290266509));
#32275=CARTESIAN_POINT('Ctrl Pts',(-67.0551030464715,0.642369656429121,
3.06906179282505));
#32276=CARTESIAN_POINT('Ctrl Pts',(-67.0578709601415,-0.000678769155101162,
3.10407471946232));
#32277=CARTESIAN_POINT('Ctrl Pts',(-67.0572522603608,0.00120217803180282,
2.34592528053767));
#32278=CARTESIAN_POINT('Ctrl Pts',(-67.0530108672503,-0.608976283722039,
2.37912206126567));
#32279=CARTESIAN_POINT('Ctrl Pts',(-66.4420019119215,-1.9074607758001,2.44936480551635));
#32280=CARTESIAN_POINT('Ctrl Pts',(-64.234427664365,-2.30481703186257,2.55665351328971));
#32281=CARTESIAN_POINT('Ctrl Pts',(-62.6483896081628,-0.606804018161647,
2.66779140385776));
#32282=CARTESIAN_POINT('Ctrl Pts',(-63.214807212685,1.64662359498827,2.77892929442579));
#32283=CARTESIAN_POINT('Ctrl Pts',(-65.4152320208998,2.39287795766376,2.89006718499384));
#32284=CARTESIAN_POINT('Ctrl Pts',(-66.8729657074861,1.23655088859839,2.97906584703113));
#32285=CARTESIAN_POINT('Ctrl Pts',(-67.0531887228005,0.276857109673468,
3.03101854554574));
#32286=CARTESIAN_POINT('Ctrl Pts',(-67.0519256006226,0.00103910123989245,
3.04592528053768));
#32287=CARTESIAN_POINT('Origin',(-65.,8.88178419700125E-15,-3.54592528053767));
#32288=CARTESIAN_POINT('',(-67.0555677501283,-0.00179912738464016,1.64592528053767));
#32289=CARTESIAN_POINT('',(-67.0526273462695,0.00148795516933967,1.70407471946232));
#32290=CARTESIAN_POINT('',(-67.05475,-9.40612120991423E-14,-3.54592528053767));
#32291=CARTESIAN_POINT('Ctrl Pts',(-67.0526273462695,0.00148795516933968,
1.70407471946232));
#32292=CARTESIAN_POINT('Ctrl Pts',(-67.049634688556,-0.444939705966109,
1.72822286074222));
#32293=CARTESIAN_POINT('Ctrl Pts',(-66.6869954305654,-1.58066428073723,
1.78941696554481));
#32294=CARTESIAN_POINT('Ctrl Pts',(-64.8130956691436,-2.42143513885566,
1.88765703387008));
#32295=CARTESIAN_POINT('Ctrl Pts',(-62.864249480632,-1.15622276382909,1.99879492443812));
#32296=CARTESIAN_POINT('Ctrl Pts',(-62.8702799635561,1.1672934193881,2.10993281500616));
#32297=CARTESIAN_POINT('Ctrl Pts',(-64.8256673485052,2.42237269783169,2.2210707055742));
#32298=CARTESIAN_POINT('Ctrl Pts',(-66.6915092429239,1.57355497286028,2.31911800705959));
#32299=CARTESIAN_POINT('Ctrl Pts',(-67.0496611290802,0.441455485498574,
2.3801193450223));
#32300=CARTESIAN_POINT('Ctrl Pts',(-67.0525490214284,-0.00145097609280675,
2.40407471946232));
#32301=CARTESIAN_POINT('Ctrl Pts',(-67.0555677501283,-0.00179912738464004,
1.64592528053767));
#32302=CARTESIAN_POINT('Ctrl Pts',(-67.0567846151392,-0.134576239702309,
1.65313364994024));
#32303=CARTESIAN_POINT('Ctrl Pts',(-66.9845642825309,-0.948416460674393,
1.69738798286549));
#32304=CARTESIAN_POINT('Ctrl Pts',(-65.898842928637,-2.25618349012117,1.77868827931342));
#32305=CARTESIAN_POINT('Ctrl Pts',(-63.5919355659201,-1.97879688218178,
1.88982616988146));
#32306=CARTESIAN_POINT('Ctrl Pts',(-62.5738455482538,0.109804953100741,
2.0009640604495));
#32307=CARTESIAN_POINT('Ctrl Pts',(-63.7764422147334,2.0979010695377,2.11210195101754));
#32308=CARTESIAN_POINT('Ctrl Pts',(-66.0989751981566,2.16576454521031,2.22323984158559));
#32309=CARTESIAN_POINT('Ctrl Pts',(-67.0223280499568,0.823134106038546,
2.30118095142563));
#32310=CARTESIAN_POINT('Ctrl Pts',(-67.0577440519451,0.0719526660358392,
2.34207609774299));
#32311=CARTESIAN_POINT('Ctrl Pts',(-67.0572522603608,0.00120217803180282,
2.34592528053767));
#32312=CARTESIAN_POINT('Origin',(-65.,8.88178419700125E-15,-3.54592528053767));
#32313=CARTESIAN_POINT('',(-67.0514068858608,-7.81013517094087E-5,0.945925280537675));
#32314=CARTESIAN_POINT('',(-67.0579182146741,0.000617375283499791,1.00407471946232));
#32315=CARTESIAN_POINT('',(-67.05475,-9.40612120991423E-14,-3.54592528053767));
#32316=CARTESIAN_POINT('Ctrl Pts',(-67.0579182146741,0.000617375283499685,
1.00407471946232));
#32317=CARTESIAN_POINT('Ctrl Pts',(-67.0553588641481,-0.645931829998605,
1.03928041293948));
#32318=CARTESIAN_POINT('Ctrl Pts',(-66.378434179731,-1.977444237299,1.11153206993931));
#32319=CARTESIAN_POINT('Ctrl Pts',(-64.1109273576576,-2.26005114925192,
1.22082969046183));
#32320=CARTESIAN_POINT('Ctrl Pts',(-62.6190202559434,-0.47876593338251,
1.33196758102987));
#32321=CARTESIAN_POINT('Ctrl Pts',(-63.3064509161112,1.74073917087914,1.44310547159791));
#32322=CARTESIAN_POINT('Ctrl Pts',(-65.5440062589152,2.36692597071417,1.55424336216595));
#32323=CARTESIAN_POINT('Ctrl Pts',(-66.9056402449312,1.161313621274,1.64123311145409));
#32324=CARTESIAN_POINT('Ctrl Pts',(-67.0542257619312,0.239930514819847,
1.69117689721954));
#32325=CARTESIAN_POINT('Ctrl Pts',(-67.0526273462695,0.00148795516933968,
1.70407471946232));
#32326=CARTESIAN_POINT('Ctrl Pts',(-67.0514068858608,-7.81013517092005E-5,
0.945925280537675));
#32327=CARTESIAN_POINT('Ctrl Pts',(-67.0515215449353,-0.338264400941531,
0.964191202137492));
#32328=CARTESIAN_POINT('Ctrl Pts',(-66.8123460743743,-1.36218935655874,
1.01950308725999));
#32329=CARTESIAN_POINT('Ctrl Pts',(-65.1973793755662,-2.42060404314487,
1.11186093590517));
#32330=CARTESIAN_POINT('Ctrl Pts',(-63.0733618200821,-1.47863040518406,
1.22299882647321));
#32331=CARTESIAN_POINT('Ctrl Pts',(-62.7128180402749,0.816750411403611,
1.33413671704125));
#32332=CARTESIAN_POINT('Ctrl Pts',(-64.4457578465939,2.36455031387797,1.4452746076093));
#32333=CARTESIAN_POINT('Ctrl Pts',(-66.5407002488233,1.78803648666642,1.54920412877477));
#32334=CARTESIAN_POINT('Ctrl Pts',(-67.0505307823665,0.547805001444303,
1.61608768641756));
#32335=CARTESIAN_POINT('Ctrl Pts',(-67.0555677501283,-0.00179912738464004,
1.64592528053767));
#32336=CARTESIAN_POINT('Origin',(-65.,8.88178419700125E-15,-3.54592528053767));
#32337=CARTESIAN_POINT('',(-67.05528106155,0.00183967754518982,0.245925280537674));
#32338=CARTESIAN_POINT('',(-67.0544463703074,-0.0018770168378236,0.304074719462319));
#32339=CARTESIAN_POINT('',(-67.05475,-9.40612120991423E-14,-3.54592528053767));
#32340=CARTESIAN_POINT('Ctrl Pts',(-67.0544463703074,-0.00187701683782321,
0.304074719462319));
#32341=CARTESIAN_POINT('Ctrl Pts',(-67.0559854674868,-0.171895547286461,
0.313292001614044));
#32342=CARTESIAN_POINT('Ctrl Pts',(-66.9589165461202,-1.02351658402418,
0.359555247288449));
#32343=CARTESIAN_POINT('Ctrl Pts',(-65.7755372964953,-2.30148283939099,
0.442864456485536));
#32344=CARTESIAN_POINT('Ctrl Pts',(-63.4870029209119,-1.89976872281361,
0.554002347053577));
#32345=CARTESIAN_POINT('Ctrl Pts',(-62.5833319303427,0.240825251495458,
0.665140237621619));
#32346=CARTESIAN_POINT('Ctrl Pts',(-63.8916646308255,2.16098914151126,0.77627812818966));
#32347=CARTESIAN_POINT('Ctrl Pts',(-66.2144692640843,2.10317516324911,0.887416018757702));
#32348=CARTESIAN_POINT('Ctrl Pts',(-67.0419827284221,0.748425825038287,
0.963348215848589));
#32349=CARTESIAN_POINT('Ctrl Pts',(-67.058051996902,0.0344137592749453,
1.0022344494168));
#32350=CARTESIAN_POINT('Ctrl Pts',(-67.0579182146741,0.000617375283499685,
1.00407471946232));
#32351=CARTESIAN_POINT('Ctrl Pts',(-67.05528106155,0.00183967754518984,
0.245925280537674));
#32352=CARTESIAN_POINT('Ctrl Pts',(-67.0502944995635,-0.538488282262975,
0.275248754334741));
#32353=CARTESIAN_POINT('Ctrl Pts',(-66.5549829233901,-1.76953115899707,
0.341618191654489));
#32354=CARTESIAN_POINT('Ctrl Pts',(-64.4785452214709,-2.37199651591817,
0.445033592496919));
#32355=CARTESIAN_POINT('Ctrl Pts',(-62.7243441135659,-0.848335334231208,
0.55617148306496));
#32356=CARTESIAN_POINT('Ctrl Pts',(-63.0530766482751,1.45181679686654,0.667309373633002));
#32357=CARTESIAN_POINT('Ctrl Pts',(-65.1638502053818,2.42310455048397,0.778447264201043));
#32358=CARTESIAN_POINT('Ctrl Pts',(-66.8023851755325,1.38138173267995,0.871319233169269));
#32359=CARTESIAN_POINT('Ctrl Pts',(-67.0512889995436,0.34762693227213,0.927145238614812));
#32360=CARTESIAN_POINT('Ctrl Pts',(-67.0514068858608,-7.81013517092005E-5,
0.945925280537675));
#32361=CARTESIAN_POINT('Origin',(-65.,8.88178419700125E-15,-3.54592528053767));
#32362=CARTESIAN_POINT('',(-67.0574561899986,-0.00106563322407216,-0.454074719462326));
#32363=CARTESIAN_POINT('',(-67.0515283628764,0.0005255561532822,-0.39592528053768));
#32364=CARTESIAN_POINT('',(-67.05475,-9.40612120991423E-14,-3.54592528053767));
#32365=CARTESIAN_POINT('Ctrl Pts',(-67.0515283628764,0.000525556153282321,
-0.39592528053768));
#32366=CARTESIAN_POINT('Ctrl Pts',(-67.0506691385159,-0.374799386930345,
-0.375650446188706));
#32367=CARTESIAN_POINT('Ctrl Pts',(-66.7723630529996,-1.43710026477804,
-0.318329648317051));
#32368=CARTESIAN_POINT('Ctrl Pts',(-65.0662097961853,-2.42773505180942,
-0.223962886922715));
#32369=CARTESIAN_POINT('Ctrl Pts',(-62.9962315570428,-1.37229494871089,
-0.112824996354674));
#32370=CARTESIAN_POINT('Ctrl Pts',(-62.7603252963136,0.939222336522791,
-0.00168710578663132));
#32371=CARTESIAN_POINT('Ctrl Pts',(-64.5744186923722,2.39105873890073,0.10945078478141));
#32372=CARTESIAN_POINT('Ctrl Pts',(-66.5952919861857,1.71543281453755,0.211371393197727));
#32373=CARTESIAN_POINT('Ctrl Pts',(-67.0497995509631,0.511440405058386,
0.276246038091363));
#32374=CARTESIAN_POINT('Ctrl Pts',(-67.0544463703074,-0.00187701683782321,
0.304074719462319));
#32375=CARTESIAN_POINT('Ctrl Pts',(-67.0574561899986,-0.00106563322407194,
-0.454074719462326));
#32376=CARTESIAN_POINT('Ctrl Pts',(-67.057843018648,-0.062350262845054,
-0.450739656990689));
#32377=CARTESIAN_POINT('Ctrl Pts',(-67.0275621697751,-0.803998615243591,
-0.410358630996372));
#32378=CARTESIAN_POINT('Ctrl Pts',(-66.1288520704621,-2.15034287637184,
-0.332931641479373));
#32379=CARTESIAN_POINT('Ctrl Pts',(-63.8056023683761,-2.11463875683277,
-0.221793750911332));
#32380=CARTESIAN_POINT('Ctrl Pts',(-62.5755981242121,-0.143381478345974,
-0.110655860343291));
#32381=CARTESIAN_POINT('Ctrl Pts',(-63.5646765331008,1.95911432942999,0.00048203022475183));
#32382=CARTESIAN_POINT('Ctrl Pts',(-65.8675227272721,2.26841065672896,0.111619920792793));
#32383=CARTESIAN_POINT('Ctrl Pts',(-66.9782240837151,0.967625288007812,
0.193434337563767));
#32384=CARTESIAN_POINT('Ctrl Pts',(-67.0565942986505,0.144137863188435,
0.238202790812061));
#32385=CARTESIAN_POINT('Ctrl Pts',(-67.05528106155,0.00183967754518984,
0.245925280537674));
#32386=CARTESIAN_POINT('Origin',(-65.,8.88178419700125E-15,-3.54592528053767));
#32387=CARTESIAN_POINT('',(-67.0520762837074,-0.00116136879358866,-1.15407471946233));
#32388=CARTESIAN_POINT('',(-67.0563730581704,0.00160407492546517,-1.09592528053768));
#32389=CARTESIAN_POINT('',(-67.05475,-9.40612120991423E-14,-3.54592528053767));
#32390=CARTESIAN_POINT('Ctrl Pts',(-67.0563730581704,0.00160407492546514,
-1.09592528053768));
#32391=CARTESIAN_POINT('Ctrl Pts',(-67.051425463294,-0.57494887244027,-1.06459289399146));
#32392=CARTESIAN_POINT('Ctrl Pts',(-66.4979405147664,-1.84151750410658,
-0.99621454392255));
#32393=CARTESIAN_POINT('Ctrl Pts',(-64.3510553719621,-2.34032995360773,
-0.890790230330967));
#32394=CARTESIAN_POINT('Ctrl Pts',(-62.6818041989874,-0.724051597351479,
-0.779652339762924));
#32395=CARTESIAN_POINT('Ctrl Pts',(-63.1344238327198,1.55496249063294,-0.668514449194883));
#32396=CARTESIAN_POINT('Ctrl Pts',(-65.2946265402067,2.41070020734328,-0.55737655862684));
#32397=CARTESIAN_POINT('Ctrl Pts',(-66.8402661138972,1.30632380217905,-0.466513502407773));
#32398=CARTESIAN_POINT('Ctrl Pts',(-67.0522391042067,0.310990391240222,
-0.412696409711387));
#32399=CARTESIAN_POINT('Ctrl Pts',(-67.0515283628764,0.000525556153282321,
-0.39592528053768));
#32400=CARTESIAN_POINT('Ctrl Pts',(-67.0520762837074,-0.0011613687935888,
-1.15407471946233));
#32401=CARTESIAN_POINT('Ctrl Pts',(-67.053454237916,-0.267420438121926,
-1.13968210479344));
#32402=CARTESIAN_POINT('Ctrl Pts',(-66.8815877450925,-1.21731358290939,
-1.08824352660187));
#32403=CARTESIAN_POINT('Ctrl Pts',(-65.4483108550045,-2.38688976599862,
-0.999758984887625));
#32404=CARTESIAN_POINT('Ctrl Pts',(-63.2377776981899,-1.67118490708905,
-0.888621094319582));
#32405=CARTESIAN_POINT('Ctrl Pts',(-62.6402125087857,0.574193448178942,
-0.777483203751542));
#32406=CARTESIAN_POINT('Ctrl Pts',(-64.2025947176117,2.29399639382146,-0.666345313183498));
#32407=CARTESIAN_POINT('Ctrl Pts',(-66.4260607263055,1.92548386768539,-0.558542485087094));
#32408=CARTESIAN_POINT('Ctrl Pts',(-67.0535461156186,0.618401049236239,
-0.48778562051337));
#32409=CARTESIAN_POINT('Ctrl Pts',(-67.0574561899986,-0.00106563322407194,
-0.454074719462326));
#32410=CARTESIAN_POINT('Origin',(-65.,8.88178419700125E-15,-3.54592528053767));
#32411=CARTESIAN_POINT('',(-67.052679279082,0.0023836951352374,-1.85407471946233));
#32412=CARTESIAN_POINT('',(-67.0565599569794,-0.0014937474477788,-1.79592528053768));
#32413=CARTESIAN_POINT('',(-67.05475,-9.40612120991423E-14,-3.54592528053767));
#32414=CARTESIAN_POINT('',(-65.5301702171886,1.98517432567173,-2.));
#32415=CARTESIAN_POINT('Ctrl Pts',(-65.5301702171886,1.98517432567173,-2.));
#32416=CARTESIAN_POINT('Ctrl Pts',(-66.1902879097456,1.80888011517989,-1.96295403647732));
#32417=CARTESIAN_POINT('Ctrl Pts',(-66.9249664054372,1.11286144556364,-1.91431227629809));
#32418=CARTESIAN_POINT('Ctrl Pts',(-67.0542991139265,0.216633244974153,
-1.86567051611887));
#32419=CARTESIAN_POINT('Ctrl Pts',(-67.052679279082,0.0023836951352375,
-1.85407471946232));
#32420=CARTESIAN_POINT('',(-64.468704775017,1.98873730573667,-2.));
#32421=CARTESIAN_POINT('Origin',(-65.,8.88178419700125E-15,-2.));
#32422=CARTESIAN_POINT('Ctrl Pts',(-64.4687042096542,1.98873909628093,-2.));
#32423=CARTESIAN_POINT('Ctrl Pts',(-65.1133181823237,2.16007183004146,-1.96367708181445));
#32424=CARTESIAN_POINT('Ctrl Pts',(-66.4930415100228,1.84061483765585,-1.89565217532701));
#32425=CARTESIAN_POINT('Ctrl Pts',(-67.051699865038,0.581583302606364,-1.82762726883957));
#32426=CARTESIAN_POINT('Ctrl Pts',(-67.0565599569794,-0.00149374744777858,
-1.79592528053768));
#32427=CARTESIAN_POINT('Origin',(-32.5,-56.2916512459885,3.));
#32428=CARTESIAN_POINT('',(-33.334828594439,-57.735188017533,6.12851963660979));
#32429=CARTESIAN_POINT('',(-33.3331620889267,-57.736668395617,6.32148036339022));
#32430=CARTESIAN_POINT('',(-33.333,-57.7344495686934,3.));
#32431=CARTESIAN_POINT('',(-33.5940263469955,-57.5480995545471,7.));
#32432=CARTESIAN_POINT('Ctrl Pts',(-33.3331620889267,-57.736668395617,6.32148036339022));
#32433=CARTESIAN_POINT('Ctrl Pts',(-33.2830618082469,-57.7660644611829,
6.3253777944574));
#32434=CARTESIAN_POINT('Ctrl Pts',(-33.2314063486239,-57.7926890534068,
6.32927522552458));
#32435=CARTESIAN_POINT('Ctrl Pts',(-33.1783991110197,-57.816276539757,6.33317265659176));
#32436=CARTESIAN_POINT('Ctrl Pts',(-32.6745533323838,-58.0404809307675,
6.37021862011444));
#32437=CARTESIAN_POINT('Ctrl Pts',(-32.0485753278831,-57.9902848612727,
6.40726458363712));
#32438=CARTESIAN_POINT('Ctrl Pts',(-31.5869763637319,-57.6885282775577,
6.4443105471598));
#32439=CARTESIAN_POINT('Ctrl Pts',(-31.1253773995808,-57.3867716938426,
6.48135651068248));
#32440=CARTESIAN_POINT('Ctrl Pts',(-30.8281574757792,-56.8334545959073,
6.51840247420516));
#32441=CARTESIAN_POINT('Ctrl Pts',(-30.8312835014825,-56.2820697925606,
6.55544843772784));
#32442=CARTESIAN_POINT('Ctrl Pts',(-30.8344095271858,-55.730684989214,6.59249440125052));
#32443=CARTESIAN_POINT('Ctrl Pts',(-31.1378815023941,-55.181232480456,6.6295403647732));
#32444=CARTESIAN_POINT('Ctrl Pts',(-31.6029277671502,-54.8846445462124,
6.66658632829588));
#32445=CARTESIAN_POINT('Ctrl Pts',(-32.0679740319062,-54.5880566119689,
6.70363229181856));
#32446=CARTESIAN_POINT('Ctrl Pts',(-32.69459458621,-54.5443332522399,6.74067825534124));
#32447=CARTESIAN_POINT('Ctrl Pts',(-33.1957905862087,-54.7745591362764,
6.77772421886393));
#32448=CARTESIAN_POINT('Ctrl Pts',(-33.6969865862074,-55.0047850203128,
6.81477018238661));
#32449=CARTESIAN_POINT('Ctrl Pts',(-34.072758031901,-55.5089601481148,6.85181614590929));
#32450=CARTESIAN_POINT('Ctrl Pts',(-34.1514677107856,-56.0538413345857,
6.88886210943197));
#32451=CARTESIAN_POINT('Ctrl Pts',(-34.2301773896702,-56.5987225210566,
6.92590807295465));
#32452=CARTESIAN_POINT('Ctrl Pts',(-34.0118253017458,-57.1843097661965,
6.96295403647733));
#32453=CARTESIAN_POINT('Ctrl Pts',(-33.5940263469955,-57.5480995545471,
7.00000000000001));
#32454=CARTESIAN_POINT('',(-31.0815846268762,-57.1712794637622,7.));
#32455=CARTESIAN_POINT('Origin',(-32.5,-56.2916512459885,7.));
#32456=CARTESIAN_POINT('',(-33.3322874886545,-57.7319139206533,6.82851963660979));
#32457=CARTESIAN_POINT('Ctrl Pts',(-31.0815830733444,-57.1712803260695,
7.));
#32458=CARTESIAN_POINT('Ctrl Pts',(-31.3671885733957,-57.6305045882042,
6.96367708181444));
#32459=CARTESIAN_POINT('Ctrl Pts',(-31.8971081113245,-57.9389632567025,
6.92735416362889));
#32460=CARTESIAN_POINT('Ctrl Pts',(-32.4375390310396,-57.9591354579208,
6.89103124544334));
#32461=CARTESIAN_POINT('Ctrl Pts',(-32.747565573898,-57.9707075526648,6.87019404249882));
#32462=CARTESIAN_POINT('Ctrl Pts',(-33.0610513288344,-57.8874068657131,
6.8493568395543));
#32463=CARTESIAN_POINT('Ctrl Pts',(-33.3322874886545,-57.7319139206533,
6.82851963660979));
#32464=CARTESIAN_POINT('',(-33.333,-57.7344495686934,8.));
#32465=CARTESIAN_POINT('',(-33.333,-57.7344495686934,3.));
#32466=CARTESIAN_POINT('Origin',(-32.5,-56.2916512459885,8.));
#32467=CARTESIAN_POINT('Ctrl Pts',(-33.3322874886545,-57.7319139206533,
6.82851963660979));
#32468=CARTESIAN_POINT('Ctrl Pts',(-33.5432755942256,-57.6109596867872,
6.81231087603162));
#32469=CARTESIAN_POINT('Ctrl Pts',(-33.7286988454439,-57.4463225594196,
6.79610211545346));
#32470=CARTESIAN_POINT('Ctrl Pts',(-33.8670427528186,-57.2486779404331,
6.77989335487529));
#32471=CARTESIAN_POINT('Ctrl Pts',(-34.1832349330579,-56.796950906147,6.74284739135261));
#32472=CARTESIAN_POINT('Ctrl Pts',(-34.2534965093546,-56.1728010705694,
6.70580142782993));
#32473=CARTESIAN_POINT('Ctrl Pts',(-34.0454742915244,-55.6620590905692,
6.66875546430725));
#32474=CARTESIAN_POINT('Ctrl Pts',(-33.8374520736943,-55.151317110569,6.63170950078457));
#32475=CARTESIAN_POINT('Ctrl Pts',(-33.3511460617375,-54.7539829861461,
6.59466353726189));
#32476=CARTESIAN_POINT('Ctrl Pts',(-32.8092161915406,-54.651806090904,6.55761757373921));
#32477=CARTESIAN_POINT('Ctrl Pts',(-32.2672863213437,-54.549629195662,6.52057161021653));
#32478=CARTESIAN_POINT('Ctrl Pts',(-31.6697325929069,-54.7426095296008,
6.48352564669385));
#32479=CARTESIAN_POINT('Ctrl Pts',(-31.2899790079621,-55.1424751852064,
6.44647968317117));
#32480=CARTESIAN_POINT('Ctrl Pts',(-30.9102254230173,-55.542340840812,6.40943371964849));
#32481=CARTESIAN_POINT('Ctrl Pts',(-30.7482719815646,-56.1490918180843,
6.37238775612581));
#32482=CARTESIAN_POINT('Ctrl Pts',(-30.8782626384457,-56.6850216626072,
6.33534179260313));
#32483=CARTESIAN_POINT('Ctrl Pts',(-31.0082532953267,-57.2209515071302,
6.29829582908045));
#32484=CARTESIAN_POINT('Ctrl Pts',(-31.4301880505415,-57.6860602189039,
6.26124986555777));
#32485=CARTESIAN_POINT('Ctrl Pts',(-31.9509534890594,-57.8674999291041,
6.22420390203509));
#32486=CARTESIAN_POINT('Ctrl Pts',(-32.3993069550896,-58.023710608475,6.19230914689332));
#32487=CARTESIAN_POINT('Ctrl Pts',(-32.9209173239095,-57.9696554900369,
6.16041439175155));
#32488=CARTESIAN_POINT('Ctrl Pts',(-33.334828594439,-57.735188017533,6.12851963660979));
#32489=CARTESIAN_POINT('Origin',(-32.5,-56.2916512459885,3.));
#32490=CARTESIAN_POINT('',(-33.3324736911222,-57.7361875215801,5.42851963660979));
#32491=CARTESIAN_POINT('',(-33.3311322154953,-57.7328790961699,5.62148036339021));
#32492=CARTESIAN_POINT('',(-33.333,-57.7344495686934,3.));
#32493=CARTESIAN_POINT('Ctrl Pts',(-33.3311322154953,-57.7328790961699,
5.62148036339021));
#32494=CARTESIAN_POINT('Ctrl Pts',(-33.1373356857267,-57.8459393971242,
5.63643534665465));
#32495=CARTESIAN_POINT('Ctrl Pts',(-32.9222440320564,-57.9213835767879,
5.65139032991907));
#32496=CARTESIAN_POINT('Ctrl Pts',(-32.7012486057465,-57.9482311745983,
5.6663453131835));
#32497=CARTESIAN_POINT('Ctrl Pts',(-32.1538064350001,-58.0147371085448,
5.70339127670618));
#32498=CARTESIAN_POINT('Ctrl Pts',(-31.5701366653479,-57.7830375418651,
5.74043724022886));
#32499=CARTESIAN_POINT('Ctrl Pts',(-31.2173595401895,-57.3591689672607,
5.77748320375154));
#32500=CARTESIAN_POINT('Ctrl Pts',(-30.8645824150311,-56.9353003926564,
5.81452916727423));
#32501=CARTESIAN_POINT('Ctrl Pts',(-30.7426979343665,-56.3192628101275,
5.85157513079691));
#32502=CARTESIAN_POINT('Ctrl Pts',(-30.9074862986933,-55.7929935490272,
5.88862109431959));
#32503=CARTESIAN_POINT('Ctrl Pts',(-31.0722746630201,-55.266724287927,5.92566705784227));
#32504=CARTESIAN_POINT('Ctrl Pts',(-31.5237358723384,-54.8302233482555,
5.96271302136495));
#32505=CARTESIAN_POINT('Ctrl Pts',(-32.0552579823816,-54.6832494251182,
5.99975898488763));
#32506=CARTESIAN_POINT('Ctrl Pts',(-32.5867800924248,-54.5362755019809,
6.03680494841031));
#32507=CARTESIAN_POINT('Ctrl Pts',(-33.1983631031929,-54.6788285953779,
6.07385091193299));
#32508=CARTESIAN_POINT('Ctrl Pts',(-33.6101089221165,-55.0456852682332,
6.11089687545567));
#32509=CARTESIAN_POINT('Ctrl Pts',(-34.02185474104,-55.4125419410885,6.14794283897835));
#32510=CARTESIAN_POINT('Ctrl Pts',(-34.233763368119,-56.003702193402,6.18498880250103));
#32511=CARTESIAN_POINT('Ctrl Pts',(-34.1488609052729,-56.5485847453165,
6.22203476602372));
#32512=CARTESIAN_POINT('Ctrl Pts',(-34.0728906300368,-57.0361427742909,
6.25518329847922));
#32513=CARTESIAN_POINT('Ctrl Pts',(-33.7592763040381,-57.4866482113774,
6.28833183093472));
#32514=CARTESIAN_POINT('Ctrl Pts',(-33.3331620889267,-57.736668395617,6.32148036339022));
#32515=CARTESIAN_POINT('Ctrl Pts',(-33.334828594439,-57.735188017533,6.12851963660979));
#32516=CARTESIAN_POINT('Ctrl Pts',(-33.4016779305205,-57.6973200105818,
6.12336842822887));
#32517=CARTESIAN_POINT('Ctrl Pts',(-33.4657180077386,-57.6547460681795,
6.11821721984796));
#32518=CARTESIAN_POINT('Ctrl Pts',(-33.5261864969391,-57.6075919565364,
6.11306601146705));
#32519=CARTESIAN_POINT('Ctrl Pts',(-33.96105794448,-57.2684735651416,6.07602004794436));
#32520=CARTESIAN_POINT('Ctrl Pts',(-34.2112047177408,-56.6924660737253,
6.03897408442168));
#32521=CARTESIAN_POINT('Ctrl Pts',(-34.1621425519641,-56.1431855476954,
6.001928120899));
#32522=CARTESIAN_POINT('Ctrl Pts',(-34.1130803861875,-55.5939050216654,
5.96488215737632));
#32523=CARTESIAN_POINT('Ctrl Pts',(-33.7648092813734,-55.0713514610218,
5.92783619385364));
#32524=CARTESIAN_POINT('Ctrl Pts',(-33.2767190788242,-54.8146729733941,
5.89079023033096));
#32525=CARTESIAN_POINT('Ctrl Pts',(-32.788628876275,-54.5579944857664,5.85374426680828));
#32526=CARTESIAN_POINT('Ctrl Pts',(-32.1607195759906,-54.5671910711545,
5.8166983032856));
#32527=CARTESIAN_POINT('Ctrl Pts',(-31.6803566282498,-54.8380546099095,
5.77965233976292));
#32528=CARTESIAN_POINT('Ctrl Pts',(-31.199993680509,-55.1089181486644,5.74260637624024));
#32529=CARTESIAN_POINT('Ctrl Pts',(-30.8671770853119,-55.6414486407862,
5.70556041271756));
#32530=CARTESIAN_POINT('Ctrl Pts',(-30.834222647304,-56.1919301102113,5.66851444919488));
#32531=CARTESIAN_POINT('Ctrl Pts',(-30.8012682092961,-56.7424115796364,
5.63146848567219));
#32532=CARTESIAN_POINT('Ctrl Pts',(-31.0681759284774,-57.3108440263648,
5.59442252214951));
#32533=CARTESIAN_POINT('Ctrl Pts',(-31.5127937714062,-57.6370813071645,
5.55737655862683));
#32534=CARTESIAN_POINT('Ctrl Pts',(-31.9574116143351,-57.9633185879642,
5.52033059510415));
#32535=CARTESIAN_POINT('Ctrl Pts',(-32.5797395810114,-58.0473607028353,
5.48328463158148));
#32536=CARTESIAN_POINT('Ctrl Pts',(-33.0949658502735,-57.8507452062819,
5.4462386680588));
#32537=CARTESIAN_POINT('Ctrl Pts',(-33.1771098465446,-57.8193982358743,
5.44033232424246));
#32538=CARTESIAN_POINT('Ctrl Pts',(-33.2565314423349,-57.7809172756724,
5.43442598042612));
#32539=CARTESIAN_POINT('Ctrl Pts',(-33.3324736911222,-57.7361875215801,
5.42851963660979));
#32540=CARTESIAN_POINT('Origin',(-32.5,-56.2916512459885,3.));
#32541=CARTESIAN_POINT('',(-33.3313578105535,-57.7323657066332,4.72851963660978));
#32542=CARTESIAN_POINT('',(-33.3337300498339,-57.7328514726872,4.92148036339021));
#32543=CARTESIAN_POINT('',(-33.333,-57.7344495686934,3.));
#32544=CARTESIAN_POINT('Ctrl Pts',(-33.3337300498339,-57.7328514726872,
4.92148036339021));
#32545=CARTESIAN_POINT('Ctrl Pts',(-32.9948149402968,-57.9248393749082,
4.94749289885189));
#32546=CARTESIAN_POINT('Ctrl Pts',(-32.5875734400098,-58.0025082442025,
4.97350543431357));
#32547=CARTESIAN_POINT('Ctrl Pts',(-32.2063909254829,-57.9343784669252,
4.99951796977525));
#32548=CARTESIAN_POINT('Ctrl Pts',(-31.6635267533437,-57.8373508916032,
5.03656393329793));
#32549=CARTESIAN_POINT('Ctrl Pts',(-31.1735161025779,-57.4446106606261,
5.07360989682062));
#32550=CARTESIAN_POINT('Ctrl Pts',(-30.9606151335011,-56.9358975335329,
5.1106558603433));
#32551=CARTESIAN_POINT('Ctrl Pts',(-30.7477141644243,-56.4271844064398,
5.14770182386598));
#32552=CARTESIAN_POINT('Ctrl Pts',(-30.8119228770365,-55.8024983832305,
5.18474778738865));
#32553=CARTESIAN_POINT('Ctrl Pts',(-31.1238557751029,-55.3477306326436,
5.22179375091133));
#32554=CARTESIAN_POINT('Ctrl Pts',(-31.4357886731693,-54.8929628820567,
5.25883971443402));
#32555=CARTESIAN_POINT('Ctrl Pts',(-31.9954457566899,-54.6081134040922,
5.2958856779567));
#32556=CARTESIAN_POINT('Ctrl Pts',(-32.5466968174263,-54.6235450421449,
5.33293164147938));
#32557=CARTESIAN_POINT('Ctrl Pts',(-33.0979478781627,-54.6389766801977,
5.36997760500206));
#32558=CARTESIAN_POINT('Ctrl Pts',(-33.6407929161149,-54.9546894342676,
5.40702356852474));
#32559=CARTESIAN_POINT('Ctrl Pts',(-33.9267957627755,-55.4261958418307,
5.44406953204742));
#32560=CARTESIAN_POINT('Ctrl Pts',(-34.2127986094362,-55.8977022493938,
5.4811154955701));
#32561=CARTESIAN_POINT('Ctrl Pts',(-34.2419592648052,-56.5250023104501,
5.51816145909278));
#32562=CARTESIAN_POINT('Ctrl Pts',(-34.0009323065694,-57.0210080582645,
5.55520742261547));
#32563=CARTESIAN_POINT('Ctrl Pts',(-33.8572048591017,-57.3167826080678,
5.57729840287372));
#32564=CARTESIAN_POINT('Ctrl Pts',(-33.6174016975492,-57.565870358533,5.59938938313197));
#32565=CARTESIAN_POINT('Ctrl Pts',(-33.3311322154953,-57.7328790961699,
5.62148036339021));
#32566=CARTESIAN_POINT('Ctrl Pts',(-33.3324736911222,-57.7361875215801,
5.42851963660979));
#32567=CARTESIAN_POINT('Ctrl Pts',(-33.7328589074961,-57.5003618440874,
5.39738001690344));
#32568=CARTESIAN_POINT('Ctrl Pts',(-34.0365306675145,-57.0908419490654,
5.36624039719709));
#32569=CARTESIAN_POINT('Ctrl Pts',(-34.1325589902306,-56.6373526743003,
5.33510077749075));
#32570=CARTESIAN_POINT('Ctrl Pts',(-34.246801289078,-56.0978487468504,5.29805481396807));
#32571=CARTESIAN_POINT('Ctrl Pts',(-34.0671613149251,-55.4961139999285,
5.26100885044539));
#32572=CARTESIAN_POINT('Ctrl Pts',(-33.6758523462209,-55.1075357285357,
5.22396288692271));
#32573=CARTESIAN_POINT('Ctrl Pts',(-33.2845433775166,-54.7189574571428,
5.18691692340003));
#32574=CARTESIAN_POINT('Ctrl Pts',(-32.681565414261,-54.5435356612789,5.14987095987735));
#32575=CARTESIAN_POINT('Ctrl Pts',(-32.1428747275693,-54.6615531325857,
5.11282499635467));
#32576=CARTESIAN_POINT('Ctrl Pts',(-31.6041840408777,-54.7795706038924,
5.07577903283198));
#32577=CARTESIAN_POINT('Ctrl Pts',(-31.12978063075,-55.1910273423697,5.03873306930931));
#32578=CARTESIAN_POINT('Ctrl Pts',(-30.9367779143555,-55.7076178324787,
5.00168710578663));
#32579=CARTESIAN_POINT('Ctrl Pts',(-30.7437751979609,-56.2242083225877,
4.96464114226394));
#32580=CARTESIAN_POINT('Ctrl Pts',(-30.8321731752993,-56.8459325643283,
4.92759517874126));
#32581=CARTESIAN_POINT('Ctrl Pts',(-31.1615160075389,-57.2882549360944,
4.89054921521858));
#32582=CARTESIAN_POINT('Ctrl Pts',(-31.4908588397784,-57.7305773078605,
4.8535032516959));
#32583=CARTESIAN_POINT('Ctrl Pts',(-32.0611465269192,-57.9934978096521,
4.81645728817322));
#32584=CARTESIAN_POINT('Ctrl Pts',(-32.6113836768238,-57.956689381435,4.77941132465054));
#32585=CARTESIAN_POINT('Ctrl Pts',(-32.8633454266668,-57.93983425636,4.76244742863696));
#32586=CARTESIAN_POINT('Ctrl Pts',(-33.1111028597659,-57.8601301739612,
4.74548353262337));
#32587=CARTESIAN_POINT('Ctrl Pts',(-33.3313578105535,-57.7323657066332,
4.72851963660978));
#32588=CARTESIAN_POINT('Origin',(-32.5,-56.2916512459885,3.));
#32589=CARTESIAN_POINT('',(-33.3342430690557,-57.7335557705023,4.02851963660978));
#32590=CARTESIAN_POINT('',(-33.3343740412804,-57.7368429003791,4.22148036339021));
#32591=CARTESIAN_POINT('',(-33.333,-57.7344495686934,3.));
#32592=CARTESIAN_POINT('Ctrl Pts',(-33.3343740344483,-57.7368428884788,
4.22148036339021));
#32593=CARTESIAN_POINT('Ctrl Pts',(-32.8564950497481,-58.0127845069312,
4.25855045104914));
#32594=CARTESIAN_POINT('Ctrl Pts',(-32.2282029771155,-58.0281412318725,
4.29562053870807));
#32595=CARTESIAN_POINT('Ctrl Pts',(-31.7373727175272,-57.7759553439527,
4.332690626367));
#32596=CARTESIAN_POINT('Ctrl Pts',(-31.2468618760144,-57.5239335712834,
4.36973658988968));
#32597=CARTESIAN_POINT('Ctrl Pts',(-30.8936340516087,-57.0047173912526,
4.40678255341236));
#32598=CARTESIAN_POINT('Ctrl Pts',(-30.8393459612069,-56.4559290322592,
4.44382851693504));
#32599=CARTESIAN_POINT('Ctrl Pts',(-30.7850578708051,-55.9071406732657,
4.48087448045772));
#32600=CARTESIAN_POINT('Ctrl Pts',(-31.0297095144072,-55.3287801353096,
4.51792044398041));
#32601=CARTESIAN_POINT('Ctrl Pts',(-31.4613346798115,-54.9855373992054,
4.55496640750309));
#32602=CARTESIAN_POINT('Ctrl Pts',(-31.8929598452159,-54.6422946631012,
4.59201237102577));
#32603=CARTESIAN_POINT('Ctrl Pts',(-32.5115585324226,-54.5341697288488,
4.62905833454844));
#32604=CARTESIAN_POINT('Ctrl Pts',(-33.0340255450119,-54.7106465835455,
4.66610429807112));
#32605=CARTESIAN_POINT('Ctrl Pts',(-33.5564925576013,-54.8871234382422,
4.70315026159381));
#32606=CARTESIAN_POINT('Ctrl Pts',(-33.9828278955734,-55.348202081888,4.74019622511649));
#32607=CARTESIAN_POINT('Ctrl Pts',(-34.1179167730764,-55.8828672630521,
4.77724218863917));
#32608=CARTESIAN_POINT('Ctrl Pts',(-34.2530056505794,-56.4175324442162,
4.81428815216185));
#32609=CARTESIAN_POINT('Ctrl Pts',(-34.0968480676134,-57.0257841628987,
4.85133411568453));
#32610=CARTESIAN_POINT('Ctrl Pts',(-33.7209104293741,-57.4292525624064,
4.88838007920721));
#32611=CARTESIAN_POINT('Ctrl Pts',(-33.6089446308763,-57.5494178688947,
4.89941350726821));
#32612=CARTESIAN_POINT('Ctrl Pts',(-33.4774836445334,-57.6514182455857,
4.91044693532921));
#32613=CARTESIAN_POINT('Ctrl Pts',(-33.3337300498339,-57.7328514726872,
4.92148036339021));
#32614=CARTESIAN_POINT('Ctrl Pts',(-33.3313578105535,-57.7323657066332,
4.72851963660978));
#32615=CARTESIAN_POINT('Ctrl Pts',(-33.5920983142318,-57.5811165681046,
4.70843756910069));
#32616=CARTESIAN_POINT('Ctrl Pts',(-33.8142965260144,-57.3625150588492,
4.68835550159159));
#32617=CARTESIAN_POINT('Ctrl Pts',(-33.9593006043585,-57.1010955378143,
4.6682734340825));
#32618=CARTESIAN_POINT('Ctrl Pts',(-34.22679376932,-56.6188474806364,4.63122747055982));
#32619=CARTESIAN_POINT('Ctrl Pts',(-34.2315934865741,-55.9908887245065,
4.59418150703714));
#32620=CARTESIAN_POINT('Ctrl Pts',(-33.9715031387158,-55.5046081545498,
4.55713554351446));
#32621=CARTESIAN_POINT('Ctrl Pts',(-33.7114127908575,-55.0183275845932,
4.52008957999178));
#32622=CARTESIAN_POINT('Ctrl Pts',(-33.1864323778867,-54.6737252008098,
4.4830436164691));
#32623=CARTESIAN_POINT('Ctrl Pts',(-32.6368221624337,-54.6285102383604,
4.44599765294642));
#32624=CARTESIAN_POINT('Ctrl Pts',(-32.0872119469808,-54.5832952759111,
4.40895168942373));
#32625=CARTESIAN_POINT('Ctrl Pts',(-31.5129719290456,-54.8374677347958,
4.37190572590106));
#32626=CARTESIAN_POINT('Ctrl Pts',(-31.1769063091028,-55.2747041478526,
4.33485976237838));
#32627=CARTESIAN_POINT('Ctrl Pts',(-30.84084068916,-55.7119405609094,4.2978137988557));
#32628=CARTESIAN_POINT('Ctrl Pts',(-30.7429494672094,-56.3322409281384,
4.26076783533301));
#32629=CARTESIAN_POINT('Ctrl Pts',(-30.9280331160056,-56.8517212691839,
4.22372187181033));
#32630=CARTESIAN_POINT('Ctrl Pts',(-31.1131167648017,-57.3712016102293,
4.18667590828765));
#32631=CARTESIAN_POINT('Ctrl Pts',(-31.5811752843445,-57.7898619250913,
4.14962994476497));
#32632=CARTESIAN_POINT('Ctrl Pts',(-32.1179990391191,-57.9160999466831,
4.11258398124229));
#32633=CARTESIAN_POINT('Ctrl Pts',(-32.5240508086608,-58.0115859820809,
4.08456253303146));
#32634=CARTESIAN_POINT('Ctrl Pts',(-32.9694456528715,-57.939766662088,4.05654108482062));
#32635=CARTESIAN_POINT('Ctrl Pts',(-33.3342430690557,-57.7335557705023,
4.02851963660978));
#32636=CARTESIAN_POINT('Origin',(-32.5,-56.2916512459885,3.));
#32637=CARTESIAN_POINT('',(-33.3337922536522,-57.7369224948681,3.32851963660979));
#32638=CARTESIAN_POINT('',(-33.3312448475264,-57.7342636967217,3.52148036339021));
#32639=CARTESIAN_POINT('',(-33.333,-57.7344495686934,3.));
#32640=CARTESIAN_POINT('Ctrl Pts',(-33.3312448475264,-57.7342636967217,
3.52148036339021));
#32641=CARTESIAN_POINT('Ctrl Pts',(-33.1882152402262,-57.8184056914071,
3.53256203972371));
#32642=CARTESIAN_POINT('Ctrl Pts',(-33.0334203647077,-57.8814418696117,
3.54364371605721));
#32643=CARTESIAN_POINT('Ctrl Pts',(-32.8726233824478,-57.9182768459085,
3.55472539239071));
#32644=CARTESIAN_POINT('Ctrl Pts',(-32.3350802382442,-58.0414159042227,
3.59177135591339));
#32645=CARTESIAN_POINT('Ctrl Pts',(-31.7304599472088,-57.871740798566,3.62881731943607));
#32646=CARTESIAN_POINT('Ctrl Pts',(-31.3354704139632,-57.4869043031699,
3.66586328295875));
#32647=CARTESIAN_POINT('Ctrl Pts',(-30.9404808807176,-57.1020678077737,
3.70290924648143));
#32648=CARTESIAN_POINT('Ctrl Pts',(-30.7551221052618,-56.5020699226381,
3.73995521000411));
#32649=CARTESIAN_POINT('Ctrl Pts',(-30.8642245822409,-55.961503082106,3.77700117352679));
#32650=CARTESIAN_POINT('Ctrl Pts',(-30.9733270592199,-55.4209362415738,
3.81404713704947));
#32651=CARTESIAN_POINT('Ctrl Pts',(-31.3768907886338,-54.9398004456451,
3.85109310057215));
#32652=CARTESIAN_POINT('Ctrl Pts',(-31.8902225413504,-54.7382902195697,
3.88813906409484));
#32653=CARTESIAN_POINT('Ctrl Pts',(-32.403554294067,-54.5367799934943,3.92518502761751));
#32654=CARTESIAN_POINT('Ctrl Pts',(-33.0266540700863,-54.6148953372722,
3.96223099114019));
#32655=CARTESIAN_POINT('Ctrl Pts',(-33.4743567237048,-54.9368863208444,
3.99927695466287));
#32656=CARTESIAN_POINT('Ctrl Pts',(-33.9220593773232,-55.2588773044166,
4.03632291818555));
#32657=CARTESIAN_POINT('Ctrl Pts',(-34.1943649085407,-55.8247439277831,
4.07336888170824));
#32658=CARTESIAN_POINT('Ctrl Pts',(-34.1666511469031,-56.3755141221477,
4.11041484523092));
#32659=CARTESIAN_POINT('Ctrl Pts',(-34.138955432321,-56.9259256578638,4.14743668461735));
#32660=CARTESIAN_POINT('Ctrl Pts',(-33.8116310396246,-57.4612604196062,
4.18445852400378));
#32661=CARTESIAN_POINT('Ctrl Pts',(-33.3343740344483,-57.7368428884788,
4.22148036339021));
#32662=CARTESIAN_POINT('Ctrl Pts',(-33.3342430690557,-57.7335557705023,
4.02851963660978));
#32663=CARTESIAN_POINT('Ctrl Pts',(-33.4517287836878,-57.6671440228088,
4.01949512129794));
#32664=CARTESIAN_POINT('Ctrl Pts',(-33.560854853963,-57.5867930493783,4.01047060598609));
#32665=CARTESIAN_POINT('Ctrl Pts',(-33.6576147739257,-57.4936023059229,
4.00144609067425));
#32666=CARTESIAN_POINT('Ctrl Pts',(-34.0548177639512,-57.1110509152492,
3.96440012715157));
#32667=CARTESIAN_POINT('Ctrl Pts',(-34.2436347539959,-56.5121324055803,
3.92735416362889));
#32668=CARTESIAN_POINT('Ctrl Pts',(-34.1376525779071,-55.9709452289588,
3.89030820010621));
#32669=CARTESIAN_POINT('Ctrl Pts',(-34.0316704018183,-55.4297580523374,
3.85326223658353));
#32670=CARTESIAN_POINT('Ctrl Pts',(-33.6308890595962,-54.9463022087633,
3.81621627306085));
#32671=CARTESIAN_POINT('Ctrl Pts',(-33.1187284050901,-54.7418340064325,
3.77917030953817));
#32672=CARTESIAN_POINT('Ctrl Pts',(-32.6065677505839,-54.5373658041018,
3.74212434601549));
#32673=CARTESIAN_POINT('Ctrl Pts',(-31.9830277837939,-54.6118852430143,
3.70507838249281));
#32674=CARTESIAN_POINT('Ctrl Pts',(-31.5334751062351,-54.9312880793963,
3.66803241897012));
#32675=CARTESIAN_POINT('Ctrl Pts',(-31.0839224286763,-55.2506909157783,
3.63098645544744));
#32676=CARTESIAN_POINT('Ctrl Pts',(-30.8083570403488,-55.8149771496297,
3.59394049192477));
#32677=CARTESIAN_POINT('Ctrl Pts',(-30.8328930037818,-56.3658979863087,
3.55689452840208));
#32678=CARTESIAN_POINT('Ctrl Pts',(-30.8574289672149,-56.9168188229877,
3.5198485648794));
#32679=CARTESIAN_POINT('Ctrl Pts',(-31.1820662824085,-57.4543742624943,
3.48280260135672));
#32680=CARTESIAN_POINT('Ctrl Pts',(-31.6582328412459,-57.7325490097911,
3.44575663783404));
#32681=CARTESIAN_POINT('Ctrl Pts',(-32.1343994000833,-58.010723757088,3.40871067431136));
#32682=CARTESIAN_POINT('Ctrl Pts',(-32.7620952025646,-58.0295178121752,
3.37166471078868));
#32683=CARTESIAN_POINT('Ctrl Pts',(-33.2540517054067,-57.7803299691728,
3.334618747266));
#32684=CARTESIAN_POINT('Ctrl Pts',(-33.2810496728284,-57.766654847026,3.3325857103806));
#32685=CARTESIAN_POINT('Ctrl Pts',(-33.3076388370087,-57.7521726493388,
3.33055267349519));
#32686=CARTESIAN_POINT('Ctrl Pts',(-33.3337922536522,-57.7369224948681,
3.32851963660979));
#32687=CARTESIAN_POINT('Origin',(-32.5,-56.2916512459885,3.));
#32688=CARTESIAN_POINT('',(-33.3310924906901,-57.7334985910042,2.62851963660979));
#32689=CARTESIAN_POINT('',(-33.3325882586835,-57.7320513890704,2.82148036339021));
#32690=CARTESIAN_POINT('',(-33.333,-57.7344495686934,3.));
#32691=CARTESIAN_POINT('Ctrl Pts',(-33.3325882586835,-57.7320513890704,
2.82148036339021));
#32692=CARTESIAN_POINT('Ctrl Pts',(-33.0441865216604,-57.8968038534098,
2.84361959192096));
#32693=CARTESIAN_POINT('Ctrl Pts',(-32.7077104550096,-57.9799132231487,
2.86575882045171));
#32694=CARTESIAN_POINT('Ctrl Pts',(-32.3790127353427,-57.9560193270483,
2.88789804898246));
#32695=CARTESIAN_POINT('Ctrl Pts',(-31.8289970147924,-57.9160372471796,
2.92494401250514));
#32696=CARTESIAN_POINT('Ctrl Pts',(-31.3007606051993,-57.5764468565745,
2.96198997602782));
#32697=CARTESIAN_POINT('Ctrl Pts',(-31.0360538947178,-57.0926636231019,
2.9990359395505));
#32698=CARTESIAN_POINT('Ctrl Pts',(-30.7713471842363,-56.6088803896294,
3.03608190307318));
#32699=CARTESIAN_POINT('Ctrl Pts',(-30.7701701728664,-55.9809043132894,
3.07312786659586));
#32700=CARTESIAN_POINT('Ctrl Pts',(-31.0330615265357,-55.4961322062854,
3.11017383011854));
#32701=CARTESIAN_POINT('Ctrl Pts',(-31.2959528802049,-55.0113600992815,
3.14721979364122));
#32702=CARTESIAN_POINT('Ctrl Pts',(-31.8229125989134,-54.6697919616135,
3.1842657571639));
#32703=CARTESIAN_POINT('Ctrl Pts',(-32.3727745793293,-54.6277483883086,
3.22131172068658));
#32704=CARTESIAN_POINT('Ctrl Pts',(-32.9226365597451,-54.5857048150036,
3.25835768420926));
#32705=CARTESIAN_POINT('Ctrl Pts',(-33.4954008018683,-54.8431858060618,
3.29540364773194));
#32706=CARTESIAN_POINT('Ctrl Pts',(-33.8289385024972,-55.2823537259082,
3.33244961125463));
#32707=CARTESIAN_POINT('Ctrl Pts',(-34.162476203126,-55.7215216457546,3.36949557477731));
#32708=CARTESIAN_POINT('Ctrl Pts',(-34.2567873622605,-56.3423764943892,
3.40654153829999));
#32709=CARTESIAN_POINT('Ctrl Pts',(-34.0687099431419,-56.8607805298492,
3.44358750182267));
#32710=CARTESIAN_POINT('Ctrl Pts',(-33.9368927177428,-57.2241127252305,
3.46955178901185));
#32711=CARTESIAN_POINT('Ctrl Pts',(-33.6663621789423,-57.5371196140996,
3.49551607620103));
#32712=CARTESIAN_POINT('Ctrl Pts',(-33.3312448475264,-57.7342636967217,
3.52148036339021));
#32713=CARTESIAN_POINT('Ctrl Pts',(-33.3337922536522,-57.7369224948681,
3.32851963660979));
#32714=CARTESIAN_POINT('Ctrl Pts',(-33.7842059499452,-57.4742845941374,
3.29350670997251));
#32715=CARTESIAN_POINT('Ctrl Pts',(-34.1053783658087,-56.9838732473919,
3.25849378333524));
#32716=CARTESIAN_POINT('Ctrl Pts',(-34.1596784920807,-56.465506410459,3.22348085669796));
#32717=CARTESIAN_POINT('Ctrl Pts',(-34.2171315727097,-55.9170404358397,
3.18643489317528));
#32718=CARTESIAN_POINT('Ctrl Pts',(-33.975820530765,-55.3372782276934,3.1493889296526));
#32719=CARTESIAN_POINT('Ctrl Pts',(-33.5461827329191,-54.9915512480536,
3.11234296612992));
#32720=CARTESIAN_POINT('Ctrl Pts',(-33.1165449350731,-54.6458242684137,
3.07529700260724));
#32721=CARTESIAN_POINT('Ctrl Pts',(-32.498580381326,-54.5341325172804,3.03825103908455));
#32722=CARTESIAN_POINT('Ctrl Pts',(-31.9751040537975,-54.7075923578949,
3.00120507556188));
#32723=CARTESIAN_POINT('Ctrl Pts',(-31.4516277262689,-54.8810521985094,
2.96415911203919));
#32724=CARTESIAN_POINT('Ctrl Pts',(-31.0226396249589,-55.3396636308718,
2.92711314851652));
#32725=CARTESIAN_POINT('Ctrl Pts',(-30.88446858696,-55.8735405324578,2.89006718499383));
#32726=CARTESIAN_POINT('Ctrl Pts',(-30.746297548961,-56.4074174340438,2.85302122147115));
#32727=CARTESIAN_POINT('Ctrl Pts',(-30.8989435742731,-57.0165598048535,
2.81597525794847));
#32728=CARTESIAN_POINT('Ctrl Pts',(-31.2725473438504,-57.4221901848134,
2.77892929442579));
#32729=CARTESIAN_POINT('Ctrl Pts',(-31.6461511134276,-57.8278205647734,
2.74188333090311));
#32730=CARTESIAN_POINT('Ctrl Pts',(-32.24071262727,-58.0299389538838,2.70483736738043));
#32731=CARTESIAN_POINT('Ctrl Pts',(-32.7841274371744,-57.9360447252789,
2.66779140385775));
#32732=CARTESIAN_POINT('Ctrl Pts',(-32.9761488965038,-57.9028661911818,
2.6547008147751));
#32733=CARTESIAN_POINT('Ctrl Pts',(-33.1617839833806,-57.8327263930767,
2.64161022569244));
#32734=CARTESIAN_POINT('Ctrl Pts',(-33.3310924906901,-57.7334985910042,
2.62851963660979));
#32735=CARTESIAN_POINT('Origin',(-32.5,-56.2916512459885,3.));
#32736=CARTESIAN_POINT('',(-33.3331879029845,-57.7323621350135,1.92851963660978));
#32737=CARTESIAN_POINT('',(-33.3348622165511,-57.7357255517676,2.12148036339021));
#32738=CARTESIAN_POINT('',(-33.333,-57.7344495686934,3.));
#32739=CARTESIAN_POINT('Ctrl Pts',(-33.3348622165511,-57.7357255517676,
2.12148036339021));
#32740=CARTESIAN_POINT('Ctrl Pts',(-32.9046875435881,-57.9801160523425,
2.15467714411821));
#32741=CARTESIAN_POINT('Ctrl Pts',(-32.3567184702117,-58.0261342906593,
2.18787392484621));
#32742=CARTESIAN_POINT('Ctrl Pts',(-31.8960497135599,-57.8472871542167,
2.22107070557421));
#32743=CARTESIAN_POINT('Ctrl Pts',(-31.3819661915825,-57.6477026057306,
2.25811666909689));
#32744=CARTESIAN_POINT('Ctrl Pts',(-30.9766017246916,-57.1680829785327,
2.29516263261957));
#32745=CARTESIAN_POINT('Ctrl Pts',(-30.8654736597328,-56.6279289146383,
2.33220859614225));
#32746=CARTESIAN_POINT('Ctrl Pts',(-30.7543455947739,-56.0877748507439,
2.36925455966493));
#32747=CARTESIAN_POINT('Ctrl Pts',(-30.9374539317471,-55.4870863501531,
2.40630052318761));
#32748=CARTESIAN_POINT('Ctrl Pts',(-31.3309981019417,-55.1007719112966,
2.44334648671029));
#32749=CARTESIAN_POINT('Ctrl Pts',(-31.7245422721363,-54.7144574724402,
2.48039245023297));
#32750=CARTESIAN_POINT('Ctrl Pts',(-32.3285222755522,-54.5425170953181,
2.51743841375565));
#32751=CARTESIAN_POINT('Ctrl Pts',(-32.8665232388267,-54.6636402684886,
2.55448437727833));
#32752=CARTESIAN_POINT('Ctrl Pts',(-33.4045242021011,-54.7847634416591,
2.59153034080102));
#32753=CARTESIAN_POINT('Ctrl Pts',(-33.876546125234,-55.1989501651221,2.62857630432369));
#32754=CARTESIAN_POINT('Ctrl Pts',(-34.0665654985573,-55.7166455362864,
2.66562226784638));
#32755=CARTESIAN_POINT('Ctrl Pts',(-34.2565848718806,-56.2343409074507,
2.70266823136906));
#32756=CARTESIAN_POINT('Ctrl Pts',(-34.1646016953943,-56.8555449263162,
2.73971419489174));
#32757=CARTESIAN_POINT('Ctrl Pts',(-33.8327125913974,-57.2959600511828,
2.77676015841442));
#32758=CARTESIAN_POINT('Ctrl Pts',(-33.6991654394395,-57.4731764312833,
2.79166689340635));
#32759=CARTESIAN_POINT('Ctrl Pts',(-33.5267742601986,-57.6211206345609,
2.80657362839828));
#32760=CARTESIAN_POINT('Ctrl Pts',(-33.3325882586835,-57.7320513890704,
2.82148036339021));
#32761=CARTESIAN_POINT('Ctrl Pts',(-33.3310924906901,-57.7334985910042,
2.62851963660979));
#32762=CARTESIAN_POINT('Ctrl Pts',(-33.6409218393061,-57.5519147723922,
2.60456426216976));
#32763=CARTESIAN_POINT('Ctrl Pts',(-33.8960769478414,-57.272921419479,2.58060888772973));
#32764=CARTESIAN_POINT('Ctrl Pts',(-34.0356424650284,-56.9447672654595,
2.55665351328971));
#32765=CARTESIAN_POINT('Ctrl Pts',(-34.2514745770115,-56.4372908805649,
2.51960754976703));
#32766=CARTESIAN_POINT('Ctrl Pts',(-34.190870695011,-55.8122449570956,2.48256158624435));
#32767=CARTESIAN_POINT('Ctrl Pts',(-33.8815665292719,-55.3556853061788,
2.44551562272167));
#32768=CARTESIAN_POINT('Ctrl Pts',(-33.5722623635329,-54.899125655262,2.40846965919899));
#32769=CARTESIAN_POINT('Ctrl Pts',(-33.0142579140552,-54.6110522768978,
2.37142369567631));
#32770=CARTESIAN_POINT('Ctrl Pts',(-32.4629270812427,-54.6233035861816,
2.33437773215363));
#32771=CARTESIAN_POINT('Ctrl Pts',(-31.9115962484303,-54.6355548954655,
2.29733176863094));
#32772=CARTESIAN_POINT('Ctrl Pts',(-31.3669390322832,-54.9481308923973,
2.26028580510826));
#32773=CARTESIAN_POINT('Ctrl Pts',(-31.0782208961876,-55.417979399555,2.22323984158558));
#32774=CARTESIAN_POINT('Ctrl Pts',(-30.789502760092,-55.8878279067126,2.1861938780629));
#32775=CARTESIAN_POINT('Ctrl Pts',(-30.7567237040478,-56.514948924096,2.14914791454022));
#32776=CARTESIAN_POINT('Ctrl Pts',(-30.9948852489237,-57.0123369620816,
2.11210195101754));
#32777=CARTESIAN_POINT('Ctrl Pts',(-31.2330467937995,-57.5097250000671,
2.07505598749486));
#32778=CARTESIAN_POINT('Ctrl Pts',(-31.7421489395953,-57.8773800586549,
2.03801002397218));
#32779=CARTESIAN_POINT('Ctrl Pts',(-32.2891982024822,-57.9470427155362,
2.0009640604495));
#32780=CARTESIAN_POINT('Ctrl Pts',(-32.6457882768413,-57.9924518106263,
1.9768159191696));
#32781=CARTESIAN_POINT('Ctrl Pts',(-33.018502040246,-57.9112442562479,1.95266777788969));
#32782=CARTESIAN_POINT('Ctrl Pts',(-33.3331879029845,-57.7323621350135,
1.92851963660978));
#32783=CARTESIAN_POINT('Origin',(-32.5,-56.2916512459885,3.));
#32784=CARTESIAN_POINT('',(-33.3347215376786,-57.7364302140763,1.22851963660979));
#32785=CARTESIAN_POINT('',(-33.3320718525009,-57.735759463036,1.42148036339021));
#32786=CARTESIAN_POINT('',(-33.333,-57.7344495686934,3.));
#32787=CARTESIAN_POINT('Ctrl Pts',(-33.3320718525009,-57.735759463036,1.42148036339021));
#32788=CARTESIAN_POINT('Ctrl Pts',(-33.2393317234316,-57.7904422794385,
1.42868873279278));
#32789=CARTESIAN_POINT('Ctrl Pts',(-33.1414800191062,-57.8359234203097,
1.43589710219535));
#32790=CARTESIAN_POINT('Ctrl Pts',(-33.0399483052832,-57.8706429670186,
1.44310547159792));
#32791=CARTESIAN_POINT('Ctrl Pts',(-32.5181465001006,-58.0490770883944,
1.4801514351206));
#32792=CARTESIAN_POINT('Ctrl Pts',(-31.8991468445914,-57.9432717752442,
1.51719739864328));
#32793=CARTESIAN_POINT('Ctrl Pts',(-31.4662380410665,-57.6016494290873,
1.55424336216596));
#32794=CARTESIAN_POINT('Ctrl Pts',(-31.0333292375416,-57.2600270829305,
1.59128932568864));
#32795=CARTESIAN_POINT('Ctrl Pts',(-30.7865112860008,-56.6825877037672,
1.62833528921132));
#32796=CARTESIAN_POINT('Ctrl Pts',(-30.8387418215198,-56.1335996977756,
1.665381252734));
#32797=CARTESIAN_POINT('Ctrl Pts',(-30.8909723570387,-55.5846116917841,
1.70242721625668));
#32798=CARTESIAN_POINT('Ctrl Pts',(-31.2422513796173,-55.0640750589644,
1.73947317977936));
#32799=CARTESIAN_POINT('Ctrl Pts',(-31.7318140526851,-54.8102163409698,
1.77651914330204));
#32800=CARTESIAN_POINT('Ctrl Pts',(-32.2213767257528,-54.5563576229751,
1.81356510682472));
#32801=CARTESIAN_POINT('Ctrl Pts',(-32.8492230493096,-54.5691768198056,
1.8506110703474));
#32802=CARTESIAN_POINT('Ctrl Pts',(-33.3280155932489,-54.842807153342,1.88765703387008));
#32803=CARTESIAN_POINT('Ctrl Pts',(-33.8068081371883,-55.1164374868783,
1.92470299739276));
#32804=CARTESIAN_POINT('Ctrl Pts',(-34.1365469015101,-55.6508789571206,
1.96174896091544));
#32805=CARTESIAN_POINT('Ctrl Pts',(-34.1663250709766,-56.2015413947231,
1.99879492443812));
#32806=CARTESIAN_POINT('Ctrl Pts',(-34.1961032404431,-56.7522038323256,
2.03584088796081));
#32807=CARTESIAN_POINT('Ctrl Pts',(-33.9259208150542,-57.3190872372884,
2.07288685148349));
#32808=CARTESIAN_POINT('Ctrl Pts',(-33.4794283138278,-57.6427542048827,
2.10993281500617));
#32809=CARTESIAN_POINT('Ctrl Pts',(-33.4330364511186,-57.6763841392777,
2.11378199780085));
#32810=CARTESIAN_POINT('Ctrl Pts',(-33.384741178112,-57.707388354926,2.11763118059553));
#32811=CARTESIAN_POINT('Ctrl Pts',(-33.3348622165511,-57.7357255517676,
2.12148036339021));
#32812=CARTESIAN_POINT('Ctrl Pts',(-33.3331879029845,-57.7323621350135,
1.92851963660978));
#32813=CARTESIAN_POINT('Ctrl Pts',(-33.501265531522,-57.6368189718627,1.91562181436701));
#32814=CARTESIAN_POINT('Ctrl Pts',(-33.6527891880219,-57.5134115911553,
1.90272399212423));
#32815=CARTESIAN_POINT('Ctrl Pts',(-33.7764604319637,-57.3665498834978,
1.88982616988146));
#32816=CARTESIAN_POINT('Ctrl Pts',(-34.1316770185806,-56.9447241394031,
1.85278020635878));
#32817=CARTESIAN_POINT('Ctrl Pts',(-34.2571138118367,-56.3294023960388,
1.8157342428361));
#32818=CARTESIAN_POINT('Ctrl Pts',(-34.0953639520231,-55.8021901383674,
1.77868827931342));
#32819=CARTESIAN_POINT('Ctrl Pts',(-33.9336140922095,-55.2749778806959,
1.74164231579074));
#32820=CARTESIAN_POINT('Ctrl Pts',(-33.4846775793262,-54.8358751087172,
1.70459635226806));
#32821=CARTESIAN_POINT('Ctrl Pts',(-32.9540127541378,-54.6858396959092,
1.66755038874538));
#32822=CARTESIAN_POINT('Ctrl Pts',(-32.4233479289495,-54.5358042831011,
1.63050442522269));
#32823=CARTESIAN_POINT('Ctrl Pts',(-31.8109547914561,-54.6748362294637,
1.59345846170001));
#32824=CARTESIAN_POINT('Ctrl Pts',(-31.3970985335358,-55.0393067763799,
1.55641249817733));
#32825=CARTESIAN_POINT('Ctrl Pts',(-30.9832422756156,-55.4037773232961,
1.51936653465465));
#32826=CARTESIAN_POINT('Ctrl Pts',(-30.7679228972685,-55.993686470766,1.48232057113197));
#32827=CARTESIAN_POINT('Ctrl Pts',(-30.8496825329409,-56.5390589524362,
1.44527460760929));
#32828=CARTESIAN_POINT('Ctrl Pts',(-30.9314421686133,-57.0844314341065,
1.40822864408661));
#32829=CARTESIAN_POINT('Ctrl Pts',(-31.3102808183052,-57.5852672499772,
1.37118268056393));
#32830=CARTESIAN_POINT('Ctrl Pts',(-31.8128208258201,-57.8123560489854,
1.33413671704125));
#32831=CARTESIAN_POINT('Ctrl Pts',(-32.2903969982888,-58.0281641395237,
1.29893102356409));
#32832=CARTESIAN_POINT('Ctrl Pts',(-32.8796899699103,-57.9967466454786,
1.26372533008694));
#32833=CARTESIAN_POINT('Ctrl Pts',(-33.3347215376786,-57.7364302140763,
1.22851963660979));
#32834=CARTESIAN_POINT('Origin',(-32.5,-56.2916512459885,3.));
#32835=CARTESIAN_POINT('',(-33.3315625259448,-57.7350035902351,0.528519636609785));
#32836=CARTESIAN_POINT('',(-33.3315934922345,-57.7321400761417,0.721480363390208));
#32837=CARTESIAN_POINT('',(-33.333,-57.7344495686934,3.));
#32838=CARTESIAN_POINT('Ctrl Pts',(-33.3315934922345,-57.7321400761417,
0.721480363390208));
#32839=CARTESIAN_POINT('Ctrl Pts',(-33.094172273388,-57.8693226291885,0.739746284990028));
#32840=CARTESIAN_POINT('Ctrl Pts',(-32.8247195065089,-57.9509431527902,
0.758012206589848));
#32841=CARTESIAN_POINT('Ctrl Pts',(-32.552949516444,-57.9595707213043,0.776278128189667));
#32842=CARTESIAN_POINT('Ctrl Pts',(-32.001760183703,-57.97706869351,0.813324091712348));
#32843=CARTESIAN_POINT('Ctrl Pts',(-31.4410392363067,-57.6943190569763,
0.850370055235028));
#32844=CARTESIAN_POINT('Ctrl Pts',(-31.1274037953482,-57.2407237861293,
0.887416018757709));
#32845=CARTESIAN_POINT('Ctrl Pts',(-30.8137683543896,-56.7871285152822,
0.92446198228039));
#32846=CARTESIAN_POINT('Ctrl Pts',(-30.7472184198688,-56.1626876101218,
0.96150794580307));
#32847=CARTESIAN_POINT('Ctrl Pts',(-30.9582109466765,-55.653179991732,0.998553909325751));
#32848=CARTESIAN_POINT('Ctrl Pts',(-31.1692034734841,-55.1436723733423,
1.03559987284843));
#32849=CARTESIAN_POINT('Ctrl Pts',(-31.6577384616201,-54.7490980417232,
1.07264583637111));
#32850=CARTESIAN_POINT('Ctrl Pts',(-32.2002351035856,-54.6500361771206,
1.10969179989379));
#32851=CARTESIAN_POINT('Ctrl Pts',(-32.7427317455511,-54.550974312518,1.14673776341647));
#32852=CARTESIAN_POINT('Ctrl Pts',(-33.3391900413461,-54.7474249149318,
1.18378372693915));
#32853=CARTESIAN_POINT('Ctrl Pts',(-33.7166374697497,-55.1494812522209,
1.22082969046183));
#32854=CARTESIAN_POINT('Ctrl Pts',(-34.0940848981533,-55.5515375895099,
1.25787565398451));
#32855=CARTESIAN_POINT('Ctrl Pts',(-34.2525214591656,-56.1591996616743,
1.2949216175072));
#32856=CARTESIAN_POINT('Ctrl Pts',(-34.1194377622437,-56.6943674757075,
1.33196758102988));
#32857=CARTESIAN_POINT('Ctrl Pts',(-34.0122493682821,-57.1254028302473,
1.36180517514999));
#32858=CARTESIAN_POINT('Ctrl Pts',(-33.7159509484902,-57.5094109520148,
1.3916427692701));
#32859=CARTESIAN_POINT('Ctrl Pts',(-33.3320718525009,-57.735759463036,1.42148036339021));
#32860=CARTESIAN_POINT('Ctrl Pts',(-33.3347215376786,-57.7364302140763,
1.22851963660979));
#32861=CARTESIAN_POINT('Ctrl Pts',(-33.3585069224055,-57.7228229680956,
1.22667936656426));
#32862=CARTESIAN_POINT('Ctrl Pts',(-33.3819254571596,-57.7085902886951,
1.22483909651873));
#32863=CARTESIAN_POINT('Ctrl Pts',(-33.4049420099643,-57.6937347933887,
1.22299882647321));
#32864=CARTESIAN_POINT('Ctrl Pts',(-33.8682818212557,-57.394682956638,1.18595286295053));
#32865=CARTESIAN_POINT('Ctrl Pts',(-34.1687200785007,-56.8432375009908,
1.14890689942785));
#32866=CARTESIAN_POINT('Ctrl Pts',(-34.1687595096553,-56.2917705661426,
1.11186093590517));
#32867=CARTESIAN_POINT('Ctrl Pts',(-34.1687989408099,-55.7403036312943,
1.07481497238249));
#32868=CARTESIAN_POINT('Ctrl Pts',(-33.8684395458741,-55.188815217245,1.03776900885981));
#32869=CARTESIAN_POINT('Ctrl Pts',(-33.4051425051238,-54.8896971238163,
1.00072304533712));
#32870=CARTESIAN_POINT('Ctrl Pts',(-32.9418454643735,-54.5905790303876,
0.963677081814444));
#32871=CARTESIAN_POINT('Ctrl Pts',(-32.3156107778087,-54.5438312575796,
0.926631118291762));
#32872=CARTESIAN_POINT('Ctrl Pts',(-31.8130383006683,-54.7708481887354,
0.889585154769081));
#32873=CARTESIAN_POINT('Ctrl Pts',(-31.310465823528,-54.9978651198912,0.8525391912464));
#32874=CARTESIAN_POINT('Ctrl Pts',(-30.9315555558122,-55.4986467550108,
0.815493227723721));
#32875=CARTESIAN_POINT('Ctrl Pts',(-30.8497179302269,-56.0440075390777,
0.778447264201041));
#32876=CARTESIAN_POINT('Ctrl Pts',(-30.7678803046417,-56.5893683231447,
0.74140130067836));
#32877=CARTESIAN_POINT('Ctrl Pts',(-30.9831153211871,-57.179308256159,0.704355337155679));
#32878=CARTESIAN_POINT('Ctrl Pts',(-31.3969194538394,-57.5438379827469,
0.667309373632999));
#32879=CARTESIAN_POINT('Ctrl Pts',(-31.8107235864918,-57.9083677093349,
0.630263410110318));
#32880=CARTESIAN_POINT('Ctrl Pts',(-32.4230968352511,-58.0474872294965,
0.593217446587637));
#32881=CARTESIAN_POINT('Ctrl Pts',(-32.9537831109001,-57.8975277056554,
0.556171483064956));
#32882=CARTESIAN_POINT('Ctrl Pts',(-33.0858213863713,-57.860216778603,0.546954200913232));
#32883=CARTESIAN_POINT('Ctrl Pts',(-33.2128028501901,-57.805010485588,0.537736918761509));
#32884=CARTESIAN_POINT('Ctrl Pts',(-33.3315625259448,-57.7350035902351,
0.528519636609785));
#32885=CARTESIAN_POINT('Origin',(-32.5,-56.2916512459885,3.));
#32886=CARTESIAN_POINT('',(-33.332066590478,-57.7319806121586,-0.171480363390217));
#32887=CARTESIAN_POINT('',(-33.3345107245666,-57.7340829700271,0.0214803633902086));
#32888=CARTESIAN_POINT('',(-33.333,-57.7344495686934,3.));
#32889=CARTESIAN_POINT('Ctrl Pts',(-33.3345107245666,-57.7340829700271,
0.0214803633902086));
#32890=CARTESIAN_POINT('Ctrl Pts',(-32.9530815922347,-57.9496325625699,
0.0508038371872777));
#32891=CARTESIAN_POINT('Ctrl Pts',(-32.4824461880261,-58.016467684898,0.0801273109843468));
#32892=CARTESIAN_POINT('Ctrl Pts',(-32.0612908438827,-57.9017112764627,
0.109450784781416));
#32893=CARTESIAN_POINT('Ctrl Pts',(-31.5292220438324,-57.7567331694926,
0.146496748304096));
#32894=CARTESIAN_POINT('Ctrl Pts',(-31.0761267049974,-57.3219229222043,
0.183542711826777));
#32895=CARTESIAN_POINT('Ctrl Pts',(-30.9093664792402,-56.796273907743,0.220588675349458));
#32896=CARTESIAN_POINT('Ctrl Pts',(-30.7426062534831,-56.2706248932817,
0.257634638872138));
#32897=CARTESIAN_POINT('Ctrl Pts',(-30.8621811408039,-55.6541371116475,
0.294680602394819));
#32898=CARTESIAN_POINT('Ctrl Pts',(-31.2133670155729,-55.2289496928674,
0.3317265659175));
#32899=CARTESIAN_POINT('Ctrl Pts',(-31.564552890342,-54.8037622740873,0.36877252944018));
#32900=CARTESIAN_POINT('Ctrl Pts',(-32.1473497525593,-54.5698752181613,
0.405818492962861));
#32901=CARTESIAN_POINT('Ctrl Pts',(-32.6950373137549,-54.6343282619421,
0.442864456485541));
#32902=CARTESIAN_POINT('Ctrl Pts',(-33.2427248749505,-54.6987813057228,
0.479910420008222));
#32903=CARTESIAN_POINT('Ctrl Pts',(-33.7553031351243,-55.0615744492104,
0.516956383530902));
#32904=CARTESIAN_POINT('Ctrl Pts',(-33.9981877468876,-55.5566733533727,
0.554002347053583));
#32905=CARTESIAN_POINT('Ctrl Pts',(-34.2410723586509,-56.0517722575349,
0.591048310576264));
#32906=CARTESIAN_POINT('Ctrl Pts',(-34.2142633220036,-56.6791769223718,
0.628094274098944));
#32907=CARTESIAN_POINT('Ctrl Pts',(-33.9300299446371,-57.1517520452627,
0.665140237621625));
#32908=CARTESIAN_POINT('Ctrl Pts',(-33.7859409742004,-57.3913187827875,
0.683920279544486));
#32909=CARTESIAN_POINT('Ctrl Pts',(-33.5756972687095,-57.5910963251749,
0.702700321467347));
#32910=CARTESIAN_POINT('Ctrl Pts',(-33.3315934922345,-57.7321400761417,
0.721480363390208));
#32911=CARTESIAN_POINT('Ctrl Pts',(-33.3315625259448,-57.7350035902351,
0.528519636609785));
#32912=CARTESIAN_POINT('Ctrl Pts',(-33.6901199750816,-57.523639811577,0.500690955238828));
#32913=CARTESIAN_POINT('Ctrl Pts',(-33.9737318881584,-57.1773614538061,
0.472862273867871));
#32914=CARTESIAN_POINT('Ctrl Pts',(-34.0952939407749,-56.781340492839,0.445033592496915));
#32915=CARTESIAN_POINT('Ctrl Pts',(-34.2571191924618,-56.2541513717075,
0.407987628974234));
#32916=CARTESIAN_POINT('Ctrl Pts',(-34.131770393297,-55.6388116972881,0.370941665451553));
#32917=CARTESIAN_POINT('Ctrl Pts',(-33.7766141338562,-55.2169351595517,
0.333895701928873));
#32918=CARTESIAN_POINT('Ctrl Pts',(-33.4214578744155,-54.7950586218153,
0.296849738406192));
#32919=CARTESIAN_POINT('Ctrl Pts',(-32.8364941546989,-54.566645220762,0.259803774883511));
#32920=CARTESIAN_POINT('Ctrl Pts',(-32.289434934298,-54.636229647045,0.222757811360831));
#32921=CARTESIAN_POINT('Ctrl Pts',(-31.7423757138972,-54.705814073328,0.18571184783815));
#32922=CARTESIAN_POINT('Ctrl Pts',(-31.2332209928121,-55.0733963269474,
0.148665884315469));
#32923=CARTESIAN_POINT('Ctrl Pts',(-30.9949883236289,-55.5707503002861,
0.111619920792788));
#32924=CARTESIAN_POINT('Ctrl Pts',(-30.7567556544457,-56.0681042736247,
0.0745739572701072));
#32925=CARTESIAN_POINT('Ctrl Pts',(-30.7894450371644,-56.6952299666827,
0.0375279937474265));
#32926=CARTESIAN_POINT('Ctrl Pts',(-31.0780959757366,-57.1651197597709,
0.000482030224745822));
#32927=CARTESIAN_POINT('Ctrl Pts',(-31.3667469143089,-57.635009552859,-0.0365639332979349));
#32928=CARTESIAN_POINT('Ctrl Pts',(-31.9113594087348,-57.9476634459773,
-0.0736098968206155));
#32929=CARTESIAN_POINT('Ctrl Pts',(-32.4626884920092,-57.9599935925982,
-0.110655860343296));
#32930=CARTESIAN_POINT('Ctrl Pts',(-32.7644246265901,-57.9667417415587,
-0.13093069469227));
#32931=CARTESIAN_POINT('Ctrl Pts',(-33.0681725463472,-57.8835354694765,
-0.151205529041244));
#32932=CARTESIAN_POINT('Ctrl Pts',(-33.332066590478,-57.7319806121586,-0.171480363390217));
#32933=CARTESIAN_POINT('Origin',(-32.5,-56.2916512459885,3.));
#32934=CARTESIAN_POINT('',(-33.3347877909359,-57.7349452754743,-0.871480363390215));
#32935=CARTESIAN_POINT('',(-33.333352483612,-57.7367881187288,-0.678519636609791));
#32936=CARTESIAN_POINT('',(-33.333,-57.7344495686934,3.));
#32937=CARTESIAN_POINT('Ctrl Pts',(-33.333352483612,-57.7367881187288,-0.678519636609791));
#32938=CARTESIAN_POINT('Ctrl Pts',(-33.2904764567157,-57.7619047682302,
-0.675184574138153));
#32939=CARTESIAN_POINT('Ctrl Pts',(-33.2464522145773,-57.7849807415505,
-0.671849511666514));
#32940=CARTESIAN_POINT('Ctrl Pts',(-33.2014046817541,-57.8058476261432,
-0.668514449194876));
#32941=CARTESIAN_POINT('Ctrl Pts',(-32.701015477069,-58.0376375407332,-0.631468485672195));
#32942=CARTESIAN_POINT('Ctrl Pts',(-32.0743642145055,-57.9968518393257,
-0.594422522149515));
#32943=CARTESIAN_POINT('Ctrl Pts',(-31.608241296104,-57.7021565859588,-0.557376558626834));
#32944=CARTESIAN_POINT('Ctrl Pts',(-31.1421183777026,-57.407461332592,-0.520330595104154));
#32945=CARTESIAN_POINT('Ctrl Pts',(-30.8365238034633,-56.8588565272658,
-0.483284631581473));
#32946=CARTESIAN_POINT('Ctrl Pts',(-30.8313147141679,-56.3074141411014,
-0.446238668058792));
#32947=CARTESIAN_POINT('Ctrl Pts',(-30.8261056248724,-55.755971754937,-0.409192704536112));
#32948=CARTESIAN_POINT('Ctrl Pts',(-31.1212820205207,-55.2016917879344,
-0.372146741013431));
#32949=CARTESIAN_POINT('Ctrl Pts',(-31.5817547242443,-54.8982436746824,
-0.335100777490751));
#32950=CARTESIAN_POINT('Ctrl Pts',(-32.042227427968,-54.5947955614304,-0.29805481396807));
#32951=CARTESIAN_POINT('Ctrl Pts',(-32.667996439767,-54.5421793019291,-0.26100885044539));
#32952=CARTESIAN_POINT('Ctrl Pts',(-33.1726750359156,-54.7644749931934,
-0.223962886922709));
#32953=CARTESIAN_POINT('Ctrl Pts',(-33.6773536320643,-54.9867706844577,
-0.186916923400029));
#32954=CARTESIAN_POINT('Ctrl Pts',(-34.0609418125626,-55.4839783264877,
-0.149870959877348));
#32955=CARTESIAN_POINT('Ctrl Pts',(-34.1478882650458,-56.0285480388725,
-0.112824996354667));
#32956=CARTESIAN_POINT('Ctrl Pts',(-34.2348347175289,-56.5731177512574,
-0.0757790328319867));
#32957=CARTESIAN_POINT('Ctrl Pts',(-34.0251394419968,-57.1650495339971,
-0.038733069309306));
#32958=CARTESIAN_POINT('Ctrl Pts',(-33.6147706735979,-57.533442442041,-0.00168710578662554));
#32959=CARTESIAN_POINT('Ctrl Pts',(-33.529226438914,-57.6102365155873,0.00603538393898582));
#32960=CARTESIAN_POINT('Ctrl Pts',(-33.4349620754491,-57.6773168608924,
0.0137578736645972));
#32961=CARTESIAN_POINT('Ctrl Pts',(-33.3345107245666,-57.7340829700271,
0.0214803633902086));
#32962=CARTESIAN_POINT('Ctrl Pts',(-33.332066590478,-57.7319806121586,-0.171480363390217));
#32963=CARTESIAN_POINT('Ctrl Pts',(-33.550356960999,-57.6066160323434,-0.188251492563924));
#32964=CARTESIAN_POINT('Ctrl Pts',(-33.7413776202382,-57.4344844529175,
-0.205022621737631));
#32965=CARTESIAN_POINT('Ctrl Pts',(-33.8814326840108,-57.2278147357495,
-0.221793750911338));
#32966=CARTESIAN_POINT('Ctrl Pts',(-34.1908021206152,-56.7712993321565,
-0.258839714434018));
#32967=CARTESIAN_POINT('Ctrl Pts',(-34.251495321701,-56.1462621248468,-0.295885677956699));
#32968=CARTESIAN_POINT('Ctrl Pts',(-34.0357358154562,-55.6387548587911,
-0.332931641479379));
#32969=CARTESIAN_POINT('Ctrl Pts',(-33.8199763092115,-55.1312475927354,
-0.36997760500206));
#32970=CARTESIAN_POINT('Ctrl Pts',(-33.3277640956362,-54.7412702679336,
-0.40702356852474));
#32971=CARTESIAN_POINT('Ctrl Pts',(-32.7843626547692,-54.6472983719835,
-0.444069532047421));
#32972=CARTESIAN_POINT('Ctrl Pts',(-32.2409612139021,-54.5533264760334,
-0.481115495570101));
#32973=CARTESIAN_POINT('Ctrl Pts',(-31.6463705457434,-54.7553600089348,
-0.518161459092782));
#32974=CARTESIAN_POINT('Ctrl Pts',(-31.2727089000175,-55.1609368730463,
-0.555207422615462));
#32975=CARTESIAN_POINT('Ctrl Pts',(-30.8990472542916,-55.5665137371577,
-0.592253386138142));
#32976=CARTESIAN_POINT('Ctrl Pts',(-30.7463146309986,-56.1756339324792,
-0.629299349660823));
#32977=CARTESIAN_POINT('Ctrl Pts',(-30.8844090678351,-56.7095307561729,
-0.666345313183503));
#32978=CARTESIAN_POINT('Ctrl Pts',(-31.0225035046717,-57.2434275798666,
-0.703391276706184));
#32979=CARTESIAN_POINT('Ctrl Pts',(-31.4514250016378,-57.7021010319326,
-0.740437240228864));
#32980=CARTESIAN_POINT('Ctrl Pts',(-31.9748770216297,-57.8756353949644,
-0.777483203751545));
#32981=CARTESIAN_POINT('Ctrl Pts',(-32.4175973471179,-58.0224056561358,
-0.808815590297768));
#32982=CARTESIAN_POINT('Ctrl Pts',(-32.9279379927888,-57.9652079725634,
-0.840147976843991));
#32983=CARTESIAN_POINT('Ctrl Pts',(-33.3347877909359,-57.7349452754743,
-0.871480363390215));
#32984=CARTESIAN_POINT('Origin',(-32.5,-56.2916512459885,3.));
#32985=CARTESIAN_POINT('',(-33.3326856027611,-57.7363329907929,-1.57148036339021));
#32986=CARTESIAN_POINT('',(-33.3311039683456,-57.7330494773494,-1.37851963660979));
#32987=CARTESIAN_POINT('',(-33.333,-57.7344495686934,3.));
#32988=CARTESIAN_POINT('',(-30.9307125467393,-55.7322829513575,-2.));
#32989=CARTESIAN_POINT('Ctrl Pts',(-33.3326856027611,-57.7363329907929,
-1.57148036339021));
#32990=CARTESIAN_POINT('Ctrl Pts',(-33.7401458440335,-57.496539311517,-1.6031823516921));
#32991=CARTESIAN_POINT('Ctrl Pts',(-34.0466143999381,-57.0758524794489,
-1.63488433999399));
#32992=CARTESIAN_POINT('Ctrl Pts',(-34.1374824480444,-56.6126749242947,
-1.66658632829588));
#32993=CARTESIAN_POINT('Ctrl Pts',(-34.243668040048,-56.0714199515982,-1.70363229181856));
#32994=CARTESIAN_POINT('Ctrl Pts',(-34.0554395585675,-55.472141614315,-1.74067825534124));
#32995=CARTESIAN_POINT('Ctrl Pts',(-33.6580205398159,-55.0897022763625,
-1.77772421886392));
#32996=CARTESIAN_POINT('Ctrl Pts',(-33.2606015210643,-54.70726293841,-1.8147701823866));
#32997=CARTESIAN_POINT('Ctrl Pts',(-32.6539919650415,-54.5416625997882,
-1.85181614590928));
#32998=CARTESIAN_POINT('Ctrl Pts',(-32.1180205379334,-54.6674612497455,
-1.88886210943196));
#32999=CARTESIAN_POINT('Ctrl Pts',(-31.5820491108253,-54.7932598997029,
-1.92590807295464));
#33000=CARTESIAN_POINT('Ctrl Pts',(-31.116715812632,-55.2104575382394,-1.96295403647732));
#33001=CARTESIAN_POINT('Ctrl Pts',(-30.9307125467393,-55.7322829513575,
-2.));
#33002=CARTESIAN_POINT('',(-32.1993827818329,-57.933381219007,-2.));
#33003=CARTESIAN_POINT('Origin',(-32.5,-56.2916512459885,-2.));
#33004=CARTESIAN_POINT('Ctrl Pts',(-32.1993825459688,-57.9333829869217,
-2.));
#33005=CARTESIAN_POINT('Ctrl Pts',(-31.6675596070897,-57.835293698039,-1.96367708181444));
#33006=CARTESIAN_POINT('Ctrl Pts',(-31.1868214355218,-57.454698369386,-1.92735416362889));
#33007=CARTESIAN_POINT('Ctrl Pts',(-30.9706018866113,-56.9589951265537,
-1.89103124544334));
#33008=CARTESIAN_POINT('Ctrl Pts',(-30.7500782634566,-56.4534243968501,
-1.85398528192066));
#33009=CARTESIAN_POINT('Ctrl Pts',(-30.8047091132838,-55.8281174567283,
-1.81693931839798));
#33010=CARTESIAN_POINT('Ctrl Pts',(-31.1096921022324,-55.3687479433185,
-1.77989335487529));
#33011=CARTESIAN_POINT('Ctrl Pts',(-31.4146750911809,-54.9093784299087,
-1.74284739135261));
#33012=CARTESIAN_POINT('Ctrl Pts',(-31.9700102192507,-54.6159463432109,
-1.70580142782993));
#33013=CARTESIAN_POINT('Ctrl Pts',(-32.521445594378,-54.6229937951642,-1.66875546430725));
#33014=CARTESIAN_POINT('Ctrl Pts',(-33.0728809695053,-54.6300412471175,
-1.63170950078457));
#33015=CARTESIAN_POINT('Ctrl Pts',(-33.62041659169,-54.9375682377219,-1.59466353726189));
#33016=CARTESIAN_POINT('Ctrl Pts',(-33.9135196580233,-55.4047071572134,
-1.55761757373921));
#33017=CARTESIAN_POINT('Ctrl Pts',(-34.2066227243565,-55.8718460767048,
-1.52057161021653));
#33018=CARTESIAN_POINT('Ctrl Pts',(-34.2452932348383,-56.4985969250833,
-1.48352564669385));
#33019=CARTESIAN_POINT('Ctrl Pts',(-34.0118083132187,-56.9981869719763,
-1.44647968317117));
#33020=CARTESIAN_POINT('Ctrl Pts',(-33.869033908706,-57.3036828084989,-1.42382633431738));
#33021=CARTESIAN_POINT('Ctrl Pts',(-33.6244941277174,-57.5616302028088,
-1.40117298546358));
#33022=CARTESIAN_POINT('Ctrl Pts',(-33.3311039683456,-57.7330494773494,
-1.37851963660979));
#33023=CARTESIAN_POINT('Origin',(-32.5,-56.2916512459885,-3.54592528053767));
#33024=CARTESIAN_POINT('',(-33.5275749112977,-58.0738535198176,6.54592528053768));
#33025=CARTESIAN_POINT('',(-33.5264962288792,-58.0679896197986,6.60407471946233));
#33026=CARTESIAN_POINT('',(-33.5273749999999,-58.0711169444146,-3.54592528053767));
#33027=CARTESIAN_POINT('',(-32.2716262263503,-54.2496319067047,7.));
#33028=CARTESIAN_POINT('Ctrl Pts',(-33.5264962288792,-58.0679896197986,
6.60407471946233));
#33029=CARTESIAN_POINT('Ctrl Pts',(-33.1919689183208,-58.2597658075907,
6.62491192240684));
#33030=CARTESIAN_POINT('Ctrl Pts',(-32.1179432461624,-58.5451601991561,
6.68279508887404));
#33031=CARTESIAN_POINT('Ctrl Pts',(-30.4105200538552,-57.5324032730232,
6.77772421886391));
#33032=CARTESIAN_POINT('Ctrl Pts',(-30.3280193568976,-55.2072605605051,
6.88886210943196));
#33033=CARTESIAN_POINT('Ctrl Pts',(-31.592606214368,-54.3255716196824,6.96295403647732));
#33034=CARTESIAN_POINT('Ctrl Pts',(-32.2716262263503,-54.2496319067047,
7.));
#33035=CARTESIAN_POINT('',(-33.3217794842373,-54.4043178444011,6.99999999999999));
#33036=CARTESIAN_POINT('Origin',(-32.5,-56.2916512459885,7.));
#33037=CARTESIAN_POINT('Ctrl Pts',(-33.5275749112977,-58.0738535198176,
6.54592528053768));
#33038=CARTESIAN_POINT('Ctrl Pts',(-33.4657840639227,-58.1101089614272,
6.54982271160486));
#33039=CARTESIAN_POINT('Ctrl Pts',(-32.7965074863137,-58.455071838418,6.59076610619472));
#33040=CARTESIAN_POINT('Ctrl Pts',(-31.1711925871668,-58.3247407101007,
6.66875546430726));
#33041=CARTESIAN_POINT('Ctrl Pts',(-30.0714699489351,-56.2774508415845,
6.7798933548753));
#33042=CARTESIAN_POINT('Ctrl Pts',(-31.1870202472961,-54.2576863817542,
6.89030820010621));
#33043=CARTESIAN_POINT('Ctrl Pts',(-32.7099100739971,-54.1388320417446,
6.96367708181444));
#33044=CARTESIAN_POINT('Ctrl Pts',(-33.3217804591137,-54.4043158724519,
6.99999999999999));
#33045=CARTESIAN_POINT('Origin',(-32.5,-56.2916512459885,-3.54592528053767));
#33046=CARTESIAN_POINT('',(-33.5250713804254,-58.0691800125914,5.84592528053768));
#33047=CARTESIAN_POINT('',(-33.5296302847681,-58.0720277053709,5.90407471946233));
#33048=CARTESIAN_POINT('',(-33.5273749999999,-58.0711169444146,-3.54592528053767));
#33049=CARTESIAN_POINT('Ctrl Pts',(-33.5296302847681,-58.0720277053709,
5.90407471946233));
#33050=CARTESIAN_POINT('Ctrl Pts',(-33.0191355770127,-58.3612066004053,
5.93596947460409));
#33051=CARTESIAN_POINT('Ctrl Pts',(-31.6285851526934,-58.5053110361567,
6.00491019326854));
#33052=CARTESIAN_POINT('Ctrl Pts',(-30.1397737216657,-56.8641588006487,
6.11089687545567));
#33053=CARTESIAN_POINT('Ctrl Pts',(-30.7390063155881,-54.6191619749281,
6.2220347660237));
#33054=CARTESIAN_POINT('Ctrl Pts',(-32.9499730445898,-53.9051289476276,
6.33317265659175));
#33055=CARTESIAN_POINT('Ctrl Pts',(-34.7493198838486,-55.3752771327861,
6.44431054715979));
#33056=CARTESIAN_POINT('Ctrl Pts',(-34.5380916131597,-57.2516667239215,
6.53461123478332));
#33057=CARTESIAN_POINT('Ctrl Pts',(-33.7867170031423,-57.9188115213373,
6.58786595888416));
#33058=CARTESIAN_POINT('Ctrl Pts',(-33.5264962288792,-58.0679896197986,
6.60407471946233));
#33059=CARTESIAN_POINT('Ctrl Pts',(-33.5250713804254,-58.0691800125914,
5.84592528053768));
#33060=CARTESIAN_POINT('Ctrl Pts',(-33.2860537216367,-58.2086221814904,
5.86088026380211));
#33061=CARTESIAN_POINT('Ctrl Pts',(-32.3636248873145,-58.5321674493612,
5.91288121058921));
#33062=CARTESIAN_POINT('Ctrl Pts',(-30.6332940299706,-57.8452774805725,
6.00192812089901));
#33063=CARTESIAN_POINT('Ctrl Pts',(-30.1823177935136,-55.5659199366928,
6.11306601146705));
#33064=CARTESIAN_POINT('Ctrl Pts',(-31.8527378172474,-53.9508533596396,
6.22420390203509));
#33065=CARTESIAN_POINT('Ctrl Pts',(-34.1156133119216,-54.4783040835128,
6.33534179260312));
#33066=CARTESIAN_POINT('Ctrl Pts',(-34.8721855502189,-56.5889092129518,
6.442582252104));
#33067=CARTESIAN_POINT('Ctrl Pts',(-34.0531200394491,-57.7654927913865,
6.51277674808218));
#33068=CARTESIAN_POINT('Ctrl Pts',(-33.5275749112977,-58.0738535198176,
6.54592528053768));
#33069=CARTESIAN_POINT('Origin',(-32.5,-56.2916512459885,-3.54592528053767));
#33070=CARTESIAN_POINT('',(-33.5282754020984,-58.069145943353,5.14592528053768));
#33071=CARTESIAN_POINT('',(-33.5267258804522,-58.0732604370279,5.20407471946232));
#33072=CARTESIAN_POINT('',(-33.5273749999999,-58.0711169444146,-3.54592528053767));
#33073=CARTESIAN_POINT('Ctrl Pts',(-33.5267258804522,-58.0732604370279,
5.20407471946232));
#33074=CARTESIAN_POINT('Ctrl Pts',(-33.4330630138881,-58.1284275812183,
5.20998106327866));
#33075=CARTESIAN_POINT('Ctrl Pts',(-32.7207180221807,-58.473569466158,5.25293337061767));
#33076=CARTESIAN_POINT('Ctrl Pts',(-31.0632581782874,-58.2497382420229,
5.33293164147938));
#33077=CARTESIAN_POINT('Ctrl Pts',(-30.0756916068807,-56.1465211293305,
5.44406953204741));
#33078=CARTESIAN_POINT('Ctrl Pts',(-31.3071229976034,-54.1761423261723,
5.55520742261546));
#33079=CARTESIAN_POINT('Ctrl Pts',(-33.6304062534726,-54.1421146842281,
5.66634531318349));
#33080=CARTESIAN_POINT('Ctrl Pts',(-34.9190197935987,-56.0755785414895,
5.77748320375154));
#33081=CARTESIAN_POINT('Ctrl Pts',(-34.2590870859834,-57.5951911211838,
5.85672633917782));
#33082=CARTESIAN_POINT('Ctrl Pts',(-33.6120784680294,-58.0253234512995,
5.89892351108141));
#33083=CARTESIAN_POINT('Ctrl Pts',(-33.5296302847681,-58.0720277053709,
5.90407471946233));
#33084=CARTESIAN_POINT('Ctrl Pts',(-33.5282754020984,-58.069145943353,5.14592528053768));
#33085=CARTESIAN_POINT('Ctrl Pts',(-33.1102767098287,-58.3059329434062,
5.17193781599936));
#33086=CARTESIAN_POINT('Ctrl Pts',(-31.8926982278611,-58.5381488249037,
5.23499631498372));
#33087=CARTESIAN_POINT('Ctrl Pts',(-30.2596385516872,-57.2292625110704,
5.33510077749076));
#33088=CARTESIAN_POINT('Ctrl Pts',(-30.4972127153845,-54.9179054771162,
5.44623866805879));
#33089=CARTESIAN_POINT('Ctrl Pts',(-32.5679607208419,-53.8639538597436,
5.55737655862685));
#33090=CARTESIAN_POINT('Ctrl Pts',(-34.5765036531329,-55.0321005249753,
5.66851444919488));
#33091=CARTESIAN_POINT('Ctrl Pts',(-34.6698803007257,-57.0408062963268,
5.7646973564985));
#33092=CARTESIAN_POINT('Ctrl Pts',(-33.878139938799,-57.8632008987502,5.82383430027943));
#33093=CARTESIAN_POINT('Ctrl Pts',(-33.5250713804254,-58.0691800125914,
5.84592528053768));
#33094=CARTESIAN_POINT('Origin',(-32.5,-56.2916512459885,-3.54592528053767));
#33095=CARTESIAN_POINT('',(-33.5290696646583,-58.0740687441032,4.44592528053768));
#33096=CARTESIAN_POINT('',(-33.5253496165875,-58.0685468270268,4.50407471946233));
#33097=CARTESIAN_POINT('',(-33.5273749999999,-58.0711169444146,-3.54592528053767));
#33098=CARTESIAN_POINT('Ctrl Pts',(-33.5253496165874,-58.0685468270268,
4.50407471946233));
#33099=CARTESIAN_POINT('Ctrl Pts',(-33.2536996405186,-58.2261242815538,
4.52103861547591));
#33100=CARTESIAN_POINT('Ctrl Pts',(-32.2808222041073,-58.5391009797129,
4.57504847501218));
#33101=CARTESIAN_POINT('Ctrl Pts',(-30.5520219543112,-57.7420698681824,
4.66610429807112));
#33102=CARTESIAN_POINT('Ctrl Pts',(-30.2249467851584,-55.4416715145514,
4.77724218863917));
#33103=CARTESIAN_POINT('Ctrl Pts',(-31.9802536404281,-53.9192692335435,
4.8883800792072));
#33104=CARTESIAN_POINT('Ctrl Pts',(-34.2112902010514,-54.5683351429997,
4.99951796977525));
#33105=CARTESIAN_POINT('Ctrl Pts',(-34.8406399092008,-56.6764493817394,
5.10474951652696));
#33106=CARTESIAN_POINT('Ctrl Pts',(-34.0205383194344,-57.7824064089199,
5.17293509975598));
#33107=CARTESIAN_POINT('Ctrl Pts',(-33.5267258804522,-58.0732604370279,
5.20407471946232));
#33108=CARTESIAN_POINT('Ctrl Pts',(-33.529069656232,-58.0740687294261,4.44592528053768));
#33109=CARTESIAN_POINT('Ctrl Pts',(-33.5286860990811,-58.0742902067967,
4.44594940467393));
#33110=CARTESIAN_POINT('Ctrl Pts',(-32.9391765838663,-58.414411936218,4.48301949233286));
#33111=CARTESIAN_POINT('Ctrl Pts',(-31.3901016278141,-58.451850257884,4.55713554351447));
#33112=CARTESIAN_POINT('Ctrl Pts',(-30.0831480764379,-56.5307348090517,
4.6682734340825));
#33113=CARTESIAN_POINT('Ctrl Pts',(-30.9883665002518,-54.3907834608548,
4.77941132465055));
#33114=CARTESIAN_POINT('Ctrl Pts',(-33.2772002083032,-53.990717959075,4.89054921521859));
#33115=CARTESIAN_POINT('Ctrl Pts',(-34.8546537539781,-55.6967227784588,
5.00168710578663));
#33116=CARTESIAN_POINT('Ctrl Pts',(-34.4121009342633,-57.4205168337107,
5.08681246089299));
#33117=CARTESIAN_POINT('Ctrl Pts',(-33.705572940339,-57.9687108152697,5.13489185247668));
#33118=CARTESIAN_POINT('Ctrl Pts',(-33.5282754020984,-58.069145943353,5.14592528053768));
#33119=CARTESIAN_POINT('Origin',(-32.5,-56.2916512459885,-3.54592528053767));
#33120=CARTESIAN_POINT('',(-33.5252102943906,-58.0708877004567,3.74592528053768));
#33121=CARTESIAN_POINT('',(-33.5289081309377,-58.0700145843707,3.80407471946232));
#33122=CARTESIAN_POINT('',(-33.5273749999999,-58.0711169444146,-3.54592528053767));
#33123=CARTESIAN_POINT('Ctrl Pts',(-33.5289081309377,-58.0700145843707,
3.80407471946232));
#33124=CARTESIAN_POINT('Ctrl Pts',(-33.0789876682099,-58.3243434135938,
3.83209616767316));
#33125=CARTESIAN_POINT('Ctrl Pts',(-31.8034240249953,-58.5300263366319,
3.89716357940668));
#33126=CARTESIAN_POINT('Ctrl Pts',(-30.2122199456457,-57.106755585101,3.99927695466286));
#33127=CARTESIAN_POINT('Ctrl Pts',(-30.5744204047746,-54.811625609896,4.11041484523092));
#33128=CARTESIAN_POINT('Ctrl Pts',(-32.6991257052286,-53.8711798837978,
4.22155273579895));
#33129=CARTESIAN_POINT('Ctrl Pts',(-34.6415689889353,-55.1462190460047,
4.332690626367));
#33130=CARTESIAN_POINT('Ctrl Pts',(-34.6265206091307,-57.1150354081818,
4.42686462092145));
#33131=CARTESIAN_POINT('Ctrl Pts',(-33.8469321795724,-57.8820047097448,
4.48399265195323));
#33132=CARTESIAN_POINT('Ctrl Pts',(-33.5253496165874,-58.0685468270268,
4.50407471946233));
#33133=CARTESIAN_POINT('Ctrl Pts',(-33.5252102943906,-58.0708877004567,
3.74592528053768));
#33134=CARTESIAN_POINT('Ctrl Pts',(-33.3488056811853,-58.174663668992,3.75700695687117));
#33135=CARTESIAN_POINT('Ctrl Pts',(-32.5196622305249,-58.5123107269966,
3.80513459672735));
#33136=CARTESIAN_POINT('Ctrl Pts',(-30.8051884955116,-58.0311765069792,
3.89030820010621));
#33137=CARTESIAN_POINT('Ctrl Pts',(-30.1193554633367,-55.8111663248381,
4.00144609067426));
#33138=CARTESIAN_POINT('Ctrl Pts',(-31.6125533739246,-54.0309494400522,
4.11258398124229));
#33139=CARTESIAN_POINT('Ctrl Pts',(-33.9180412456697,-54.3199785564283,
4.22372187181034));
#33140=CARTESIAN_POINT('Ctrl Pts',(-34.9253611823253,-56.4132475717748,
4.33483563824213));
#33141=CARTESIAN_POINT('Ctrl Pts',(-34.1176914037626,-57.7341809275558,
4.40890344115124));
#33142=CARTESIAN_POINT('Ctrl Pts',(-33.529069656232,-58.0740687294261,4.44592528053768));
#33143=CARTESIAN_POINT('Origin',(-32.5,-56.2916512459885,-3.54592528053767));
#33144=CARTESIAN_POINT('',(-33.5268671815904,-58.0681591655549,3.04592528053768));
#33145=CARTESIAN_POINT('',(-33.5283521207634,-58.0741669114358,3.10407471946233));
#33146=CARTESIAN_POINT('',(-33.5273749999999,-58.0711169444146,-3.54592528053767));
#33147=CARTESIAN_POINT('Ctrl Pts',(-33.5283521207634,-58.0741669114359,
3.10407471946232));
#33148=CARTESIAN_POINT('Ctrl Pts',(-33.4960959785975,-58.0929755878456,
3.10610775634773));
#33149=CARTESIAN_POINT('Ctrl Pts',(-32.8657385633012,-58.4363094602464,
3.14518675675581));
#33150=CARTESIAN_POINT('Ctrl Pts',(-31.2749245001037,-58.3886783513254,
3.22131172068658));
#33151=CARTESIAN_POINT('Ctrl Pts',(-30.0737566908708,-56.3997070920348,
3.33244961125462));
#33152=CARTESIAN_POINT('Ctrl Pts',(-31.0933568979523,-54.3118310914232,
3.44358750182266));
#33153=CARTESIAN_POINT('Ctrl Pts',(-33.4004734887601,-54.0361069309691,
3.5547253923907));
#33154=CARTESIAN_POINT('Ctrl Pts',(-34.8833764832336,-55.8249080616723,
3.66586328295875));
#33155=CARTESIAN_POINT('Ctrl Pts',(-34.3608947477859,-57.4821952700404,
3.74897972531595));
#33156=CARTESIAN_POINT('Ctrl Pts',(-33.6738083543112,-57.9881060978322,
3.79505020415048));
#33157=CARTESIAN_POINT('Ctrl Pts',(-33.5289081309377,-58.0700145843707,
3.80407471946232));
#33158=CARTESIAN_POINT('Ctrl Pts',(-33.5268671815904,-58.0681591655549,
3.04592528053768));
#33159=CARTESIAN_POINT('Ctrl Pts',(-33.1711688207572,-58.2713555197574,
3.06806450906843));
#33160=CARTESIAN_POINT('Ctrl Pts',(-32.0617673212825,-58.5453769689692,
3.12724970112185));
#33161=CARTESIAN_POINT('Ctrl Pts',(-30.3694292262435,-57.4574138064661,
3.22348085669796));
#33162=CARTESIAN_POINT('Ctrl Pts',(-30.3650742488504,-55.1338834771873,
3.334618747266));
#33163=CARTESIAN_POINT('Ctrl Pts',(-32.3148410231895,-53.870071116671,3.44575663783405));
#33164=CARTESIAN_POINT('Ctrl Pts',(-34.4340859088485,-54.822758511107,3.55689452840208));
#33165=CARTESIAN_POINT('Ctrl Pts',(-34.7482454446892,-56.8908856856794,
3.65695074263663));
#33166=CARTESIAN_POINT('Ctrl Pts',(-33.9385250223179,-57.8277413596598,
3.71996099334849));
#33167=CARTESIAN_POINT('Ctrl Pts',(-33.5252102943906,-58.0708877004567,
3.74592528053768));
#33168=CARTESIAN_POINT('Origin',(-32.5,-56.2916512459885,-3.54592528053767));
#33169=CARTESIAN_POINT('',(-33.5296717523759,-58.0726906696378,2.34592528053768));
#33170=CARTESIAN_POINT('',(-33.5250223861017,-58.0699440624176,2.40407471946232));
#33171=CARTESIAN_POINT('',(-33.5273749999999,-58.0711169444146,-3.54592528053767));
#33172=CARTESIAN_POINT('Ctrl Pts',(-33.5250223861017,-58.0699440624176,
2.40407471946232));
#33173=CARTESIAN_POINT('Ctrl Pts',(-33.3162068666574,-58.1923260109822,
2.41716530854498));
#33174=CARTESIAN_POINT('Ctrl Pts',(-32.4393285405002,-58.523643057744,2.46730186115031));
#33175=CARTESIAN_POINT('Ctrl Pts',(-30.7136126829218,-57.9369940717681,
2.55448437727833));
#33176=CARTESIAN_POINT('Ctrl Pts',(-30.1488178080539,-55.6831490181888,
2.66562226784637));
#33177=CARTESIAN_POINT('Ctrl Pts',(-31.7360866576937,-53.9862729545993,
2.77676015841441));
#33178=CARTESIAN_POINT('Ctrl Pts',(-34.0225740529132,-54.3995357858862,
2.88789804898245));
#33179=CARTESIAN_POINT('Ctrl Pts',(-34.8990991658235,-56.5054325192522,
2.99700290266509));
#33180=CARTESIAN_POINT('Ctrl Pts',(-34.0838668521307,-57.7502442064381,
3.06906179282505));
#33181=CARTESIAN_POINT('Ctrl Pts',(-33.5283521207634,-58.0741669114359,
3.10407471946232));
#33182=CARTESIAN_POINT('Ctrl Pts',(-33.5296717523759,-58.0726906696378,
2.34592528053768));
#33183=CARTESIAN_POINT('Ctrl Pts',(-32.9991186855868,-58.3741080652297,
2.37912206126567));
#33184=CARTESIAN_POINT('Ctrl Pts',(-31.5690873940506,-58.494201559501,2.44936480551635));
#33185=CARTESIAN_POINT('Ctrl Pts',(-30.1211733226087,-56.7810568122912,
2.55665351328971));
#33186=CARTESIAN_POINT('Ctrl Pts',(-30.7986796648578,-54.5584913322389,
2.66779140385775));
#33187=CARTESIAN_POINT('Ctrl Pts',(-33.0334238041475,-53.9223067766118,
2.7789292944258));
#33188=CARTESIAN_POINT('Ctrl Pts',(-34.7799190860636,-55.4548100839991,
2.89006718499384));
#33189=CARTESIAN_POINT('Ctrl Pts',(-34.5073761199108,-57.29541607691,2.97906584703113));
#33190=CARTESIAN_POINT('Ctrl Pts',(-33.7663651927628,-57.931343458575,3.03101854554575));
#33191=CARTESIAN_POINT('Ctrl Pts',(-33.5268671815904,-58.0681591655549,
3.04592528053768));
#33192=CARTESIAN_POINT('Origin',(-32.5,-56.2916512459885,-3.54592528053767));
#33193=CARTESIAN_POINT('',(-33.5262302754658,-58.0727324938748,1.64592528053768));
#33194=CARTESIAN_POINT('',(-33.5276067488939,-58.0685424219934,1.70407471946232));
#33195=CARTESIAN_POINT('',(-33.5273749999999,-58.0711169444146,-3.54592528053767));
#33196=CARTESIAN_POINT('Ctrl Pts',(-33.5276067488939,-58.0685424219934,
1.70407471946232));
#33197=CARTESIAN_POINT('Ctrl Pts',(-33.1394910367319,-58.2891654943862,
1.72822286074223));
#33198=CARTESIAN_POINT('Ctrl Pts',(-31.9746000084876,-58.542974075687,1.78941696554481));
#33199=CARTESIAN_POINT('Ctrl Pts',(-30.3095139648772,-57.3405094780172,
1.88765703387008));
#33200=CARTESIAN_POINT('Ctrl Pts',(-30.4307974560059,-55.0201428925398,
1.99879492443812));
#33201=CARTESIAN_POINT('Ctrl Pts',(-32.4460455020051,-53.8636023228594,
2.10993281500616));
#33202=CARTESIAN_POINT('Ctrl Pts',(-34.5106787119048,-54.9294824684668,
2.2210707055742));
#33203=CARTESIAN_POINT('Ctrl Pts',(-34.7085028063896,-56.9697666836067,
2.31911800705959));
#33204=CARTESIAN_POINT('Ctrl Pts',(-33.9071483489281,-57.8459888695647,
2.3801193450223));
#33205=CARTESIAN_POINT('Ctrl Pts',(-33.5250223861017,-58.0699440624176,
2.40407471946232));
#33206=CARTESIAN_POINT('Ctrl Pts',(-33.5262302754658,-58.0727324938748,
1.64592528053768));
#33207=CARTESIAN_POINT('Ctrl Pts',(-33.4118498551747,-58.1401751811515,
1.65313364994024));
#33208=CARTESIAN_POINT('Ctrl Pts',(-32.670930140884,-58.4845521558011,1.69738798286549));
#33209=CARTESIAN_POINT('Ctrl Pts',(-30.9955026631254,-58.198172143523,1.77868827931342));
#33210=CARTESIAN_POINT('Ctrl Pts',(-30.0822688349231,-56.0616291105052,
1.88982616988146));
#33211=CARTESIAN_POINT('Ctrl Pts',(-31.3820117610517,-54.1356279467243,
2.0009640604495));
#33212=CARTESIAN_POINT('Ctrl Pts',(-33.7050620011389,-54.1830593597269,
2.11210195101755));
#33213=CARTESIAN_POINT('Ctrl Pts',(-34.9251053252509,-56.1605088392832,
2.22323984158559));
#33214=CARTESIAN_POINT('Ctrl Pts',(-34.224026615261,-57.6314775216245,2.30118095142563));
#33215=CARTESIAN_POINT('Ctrl Pts',(-33.5911896372902,-58.0377411767145,
2.34207609774299));
#33216=CARTESIAN_POINT('Ctrl Pts',(-33.5296717523759,-58.0726906696378,
2.34592528053768));
#33217=CARTESIAN_POINT('Origin',(-32.5,-56.2916512459885,-3.54592528053767));
#33218=CARTESIAN_POINT('',(-33.5256402930183,-58.0682685471634,0.945925280537677));
#33219=CARTESIAN_POINT('',(-33.5294982470258,-58.0735597602013,1.00407471946232));
#33220=CARTESIAN_POINT('',(-33.5273749999999,-58.0711169444146,-3.54592528053767));
#33221=CARTESIAN_POINT('Ctrl Pts',(-33.5294982470258,-58.0735597602013,
1.00407471946232));
#33222=CARTESIAN_POINT('Ctrl Pts',(-32.9682880946418,-58.3946192964701,
1.03928041293948));
#33223=CARTESIAN_POINT('Ctrl Pts',(-31.4766956957228,-58.4741418727902,
1.11153206993931));
#33224=CARTESIAN_POINT('Ctrl Pts',(-30.0981915249122,-56.6517188923722,
1.22082969046183));
#33225=CARTESIAN_POINT('Ctrl Pts',(-30.8948796869627,-54.4690373423775,
1.33196758102987));
#33226=CARTESIAN_POINT('Ctrl Pts',(-33.1607526748339,-53.9546149682087,
1.44310547159791));
#33227=CARTESIAN_POINT('Ctrl Pts',(-34.8218312459871,-55.5793084028841,
1.55424336216595));
#33228=CARTESIAN_POINT('Ctrl Pts',(-34.4585557374772,-57.3613319496871,
1.64123311145409));
#33229=CARTESIAN_POINT('Ctrl Pts',(-33.7349041722058,-57.9507048982935,
1.69117689721955));
#33230=CARTESIAN_POINT('Ctrl Pts',(-33.5276067488939,-58.0685424219934,
1.70407471946232));
#33231=CARTESIAN_POINT('Ctrl Pts',(-33.5256402930184,-58.0682685471634,
0.945925280537676));
#33232=CARTESIAN_POINT('Ctrl Pts',(-33.2328184146122,-58.2374617349622,
0.964191202137493));
#33233=CARTESIAN_POINT('Ctrl Pts',(-32.2264812528154,-58.542293513151,1.01950308725999));
#33234=CARTESIAN_POINT('Ctrl Pts',(-30.5023763530244,-57.6728948648119,
1.11186093590517));
#33235=CARTESIAN_POINT('Ctrl Pts',(-30.2561395980006,-55.3624447749947,
1.22299882647321));
#33236=CARTESIAN_POINT('Ctrl Pts',(-32.0637337160182,-53.9025079060376,
1.33413671704125));
#33237=CARTESIAN_POINT('Ctrl Pts',(-34.2706473113688,-54.629381030845,1.4452746076093));
#33238=CARTESIAN_POINT('Ctrl Pts',(-34.8188452912069,-56.7319204842157,
1.54920412877477));
#33239=CARTESIAN_POINT('Ctrl Pts',(-33.9996850008464,-57.7935670658911,
1.61608768641756));
#33240=CARTESIAN_POINT('Ctrl Pts',(-33.5262302754658,-58.0727324938748,
1.64592528053768));
#33241=CARTESIAN_POINT('Origin',(-32.5,-56.2916512459885,-3.54592528053767));
#33242=CARTESIAN_POINT('',(-33.5292382420786,-58.0706648023921,0.245925280537673));
#33243=CARTESIAN_POINT('',(-33.5256021009514,-58.0718002431918,0.304074719462323));
#33244=CARTESIAN_POINT('',(-33.5273749999999,-58.0711169444146,-3.54592528053767));
#33245=CARTESIAN_POINT('Ctrl Pts',(-33.5256021009514,-58.0718002431918,
0.304074719462322));
#33246=CARTESIAN_POINT('Ctrl Pts',(-33.3791306461153,-58.1581427811428,
0.313292001614045));
#33247=CARTESIAN_POINT('Ctrl Pts',(-32.5930673149393,-58.4998906338152,
0.35955524728845));
#33248=CARTESIAN_POINT('Ctrl Pts',(-30.8946190614981,-58.1140355911318,
0.442864456485535));
#33249=CARTESIAN_POINT('Ctrl Pts',(-30.0982430406458,-55.931240133699,0.554002347053576));
#33250=CARTESIAN_POINT('Ctrl Pts',(-31.5002224030512,-54.0783330542954,
0.665140237621618));
#33251=CARTESIAN_POINT('Ctrl Pts',(-33.8173095378994,-54.2513012166797,
0.776278128189661));
#33252=CARTESIAN_POINT('Ctrl Pts',(-34.9286483135496,-56.291824899935,0.887416018757701));
#33253=CARTESIAN_POINT('Ctrl Pts',(-34.1691544002423,-57.6858533133783,
0.96334821584859));
#33254=CARTESIAN_POINT('Ctrl Pts',(-33.5588337928047,-58.0567773540314,
1.0022344494168));
#33255=CARTESIAN_POINT('Ctrl Pts',(-33.5294982470258,-58.0735597602013,
1.00407471946232));
#33256=CARTESIAN_POINT('Ctrl Pts',(-33.5292382420786,-58.0706648023921,
0.245925280537675));
#33257=CARTESIAN_POINT('Ctrl Pts',(-33.0588051630516,-58.33651145622,0.275248754334742));
#33258=CARTESIAN_POINT('Ctrl Pts',(-31.7450292213916,-58.5230813041051,
0.34161819165449));
#33259=CARTESIAN_POINT('Ctrl Pts',(-30.1850532410697,-57.0260596319961,
0.445033592496918));
#33260=CARTESIAN_POINT('Ctrl Pts',(-30.6274839128386,-54.7450363379152,
0.556171483064961));
#33261=CARTESIAN_POINT('Ctrl Pts',(-32.783849793945,-53.8796472115696,0.667309373633002));
#33262=CARTESIAN_POINT('Ctrl Pts',(-34.6804047400893,-55.2219927306232,
0.778447264201044));
#33263=CARTESIAN_POINT('Ctrl Pts',(-34.5975134385767,-57.1618755368451,
0.871319233169269));
#33264=CARTESIAN_POINT('Ctrl Pts',(-33.8267040593522,-57.8943131766358,
0.927145238614813));
#33265=CARTESIAN_POINT('Ctrl Pts',(-33.5256402930184,-58.0682685471634,
0.945925280537676));
#33266=CARTESIAN_POINT('Origin',(-32.5,-56.2916512459885,-3.54592528053767));
#33267=CARTESIAN_POINT('',(-33.5278097333142,-58.0740011795199,-0.454074719462327));
#33268=CARTESIAN_POINT('',(-33.526223785585,-58.0680718733222,-0.395925280537678));
#33269=CARTESIAN_POINT('',(-33.5273749999999,-58.0711169444146,-3.54592528053767));
#33270=CARTESIAN_POINT('Ctrl Pts',(-33.526223785585,-58.0680718733222,-0.395925280537677));
#33271=CARTESIAN_POINT('Ctrl Pts',(-33.2007518244939,-58.254991046836,-0.375650446188704));
#33272=CARTESIAN_POINT('Ctrl Pts',(-32.1416146375096,-58.5451226040268,
-0.31832964831705));
#33273=CARTESIAN_POINT('Ctrl Pts',(-30.4306156658192,-57.5628636674515,
-0.223962886922716));
#33274=CARTESIAN_POINT('Ctrl Pts',(-30.3096639686861,-55.2424797818376,
-0.112824996354674));
#33275=CARTESIAN_POINT('Ctrl Pts',(-32.1935517174549,-53.8824144115655,
-0.00168710578663172));
#33276=CARTESIAN_POINT('Ctrl Pts',(-34.3579350363402,-54.7275508506072,
0.10945078478141));
#33277=CARTESIAN_POINT('Ctrl Pts',(-34.7832643179972,-56.8155005034113,
0.211371393197728));
#33278=CARTESIAN_POINT('Ctrl Pts',(-33.967826541896,-57.8111161350299,0.276246038091365));
#33279=CARTESIAN_POINT('Ctrl Pts',(-33.5256021009514,-58.0718002431918,
0.304074719462322));
#33280=CARTESIAN_POINT('Ctrl Pts',(-33.5278097333142,-58.0740011795199,
-0.454074719462325));
#33281=CARTESIAN_POINT('Ctrl Pts',(-33.4749288712104,-58.1049786318385,
-0.450739656990689));
#33282=CARTESIAN_POINT('Ctrl Pts',(-32.8174992673745,-58.4495803163018,
-0.410358630996371));
#33283=CARTESIAN_POINT('Ctrl Pts',(-31.2021687803137,-58.3444462635109,
-0.332931641479373));
#33284=CARTESIAN_POINT('Ctrl Pts',(-30.0714596841225,-56.3145920190741,
-0.221793750911332));
#33285=CARTESIAN_POINT('Ctrl Pts',(-31.1636212068567,-54.2637395061114,
-0.11065586034329));
#33286=CARTESIAN_POINT('Ctrl Pts',(-33.4789853310955,-54.069057766837,0.000482030224751219));
#33287=CARTESIAN_POINT('Ctrl Pts',(-34.8982731111897,-55.908740964546,0.111619920792794));
#33288=CARTESIAN_POINT('Ctrl Pts',(-34.3271081175644,-57.521036291931,0.193434337563768));
#33289=CARTESIAN_POINT('Ctrl Pts',(-33.6531292464159,-58.0006526999044,
0.238202790812062));
#33290=CARTESIAN_POINT('Ctrl Pts',(-33.5292382420786,-58.0706648023921,
0.245925280537675));
#33291=CARTESIAN_POINT('Origin',(-32.5,-56.2916512459885,-3.54592528053767));
#33292=CARTESIAN_POINT('',(-33.5250365419916,-58.0693901510839,-1.15407471946233));
#33293=CARTESIAN_POINT('',(-33.5295799600393,-58.0717283210701,-1.09592528053768));
#33294=CARTESIAN_POINT('',(-33.5273749999999,-58.0711169444146,-3.54592528053767));
#33295=CARTESIAN_POINT('Ctrl Pts',(-33.5295799600393,-58.0717283210701,
-1.09592528053768));
#33296=CARTESIAN_POINT('Ctrl Pts',(-33.0277944721986,-58.3557212843617,
-1.06459289399145));
#33297=CARTESIAN_POINT('Ctrl Pts',(-31.6541659742537,-58.5096740781238,
-0.99621454392255));
#33298=CARTESIAN_POINT('Ctrl Pts',(-30.1487320710282,-56.8998163998922,
-0.890790230330965));
#33299=CARTESIAN_POINT('Ctrl Pts',(-30.7138473610247,-54.6460533962845,
-0.779652339762925));
#33300=CARTESIAN_POINT('Ctrl Pts',(-32.91385067807,-53.8985232611178,-0.668514449194883));
#33301=CARTESIAN_POINT('Ctrl Pts',(-34.7350506405739,-55.3414510668855,
-0.557376558626841));
#33302=CARTESIAN_POINT('Ctrl Pts',(-34.5514515687201,-57.2322106426396,
-0.466513502407772));
#33303=CARTESIAN_POINT('Ctrl Pts',(-33.7954507596715,-57.9134543040693,
-0.412696409711384));
#33304=CARTESIAN_POINT('Ctrl Pts',(-33.526223785585,-58.0680718733222,-0.395925280537677));
#33305=CARTESIAN_POINT('Ctrl Pts',(-33.5250365419916,-58.0693901510839,
-1.15407471946233));
#33306=CARTESIAN_POINT('Ctrl Pts',(-33.2951376806275,-58.203713320331,-1.13968210479344));
#33307=CARTESIAN_POINT('Ctrl Pts',(-32.3865699532721,-58.5298194771329,
-1.08824352660187));
#33308=CARTESIAN_POINT('Ctrl Pts',(-30.6570393620673,-57.873352597378,-0.999758984887624));
#33309=CARTESIAN_POINT('Ctrl Pts',(-30.1715905180573,-55.6011108576298,
-0.888621094319583));
#33310=CARTESIAN_POINT('Ctrl Pts',(-31.817369145763,-53.960908709333,-0.77748320375154));
#33311=CARTESIAN_POINT('Ctrl Pts',(-34.087963584719,-54.4540716106361,-0.666345313183499));
#33312=CARTESIAN_POINT('Ctrl Pts',(-34.8805586635865,-56.5639154031852,
-0.558542485087094));
#33313=CARTESIAN_POINT('Ctrl Pts',(-34.0623309079662,-57.7608802593549,
-0.487785620513369));
#33314=CARTESIAN_POINT('Ctrl Pts',(-33.5278097333142,-58.0740011795199,
-0.454074719462325));
#33315=CARTESIAN_POINT('Origin',(-32.5,-56.2916512459885,-3.54592528053767));
#33316=CARTESIAN_POINT('',(-33.5283546803393,-58.0681541983481,-1.85407471946233));
#33317=CARTESIAN_POINT('',(-33.5269872402601,-58.0734398505124,-1.79592528053768));
#33318=CARTESIAN_POINT('',(-33.5273749999999,-58.0711169444146,-3.54592528053767));
#33319=CARTESIAN_POINT('',(-34.4842965055667,-55.7582049595679,-2.));
#33320=CARTESIAN_POINT('Ctrl Pts',(-34.4842965055667,-55.7582049595679,
-2.));
#33321=CARTESIAN_POINT('Ctrl Pts',(-34.6616800870191,-56.4180307560557,
-1.96295403647732));
#33322=CARTESIAN_POINT('Ctrl Pts',(-34.426165795488,-57.4023224375314,-1.91431227629809));
#33323=CARTESIAN_POINT('Ctrl Pts',(-33.7147012993046,-57.9624349357751,
-1.86567051611887));
#33324=CARTESIAN_POINT('Ctrl Pts',(-33.5283546803393,-58.0681541983481,
-1.85407471946233));
#33325=CARTESIAN_POINT('',(-33.9566395923166,-54.8371582344187,-2.));
#33326=CARTESIAN_POINT('Origin',(-32.5,-56.2916512459885,-2.));
#33327=CARTESIAN_POINT('Ctrl Pts',(-33.9566410663199,-54.8371566128168,
-2.));
#33328=CARTESIAN_POINT('Ctrl Pts',(-34.4273146919907,-55.3097386618185,
-1.96367708181445));
#33329=CARTESIAN_POINT('Ctrl Pts',(-34.8405825937333,-56.6643607585548,
-1.89565217532701));
#33330=CARTESIAN_POINT('Ctrl Pts',(-34.0295256140623,-57.7776919138425,
-1.82762726883957));
#33331=CARTESIAN_POINT('Ctrl Pts',(-33.5269872402601,-58.0734398505124,
-1.79592528053768));
#33332=CARTESIAN_POINT('Origin',(32.5,-56.2916512459885,3.));
#33333=CARTESIAN_POINT('',(33.3327252244638,-57.7364024133914,6.12851963660979));
#33334=CARTESIAN_POINT('',(33.3348404573523,-57.735699266238,6.32148036339021));
#33335=CARTESIAN_POINT('',(33.333,-57.7344495686934,3.));
#33336=CARTESIAN_POINT('',(33.0411029802559,-57.8673300091754,7.));
#33337=CARTESIAN_POINT('Ctrl Pts',(33.3348404573523,-57.735699266238,6.32148036339021));
#33338=CARTESIAN_POINT('Ctrl Pts',(33.3853483348093,-57.7070091850913,6.32537779445739));
#33339=CARTESIAN_POINT('Ctrl Pts',(33.4342336358034,-57.6755865432426,6.32927522552457));
#33340=CARTESIAN_POINT('Ctrl Pts',(33.4811646154108,-57.6414746748817,6.33317265659175));
#33341=CARTESIAN_POINT('Ctrl Pts',(33.9272541879144,-57.3172336532427,6.37021862011443));
#33342=CARTESIAN_POINT('Ctrl Pts',(34.196772145609,-56.7500228359926,6.40726458363711));
#33343=CARTESIAN_POINT('Ctrl Pts',(34.1662427495344,-56.1993881251835,6.44431054715979));
#33344=CARTESIAN_POINT('Ctrl Pts',(34.1357133534598,-55.6487534143744,6.48135651068247));
#33345=CARTESIAN_POINT('Ctrl Pts',(33.805136603616,-55.1146948100064,6.51840247420515));
#33346=CARTESIAN_POINT('Ctrl Pts',(33.3260603863118,-54.8417096746677,6.55544843772783));
#33347=CARTESIAN_POINT('Ctrl Pts',(32.8469841690075,-54.5687245393289,6.59249440125051));
#33348=CARTESIAN_POINT('Ctrl Pts',(32.2194084842428,-54.5568128730195,6.62954036477319));
#33349=CARTESIAN_POINT('Ctrl Pts',(31.7300326690205,-54.8112607055414,6.66658632829587));
#33350=CARTESIAN_POINT('Ctrl Pts',(31.2406568537983,-55.0657085380633,6.70363229181855));
#33351=CARTESIAN_POINT('Ctrl Pts',(30.8894809081185,-55.5865158694165,6.74067825534124));
#33352=CARTESIAN_POINT('Ctrl Pts',(30.8382644239114,-56.1356774091288,6.77772421886392));
#33353=CARTESIAN_POINT('Ctrl Pts',(30.7870479397043,-56.6848389488411,6.8147701823866));
#33354=CARTESIAN_POINT('Ctrl Pts',(31.0357909169699,-57.2623546969125,6.85181614590928));
#33355=CARTESIAN_POINT('Ctrl Pts',(31.4683170081768,-57.6029598655743,6.88886210943196));
#33356=CARTESIAN_POINT('Ctrl Pts',(31.9008430993836,-57.9435650342362,6.92590807295464));
#33357=CARTESIAN_POINT('Ctrl Pts',(32.5171523045318,-58.0472596234885,6.96295403647732));
#33358=CARTESIAN_POINT('Ctrl Pts',(33.0411029802559,-57.8673300091754,7.));
#33359=CARTESIAN_POINT('',(33.9709880617748,-55.5030815934935,7.));
#33360=CARTESIAN_POINT('Origin',(32.5,-56.2916512459885,7.));
#33361=CARTESIAN_POINT('',(33.3311603318023,-57.7325647065031,6.82851963660979));
#33362=CARTESIAN_POINT('Ctrl Pts',(33.9709895856635,-55.503080679032,7.));
#33363=CARTESIAN_POINT('Ctrl Pts',(34.2258866982027,-55.980034418951,6.96367708181445));
#33364=CARTESIAN_POINT('Ctrl Pts',(34.2280600118627,-56.5931875605705,6.92735416362889));
#33365=CARTESIAN_POINT('Ctrl Pts',(33.9753141969146,-57.071300576271,6.89103124544334));
#33366=CARTESIAN_POINT('Ctrl Pts',(33.8303226570678,-57.3455774911288,6.87019404249882));
#33367=CARTESIAN_POINT('Ctrl Pts',(33.6014392610868,-57.5754137754314,6.84935683955431));
#33368=CARTESIAN_POINT('Ctrl Pts',(33.3311603318023,-57.7325647065031,6.82851963660979));
#33369=CARTESIAN_POINT('',(33.333,-57.7344495686934,8.));
#33370=CARTESIAN_POINT('',(33.333,-57.7344495686934,3.));
#33371=CARTESIAN_POINT('Origin',(32.5,-56.2916512459885,8.));
#33372=CARTESIAN_POINT('Ctrl Pts',(33.3311603318023,-57.7325647065031,6.82851963660979));
#33373=CARTESIAN_POINT('Ctrl Pts',(33.1209168329143,-57.8548086479361,6.81231087603163));
#33374=CARTESIAN_POINT('Ctrl Pts',(32.8856252648826,-57.9330713283932,6.79610211545346));
#33375=CARTESIAN_POINT('Ctrl Pts',(32.6452880462139,-57.9540583561263,6.7798933548753));
#33376=CARTESIAN_POINT('Ctrl Pts',(32.0959848596434,-58.0020252972197,6.74284739135262));
#33377=CARTESIAN_POINT('Ctrl Pts',(31.5203244682533,-57.7507986915125,6.70580142782993));
#33378=CARTESIAN_POINT('Ctrl Pts',(31.1820200481674,-57.3152751741702,6.66875546430725));
#33379=CARTESIAN_POINT('Ctrl Pts',(30.8437156280816,-56.8797516568278,6.63170950078457));
#33380=CARTESIAN_POINT('Ctrl Pts',(30.7427671793,-56.2599312278504,6.59466353726189));
#33381=CARTESIAN_POINT('Ctrl Pts',(30.9252443270203,-55.739517741093,6.55761757373921));
#33382=CARTESIAN_POINT('Ctrl Pts',(31.1077214747406,-55.2191042543355,6.52057161021653));
#33383=CARTESIAN_POINT('Ctrl Pts',(31.5736242189628,-54.7980977097981,6.48352564669386));
#33384=CARTESIAN_POINT('Ctrl Pts',(32.1097948324389,-54.6691542850846,6.44647968317117));
#33385=CARTESIAN_POINT('Ctrl Pts',(32.645965445915,-54.540210860371,6.40943371964849));
#33386=CARTESIAN_POINT('Ctrl Pts',(33.2524039286451,-54.7033305554813,6.37238775612581));
#33387=CARTESIAN_POINT('Ctrl Pts',(33.6515374626529,-55.0838706916793,6.33534179260313));
#33388=CARTESIAN_POINT('Ctrl Pts',(34.0506709966607,-55.4644108278772,6.29829582908045));
#33389=CARTESIAN_POINT('Ctrl Pts',(34.2424995819463,-56.0623714051629,6.26124986555777));
#33390=CARTESIAN_POINT('Ctrl Pts',(34.1392482605268,-56.6040873635991,6.22420390203509));
#33391=CARTESIAN_POINT('Ctrl Pts',(34.0503539438025,-57.0704781983289,6.19230914689333));
#33392=CARTESIAN_POINT('Ctrl Pts',(33.7427356506951,-57.4951784726194,6.16041439175156));
#33393=CARTESIAN_POINT('Ctrl Pts',(33.3327252244638,-57.7364024133914,6.12851963660979));
#33394=CARTESIAN_POINT('Origin',(32.5,-56.2916512459885,3.));
#33395=CARTESIAN_POINT('',(33.3347682721563,-57.7348627592986,5.4285196366098));
#33396=CARTESIAN_POINT('',(33.3325737793451,-57.732046708219,5.62148036339021));
#33397=CARTESIAN_POINT('',(33.333,-57.7344495686934,3.));
#33398=CARTESIAN_POINT('Ctrl Pts',(33.3325737793451,-57.732046708219,5.62148036339021));
#33399=CARTESIAN_POINT('Ctrl Pts',(33.5273851267366,-57.6207441464882,5.63643534665464));
#33400=CARTESIAN_POINT('Ctrl Pts',(33.7002675206604,-57.4721914078235,5.65139032991906));
#33401=CARTESIAN_POINT('Ctrl Pts',(33.8340159287012,-57.2942275627961,5.66634531318349));
#33402=CARTESIAN_POINT('Ctrl Pts',(34.1653328254098,-56.853381726016,5.70339127670617));
#33403=CARTESIAN_POINT('Ctrl Pts',(34.2565099960995,-56.2320591280653,5.74043724022885));
#33404=CARTESIAN_POINT('Ctrl Pts',(34.0658176145798,-55.7146109150825,5.77748320375153));
#33405=CARTESIAN_POINT('Ctrl Pts',(33.8751252330602,-55.1971627020998,5.81452916727421));
#33406=CARTESIAN_POINT('Ctrl Pts',(33.4025632993312,-54.7835888740851,5.8515751307969));
#33407=CARTESIAN_POINT('Ctrl Pts',(32.8644065969169,-54.6631651603563,5.88862109431958));
#33408=CARTESIAN_POINT('Ctrl Pts',(32.3262498945026,-54.5427414466275,5.92566705784226));
#33409=CARTESIAN_POINT('Ctrl Pts',(31.722498423403,-54.7154678471846,5.96271302136494));
#33410=CARTESIAN_POINT('Ctrl Pts',(31.3294542359751,-55.1022925139248,5.99975898488762));
#33411=CARTESIAN_POINT('Ctrl Pts',(30.9364100485472,-55.4891171806649,6.0368049484103));
#33412=CARTESIAN_POINT('Ctrl Pts',(30.7540731447909,-56.0900401135881,6.07385091193298));
#33413=CARTESIAN_POINT('Ctrl Pts',(30.8659074307874,-56.6300507637272,6.11089687545566));
#33414=CARTESIAN_POINT('Ctrl Pts',(30.9777417167839,-57.1700614138663,6.14794283897834));
#33415=CARTESIAN_POINT('Ctrl Pts',(31.3837471925331,-57.6491597812213,6.18498880250102));
#33416=CARTESIAN_POINT('Ctrl Pts',(31.8980805240639,-57.8480733518849,6.2220347660237));
#33417=CARTESIAN_POINT('Ctrl Pts',(32.3583032720229,-58.0260601641038,6.25518329847921));
#33418=CARTESIAN_POINT('Ctrl Pts',(32.9052595394904,-57.9797148933652,6.28833183093471));
#33419=CARTESIAN_POINT('Ctrl Pts',(33.3348404573523,-57.735699266238,6.32148036339021));
#33420=CARTESIAN_POINT('Ctrl Pts',(33.3327252244638,-57.7364024133914,6.12851963660979));
#33421=CARTESIAN_POINT('Ctrl Pts',(33.2665058998609,-57.7753616334844,6.12336842822888));
#33422=CARTESIAN_POINT('Ctrl Pts',(33.1976157450274,-57.8095349962739,6.11821721984796));
#33423=CARTESIAN_POINT('Ctrl Pts',(33.1265448412824,-57.8383251884469,6.11306601146705));
#33424=CARTESIAN_POINT('Ctrl Pts',(32.6154239715823,-58.0453757152716,6.07602004794436));
#33425=CARTESIAN_POINT('Ctrl Pts',(31.9915134603068,-57.9740054293342,6.03897408442169));
#33426=CARTESIAN_POINT('Ctrl Pts',(31.5403536505083,-57.6568760819726,6.00192812089901));
#33427=CARTESIAN_POINT('Ctrl Pts',(31.0891938407098,-57.3397467346111,5.96488215737633));
#33428=CARTESIAN_POINT('Ctrl Pts',(30.8107847323884,-56.7768583258254,5.92783619385365));
#33429=CARTESIAN_POINT('Ctrl Pts',(30.8325397428816,-56.2258205630586,5.89079023033097));
#33430=CARTESIAN_POINT('Ctrl Pts',(30.8542947533749,-55.6747828002917,5.85374426680828));
#33431=CARTESIAN_POINT('Ctrl Pts',(31.1762138826829,-55.1355956835437,5.8166983032856));
#33432=CARTESIAN_POINT('Ctrl Pts',(31.6509700657299,-54.8550209349977,5.77965233976292));
#33433=CARTESIAN_POINT('Ctrl Pts',(32.1257262487769,-54.5744461864517,5.74260637624024));
#33434=CARTESIAN_POINT('Ctrl Pts',(32.7533194855629,-54.5524838061078,5.70556041271756));
#33435=CARTESIAN_POINT('Ctrl Pts',(33.2465276451507,-54.7991851622225,5.66851444919488));
#33436=CARTESIAN_POINT('Ctrl Pts',(33.7397358047385,-55.0458865183372,5.6314684856722));
#33437=CARTESIAN_POINT('Ctrl Pts',(34.0985588871282,-55.5612516109106,5.59442252214952));
#33438=CARTESIAN_POINT('Ctrl Pts',(34.1587797389667,-56.1094206024476,5.55737655862684));
#33439=CARTESIAN_POINT('Ctrl Pts',(34.2190005908051,-56.6575895939847,5.52033059510416));
#33440=CARTESIAN_POINT('Ctrl Pts',(33.9806192120925,-57.2385624844853,5.48328463158148));
#33441=CARTESIAN_POINT('Ctrl Pts',(33.5527320593965,-57.5864537767432,5.4462386680588));
#33442=CARTESIAN_POINT('Ctrl Pts',(33.4845127880347,-57.6419190795022,5.44033232424247));
#33443=CARTESIAN_POINT('Ctrl Pts',(33.4114765004846,-57.691459719343,5.43442598042613));
#33444=CARTESIAN_POINT('Ctrl Pts',(33.3347682721563,-57.7348627592986,5.4285196366098));
#33445=CARTESIAN_POINT('Origin',(32.5,-56.2916512459885,3.));
#33446=CARTESIAN_POINT('',(33.3320164235938,-57.7319854708824,4.72851963660979));
#33447=CARTESIAN_POINT('',(33.3312509399777,-57.7342826871321,4.9214803633902));
#33448=CARTESIAN_POINT('',(33.333,-57.7344495686934,3.));
#33449=CARTESIAN_POINT('Ctrl Pts',(33.3312509399777,-57.7342826871321,4.9214803633902));
#33450=CARTESIAN_POINT('Ctrl Pts',(33.6669748777683,-57.5367675539577,4.94749289885188));
#33451=CARTESIAN_POINT('Ctrl Pts',(33.937858827665,-57.2229205202501,4.97350543431356));
#33452=CARTESIAN_POINT('Ctrl Pts',(34.0694479601931,-56.8587419095544,4.99951796977524));
#33453=CARTESIAN_POINT('Ctrl Pts',(34.2568516913978,-56.3400939850778,5.03656393329793));
#33454=CARTESIAN_POINT('Ctrl Pts',(34.1617340046633,-55.7193622303022,5.07360989682061));
#33455=CARTESIAN_POINT('Ctrl Pts',(33.827626015315,-55.2806280419242,5.11065586034329));
#33456=CARTESIAN_POINT('Ctrl Pts',(33.4935180259667,-54.8418938535462,5.14770182386597));
#33457=CARTESIAN_POINT('Ctrl Pts',(32.9204197340046,-54.5851572315658,5.18474778738864));
#33458=CARTESIAN_POINT('Ctrl Pts',(32.370612888852,-54.6279151680597,5.22179375091132));
#33459=CARTESIAN_POINT('Ctrl Pts',(31.8208060436993,-54.6706731045537,5.25883971443401));
#33460=CARTESIAN_POINT('Ctrl Pts',(31.2942906453562,-55.0129255995219,5.29588567795669));
#33461=CARTESIAN_POINT('Ctrl Pts',(31.032029319193,-55.4980388156703,5.33293164147937));
#33462=CARTESIAN_POINT('Ctrl Pts',(30.7697679930298,-55.9831520318186,5.36997760500205));
#33463=CARTESIAN_POINT('Ctrl Pts',(30.7717607390465,-56.611125969147,5.40702356852473));
#33464=CARTESIAN_POINT('Ctrl Pts',(31.0370958289673,-57.0945648785311,5.44406953204741));
#33465=CARTESIAN_POINT('Ctrl Pts',(31.3024309188881,-57.5780037879153,5.48111549557009));
#33466=CARTESIAN_POINT('Ctrl Pts',(31.831108352713,-57.9169076693553,5.51816145909277));
#33467=CARTESIAN_POINT('Ctrl Pts',(32.3811753809891,-57.9561750722705,5.55520742261545));
#33468=CARTESIAN_POINT('Ctrl Pts',(32.7091873614286,-57.9795907251543,5.57729840287371));
#33469=CARTESIAN_POINT('Ctrl Pts',(33.0448052440539,-57.8964589747132,5.59938938313196));
#33470=CARTESIAN_POINT('Ctrl Pts',(33.3325737793451,-57.732046708219,5.62148036339021));
#33471=CARTESIAN_POINT('Ctrl Pts',(33.3347682721563,-57.7348627592986,5.4285196366098));
#33472=CARTESIAN_POINT('Ctrl Pts',(32.9303446333077,-57.9636936909789,5.39738001690345));
#33473=CARTESIAN_POINT('Ctrl Pts',(32.423854116995,-58.0219212024995,5.3662403971971));
#33474=CARTESIAN_POINT('Ctrl Pts',(31.9831067199835,-57.8783395309755,5.33510077749076));
#33475=CARTESIAN_POINT('Ctrl Pts',(31.4587614599457,-57.7075242989346,5.29805481396807));
#33476=CARTESIAN_POINT('Ctrl Pts',(31.0274638665491,-57.2510841408376,5.2610088504454));
#33477=CARTESIAN_POINT('Ctrl Pts',(30.8865996954395,-56.7179114934438,5.22396288692272));
#33478=CARTESIAN_POINT('Ctrl Pts',(30.7457355243298,-56.1847388460499,5.18691692340004));
#33479=CARTESIAN_POINT('Ctrl Pts',(30.8953047755071,-55.5748337093591,5.14987095987736));
#33480=CARTESIAN_POINT('Ctrl Pts',(31.2668562499327,-55.1673226224439,5.11282499635467));
#33481=CARTESIAN_POINT('Ctrl Pts',(31.6384077243582,-54.7598115355286,5.07577903283199));
#33482=CARTESIAN_POINT('Ctrl Pts',(32.2319414220319,-54.5546944983888,5.03873306930931));
#33483=CARTESIAN_POINT('Ctrl Pts',(32.7758232721694,-54.6458444887422,5.00168710578663));
#33484=CARTESIAN_POINT('Ctrl Pts',(33.3197051223069,-54.7369944790956,4.96464114226395));
#33485=CARTESIAN_POINT('Ctrl Pts',(33.8139351249082,-55.1244114969421,4.92759517874127));
#33486=CARTESIAN_POINT('Ctrl Pts',(34.0323261210678,-55.6307919459654,4.89054921521859));
#33487=CARTESIAN_POINT('Ctrl Pts',(34.2507171172273,-56.1371723949886,4.85350325169591));
#33488=CARTESIAN_POINT('Ctrl Pts',(34.1932691069451,-56.7625162751886,4.81645728817323));
#33489=CARTESIAN_POINT('Ctrl Pts',(33.8862734957393,-57.2206314145013,4.77941132465055));
#33490=CARTESIAN_POINT('Ctrl Pts',(33.7456956532454,-57.4304091297116,4.76244742863696));
#33491=CARTESIAN_POINT('Ctrl Pts',(33.5527911750803,-57.6051213208864,4.74548353262338));
#33492=CARTESIAN_POINT('Ctrl Pts',(33.3320164235938,-57.7319854708824,4.72851963660979));
#33493=CARTESIAN_POINT('Origin',(32.5,-56.2916512459885,3.));
#33494=CARTESIAN_POINT('',(33.3316044198824,-57.73507921,4.02851963660979));
#33495=CARTESIAN_POINT('',(33.3343856218718,-57.7368361137997,4.2214803633902));
#33496=CARTESIAN_POINT('',(33.333,-57.7344495686934,3.));
#33497=CARTESIAN_POINT('Ctrl Pts',(33.3343856149812,-57.7368361019314,4.2214803633902));
#33498=CARTESIAN_POINT('Ctrl Pts',(33.8122975339405,-57.4609515848648,4.25855045104913));
#33499=CARTESIAN_POINT('Ctrl Pts',(34.1397428670922,-56.9245130794241,4.29562053870806));
#33500=CARTESIAN_POINT('Ctrl Pts',(34.1667586100627,-56.373348690468,4.33269062636699));
#33501=CARTESIAN_POINT('Ctrl Pts',(34.1937567719725,-55.8225429832862,4.36973658988968));
#33502=CARTESIAN_POINT('Ctrl Pts',(33.9207162964575,-55.2570306535141,4.40678255341236));
#33503=CARTESIAN_POINT('Ctrl Pts',(33.4725957048462,-54.9356216253737,4.44382851693504));
#33504=CARTESIAN_POINT('Ctrl Pts',(33.0244751132349,-54.6142125972332,4.48087448045772));
#33505=CARTESIAN_POINT('Ctrl Pts',(32.4012744055273,-54.5369068707243,4.5179204439804));
#33506=CARTESIAN_POINT('Ctrl Pts',(31.8882049204609,-54.7390838502781,4.55496640750308));
#33507=CARTESIAN_POINT('Ctrl Pts',(31.3751354353946,-54.9412608298319,4.59201237102576));
#33508=CARTESIAN_POINT('Ctrl Pts',(30.9721971729695,-55.4229205154485,4.62905833454844));
#33509=CARTESIAN_POINT('Ctrl Pts',(30.8637971116759,-55.9636286201302,4.66610429807112));
#33510=CARTESIAN_POINT('Ctrl Pts',(30.7553970503824,-56.5043367248119,4.7031502615938));
#33511=CARTESIAN_POINT('Ctrl Pts',(30.9415351902203,-57.1040932485588,4.74019622511648));
#33512=CARTESIAN_POINT('Ctrl Pts',(31.3370243602463,-57.488416218779,4.77724218863916));
#33513=CARTESIAN_POINT('Ctrl Pts',(31.7325135302722,-57.8727391889992,4.81428815216184));
#33514=CARTESIAN_POINT('Ctrl Pts',(32.3373537304862,-58.0416286056927,4.85133411568452));
#33515=CARTESIAN_POINT('Ctrl Pts',(32.8747364051652,-57.9177912669506,4.8883800792072));
#33516=CARTESIAN_POINT('Ctrl Pts',(33.0347855041357,-57.8809086962641,4.8994135072682));
#33517=CARTESIAN_POINT('Ctrl Pts',(33.1888509066773,-57.8180603341074,4.9104469353292));
#33518=CARTESIAN_POINT('Ctrl Pts',(33.3312509399777,-57.7342826871321,4.9214803633902));
#33519=CARTESIAN_POINT('Ctrl Pts',(33.3320164235938,-57.7319854708824,4.72851963660979));
#33520=CARTESIAN_POINT('Ctrl Pts',(33.0706605734929,-57.8821688027457,4.70843756910069));
#33521=CARTESIAN_POINT('Ctrl Pts',(32.770247004987,-57.965297344832,4.6883555015916));
#33522=CARTESIAN_POINT('Ctrl Pts',(32.4713490172714,-57.9601647997737,4.66827343408251));
#33523=CARTESIAN_POINT('Ctrl Pts',(31.919963362139,-57.9506966473078,4.63122747055982));
#33524=CARTESIAN_POINT('Ctrl Pts',(31.3737352640037,-57.6408739439503,4.59418150703715));
#33525=CARTESIAN_POINT('Ctrl Pts',(31.082649108761,-57.1724888068712,4.55713554351447));
#33526=CARTESIAN_POINT('Ctrl Pts',(30.7915629535184,-56.7041036697921,4.52008957999179));
#33527=CARTESIAN_POINT('Ctrl Pts',(30.7556187411683,-56.0771560989914,4.4830436164691));
#33528=CARTESIAN_POINT('Ctrl Pts',(30.9912665445818,-55.5785722051981,4.44599765294642));
#33529=CARTESIAN_POINT('Ctrl Pts',(31.2269143479953,-55.0799883114048,4.40895168942374));
#33530=CARTESIAN_POINT('Ctrl Pts',(31.7341541671722,-54.709768094619,4.37190572590106));
#33531=CARTESIAN_POINT('Ctrl Pts',(32.2808448224847,-54.6373449363854,4.33485976237838));
#33532=CARTESIAN_POINT('Ctrl Pts',(32.8275354777971,-54.5649217781518,4.2978137988557));
#33533=CARTESIAN_POINT('Ctrl Pts',(33.4136769692449,-54.7902956784704,4.26076783533302));
#33534=CARTESIAN_POINT('Ctrl Pts',(33.7710183196873,-55.2103229938828,4.22372187181034));
#33535=CARTESIAN_POINT('Ctrl Pts',(34.1283596701297,-55.6303503092952,4.18667590828766));
#33536=CARTESIAN_POINT('Ctrl Pts',(34.2569008795666,-56.2450310398012,4.14962994476498));
#33537=CARTESIAN_POINT('Ctrl Pts',(34.0978143345865,-56.7730530636186,4.1125839812423));
#33538=CARTESIAN_POINT('Ctrl Pts',(33.977481781258,-57.1724472320418,4.08456253303146));
#33539=CARTESIAN_POINT('Ctrl Pts',(33.692587001381,-57.5222608245174,4.05654108482063));
#33540=CARTESIAN_POINT('Ctrl Pts',(33.3316044198824,-57.73507921,4.02851963660979));
#33541=CARTESIAN_POINT('Origin',(32.5,-56.2916512459885,3.));
#33542=CARTESIAN_POINT('',(33.3347454964364,-57.7363721546008,3.32851963660979));
#33543=CARTESIAN_POINT('',(33.333716562894,-57.7328365508938,3.5214803633902));
#33544=CARTESIAN_POINT('',(33.333,-57.7344495686934,3.));
#33545=CARTESIAN_POINT('Ctrl Pts',(33.333716562894,-57.7328365508938,3.5214803633902));
#33546=CARTESIAN_POINT('Ctrl Pts',(33.4781004639345,-57.6510402790884,3.5325620397237));
#33547=CARTESIAN_POINT('Ctrl Pts',(33.6100888264908,-57.5485020789653,3.5436437160572));
#33548=CARTESIAN_POINT('Ctrl Pts',(33.7223873369831,-57.4276653019287,3.5547253923907));
#33549=CARTESIAN_POINT('Ctrl Pts',(34.0978004421985,-57.023708833649,3.59177135591338));
#33550=CARTESIAN_POINT('Ctrl Pts',(34.2531676277225,-56.4152547808823,3.62881731943606));
#33551=CARTESIAN_POINT('Ctrl Pts',(34.1173842201124,-55.880765591048,3.66586328295874));
#33552=CARTESIAN_POINT('Ctrl Pts',(33.9816008125024,-55.3462764012136,3.70290924648142));
#33553=CARTESIAN_POINT('Ctrl Pts',(33.5546668117583,-54.8857520743114,3.7399552100041));
#33554=CARTESIAN_POINT('Ctrl Pts',(33.0319709841925,-54.709954179896,3.77700117352679));
#33555=CARTESIAN_POINT('Ctrl Pts',(32.5092751566268,-54.5341562854806,3.81404713704947));
#33556=CARTESIAN_POINT('Ctrl Pts',(31.8908175022394,-54.643084823552,3.85109310057215));
#33557=CARTESIAN_POINT('Ctrl Pts',(31.4596386734713,-54.9868880310005,3.88813906409483));
#33558=CARTESIAN_POINT('Ctrl Pts',(31.0284598447031,-55.330691238449,3.92518502761751));
#33559=CARTESIAN_POINT('Ctrl Pts',(30.7845598415543,-55.9093691152746,3.96223099114019));
#33560=CARTESIAN_POINT('Ctrl Pts',(30.8395608834388,-56.4580864498104,3.99927695466287));
#33561=CARTESIAN_POINT('Ctrl Pts',(30.8945619253233,-57.0068037843461,4.03632291818555));
#33562=CARTESIAN_POINT('Ctrl Pts',(31.248464012241,-57.525560576592,4.07336888170823));
#33563=CARTESIAN_POINT('Ctrl Pts',(31.7393018474208,-57.7769448390475,4.11041484523091));
#33564=CARTESIAN_POINT('Ctrl Pts',(32.2298200515886,-58.0281654013958,4.14743668461734));
#33565=CARTESIAN_POINT('Ctrl Pts',(32.8570957184111,-58.0123615437382,4.18445852400377));
#33566=CARTESIAN_POINT('Ctrl Pts',(33.3343856149812,-57.7368361019314,4.2214803633902));
#33567=CARTESIAN_POINT('Ctrl Pts',(33.3316044198824,-57.73507921,4.02851963660979));
#33568=CARTESIAN_POINT('Ctrl Pts',(33.2153473010664,-57.8036189501297,4.01949512129795));
#33569=CARTESIAN_POINT('Ctrl Pts',(33.0911982807713,-57.8579494129027,4.0104706059861));
#33570=CARTESIAN_POINT('Ctrl Pts',(32.9621127685743,-57.8951505902149,4.00144609067425));
#33571=CARTESIAN_POINT('Ctrl Pts',(32.4322120469391,-58.0478627758654,3.96440012715157));
#33572=CARTESIAN_POINT('Ctrl Pts',(31.8191249030656,-57.9119238300377,3.9273541636289));
#33573=CARTESIAN_POINT('Ctrl Pts',(31.4034341447794,-57.5495469821188,3.89030820010621));
#33574=CARTESIAN_POINT('Ctrl Pts',(30.9877433864933,-57.1871701341999,3.85326223658353));
#33575=CARTESIAN_POINT('Ctrl Pts',(30.7694490137944,-56.5983553841899,3.81621627306085));
#33576=CARTESIAN_POINT('Ctrl Pts',(30.8484546841662,-56.0525771412361,3.77917030953817));
#33577=CARTESIAN_POINT('Ctrl Pts',(30.9274603545379,-55.5067988982823,3.74212434601549));
#33578=CARTESIAN_POINT('Ctrl Pts',(31.3037660679802,-55.0040571623848,3.70507838249281));
#33579=CARTESIAN_POINT('Ctrl Pts',(31.8051533809355,-54.7744345397173,3.66803241897013));
#33580=CARTESIAN_POINT('Ctrl Pts',(32.3065406938908,-54.5448119170498,3.63098645544745));
#33581=CARTESIAN_POINT('Ctrl Pts',(32.9330096063591,-54.5883084076123,3.59394049192477));
#33582=CARTESIAN_POINT('Ctrl Pts',(33.39785306823,-54.8850175958567,3.55689452840209));
#33583=CARTESIAN_POINT('Ctrl Pts',(33.862696530101,-55.181726784101,3.5198485648794));
#33584=CARTESIAN_POINT('Ctrl Pts',(34.1659145413745,-55.7316486700272,3.48280260135672));
#33585=CARTESIAN_POINT('Ctrl Pts',(34.1687376598278,-56.2831083842721,3.44575663783404));
#33586=CARTESIAN_POINT('Ctrl Pts',(34.1715607782811,-56.834568098517,3.40871067431136));
#33587=CARTESIAN_POINT('Ctrl Pts',(33.873989003914,-57.3875656410806,3.37166471078868));
#33588=CARTESIAN_POINT('Ctrl Pts',(33.4122077466127,-57.6890185508993,3.334618747266));
#33589=CARTESIAN_POINT('Ctrl Pts',(33.3868657595293,-57.70556191559,3.3325857103806));
#33590=CARTESIAN_POINT('Ctrl Pts',(33.3610292261422,-57.7213477085124,3.33055267349519));
#33591=CARTESIAN_POINT('Ctrl Pts',(33.3347454964364,-57.7363721546008,3.32851963660979));
#33592=CARTESIAN_POINT('Origin',(32.5,-56.2916512459885,3.));
#33593=CARTESIAN_POINT('',(33.3331301901789,-57.7323221393285,2.62851963660979));
#33594=CARTESIAN_POINT('',(33.3311289428234,-57.732893825255,2.82148036339021));
#33595=CARTESIAN_POINT('',(33.333,-57.7344495686934,3.));
#33596=CARTESIAN_POINT('Ctrl Pts',(33.3311289428234,-57.732893825255,2.82148036339021));
#33597=CARTESIAN_POINT('Ctrl Pts',(33.6180096158229,-57.5655068353994,2.84361959192095));
#33598=CARTESIAN_POINT('Ctrl Pts',(33.8582224621032,-57.3156647118177,2.8657588204517));
#33599=CARTESIAN_POINT('Ctrl Pts',(34.0018785934241,-57.0190572038434,2.88789804898245));
#33600=CARTESIAN_POINT('Ctrl Pts',(34.2422609442965,-56.5227386033238,2.92494401250513));
#33601=CARTESIAN_POINT('Ctrl Pts',(34.2122852455117,-55.8954772908328,2.96198997602781));
#33602=CARTESIAN_POINT('Ctrl Pts',(33.9256700455925,-55.4243429628455,2.99903593955049));
#33603=CARTESIAN_POINT('Ctrl Pts',(33.6390548456733,-54.9532086348582,3.03608190307317));
#33604=CARTESIAN_POINT('Ctrl Pts',(33.0958001446195,-54.6382012913747,3.07312786659585));
#33605=CARTESIAN_POINT('Ctrl Pts',(32.5445295368321,-54.6234858293533,3.11017383011853));
#33606=CARTESIAN_POINT('Ctrl Pts',(31.9932589290447,-54.6087703673318,3.14721979364121));
#33607=CARTESIAN_POINT('Ctrl Pts',(31.4339724145236,-54.8943467867725,3.1842657571639));
#33608=CARTESIAN_POINT('Ctrl Pts',(31.1226306380098,-55.3495194199899,3.22131172068658));
#33609=CARTESIAN_POINT('Ctrl Pts',(30.8112888614961,-55.8046920532072,3.25835768420926));
#33610=CARTESIAN_POINT('Ctrl Pts',(30.7478918229898,-56.4294609002013,3.29540364773194));
#33611=CARTESIAN_POINT('Ctrl Pts',(30.9614535366484,-56.9378969554647,3.33244961125462));
#33612=CARTESIAN_POINT('Ctrl Pts',(31.175015250307,-57.4463330107281,3.3694955747773));
#33613=CARTESIAN_POINT('Ctrl Pts',(31.6655357161305,-57.838436274261,3.40654153829998));
#33614=CARTESIAN_POINT('Ctrl Pts',(32.2085254614957,-57.9347584641311,3.44358750182266));
#33615=CARTESIAN_POINT('Ctrl Pts',(32.5890889655549,-58.0022674924479,3.46955178901184));
#33616=CARTESIAN_POINT('Ctrl Pts',(32.9954261310775,-57.9244846218395,3.49551607620102));
#33617=CARTESIAN_POINT('Ctrl Pts',(33.333716562894,-57.7328365508938,3.5214803633902));
#33618=CARTESIAN_POINT('Ctrl Pts',(33.3347454964364,-57.7363721546008,3.32851963660979));
#33619=CARTESIAN_POINT('Ctrl Pts',(32.8820875508043,-57.9951229094133,3.29350670997251));
#33620=CARTESIAN_POINT('Ctrl Pts',(32.2967926538178,-58.0280607074246,3.25849378333523));
#33621=CARTESIAN_POINT('Ctrl Pts',(31.8207237377836,-57.8159025761185,3.22348085669796));
#33622=CARTESIAN_POINT('Ctrl Pts',(31.3170117264913,-57.5914254144454,3.18643489317528));
#33623=CARTESIAN_POINT('Ctrl Pts',(30.9355784441425,-57.0925628140254,3.1493889296526));
#33624=CARTESIAN_POINT('Ctrl Pts',(30.8509889952778,-56.547622072684,3.11234296612992));
#33625=CARTESIAN_POINT('Ctrl Pts',(30.7663995464132,-56.0026813313427,3.07529700260724));
#33626=CARTESIAN_POINT('Ctrl Pts',(30.9786539310327,-55.41166244908,3.03825103908456));
#33627=CARTESIAN_POINT('Ctrl Pts',(31.390612726451,-55.0450485686685,3.00120507556188));
#33628=CARTESIAN_POINT('Ctrl Pts',(31.8025715218693,-54.678434688257,2.96415911203919));
#33629=CARTESIAN_POINT('Ctrl Pts',(32.4142347280865,-54.5362258096967,2.92711314851652));
#33630=CARTESIAN_POINT('Ctrl Pts',(32.9456712104109,-54.6835046326399,2.89006718499383));
#33631=CARTESIAN_POINT('Ctrl Pts',(33.4771076927353,-54.8307834555831,2.85302122147115));
#33632=CARTESIAN_POINT('Ctrl Pts',(33.928317451167,-55.2675499800298,2.81597525794847));
#33633=CARTESIAN_POINT('Ctrl Pts',(34.0928017812263,-55.7939155294323,2.77892929442579));
#33634=CARTESIAN_POINT('Ctrl Pts',(34.2572861112857,-56.3202810788348,2.74188333090311));
#33635=CARTESIAN_POINT('Ctrl Pts',(34.1350450129727,-56.9362456531932,2.70483736738043));
#33636=CARTESIAN_POINT('Ctrl Pts',(33.7820228180845,-57.3599095722955,2.66779140385775));
#33637=CARTESIAN_POINT('Ctrl Pts',(33.6572786340789,-57.509615768241,2.6547008147751));
#33638=CARTESIAN_POINT('Ctrl Pts',(33.5037182424927,-57.6353105712173,2.64161022569244));
#33639=CARTESIAN_POINT('Ctrl Pts',(33.3331301901789,-57.7323221393285,2.62851963660979));
#33640=CARTESIAN_POINT('Origin',(32.5,-56.2916512459885,3.));
#33641=CARTESIAN_POINT('',(33.331098284258,-57.7335685916211,1.92851963660978));
#33642=CARTESIAN_POINT('',(33.3331738820163,-57.7367002116856,2.12148036339021));
#33643=CARTESIAN_POINT('',(33.333,-57.7344495686934,3.));
#33644=CARTESIAN_POINT('Ctrl Pts',(33.3331738820163,-57.7367002116856,2.12148036339021));
#33645=CARTESIAN_POINT('Ctrl Pts',(33.7599095781772,-57.4863532801825,2.1546771441182));
#33646=CARTESIAN_POINT('Ctrl Pts',(34.0737470619128,-57.0348072848651,2.1878739248462));
#33647=CARTESIAN_POINT('Ctrl Pts',(34.1491952727494,-56.5464328961311,2.2210707055742));
#33648=CARTESIAN_POINT('Ctrl Pts',(34.2333917401539,-56.0014312606204,2.25811666909688));
#33649=CARTESIAN_POINT('Ctrl Pts',(34.0207112033875,-55.4105655517268,2.29516263261956));
#33650=CARTESIAN_POINT('Ctrl Pts',(33.608488116082,-55.044248811562,2.33220859614224));
#33651=CARTESIAN_POINT('Ctrl Pts',(33.1962650287764,-54.6779320713971,2.36925455966492));
#33652=CARTESIAN_POINT('Ctrl Pts',(32.5844993909316,-54.5361642999609,2.40630052318761));
#33653=CARTESIAN_POINT('Ctrl Pts',(32.0531692156544,-54.6838263217292,2.44334648671029));
#33654=CARTESIAN_POINT('Ctrl Pts',(31.5218390403773,-54.8314883434974,2.48039245023297));
#33655=CARTESIAN_POINT('Ctrl Pts',(31.0709443276677,-55.2685801584701,2.51743841375565));
#33656=CARTESIAN_POINT('Ctrl Pts',(30.9068395995441,-55.7950642190458,2.55448437727833));
#33657=CARTESIAN_POINT('Ctrl Pts',(30.7427348714206,-56.3215482796215,2.59153034080101));
#33658=CARTESIAN_POINT('Ctrl Pts',(30.8654201278831,-56.9374245858002,2.62857630432369));
#33659=CARTESIAN_POINT('Ctrl Pts',(31.2187477656388,-57.360833853803,2.66562226784637));
#33660=CARTESIAN_POINT('Ctrl Pts',(31.5720754033946,-57.7842431218059,2.70266823136905));
#33661=CARTESIAN_POINT('Ctrl Pts',(32.1560454224436,-58.0151853516329,2.73971419489173));
#33662=CARTESIAN_POINT('Ctrl Pts',(32.7034006322329,-57.9479685222722,2.77676015841441));
#33663=CARTESIAN_POINT('Ctrl Pts',(32.9236480838557,-57.9209214875348,2.79166689340634));
#33664=CARTESIAN_POINT('Ctrl Pts',(33.1379671006765,-57.845598452492,2.80657362839827));
#33665=CARTESIAN_POINT('Ctrl Pts',(33.3311289428234,-57.732893825255,2.82148036339021));
#33666=CARTESIAN_POINT('Ctrl Pts',(33.3331301901789,-57.7323221393285,2.62851963660979));
#33667=CARTESIAN_POINT('Ctrl Pts',(33.0209593136532,-57.9098503181175,2.60456426216976));
#33668=CARTESIAN_POINT('Ctrl Pts',(32.6517664254568,-57.9913244481799,2.58060888772973));
#33669=CARTESIAN_POINT('Ctrl Pts',(32.2977938304223,-57.9481146542166,2.55665351328971));
#33670=CARTESIAN_POINT('Ctrl Pts',(31.7503903291116,-57.8812925531888,2.51960754976703));
#33671=CARTESIAN_POINT('Ctrl Pts',(31.2393866179539,-57.5162850872868,2.48256158624435));
#33672=CARTESIAN_POINT('Ctrl Pts',(30.9986464429484,-57.0201399930138,2.44551562272167));
#33673=CARTESIAN_POINT('Ctrl Pts',(30.7579062679429,-56.5239948987407,2.40846965919899));
#33674=CARTESIAN_POINT('Ctrl Pts',(30.7874296290897,-55.8967121760966,2.37142369567631));
#33675=CARTESIAN_POINT('Ctrl Pts',(31.0737049927512,-55.4253713200344,2.33437773215363));
#33676=CARTESIAN_POINT('Ctrl Pts',(31.3599803564126,-54.9540304639723,2.29733176863094));
#33677=CARTESIAN_POINT('Ctrl Pts',(31.9030077225887,-54.6386314744921,2.26028580510827));
#33678=CARTESIAN_POINT('Ctrl Pts',(32.4542675379743,-54.6235184875634,2.22323984158558));
#33679=CARTESIAN_POINT('Ctrl Pts',(33.0055273533599,-54.6084055006347,2.1861938780629));
#33680=CARTESIAN_POINT('Ctrl Pts',(33.5650196179551,-54.8935785162575,2.14914791454022));
#33681=CARTESIAN_POINT('Ctrl Pts',(33.8766895243309,-55.3485264867911,2.11210195101754));
#33682=CARTESIAN_POINT('Ctrl Pts',(34.1883594307067,-55.8034744573246,2.07505598749486));
#33683=CARTESIAN_POINT('Ctrl Pts',(34.2522069788631,-56.4281973827689,2.03801002397218));
#33684=CARTESIAN_POINT('Ctrl Pts',(34.0390119763463,-56.9367872738744,2.0009640604495));
#33685=CARTESIAN_POINT('Ctrl Pts',(33.9000423680164,-57.2683078870831,1.97681591916959));
#33686=CARTESIAN_POINT('Ctrl Pts',(33.6433576792833,-57.550483699497,1.95266777788969));
#33687=CARTESIAN_POINT('Ctrl Pts',(33.331098284258,-57.7335685916211,1.92851963660978));
#33688=CARTESIAN_POINT('Origin',(32.5,-56.2916512459885,3.));
#33689=CARTESIAN_POINT('',(33.333854526745,-57.7369307977834,1.22851963660979));
#33690=CARTESIAN_POINT('',(33.3345984319871,-57.7343006412916,1.4214803633902));
#33691=CARTESIAN_POINT('',(33.333,-57.7344495686934,3.));
#33692=CARTESIAN_POINT('Ctrl Pts',(33.3345984319871,-57.7343006412916,1.4214803633902));
#33693=CARTESIAN_POINT('Ctrl Pts',(33.4283251997872,-57.6813267445322,1.42868873279277));
#33694=CARTESIAN_POINT('Ctrl Pts',(33.5166388707302,-57.6193252564529,1.43589710219534));
#33695=CARTESIAN_POINT('Ctrl Pts',(33.5974727328825,-57.5487559900283,1.44310547159791));
#33696=CARTESIAN_POINT('Ctrl Pts',(34.0129020958151,-57.1860794506077,1.48015143512059));
#33697=CARTESIAN_POINT('Ctrl Pts',(34.2307718231603,-56.5971073981535,1.51719739864327));
#33698=CARTESIAN_POINT('Ctrl Pts',(34.1513725987927,-56.0513862321698,1.55424336216595));
#33699=CARTESIAN_POINT('Ctrl Pts',(34.071973374425,-55.5056650661862,1.59128932568863));
#33700=CARTESIAN_POINT('Ctrl Pts',(33.6953051983445,-55.0031947866731,1.62833528921131));
#33701=CARTESIAN_POINT('Ctrl Pts',(33.1937523971885,-54.7739337662501,1.66538125273399));
#33702=CARTESIAN_POINT('Ctrl Pts',(32.6921995960325,-54.5446727458272,1.70242721625667));
#33703=CARTESIAN_POINT('Ctrl Pts',(32.065762169801,-54.5886209844943,1.73947317977935));
#33704=CARTESIAN_POINT('Ctrl Pts',(31.6011327587505,-54.8856653216219,1.77651914330203));
#33705=CARTESIAN_POINT('Ctrl Pts',(31.1365033477,-55.1827096587496,1.81356510682471));
#33706=CARTESIAN_POINT('Ctrl Pts',(30.8336819518306,-55.7328500943379,1.8506110703474));
#33707=CARTESIAN_POINT('Ctrl Pts',(30.8312565000759,-56.2843117385314,1.88765703387008));
#33708=CARTESIAN_POINT('Ctrl Pts',(30.8288310483213,-56.8357733827248,1.92470299739276));
#33709=CARTESIAN_POINT('Ctrl Pts',(31.1268015406815,-57.3885562355235,1.96174896091544));
#33710=CARTESIAN_POINT('Ctrl Pts',(31.5888000917202,-57.689676089852,1.99879492443812));
#33711=CARTESIAN_POINT('Ctrl Pts',(32.050798642759,-57.9907959441805,2.0358408879608));
#33712=CARTESIAN_POINT('Ctrl Pts',(32.6768252524763,-58.040252800039,2.07288685148348));
#33713=CARTESIAN_POINT('Ctrl Pts',(33.1803752931228,-57.8154124469044,2.10993281500616));
#33714=CARTESIAN_POINT('Ctrl Pts',(33.2326955992617,-57.7920508836856,2.11378199780084));
#33715=CARTESIAN_POINT('Ctrl Pts',(33.2836936714803,-57.7657280595765,2.11763118059552));
#33716=CARTESIAN_POINT('Ctrl Pts',(33.3331738820163,-57.7367002116856,2.12148036339021));
#33717=CARTESIAN_POINT('Ctrl Pts',(33.331098284258,-57.7335685916211,1.92851963660978));
#33718=CARTESIAN_POINT('Ctrl Pts',(33.1643166622693,-57.8313565069137,1.91562181436701));
#33719=CARTESIAN_POINT('Ctrl Pts',(32.9816809059177,-57.9008761528941,1.90272399212423));
#33720=CARTESIAN_POINT('Ctrl Pts',(32.792659312829,-57.9345477382936,1.88982616988146));
#33721=CARTESIAN_POINT('Ctrl Pts',(32.2497392050189,-58.0312614548405,1.85278020635878));
#33722=CARTESIAN_POINT('Ctrl Pts',(31.6541365425887,-57.8322320311678,1.8157342428361));
#33723=CARTESIAN_POINT('Ctrl Pts',(31.2784322612968,-57.4285464115926,1.77868827931342));
#33724=CARTESIAN_POINT('Ctrl Pts',(30.902727980005,-57.0248607920174,1.74164231579074));
#33725=CARTESIAN_POINT('Ctrl Pts',(30.7469220798513,-56.4165189765397,1.70459635226806));
#33726=CARTESIAN_POINT('Ctrl Pts',(30.8823200145202,-55.881932046546,1.66755038874538));
#33727=CARTESIAN_POINT('Ctrl Pts',(31.0177179491892,-55.3473451165522,1.6305044252227));
#33728=CARTESIAN_POINT('Ctrl Pts',(31.4443197186807,-54.8865130720423,1.59345846170001));
#33729=CARTESIAN_POINT('Ctrl Pts',(31.9668886041915,-54.7103383112812,1.55641249817733));
#33730=CARTESIAN_POINT('Ctrl Pts',(32.4894574897023,-54.53416355052,1.51936653465465));
#33731=CARTESIAN_POINT('Ctrl Pts',(33.1079934912324,-54.6426460735076,1.48232057113197));
#33732=CARTESIAN_POINT('Ctrl Pts',(33.5394201003417,-54.9861382384619,1.44527460760929));
#33733=CARTESIAN_POINT('Ctrl Pts',(33.9708467094511,-55.3296304034162,1.40822864408661));
#33734=CARTESIAN_POINT('Ctrl Pts',(34.2151639261397,-55.9081322103373,1.37118268056393));
#33735=CARTESIAN_POINT('Ctrl Pts',(34.1605585908213,-56.4568890269573,1.33413671704125));
#33736=CARTESIAN_POINT('Ctrl Pts',(34.1086657929391,-56.9783861738082,1.29893102356409));
#33737=CARTESIAN_POINT('Ctrl Pts',(33.7868109567046,-57.4730201142583,1.26372533008694));
#33738=CARTESIAN_POINT('Ctrl Pts',(33.333854526745,-57.7369307977834,1.22851963660979));
#33739=CARTESIAN_POINT('Origin',(32.5,-56.2916512459885,3.));
#33740=CARTESIAN_POINT('',(33.3341985401264,-57.7334817014242,0.528519636609787));
#33741=CARTESIAN_POINT('',(33.3317031312748,-57.7320766758176,0.721480363390202));
#33742=CARTESIAN_POINT('',(33.333,-57.7344495686934,3.));
#33743=CARTESIAN_POINT('Ctrl Pts',(33.3317031312748,-57.7320766758176,0.721480363390202));
#33744=CARTESIAN_POINT('Ctrl Pts',(33.5692173042018,-57.5950551525707,0.739746284990021));
#33745=CARTESIAN_POINT('Ctrl Pts',(33.7746291238346,-57.4025124831788,0.75801220658984));
#33746=CARTESIAN_POINT('Ctrl Pts',(33.9179858048945,-57.1714665641067,0.776278128189658));
#33747=CARTESIAN_POINT('Ctrl Pts',(34.208734144542,-56.7028716102066,0.813324091712339));
#33748=CARTESIAN_POINT('Ctrl Pts',(34.2442262482397,-56.0758982397686,0.850370055235019));
#33749=CARTESIAN_POINT('Ctrl Pts',(34.008218953441,-55.5774843709492,0.887416018757699));
#33750=CARTESIAN_POINT('Ctrl Pts',(33.7722116586424,-55.0790705021297,0.92446198228038));
#33751=CARTESIAN_POINT('Ctrl Pts',(33.2647049653473,-54.7092161349289,0.961507945803061));
#33752=CARTESIAN_POINT('Ctrl Pts',(32.7179621895189,-54.6371872177157,0.998553909325741));
#33753=CARTESIAN_POINT('Ctrl Pts',(32.1712194136904,-54.5651583005025,1.03559987284842));
#33754=CARTESIAN_POINT('Ctrl Pts',(31.5852405553285,-54.790954833277,1.0726458363711));
#33755=CARTESIAN_POINT('Ctrl Pts',(31.2282021616797,-55.21123975246,1.10969179989378));
#33756=CARTESIAN_POINT('Ctrl Pts',(30.8711637680308,-55.6315246716431,1.14673776341646));
#33757=CARTESIAN_POINT('Ctrl Pts',(30.7430658390951,-56.2462979772347,1.18378372693914));
#33758=CARTESIAN_POINT('Ctrl Pts',(30.902533118419,-56.77420517993,1.22082969046182));
#33759=CARTESIAN_POINT('Ctrl Pts',(31.0620003977429,-57.3021123826252,1.2578756539845));
#33760=CARTESIAN_POINT('Ctrl Pts',(31.5090328853265,-57.7431534824239,1.29492161750718));
#33761=CARTESIAN_POINT('Ctrl Pts',(32.0390436283783,-57.8954835191299,1.33196758102987));
#33762=CARTESIAN_POINT('Ctrl Pts',(32.4659253700502,-58.0181733178376,1.36180517514998));
#33763=CARTESIAN_POINT('Ctrl Pts',(32.9466353435786,-57.9535754234504,1.39164276927009));
#33764=CARTESIAN_POINT('Ctrl Pts',(33.3345984319871,-57.7343006412916,1.4214803633902));
#33765=CARTESIAN_POINT('Ctrl Pts',(33.333854526745,-57.7369307977834,1.22851963660979));
#33766=CARTESIAN_POINT('Ctrl Pts',(33.3101776135059,-57.7507259223106,1.22667936656426));
#33767=CARTESIAN_POINT('Ctrl Pts',(33.2861424840206,-57.7638906287274,1.22483909651873));
#33768=CARTESIAN_POINT('Ctrl Pts',(33.261768971111,-57.776395800606,1.22299882647321));
#33769=CARTESIAN_POINT('Ctrl Pts',(32.7711125740444,-58.0281339313159,1.18595286295053));
#33770=CARTESIAN_POINT('Ctrl Pts',(32.1433276672365,-58.0125983664166,1.14890689942785));
#33771=CARTESIAN_POINT('Ctrl Pts',(31.6657235730868,-57.7368990452689,1.11186093590517));
#33772=CARTESIAN_POINT('Ctrl Pts',(31.1881194789371,-57.4611997241213,1.07481497238249));
#33773=CARTESIAN_POINT('Ctrl Pts',(30.8606961974455,-56.9253366467254,1.03776900885981));
#33774=CARTESIAN_POINT('Ctrl Pts',(30.8333008499707,-56.3745505890177,1.00072304533712));
#33775=CARTESIAN_POINT('Ctrl Pts',(30.8059055024959,-55.8237645313099,0.963677081814445));
#33776=CARTESIAN_POINT('Ctrl Pts',(31.0785380890378,-55.2580554932903,0.926631118291764));
#33777=CARTESIAN_POINT('Ctrl Pts',(31.5264267604979,-54.9363234239653,0.889585154769083));
#33778=CARTESIAN_POINT('Ctrl Pts',(31.974315431958,-54.6145913546402,0.852539191246403));
#33779=CARTESIAN_POINT('Ctrl Pts',(32.5974601883362,-54.5368362540097,0.815493227723723));
#33780=CARTESIAN_POINT('Ctrl Pts',(33.1106752982772,-54.7386431848419,0.778447264201043));
#33781=CARTESIAN_POINT('Ctrl Pts',(33.6238904082182,-54.940450115674,0.741401300678362));
#33782=CARTESIAN_POINT('Ctrl Pts',(34.0271758717221,-55.4218190779688,0.704355337155682));
#33783=CARTESIAN_POINT('Ctrl Pts',(34.1359658098863,-55.9624488364586,0.667309373633001));
#33784=CARTESIAN_POINT('Ctrl Pts',(34.2447557480505,-56.5030785949484,0.630263410110321));
#33785=CARTESIAN_POINT('Ctrl Pts',(34.0590501608751,-57.1029691496333,0.59321744658764));
#33786=CARTESIAN_POINT('Ctrl Pts',(33.6638382628472,-57.4875771868012,0.55617148306496));
#33787=CARTESIAN_POINT('Ctrl Pts',(33.5655069136947,-57.5832702248356,0.546954200913235));
#33788=CARTESIAN_POINT('Ctrl Pts',(33.4542061287357,-57.6656362524338,0.537736918761511));
#33789=CARTESIAN_POINT('Ctrl Pts',(33.3341985401264,-57.7334817014242,0.528519636609787));
#33790=CARTESIAN_POINT('Origin',(32.5,-56.2916512459885,3.));
#33791=CARTESIAN_POINT('',(33.3313285320323,-57.7324067450656,-0.171480363390211));
#33792=CARTESIAN_POINT('',(33.3319271105622,-57.7355745198861,0.0214803633902046));
#33793=CARTESIAN_POINT('',(33.333,-57.7344495686934,3.));
#33794=CARTESIAN_POINT('Ctrl Pts',(33.3319271105622,-57.7355745198861,0.0214803633902046));
#33795=CARTESIAN_POINT('Ctrl Pts',(33.7093130799578,-57.5130220094248,0.0508038371872728));
#33796=CARTESIAN_POINT('Ctrl Pts',(34.0025116805637,-57.1388573741434,0.080127310984341));
#33797=CARTESIAN_POINT('Ctrl Pts',(34.1137073818814,-56.7167479649788,0.109450784781409));
#33798=CARTESIAN_POINT('Ctrl Pts',(34.2541870509479,-56.1834738419089,0.14649674830409));
#33799=CARTESIAN_POINT('Ctrl Pts',(34.1041780082168,-55.5736766763093,0.18354271182677));
#33800=CARTESIAN_POINT('Ctrl Pts',(33.7323327404969,-55.1664335984773,0.22058867534945));
#33801=CARTESIAN_POINT('Ctrl Pts',(33.3604874727769,-54.7591905206453,0.257634638872131));
#33802=CARTESIAN_POINT('Ctrl Pts',(32.7668059800683,-54.5545015305809,0.294680602394811));
#33803=CARTESIAN_POINT('Ctrl Pts',(32.2229899650201,-54.6460437054155,0.331726565917492));
#33804=CARTESIAN_POINT('Ctrl Pts',(31.679173949972,-54.7375858802501,0.368772529440172));
#33805=CARTESIAN_POINT('Ctrl Pts',(31.1852234125845,-55.1253592199838,0.405818492962853));
#33806=CARTESIAN_POINT('Ctrl Pts',(30.9671976166263,-55.6318970567811,0.442864456485533));
#33807=CARTESIAN_POINT('Ctrl Pts',(30.7491718206681,-56.1384348935784,0.479910420008214));
#33808=CARTESIAN_POINT('Ctrl Pts',(30.8070707661392,-56.7637372274395,0.516956383530895));
#33809=CARTESIAN_POINT('Ctrl Pts',(31.1143966726152,-57.2216308996084,0.554002347053575));
#33810=CARTESIAN_POINT('Ctrl Pts',(31.4217225790911,-57.6795245717774,0.591048310576256));
#33811=CARTESIAN_POINT('Ctrl Pts',(31.9784754465718,-57.9700095822543,0.628094274098936));
#33812=CARTESIAN_POINT('Ctrl Pts',(32.5298541681108,-57.9601438188116,0.665140237621616));
#33813=CARTESIAN_POINT('Ctrl Pts',(32.8093695193456,-57.9551424790316,0.683920279544479));
#33814=CARTESIAN_POINT('Ctrl Pts',(33.0875037843944,-57.872954864572,0.702700321467341));
#33815=CARTESIAN_POINT('Ctrl Pts',(33.3317031312748,-57.7320766758176,0.721480363390202));
#33816=CARTESIAN_POINT('Ctrl Pts',(33.3341985401264,-57.7334817014242,0.528519636609787));
#33817=CARTESIAN_POINT('Ctrl Pts',(32.9718734110338,-57.9383196733276,0.500690955238831));
#33818=CARTESIAN_POINT('Ctrl Pts',(32.5301815965126,-58.010795616536,0.472862273867874));
#33819=CARTESIAN_POINT('Ctrl Pts',(32.1264363544929,-57.9180609610465,0.445033592496918));
#33820=CARTESIAN_POINT('Ctrl Pts',(31.5889645530468,-57.7946111784729,0.407987628974237));
#33821=CARTESIAN_POINT('Ctrl Pts',(31.1187391590349,-57.3783860936747,0.370941665451557));
#33822=CARTESIAN_POINT('Ctrl Pts',(30.9309614883813,-56.8598734778586,0.333895701928876));
#33823=CARTESIAN_POINT('Ctrl Pts',(30.7431838177278,-56.3413608620425,0.296849738406196));
#33824=CARTESIAN_POINT('Ctrl Pts',(30.8378538704326,-55.7205607152084,0.259803774883515));
#33825=CARTESIAN_POINT('Ctrl Pts',(31.1716453640502,-55.2815857427568,0.222757811360835));
#33826=CARTESIAN_POINT('Ctrl Pts',(31.5054368576678,-54.8426107703051,0.185711847838154));
#33827=CARTESIAN_POINT('Ctrl Pts',(32.0783497921982,-54.5854609722359,0.148665884315473));
#33828=CARTESIAN_POINT('Ctrl Pts',(32.6281873065731,-54.6278224157042,0.111619920792793));
#33829=CARTESIAN_POINT('Ctrl Pts',(33.1780248209479,-54.6701838591725,0.0745739572701122));
#33830=CARTESIAN_POINT('Ctrl Pts',(33.7047869151672,-55.0120565441784,0.0375279937474315));
#33831=CARTESIAN_POINT('Ctrl Pts',(33.9673979456785,-55.4969804900557,0.00048203022475119));
#33832=CARTESIAN_POINT('Ctrl Pts',(34.2300089761898,-55.981904435933,-0.0365639332979294));
#33833=CARTESIAN_POINT('Ctrl Pts',(34.2284689429929,-56.6098796426817,-0.0736098968206097));
#33834=CARTESIAN_POINT('Ctrl Pts',(33.9634826195406,-57.0935097116441,-0.11065586034329));
#33835=CARTESIAN_POINT('Ctrl Pts',(33.8184586195722,-57.3581949459313,-0.130930694692264));
#33836=CARTESIAN_POINT('Ctrl Pts',(33.5945259126096,-57.579645226435,-0.151205529041238));
#33837=CARTESIAN_POINT('Ctrl Pts',(33.3313285320323,-57.7324067450656,-0.171480363390211));
#33838=CARTESIAN_POINT('Origin',(32.5,-56.2916512459885,3.));
#33839=CARTESIAN_POINT('',(33.3325354057626,-57.7362457052863,-0.871480363390211));
#33840=CARTESIAN_POINT('',(33.3348489584778,-57.7359240281238,-0.678519636609799));
#33841=CARTESIAN_POINT('',(33.333,-57.7344495686934,3.));
#33842=CARTESIAN_POINT('Ctrl Pts',(33.3348489584778,-57.7359240281238,-0.678519636609799));
#33843=CARTESIAN_POINT('Ctrl Pts',(33.3780386262143,-57.7113506256495,-0.675184574138161));
#33844=CARTESIAN_POINT('Ctrl Pts',(33.4200351242182,-57.6847625016212,-0.671849511666524));
#33845=CARTESIAN_POINT('Ctrl Pts',(33.4606301406774,-57.6561836376047,-0.668514449194886));
#33846=CARTESIAN_POINT('Ctrl Pts',(33.9115606739847,-57.3387288484125,-0.631468485672205));
#33847=CARTESIAN_POINT('Ctrl Pts',(34.1895648369722,-56.7756401144087,-0.594422522149525));
#33848=CARTESIAN_POINT('Ctrl Pts',(34.1674127214773,-56.2246182278545,-0.557376558626844));
#33849=CARTESIAN_POINT('Ctrl Pts',(34.1452606059824,-55.6735963413003,-0.520330595104164));
#33850=CARTESIAN_POINT('Ctrl Pts',(33.8229522120051,-55.1346413021957,-0.483284631581482));
#33851=CARTESIAN_POINT('Ctrl Pts',(33.3479936663214,-54.8544089200699,-0.446238668058801));
#33852=CARTESIAN_POINT('Ctrl Pts',(32.8730351206376,-54.5741765379442,-0.40919270453612));
#33853=CARTESIAN_POINT('Ctrl Pts',(32.2454264232473,-54.5526668127973,-0.37214674101344));
#33854=CARTESIAN_POINT('Ctrl Pts',(31.7523963222819,-54.7997238024578,-0.33510077749076));
#33855=CARTESIAN_POINT('Ctrl Pts',(31.2593662213165,-55.0467807921182,-0.298054813968079));
#33856=CARTESIAN_POINT('Ctrl Pts',(30.9009147167759,-55.562404496586,-0.261008850445398));
#33857=CARTESIAN_POINT('Ctrl Pts',(30.8410891376185,-56.1106167986295,-0.223962886922717));
#33858=CARTESIAN_POINT('Ctrl Pts',(30.7812635584611,-56.658829100673,-0.186916923400036));
#33859=CARTESIAN_POINT('Ctrl Pts',(31.020063904687,-57.2396300002922,-0.149870959877356));
#33860=CARTESIAN_POINT('Ctrl Pts',(31.4482018611622,-57.5872126749714,-0.112824996354675));
#33861=CARTESIAN_POINT('Ctrl Pts',(31.8763398176374,-57.9347953496505,-0.0757790328319943));
#33862=CARTESIAN_POINT('Ctrl Pts',(32.4938153843619,-58.0491597993897,-0.0387330693093137));
#33863=CARTESIAN_POINT('Ctrl Pts',(33.0180373581563,-57.8779664839892,-0.00168710578663283));
#33864=CARTESIAN_POINT('Ctrl Pts',(33.1273150883492,-57.8422800422406,0.00603538393897965));
#33865=CARTESIAN_POINT('Ctrl Pts',(33.2325405477213,-57.7941848839699,0.0137578736645921));
#33866=CARTESIAN_POINT('Ctrl Pts',(33.3319271105622,-57.7355745198861,0.0214803633902046));
#33867=CARTESIAN_POINT('Ctrl Pts',(33.3313285320323,-57.7324067450656,-0.171480363390211));
#33868=CARTESIAN_POINT('Ctrl Pts',(33.1136144342564,-57.8587694623943,-0.188251492563918));
#33869=CARTESIAN_POINT('Ctrl Pts',(32.8690337821938,-57.9381324168355,-0.205022621737625));
#33870=CARTESIAN_POINT('Ctrl Pts',(32.6200250231441,-57.9560888015458,-0.221793750911332));
#33871=CARTESIAN_POINT('Ctrl Pts',(32.0699863639079,-57.995752891309,-0.258839714434013));
#33872=CARTESIAN_POINT('Ctrl Pts',(31.4983416591433,-57.7357961396592,-0.295885677956694));
#33873=CARTESIAN_POINT('Ctrl Pts',(31.166707224731,-57.2951892897455,-0.332931641479374));
#33874=CARTESIAN_POINT('Ctrl Pts',(30.8350727903187,-56.8545824398317,-0.369977605002055));
#33875=CARTESIAN_POINT('Ctrl Pts',(30.7434486262587,-56.233325491654,-0.407023568524736));
#33876=CARTESIAN_POINT('Ctrl Pts',(30.9337672989981,-55.7157400874939,-0.444069532047416));
#33877=CARTESIAN_POINT('Ctrl Pts',(31.1240859717375,-55.1981546833338,-0.481115495570097));
#33878=CARTESIAN_POINT('Ctrl Pts',(31.5963474812762,-54.7842408231913,-0.518161459092778));
#33879=CARTESIAN_POINT('Ctrl Pts',(32.1344181757784,-54.6634287766856,-0.555207422615458));
#33880=CARTESIAN_POINT('Ctrl Pts',(32.6724888702806,-54.5426167301798,-0.592253386138139));
#33881=CARTESIAN_POINT('Ctrl Pts',(33.2763687497463,-54.7149064973108,-0.629299349660819));
#33882=CARTESIAN_POINT('Ctrl Pts',(33.6696897466081,-55.1014482025695,-0.6663453131835));
#33883=CARTESIAN_POINT('Ctrl Pts',(34.0630107434698,-55.4879899078282,-0.70339127670618));
#33884=CARTESIAN_POINT('Ctrl Pts',(34.2457728577278,-56.0887835512146,-0.74043724022886));
#33885=CARTESIAN_POINT('Ctrl Pts',(34.1343320137704,-56.6288734837568,-0.777483203751541));
#33886=CARTESIAN_POINT('Ctrl Pts',(34.040078625064,-57.0856656664133,-0.808815590297764));
#33887=CARTESIAN_POINT('Ctrl Pts',(33.7353736531391,-57.4990347912871,-0.840147976843988));
#33888=CARTESIAN_POINT('Ctrl Pts',(33.3325354057626,-57.7362457052863,-0.871480363390211));
#33889=CARTESIAN_POINT('Origin',(32.5,-56.2916512459885,3.));
#33890=CARTESIAN_POINT('',(33.3347882996638,-57.7351190113229,-1.57148036339021));
#33891=CARTESIAN_POINT('',(33.3327354544031,-57.732107437543,-1.3785196366098));
#33892=CARTESIAN_POINT('',(33.333,-57.7344495686934,3.));
#33893=CARTESIAN_POINT('',(32.8002165734083,-54.6529242983091,-2.));
#33894=CARTESIAN_POINT('Ctrl Pts',(33.3347882996638,-57.7351190113229,-1.57148036339021));
#33895=CARTESIAN_POINT('Ctrl Pts',(32.9233907544682,-57.9680931016246,-1.6031823516921));
#33896=CARTESIAN_POINT('Ctrl Pts',(32.4058309808294,-58.0231592569492,-1.63488433999399));
#33897=CARTESIAN_POINT('Ctrl Pts',(31.9592734257387,-57.8702645075936,-1.66658632829588));
#33898=CARTESIAN_POINT('Ctrl Pts',(31.4374400713406,-57.6915964299483,-1.70363229181856));
#33899=CARTESIAN_POINT('Ctrl Pts',(31.0125640599592,-57.2289465672062,-1.74067825534124));
#33900=CARTESIAN_POINT('Ctrl Pts',(30.880071382614,-56.6935519519194,-1.77772421886392));
#33901=CARTESIAN_POINT('Ctrl Pts',(30.7475787052688,-56.1581573366326,-1.8147701823866));
#33902=CARTESIAN_POINT('Ctrl Pts',(30.9074693619599,-55.5500179688011,-1.85181614590928));
#33903=CARTESIAN_POINT('Ctrl Pts',(31.2843999047331,-55.1487524209429,-1.88886210943196));
#33904=CARTESIAN_POINT('Ctrl Pts',(31.6613304475062,-54.7474868730848,-1.92590807295464));
#33905=CARTESIAN_POINT('Ctrl Pts',(32.2553008763614,-54.5530951452,-1.96295403647732));
#33906=CARTESIAN_POINT('Ctrl Pts',(32.8002165734083,-54.6529242983091,-2.));
#33907=CARTESIAN_POINT('',(34.0720885049227,-56.8521739755916,-2.));
#33908=CARTESIAN_POINT('Origin',(32.5,-56.2916512459885,-2.));
#33909=CARTESIAN_POINT('Ctrl Pts',(34.0720901513885,-56.8521746541717,-2.));
#33910=CARTESIAN_POINT('Ctrl Pts',(34.2530538927521,-56.3425577544552,-1.96367708181445));
#33911=CARTESIAN_POINT('Ctrl Pts',(34.16381751404,-55.7359288334824,-1.92735416362889));
#33912=CARTESIAN_POINT('Ctrl Pts',(33.8426356554964,-55.3008256611299,-1.89103124544334));
#33913=CARTESIAN_POINT('Ctrl Pts',(33.5150603391364,-54.8570613091241,-1.85398528192066));
#33914=CARTESIAN_POINT('Ctrl Pts',(32.9462134040812,-54.5917194685101,-1.81693931839798));
#33915=CARTESIAN_POINT('Ctrl Pts',(32.3958963008479,-54.6261577029506,-1.7798933548753));
#33916=CARTESIAN_POINT('Ctrl Pts',(31.8455791976147,-54.6605959373912,-1.74284739135262));
#33917=CARTESIAN_POINT('Ctrl Pts',(31.3137919262033,-54.9948142468862,-1.70580142782994));
#33918=CARTESIAN_POINT('Ctrl Pts',(31.0441775058384,-55.4758950021694,-1.66875546430726));
#33919=CARTESIAN_POINT('Ctrl Pts',(30.7745630854734,-55.9569757574525,-1.63170950078458));
#33920=CARTESIAN_POINT('Ctrl Pts',(30.7671215161549,-56.5849189585237,-1.5946635372619));
#33921=CARTESIAN_POINT('Ctrl Pts',(31.0251241525943,-57.0723230889947,-1.55761757373922));
#33922=CARTESIAN_POINT('Ctrl Pts',(31.2831267890336,-57.5597272194658,-1.52057161021654));
#33923=CARTESIAN_POINT('Ctrl Pts',(31.8065736312308,-57.9065922793366,-1.48352564669386));
#33924=CARTESIAN_POINT('Ctrl Pts',(32.3559737285805,-57.9541834292484,-1.44647968317118));
#33925=CARTESIAN_POINT('Ctrl Pts',(32.6919280642789,-57.9832850861845,-1.42382633431738));
#33926=CARTESIAN_POINT('Ctrl Pts',(33.0375869381561,-57.9004811240364,-1.40117298546359));
#33927=CARTESIAN_POINT('Ctrl Pts',(33.3327354544031,-57.732107437543,-1.3785196366098));
#33928=CARTESIAN_POINT('Origin',(32.5,-56.2916512459885,-3.54592528053767));
#33929=CARTESIAN_POINT('',(33.5296449158132,-58.0726582505549,6.54592528053768));
#33930=CARTESIAN_POINT('',(33.5251060574855,-58.0687922621904,6.60407471946232));
#33931=CARTESIAN_POINT('',(33.5273750000001,-58.0711169444146,-3.54592528053767));
#33932=CARTESIAN_POINT('',(30.8457462639859,-55.0728640868079,7.));
#33933=CARTESIAN_POINT('Ctrl Pts',(33.5251060574855,-58.0687922621904,6.60407471946233));
#33934=CARTESIAN_POINT('Ctrl Pts',(33.8584527741405,-57.8749712083972,6.62491192240684));
#33935=CARTESIAN_POINT('Ctrl Pts',(34.6426244289716,-57.0875348868182,6.68279508887404));
#33936=CARTESIAN_POINT('Ctrl Pts',(34.6192626691618,-55.1024844807854,6.77772421886392));
#33937=CARTESIAN_POINT('Ctrl Pts',(32.6468806392671,-53.8684656063833,6.88886210943196));
#33938=CARTESIAN_POINT('Ctrl Pts',(31.2510219905719,-54.522785363242,6.96295403647732));
#33939=CARTESIAN_POINT('Ctrl Pts',(30.8457462639859,-55.0728640868079,7.));
#33940=CARTESIAN_POINT('',(30.4546316093048,-56.0596663160167,7.));
#33941=CARTESIAN_POINT('Origin',(32.5,-56.2916512459885,7.));
#33942=CARTESIAN_POINT('Ctrl Pts',(33.5296449158132,-58.0726582505549,6.54592528053768));
#33943=CARTESIAN_POINT('Ctrl Pts',(33.5919384699578,-58.037273530125,6.54982271160486));
#33944=CARTESIAN_POINT('Ctrl Pts',(34.225323347054,-57.6301444802746,6.59076610619471));
#33945=CARTESIAN_POINT('Ctrl Pts',(34.9251107981772,-56.157415110224,6.66875546430726));
#33946=CARTESIAN_POINT('Ctrl Pts',(33.7019669024841,-54.1813822458926,6.7798933548753));
#33947=CARTESIAN_POINT('Ctrl Pts',(31.3950249125263,-54.1375954583441,6.8903082001062));
#33948=CARTESIAN_POINT('Ctrl Pts',(30.5306488143205,-55.3970288255657,6.96367708181445));
#33949=CARTESIAN_POINT('Ctrl Pts',(30.4546294175093,-56.0596661744469,7.));
#33950=CARTESIAN_POINT('Origin',(32.5,-56.2916512459885,-3.54592528053767));
#33951=CARTESIAN_POINT('',(33.5268493235952,-58.068153392458,5.84592528053768));
#33952=CARTESIAN_POINT('',(33.5270361074232,-58.0735254724117,5.90407471946233));
#33953=CARTESIAN_POINT('',(33.5273750000001,-58.0711169444146,-3.54592528053767));
#33954=CARTESIAN_POINT('Ctrl Pts',(33.5270361074232,-58.0735254724117,5.90407471946233));
#33955=CARTESIAN_POINT('Ctrl Pts',(34.0327197348534,-57.7760135322548,5.93596947460409));
#33956=CARTESIAN_POINT('Ctrl Pts',(34.8527930569705,-56.6438137488049,6.00491019326854));
#33957=CARTESIAN_POINT('Ctrl Pts',(34.1759192345576,-54.5338890939528,6.11089687545566));
#33958=CARTESIAN_POINT('Ctrl Pts',(31.9320786480218,-53.9303413264954,6.22203476602372));
#33959=CARTESIAN_POINT('Ctrl Pts',(30.2082245117244,-55.4880781765343,6.33317265659174));
#33960=CARTESIAN_POINT('Ctrl Pts',(30.5817368018815,-57.7814323658044,6.44431054715979));
#33961=CARTESIAN_POINT('Ctrl Pts',(32.3123519600731,-58.5366981066488,6.53461123478331));
#33962=CARTESIAN_POINT('Ctrl Pts',(33.265803638914,-58.2195610128864,6.58786595888416));
#33963=CARTESIAN_POINT('Ctrl Pts',(33.5251060574855,-58.0687922621904,6.60407471946233));
#33964=CARTESIAN_POINT('Ctrl Pts',(33.5268493235952,-58.068153392458,5.84592528053768));
#33965=CARTESIAN_POINT('Ctrl Pts',(33.7671186009377,-57.930879119519,5.86088026380211));
#33966=CARTESIAN_POINT('Ctrl Pts',(34.5085314004614,-57.2938049828724,5.91288121058922));
#33967=CARTESIAN_POINT('Ctrl Pts',(34.7788326566388,-55.451849617872,6.00192812089901));
#33968=CARTESIAN_POINT('Ctrl Pts',(33.0303393193103,-53.921614042038,6.11306601146705));
#33969=CARTESIAN_POINT('Ctrl Pts',(30.7964407564499,-54.5607069079647,6.22420390203509));
#33970=CARTESIAN_POINT('Ctrl Pts',(30.1217887402557,-56.7841397946826,6.33534179260313));
#33971=CARTESIAN_POINT('Ctrl Pts',(31.571340255844,-58.4946530906763,6.442582252104));
#33972=CARTESIAN_POINT('Ctrl Pts',(32.999824152922,-58.3736132984778,6.51277674808218));
#33973=CARTESIAN_POINT('Ctrl Pts',(33.5296449158132,-58.0726582505549,6.54592528053768));
#33974=CARTESIAN_POINT('Origin',(32.5,-56.2916512459885,-3.54592528053767));
#33975=CARTESIAN_POINT('',(33.525217808475,-58.0709111221528,5.14592528053768));
#33976=CARTESIAN_POINT('',(33.5295558866825,-58.0716265502945,5.20407471946233));
#33977=CARTESIAN_POINT('',(33.5273750000001,-58.0711169444146,-3.54592528053767));
#33978=CARTESIAN_POINT('Ctrl Pts',(33.5295558866825,-58.0716265502945,5.20407471946233));
#33979=CARTESIAN_POINT('Ctrl Pts',(33.6241634690101,-58.0180957001452,5.20998106327866));
#33980=CARTESIAN_POINT('Ctrl Pts',(34.2792376101367,-57.5737577801449,5.25293337061768));
#33981=CARTESIAN_POINT('Ctrl Pts',(34.9141240107243,-56.0264398256937,5.33293164147937));
#33982=CARTESIAN_POINT('Ctrl Pts',(33.5864678368826,-54.1195735160326,5.44406953204741));
#33983=CARTESIAN_POINT('Ctrl Pts',(31.2643540254432,-54.2008349824401,5.55520742261546));
#33984=CARTESIAN_POINT('Ctrl Pts',(30.0732435855651,-56.1958434964943,5.6663453131835));
#33985=CARTESIAN_POINT('Ctrl Pts',(31.10336564197,-58.2785475024108,5.77748320375154));
#33986=CARTESIAN_POINT('Ctrl Pts',(32.7493551050699,-58.4668353041202,5.85672633917782));
#33987=CARTESIAN_POINT('Ctrl Pts',(33.4453649446213,-58.1215755669412,5.89892351108141));
#33988=CARTESIAN_POINT('Ctrl Pts',(33.5270361074232,-58.0735254724117,5.90407471946233));
#33989=CARTESIAN_POINT('Ctrl Pts',(33.525217808475,-58.0709111221528,5.14592528053768));
#33990=CARTESIAN_POINT('Ctrl Pts',(33.9392806903329,-57.8273071486294,5.17193781599936));
#33991=CARTESIAN_POINT('Ctrl Pts',(34.7491747415829,-56.8889612418333,5.23499631498371));
#33992=CARTESIAN_POINT('Ctrl Pts',(34.4321757978777,-54.8202470274371,5.33510077749076));
#33993=CARTESIAN_POINT('Ctrl Pts',(32.3116949177892,-53.8703138209288,5.44623866805879));
#33994=CARTESIAN_POINT('Ctrl Pts',(30.3635721421369,-55.1366583239951,5.55737655862685));
#33995=CARTESIAN_POINT('Ctrl Pts',(30.370945362205,-57.4601807388668,5.66851444919488));
#33996=CARTESIAN_POINT('Ctrl Pts',(32.0638471781547,-58.5454001176689,5.7646973564985));
#33997=CARTESIAN_POINT('Ctrl Pts',(33.1719319178991,-58.2709301659147,5.82383430027943));
#33998=CARTESIAN_POINT('Ctrl Pts',(33.5268493235952,-58.068153392458,5.84592528053768));
#33999=CARTESIAN_POINT('Origin',(32.5,-56.2916512459885,-3.54592528053767));
#34000=CARTESIAN_POINT('',(33.5290839475038,-58.0740603739207,4.44592528053768));
#34001=CARTESIAN_POINT('',(33.5261619125927,-58.0680778657968,4.50407471946233));
#34002=CARTESIAN_POINT('',(33.5273750000001,-58.0711169444146,-3.54592528053767));
#34003=CARTESIAN_POINT('Ctrl Pts',(33.5261619125927,-58.0680778657968,4.50407471946233));
#34004=CARTESIAN_POINT('Ctrl Pts',(33.7984529813903,-57.9116108116526,4.52103861547591));
#34005=CARTESIAN_POINT('Ctrl Pts',(34.5559374767779,-57.225562580793,4.57504847501218));
#34006=CARTESIAN_POINT('Ctrl Pts',(34.7300884128151,-55.3298620761609,4.66610429807112));
#34007=CARTESIAN_POINT('Ctrl Pts',(32.9014225703573,-53.8964074829672,4.77724218863916));
#34008=CARTESIAN_POINT('Ctrl Pts',(30.7053300758282,-54.6553466763579,4.8883800792072));
#34009=CARTESIAN_POINT('Ctrl Pts',(30.1519193575992,-56.9120139865897,4.99951796977525));
#34010=CARTESIAN_POINT('Ctrl Pts',(31.6629249999102,-58.5111039532885,5.10474951652695));
#34011=CARTESIAN_POINT('Ctrl Pts',(33.0307626862479,-58.3538536552587,5.17293509975598));
#34012=CARTESIAN_POINT('Ctrl Pts',(33.5295558866825,-58.0716265502945,5.20407471946233));
#34013=CARTESIAN_POINT('Ctrl Pts',(33.5290839390052,-58.0740603592831,4.44592528053768));
#34014=CARTESIAN_POINT('Ctrl Pts',(33.5294675225899,-58.0738389277434,4.44594940467393));
#34015=CARTESIAN_POINT('Ctrl Pts',(34.1187763075119,-57.733369594267,4.48301949233286));
#34016=CARTESIAN_POINT('Ctrl Pts',(34.9257362810773,-56.410550559801,4.55713554351446));
#34017=CARTESIAN_POINT('Ctrl Pts',(33.91547832718,-54.3181379674856,4.66827343408251));
#34018=CARTESIAN_POINT('Ctrl Pts',(31.609617005159,-54.0321044593028,4.77941132465054));
#34019=CARTESIAN_POINT('Ctrl Pts',(30.1187333412011,-55.8142597516569,4.89054921521859));
#34020=CARTESIAN_POINT('Ctrl Pts',(30.8074500449804,-58.0333768894161,5.00168710578662));
#34021=CARTESIAN_POINT('Ctrl Pts',(32.5215758081834,-58.5120119076972,5.086812460893));
#34022=CARTESIAN_POINT('Ctrl Pts',(33.3495896761677,-58.1742377248673,5.13489185247668));
#34023=CARTESIAN_POINT('Ctrl Pts',(33.525217808475,-58.0709111221528,5.14592528053768));
#34024=CARTESIAN_POINT('Origin',(32.5,-56.2916512459885,-3.54592528053767));
#34025=CARTESIAN_POINT('',(33.5282587680711,-58.0691275396584,3.74592528053768));
#34026=CARTESIAN_POINT('',(33.5256537705603,-58.071893508325,3.80407471946232));
#34027=CARTESIAN_POINT('',(33.5273750000001,-58.0711169444146,-3.54592528053767));
#34028=CARTESIAN_POINT('Ctrl Pts',(33.5256537705603,-58.071893508325,3.80407471946232));
#34029=CARTESIAN_POINT('Ctrl Pts',(33.9708692323456,-57.8094153705276,3.83209616767316));
#34030=CARTESIAN_POINT('Ctrl Pts',(34.7867776966583,-56.8075863052296,3.89716357940668));
#34031=CARTESIAN_POINT('Ctrl Pts',(34.3497911057074,-54.7179277581866,3.99927695466287));
#34032=CARTESIAN_POINT('Ctrl Pts',(32.181049996069,-53.8840375630849,4.11041484523092));
#34033=CARTESIAN_POINT('Ctrl Pts',(30.3042474418304,-55.2538634762437,4.22155273579895));
#34034=CARTESIAN_POINT('Ctrl Pts',(30.4372421062834,-57.5735883041596,4.332690626367));
#34035=CARTESIAN_POINT('Ctrl Pts',(32.1498112942942,-58.5449642134686,4.42686462092145));
#34036=CARTESIAN_POINT('Ctrl Pts',(33.2038204161972,-58.2533054775293,4.48399265195323));
#34037=CARTESIAN_POINT('Ctrl Pts',(33.5261619125927,-58.0680778657968,4.50407471946233));
#34038=CARTESIAN_POINT('Ctrl Pts',(33.5282587680711,-58.0691275396585,3.74592528053768));
#34039=CARTESIAN_POINT('Ctrl Pts',(33.7063336904378,-57.9682446528084,3.75700695687118));
#34040=CARTESIAN_POINT('Ctrl Pts',(34.4133163086311,-57.41900891881,3.80513459672736));
#34041=CARTESIAN_POINT('Ctrl Pts',(34.8538786959893,-55.6936640901668,3.89030820010621));
#34042=CARTESIAN_POINT('Ctrl Pts',(33.2742100800909,-53.9897102593703,4.00144609067426));
#34043=CARTESIAN_POINT('Ctrl Pts',(30.9858981977034,-54.3927491193985,4.11258398124229));
#34044=CARTESIAN_POINT('Ctrl Pts',(30.0834608661246,-56.5338746309362,4.22372187181035));
#34045=CARTESIAN_POINT('Ctrl Pts',(31.3926249737445,-58.4528736933808,4.33483563824212));
#34046=CARTESIAN_POINT('Ctrl Pts',(32.9404216250933,-58.4138778272018,4.40890344115125));
#34047=CARTESIAN_POINT('Ctrl Pts',(33.5290839390052,-58.0740603592831,4.44592528053768));
#34048=CARTESIAN_POINT('Origin',(32.5,-56.2916512459885,-3.54592528053767));
#34049=CARTESIAN_POINT('',(33.5250673440976,-58.0691981786102,3.04592528053768));
#34050=CARTESIAN_POINT('',(33.5295277964003,-58.073488152934,3.10407471946232));
#34051=CARTESIAN_POINT('',(33.5273750000001,-58.0711169444146,-3.54592528053767));
#34052=CARTESIAN_POINT('Ctrl Pts',(33.5295277964003,-58.073488152934,3.10407471946232));
#34053=CARTESIAN_POINT('Ctrl Pts',(33.5619446593132,-58.0549578524537,3.10610775634773));
#34054=CARTESIAN_POINT('Ctrl Pts',(34.1744592271169,-57.6807192506861,3.14518675675581));
#34055=CARTESIAN_POINT('Ctrl Pts',(34.9286165141379,-56.2792182940979,3.22131172068658));
#34056=CARTESIAN_POINT('Ctrl Pts',(33.8067007722452,-54.2444908119128,3.33244961125462));
#34057=CARTESIAN_POINT('Ctrl Pts',(31.4887469945245,-54.0835524914147,3.44358750182266));
#34058=CARTESIAN_POINT('Ctrl Pts',(30.0964045610991,-55.9437120025227,3.5547253923907));
#34059=CARTESIAN_POINT('Ctrl Pts',(30.9041002915367,-58.1223442490711,3.66586328295875));
#34060=CARTESIAN_POINT('Ctrl Pts',(32.6005939960278,-58.4985054002164,3.74897972531595));
#34061=CARTESIAN_POINT('Ctrl Pts',(33.3822688276508,-58.1564265401567,3.79505020415048));
#34062=CARTESIAN_POINT('Ctrl Pts',(33.5256537705603,-58.071893508325,3.80407471946232));
#34063=CARTESIAN_POINT('Ctrl Pts',(33.5250673440976,-58.0691981786102,3.04592528053768));
#34064=CARTESIAN_POINT('Ctrl Pts',(33.8788897107516,-57.8627525499152,3.06806450906843));
#34065=CARTESIAN_POINT('Ctrl Pts',(34.6708999553705,-57.0389934359536,3.12724970112185));
#34066=CARTESIAN_POINT('Ctrl Pts',(34.5748652707907,-55.0294041774428,3.22348085669796));
#34067=CARTESIAN_POINT('Ctrl Pts',(32.5648065727292,-53.8638675525518,3.33461874726601));
#34068=CARTESIAN_POINT('Ctrl Pts',(30.4954296836915,-54.9205088752032,3.44575663783404));
#34069=CARTESIAN_POINT('Ctrl Pts',(30.2608587385459,-57.2321723596467,3.55689452840209));
#34070=CARTESIAN_POINT('Ctrl Pts',(31.8948295568209,-58.5383060176735,3.65695074263663));
#34071=CARTESIAN_POINT('Ctrl Pts',(33.1110305179061,-58.3054954110724,3.7199609933485));
#34072=CARTESIAN_POINT('Ctrl Pts',(33.5282587680711,-58.0691275396585,3.74592528053768));
#34073=CARTESIAN_POINT('Origin',(32.5,-56.2916512459885,-3.54592528053767));
#34074=CARTESIAN_POINT('',(33.5275894562264,-58.0738927599537,2.34592528053768));
#34075=CARTESIAN_POINT('',(33.5275355691898,-58.0684930935818,2.40407471946232));
#34076=CARTESIAN_POINT('',(33.5273750000001,-58.0711169444146,-3.54592528053767));
#34077=CARTESIAN_POINT('Ctrl Pts',(33.5275355691898,-58.0684930935818,2.40407471946232));
#34078=CARTESIAN_POINT('Ctrl Pts',(33.7379292069399,-57.9488445224074,2.41716530854498));
#34079=CARTESIAN_POINT('Ctrl Pts',(34.4632973547596,-57.3551041347746,2.46730186115031));
#34080=CARTESIAN_POINT('Ctrl Pts',(34.8181023612983,-55.5672658557593,2.55448437727833));
#34081=CARTESIAN_POINT('Ctrl Pts',(33.1486127133916,-53.9512166070675,2.66562226784637));
#34082=CARTESIAN_POINT('Ctrl Pts',(30.8854404931491,-54.4773937257142,2.77676015841441));
#34083=CARTESIAN_POINT('Ctrl Pts',(30.1000928998772,-56.6641813277477,2.88789804898245));
#34084=CARTESIAN_POINT('Ctrl Pts',(31.4855904228425,-58.4762227231017,2.99700290266509));
#34085=CARTESIAN_POINT('Ctrl Pts',(32.9712451350632,-58.3926166724123,3.06906179282505));
#34086=CARTESIAN_POINT('Ctrl Pts',(33.5295277964003,-58.073488152934,3.10407471946232));
#34087=CARTESIAN_POINT('Ctrl Pts',(33.5275894562264,-58.0738927599537,2.34592528053768));
#34088=CARTESIAN_POINT('Ctrl Pts',(34.0539010838894,-57.7651290399622,2.37912206126567));
#34089=CARTESIAN_POINT('Ctrl Pts',(34.8729207037989,-56.5867324218956,2.44936480551635));
#34090=CARTESIAN_POINT('Ctrl Pts',(34.113250907707,-54.4762297900261,2.55665351328972));
#34091=CARTESIAN_POINT('Ctrl Pts',(31.8496996873681,-53.9516847809773,2.66779140385775));
#34092=CARTESIAN_POINT('Ctrl Pts',(30.1813757180883,-55.5689376143779,2.7789292944258));
#34093=CARTESIAN_POINT('Ctrl Pts',(30.63531484903,-57.8476984309217,2.89006718499383));
#34094=CARTESIAN_POINT('Ctrl Pts',(32.3655977900595,-58.5319722593688,2.97906584703113));
#34095=CARTESIAN_POINT('Ctrl Pts',(33.2868324730584,-58.2082016796998,3.03101854554575));
#34096=CARTESIAN_POINT('Ctrl Pts',(33.5250673440976,-58.0691981786102,3.04592528053768));
#34097=CARTESIAN_POINT('Origin',(32.5,-56.2916512459885,-3.54592528053767));
#34098=CARTESIAN_POINT('',(33.5293464154415,-58.0709332657958,1.64592528053768));
#34099=CARTESIAN_POINT('',(33.5250295315601,-58.0700303972121,1.70407471946232));
#34100=CARTESIAN_POINT('',(33.5273750000001,-58.0711169444146,-3.54592528053767));
#34101=CARTESIAN_POINT('Ctrl Pts',(33.5250295315601,-58.0700303972121,1.70407471946232));
#34102=CARTESIAN_POINT('Ctrl Pts',(33.9101525759349,-57.8442238653441,1.72822286074223));
#34103=CARTESIAN_POINT('Ctrl Pts',(34.7124027752875,-56.9623029261605,1.78941696554481));
#34104=CARTESIAN_POINT('Ctrl Pts',(34.5035809067649,-54.9190637984713,1.88765703387008));
#34105=CARTESIAN_POINT('Ctrl Pts',(32.4334427362781,-53.863915082053,1.99879492443812));
#34106=CARTESIAN_POINT('Ctrl Pts',(30.4242251840868,-55.0309008088856,2.10993281500616));
#34107=CARTESIAN_POINT('Ctrl Pts',(30.3149878617883,-57.3518657086808,2.2210707055742));
#34108=CARTESIAN_POINT('Ctrl Pts',(31.9830137885335,-58.5433285166528,2.31911800705959));
#34109=CARTESIAN_POINT('Ctrl Pts',(33.1425216985167,-58.2874462900805,2.3801193450223));
#34110=CARTESIAN_POINT('Ctrl Pts',(33.5275355691898,-58.0684930935818,2.40407471946232));
#34111=CARTESIAN_POINT('Ctrl Pts',(33.5293464154415,-58.0709332657958,1.64592528053768));
#34112=CARTESIAN_POINT('Ctrl Pts',(33.6449437000377,-58.0055982631749,1.65313364994024));
#34113=CARTESIAN_POINT('Ctrl Pts',(34.3136427308233,-57.5361314802505,1.69738798286549));
#34114=CARTESIAN_POINT('Ctrl Pts',(34.90334407317,-55.9419787993381,1.77868827931342));
#34115=CARTESIAN_POINT('Ctrl Pts',(33.5096605171051,-54.0828236849995,1.88982616988146));
#34116=CARTESIAN_POINT('Ctrl Pts',(31.1918232394055,-54.2454334870425,2.0009640604495));
#34117=CARTESIAN_POINT('Ctrl Pts',(30.0713749864112,-56.2809696095364,2.11210195101754));
#34118=CARTESIAN_POINT('Ctrl Pts',(31.1738747508358,-58.326282755013,2.22323984158559));
#34119=CARTESIAN_POINT('Ctrl Pts',(32.7983102681658,-58.4546151165852,2.30118095142563));
#34120=CARTESIAN_POINT('Ctrl Pts',(33.4665633682319,-58.1096940627472,2.342076097743));
#34121=CARTESIAN_POINT('Ctrl Pts',(33.5275894562264,-58.0738927599537,2.34592528053768));
#34122=CARTESIAN_POINT('Origin',(32.5,-56.2916512459885,-3.54592528053767));
#34123=CARTESIAN_POINT('',(33.5257755155984,-58.068190352796,0.945925280537676));
#34124=CARTESIAN_POINT('',(33.5284289248676,-58.0741771517811,1.00407471946232));
#34125=CARTESIAN_POINT('',(33.5273750000001,-58.0711169444146,-3.54592528053767));
#34126=CARTESIAN_POINT('Ctrl Pts',(33.5284289248676,-58.0741771517811,1.00407471946232));
#34127=CARTESIAN_POINT('Ctrl Pts',(34.0870797198612,-57.748684668604,1.03928041293948));
#34128=CARTESIAN_POINT('Ctrl Pts',(34.9017444968086,-56.4966890376489,1.11153206993931));
#34129=CARTESIAN_POINT('Ctrl Pts',(34.0127319779433,-54.3916579002223,1.22082969046183));
#34130=CARTESIAN_POINT('Ctrl Pts',(31.7241302087767,-53.9902693093903,1.33196758102987));
#34131=CARTESIAN_POINT('Ctrl Pts',(30.1456908584837,-55.6953617045704,1.44310547159791));
#34132=CARTESIAN_POINT('Ctrl Pts',(30.7221773650996,-57.9462446793952,1.55424336216595));
#34133=CARTESIAN_POINT('Ctrl Pts',(32.4470927941984,-58.5226506382555,1.64123311145409));
#34134=CARTESIAN_POINT('Ctrl Pts',(33.3193305292905,-58.1906364710101,1.69117689721955));
#34135=CARTESIAN_POINT('Ctrl Pts',(33.5250295315601,-58.0700303972121,1.70407471946232));
#34136=CARTESIAN_POINT('Ctrl Pts',(33.5257755155984,-58.068190352796,0.945925280537677));
#34137=CARTESIAN_POINT('Ctrl Pts',(33.8187120383005,-57.8991957700279,0.964191202137494));
#34138=CARTESIAN_POINT('Ctrl Pts',(34.5858726429697,-57.180098149748,1.01950308725999));
#34139=CARTESIAN_POINT('Ctrl Pts',(34.6950037716947,-55.2522802841409,1.11186093590517));
#34140=CARTESIAN_POINT('Ctrl Pts',(32.8172137752097,-53.883808025427,1.22299882647321));
#34141=CARTESIAN_POINT('Ctrl Pts',(30.6490744128704,-54.7192619732989,1.33413671704125));
#34142=CARTESIAN_POINT('Ctrl Pts',(30.1751082313325,-56.9939416545676,1.44527460760929));
#34143=CARTESIAN_POINT('Ctrl Pts',(31.7218617398001,-58.5199646784861,1.54920412877477));
#34144=CARTESIAN_POINT('Ctrl Pts',(33.0508547252211,-58.341374357417,1.61608768641756));
#34145=CARTESIAN_POINT('Ctrl Pts',(33.5293464154415,-58.0709332657958,1.64592528053768));
#34146=CARTESIAN_POINT('Origin',(32.5,-56.2916512459885,-3.54592528053767));
#34147=CARTESIAN_POINT('',(33.5260517589603,-58.0725043954729,0.245925280537677));
#34148=CARTESIAN_POINT('',(33.5288532114794,-58.0699232317666,0.304074719462321));
#34149=CARTESIAN_POINT('',(33.5273750000001,-58.0711169444146,-3.54592528053767));
#34150=CARTESIAN_POINT('Ctrl Pts',(33.5288532114794,-58.0699232317667,0.304074719462322));
#34151=CARTESIAN_POINT('Ctrl Pts',(33.6768637713204,-57.9862464992859,0.313292001614045));
#34152=CARTESIAN_POINT('Ctrl Pts',(34.365857764272,-57.4763696079473,0.35955524728845));
#34153=CARTESIAN_POINT('Ctrl Pts',(34.8809216257836,-55.8125427394079,0.442864456485535));
#34154=CARTESIAN_POINT('Ctrl Pts',(33.388753307414,-54.0314631320695,0.554002347053576));
#34155=CARTESIAN_POINT('Ctrl Pts',(31.0830990069914,-54.3191593379889,0.665140237621618));
#34156=CARTESIAN_POINT('Ctrl Pts',(30.0743502545355,-56.4122997567237,0.77627812818966));
#34157=CARTESIAN_POINT('Ctrl Pts',(31.2858262226837,-58.3950092254139,0.887416018757702));
#34158=CARTESIAN_POINT('Ctrl Pts',(32.8728372110939,-58.4342824094917,0.963348215848589));
#34159=CARTESIAN_POINT('Ctrl Pts',(33.4992271616754,-58.0911912767045,1.0022344494168));
#34160=CARTESIAN_POINT('Ctrl Pts',(33.5284289248676,-58.0741771517811,1.00407471946232));
#34161=CARTESIAN_POINT('Ctrl Pts',(33.5260517589603,-58.0725043954729,0.245925280537675));
#34162=CARTESIAN_POINT('Ctrl Pts',(33.991498229918,-57.7980207394883,0.275248754334743));
#34163=CARTESIAN_POINT('Ctrl Pts',(34.8099603858882,-56.753542377561,0.34161819165449));
#34164=CARTESIAN_POINT('Ctrl Pts',(34.2934896049409,-54.6540528227808,0.445033592496919));
#34165=CARTESIAN_POINT('Ctrl Pts',(32.096850264347,-53.8966974164154,0.55617148306496));
#34166=CARTESIAN_POINT('Ctrl Pts',(30.2692184515671,-55.3314704112853,0.667309373633002));
#34167=CARTESIAN_POINT('Ctrl Pts',(30.4834462874739,-57.6451078131478,0.778447264201044));
#34168=CARTESIAN_POINT('Ctrl Pts',(32.2048796389797,-58.543263196541,0.871319233169268));
#34169=CARTESIAN_POINT('Ctrl Pts',(33.224593878142,-58.241941528272,0.927145238614813));
#34170=CARTESIAN_POINT('Ctrl Pts',(33.5257755155984,-58.068190352796,0.945925280537677));
#34171=CARTESIAN_POINT('Origin',(32.5,-56.2916512459885,-3.54592528053767));
#34172=CARTESIAN_POINT('',(33.5296554006196,-58.0729354591292,-0.454074719462323));
#34173=CARTESIAN_POINT('',(33.5253135061185,-58.0685974415039,-0.395925280537675));
#34174=CARTESIAN_POINT('',(33.5273750000001,-58.0711169444146,-3.54592528053767));
#34175=CARTESIAN_POINT('Ctrl Pts',(33.5253135061185,-58.0685974415039,-0.395925280537677));
#34176=CARTESIAN_POINT('Ctrl Pts',(33.8499262418575,-57.8801900402997,-0.375650446188704));
#34177=CARTESIAN_POINT('Ctrl Pts',(34.6307561402675,-57.1080161029863,-0.31832964831705));
#34178=CARTESIAN_POINT('Ctrl Pts',(34.6355944339958,-55.1351180442909,-0.223962886922716));
#34179=CARTESIAN_POINT('Ctrl Pts',(32.6865588761979,-53.8701788494842,-0.112824996354674));
#34180=CARTESIAN_POINT('Ctrl Pts',(30.5667638241697,-54.8216408199215,-0.00168710578663165));
#34181=CARTESIAN_POINT('Ctrl Pts',(30.2164817879238,-57.1186199946645,0.109450784781409));
#34182=CARTESIAN_POINT('Ctrl Pts',(31.8120346004307,-58.5309407947376,0.211371393197728));
#34183=CARTESIAN_POINT('Ctrl Pts',(33.081981927564,-58.322558779647,0.276246038091365));
#34184=CARTESIAN_POINT('Ctrl Pts',(33.5288532114794,-58.0699232317667,0.304074719462322));
#34185=CARTESIAN_POINT('Ctrl Pts',(33.5296554006196,-58.0729354591292,-0.454074719462325));
#34186=CARTESIAN_POINT('Ctrl Pts',(33.5829230895642,-58.0426280169118,-0.450739656990688));
#34187=CARTESIAN_POINT('Ctrl Pts',(34.2100716718942,-57.645578141716,-0.410358630996372));
#34188=CARTESIAN_POINT('Ctrl Pts',(34.926688116847,-56.1940939537869,-0.332931641479374));
#34189=CARTESIAN_POINT('Ctrl Pts',(33.7341373860101,-54.1999441339785,-0.221793750911332));
#34190=CARTESIAN_POINT('Ctrl Pts',(31.4119663698708,-54.1203575053852,-0.11065586034329));
#34191=CARTESIAN_POINT('Ctrl Pts',(30.0856850452223,-56.0281806868171,0.000482030224751475));
#34192=CARTESIAN_POINT('Ctrl Pts',(30.9692534931351,-58.1771614464075,0.111619920792793));
#34193=CARTESIAN_POINT('Ctrl Pts',(32.6511246141561,-58.4886656996171,0.193434337563768));
#34194=CARTESIAN_POINT('Ctrl Pts',(33.4034740038597,-58.1447910975144,0.238202790812062));
#34195=CARTESIAN_POINT('Ctrl Pts',(33.5260517589603,-58.0725043954729,0.245925280537675));
#34196=CARTESIAN_POINT('Origin',(32.5,-56.2916512459885,-3.54592528053767));
#34197=CARTESIAN_POINT('',(33.5270487244507,-58.0682282925652,-1.15407471946232));
#34198=CARTESIAN_POINT('',(33.5268019957928,-58.0733321975144,-1.09592528053768));
#34199=CARTESIAN_POINT('',(33.5273750000001,-58.0711169444146,-3.54592528053767));
#34200=CARTESIAN_POINT('Ctrl Pts',(33.5268019957928,-58.0733321975144,-1.09592528053768));
#34201=CARTESIAN_POINT('Ctrl Pts',(34.0236398642182,-57.7807696971903,-1.06459289399145));
#34202=CARTESIAN_POINT('Ctrl Pts',(34.8437811491657,-56.6681489116154,-0.996214543922551));
#34203=CARTESIAN_POINT('Ctrl Pts',(34.2023204507043,-54.559476051911,-0.890790230330967));
#34204=CARTESIAN_POINT('Ctrl Pts',(31.9679467730355,-53.921998742765,-0.779652339762925));
#34205=CARTESIAN_POINT('Ctrl Pts',(30.2205650142273,-55.453492447677,-0.668514449194883));
#34206=CARTESIAN_POINT('Ctrl Pts',(30.5595771710743,-57.7521618011011,-0.557376558626841));
#34207=CARTESIAN_POINT('Ctrl Pts',(32.2888225453055,-58.5385401346075,-0.466513502407773));
#34208=CARTESIAN_POINT('Ctrl Pts',(33.2567972741827,-58.2244460570089,-0.412696409711385));
#34209=CARTESIAN_POINT('Ctrl Pts',(33.5253135061185,-58.0685974415039,-0.395925280537677));
#34210=CARTESIAN_POINT('Ctrl Pts',(33.5270487244507,-58.0682282925651,-1.15407471946232));
#34211=CARTESIAN_POINT('Ctrl Pts',(33.7583254242685,-57.9362916288018,-1.13968210479344));
#34212=CARTESIAN_POINT('Ctrl Pts',(34.4950254817816,-57.3125020026611,-1.08824352660187));
#34213=CARTESIAN_POINT('Ctrl Pts',(34.7912737376158,-55.4864512354733,-0.999758984887625));
#34214=CARTESIAN_POINT('Ctrl Pts',(33.0661792001092,-53.929919412126,-0.888621094319583));
#34215=CARTESIAN_POINT('Ctrl Pts',(30.822833264184,-54.5351044086332,-0.777483203751541));
#34216=CARTESIAN_POINT('Ctrl Pts',(30.1146276885619,-56.7480782089188,-0.6663453131835));
#34217=CARTESIAN_POINT('Ctrl Pts',(31.5455083936008,-58.4894074878943,-0.558542485087093));
#34218=CARTESIAN_POINT('Ctrl Pts',(32.9912241698707,-58.3792838991923,-0.487785620513369));
#34219=CARTESIAN_POINT('Ctrl Pts',(33.5296554006196,-58.0729354591292,-0.454074719462325));
#34220=CARTESIAN_POINT('Origin',(32.5,-56.2916512459885,-3.54592528053767));
#34221=CARTESIAN_POINT('',(33.5243188290626,-58.0704843676252,-1.85407471946232));
#34222=CARTESIAN_POINT('',(33.5295805874755,-58.0719425970214,-1.79592528053768));
#34223=CARTESIAN_POINT('',(33.5273750000001,-58.0711169444146,-3.54592528053767));
#34224=CARTESIAN_POINT('',(31.0458737116219,-57.7433792852397,-2.));
#34225=CARTESIAN_POINT('Ctrl Pts',(31.0458737116219,-57.7433792852397,-2.));
#34226=CARTESIAN_POINT('Ctrl Pts',(31.5286078227264,-58.2269108712356,-1.96295403647732));
#34227=CARTESIAN_POINT('Ctrl Pts',(32.4987857659728,-58.5150960016803,-1.91431227629809));
#34228=CARTESIAN_POINT('Ctrl Pts',(33.339589876325,-58.1790057138554,-1.86567051611887));
#34229=CARTESIAN_POINT('Ctrl Pts',(33.5243188290626,-58.0704843676252,-1.85407471946232));
#34230=CARTESIAN_POINT('',(30.5120522999331,-56.8258916115682,-2.));
#34231=CARTESIAN_POINT('Origin',(32.5,-56.2916512459885,-2.));
#34232=CARTESIAN_POINT('Ctrl Pts',(30.5120501580915,-56.825892077386,-2.));
#34233=CARTESIAN_POINT('Ctrl Pts',(30.6859814099171,-57.4697983977034,-1.96367708181445));
#34234=CARTESIAN_POINT('Ctrl Pts',(31.6524845810096,-58.5050100533593,-1.89565217532701));
#34235=CARTESIAN_POINT('Ctrl Pts',(33.0221861661125,-58.3592796390667,-1.82762726883957));
#34236=CARTESIAN_POINT('Ctrl Pts',(33.5295805874755,-58.0719425970214,-1.79592528053768));
#34237=CARTESIAN_POINT('Origin',(63.7511045350785,17.0820569767664,10.));
#34238=CARTESIAN_POINT('',(60.9122168113323,13.7189801527801,9.99965378812963));
#34239=CARTESIAN_POINT('',(60.6472937215209,13.6458118873637,9.99664393251001));
#34240=CARTESIAN_POINT('',(64.4026814811241,14.6503387090836,10.));
#34241=CARTESIAN_POINT('',(60.3826426720153,14.1985145724513,11.6359872033747));
#34242=CARTESIAN_POINT('Ctrl Pts',(60.6472937215209,13.6458118873637,9.99664393251001));
#34243=CARTESIAN_POINT('Ctrl Pts',(60.6097205320263,13.6410407802455,10.5892058593235));
#34244=CARTESIAN_POINT('Ctrl Pts',(60.5187326677745,13.8356159531908,11.1848035603042));
#34245=CARTESIAN_POINT('Ctrl Pts',(60.3826426720153,14.1985145724514,11.6359872033748));
#34246=CARTESIAN_POINT('',(59.3912531651588,17.8984305821304,11.6380816927071));
#34247=CARTESIAN_POINT('Origin',(59.8874012299222,16.0467807963563,10.));
#34248=CARTESIAN_POINT('Ctrl Pts',(59.3912467107623,17.8984546702662,11.6380966037225));
#34249=CARTESIAN_POINT('Ctrl Pts',(59.5701794123024,17.4212611177616,12.2270179049202));
#34250=CARTESIAN_POINT('Ctrl Pts',(59.8253574740883,16.659516006978,12.567422198156));
#34251=CARTESIAN_POINT('Ctrl Pts',(60.0736878712827,15.9233267283634,12.5157167035403));
#34252=CARTESIAN_POINT('Ctrl Pts',(60.3360206084697,15.1456267338052,12.4610957466079));
#34253=CARTESIAN_POINT('Ctrl Pts',(60.5907116859352,14.3964458015818,11.9688993897472));
#34254=CARTESIAN_POINT('Ctrl Pts',(60.7469740189126,14.014605944713,11.2575578209417));
#34255=CARTESIAN_POINT('Ctrl Pts',(60.8300361143405,13.8116368860468,10.8794403300265));
#34256=CARTESIAN_POINT('Ctrl Pts',(60.8852870497793,13.7124604894775,10.4394030962359));
#34257=CARTESIAN_POINT('Ctrl Pts',(60.9122168113323,13.7189801527801,9.99965378812962));
#34258=CARTESIAN_POINT('Origin',(63.7511045350785,17.0820569767664,10.));
#34259=CARTESIAN_POINT('',(61.8799991994799,13.9708704146993,9.99901528063939));
#34260=CARTESIAN_POINT('',(61.614467077582,13.8999750879731,10.0012573013837));
#34261=CARTESIAN_POINT('',(64.4026814811241,14.6503387090836,10.));
#34262=CARTESIAN_POINT('Ctrl Pts',(61.614467077582,13.8999750879731,10.0012573013837));
#34263=CARTESIAN_POINT('Ctrl Pts',(61.6099667912196,13.8982899610888,10.0766544396887));
#34264=CARTESIAN_POINT('Ctrl Pts',(61.6045451170745,13.900043500223,10.1520128061815));
#34265=CARTESIAN_POINT('Ctrl Pts',(61.5981695663354,13.9053569552699,10.2270376921985));
#34266=CARTESIAN_POINT('Ctrl Pts',(61.5284611611194,13.9634527171371,11.047337830936));
#34267=CARTESIAN_POINT('Ctrl Pts',(61.3447206686645,14.4471220222725,11.8277717281245));
#34268=CARTESIAN_POINT('Ctrl Pts',(61.1066011161457,15.1337367424348,12.2189611289229));
#34269=CARTESIAN_POINT('Ctrl Pts',(60.8684815636268,15.8203514625971,12.6101505297212));
#34270=CARTESIAN_POINT('Ctrl Pts',(60.5759829510439,16.7099115977863,12.6120954341293));
#34271=CARTESIAN_POINT('Ctrl Pts',(60.3374667150895,17.3980067606845,12.2237523563129));
#34272=CARTESIAN_POINT('Ctrl Pts',(60.0989504791351,18.0861019235826,11.8354092784964));
#34273=CARTESIAN_POINT('Ctrl Pts',(59.9144166198093,18.5727321141896,11.0567782184554));
#34274=CARTESIAN_POINT('Ctrl Pts',(59.8438645695582,18.6339764021913,10.2368654679638));
#34275=CARTESIAN_POINT('Ctrl Pts',(59.7733125193071,18.6952206901929,9.41695271747214));
#34276=CARTESIAN_POINT('Ctrl Pts',(59.8167422781307,18.3310790755891,8.55575827652985));
#34277=CARTESIAN_POINT('Ctrl Pts',(59.932110753931,17.6984585141966,8.03819621078674));
#34278=CARTESIAN_POINT('Ctrl Pts',(60.0474792297314,17.0658379528042,7.52063414504363));
#34279=CARTESIAN_POINT('Ctrl Pts',(60.2347864225085,16.1647384446231,7.34670445449967));
#34280=CARTESIAN_POINT('Ctrl Pts',(60.3874931590402,15.392769597115,7.59575134544314));
#34281=CARTESIAN_POINT('Ctrl Pts',(60.540199895572,14.6208007496069,7.84479823638661));
#34282=CARTESIAN_POINT('Ctrl Pts',(60.6583061758583,13.9779625627717,8.51682170881751));
#34283=CARTESIAN_POINT('Ctrl Pts',(60.6663289586339,13.7459615817213,9.30743209219171));
#34284=CARTESIAN_POINT('Ctrl Pts',(60.6685946628634,13.6804424696227,9.5307073994776));
#34285=CARTESIAN_POINT('Ctrl Pts',(60.6620806891943,13.6476895615158,9.76344057197144));
#34286=CARTESIAN_POINT('Ctrl Pts',(60.6472937215209,13.6458118873637,9.99664393251001));
#34287=CARTESIAN_POINT('Ctrl Pts',(60.9122168113323,13.7189801527801,9.99965378812962));
#34288=CARTESIAN_POINT('Ctrl Pts',(60.9359492362449,13.7247257446778,9.61211536100745));
#34289=CARTESIAN_POINT('Ctrl Pts',(60.9376863320054,13.8125590225005,9.22480054821085));
#34290=CARTESIAN_POINT('Ctrl Pts',(60.9170790299751,13.9837827281427,8.88028612326221));
#34291=CARTESIAN_POINT('Ctrl Pts',(60.8730881195708,14.3492981499552,8.14484277513855));
#34292=CARTESIAN_POINT('Ctrl Pts',(60.7272727102727,15.0948277750946,7.60444285964154));
#34293=CARTESIAN_POINT('Ctrl Pts',(60.5669204894781,15.8946095193188,7.49935843056474));
#34294=CARTESIAN_POINT('Ctrl Pts',(60.4065682686835,16.694391263543,7.39427400148793));
#34295=CARTESIAN_POINT('Ctrl Pts',(60.2316792363924,17.5484251268522,7.72450505883134));
#34296=CARTESIAN_POINT('Ctrl Pts',(60.1424305723414,18.0828447847106,8.34320956294502));
#34297=CARTESIAN_POINT('Ctrl Pts',(60.0531819082903,18.617264442569,8.96191406705869));
#34298=CARTESIAN_POINT('Ctrl Pts',(60.0495736124794,18.8320698949766,9.86909201794265));
#34299=CARTESIAN_POINT('Ctrl Pts',(60.1556096340356,18.6376771842086,10.6611508664113));
#34300=CARTESIAN_POINT('Ctrl Pts',(60.2616456555918,18.4432844734405,11.4532097148801));
#34301=CARTESIAN_POINT('Ctrl Pts',(60.4773259945153,17.8396935994968,12.1301494609335));
#34302=CARTESIAN_POINT('Ctrl Pts',(60.7290924921509,17.1014273477893,12.3908459426517));
#34303=CARTESIAN_POINT('Ctrl Pts',(60.9808589897866,16.3631610960817,12.6515424243699));
#34304=CARTESIAN_POINT('Ctrl Pts',(61.2687116461343,15.4902194666104,12.4959956417528));
#34305=CARTESIAN_POINT('Ctrl Pts',(61.4869914228006,14.8769273589395,11.9933937214366));
#34306=CARTESIAN_POINT('Ctrl Pts',(61.6896056365773,14.3076501674883,11.5268626736099));
#34307=CARTESIAN_POINT('Ctrl Pts',(61.8322748736988,13.9620906745726,10.7613040129743));
#34308=CARTESIAN_POINT('Ctrl Pts',(61.8799991994799,13.9708704146993,9.99901528063939));
#34309=CARTESIAN_POINT('Origin',(63.7511045350785,17.0820569767664,10.));
#34310=CARTESIAN_POINT('',(62.8445369550162,14.2348698103755,10.0018466754434));
#34311=CARTESIAN_POINT('',(62.5785998445538,14.1654859215485,10.0004462653845));
#34312=CARTESIAN_POINT('',(64.4026814811241,14.6503387090836,10.));
#34313=CARTESIAN_POINT('Ctrl Pts',(62.5785998445538,14.1654859215485,10.0004462653845));
#34314=CARTESIAN_POINT('Ctrl Pts',(62.5552558244195,14.1585827534688,10.3867702486341));
#34315=CARTESIAN_POINT('Ctrl Pts',(62.5100553152291,14.2332491130213,10.7728367424032));
#34316=CARTESIAN_POINT('Ctrl Pts',(62.4426252563818,14.3908772813227,11.1164878478952));
#34317=CARTESIAN_POINT('Ctrl Pts',(62.2977170112848,14.7296226663468,11.8549994178656));
#34318=CARTESIAN_POINT('Ctrl Pts',(62.0501467519025,15.4515079046906,12.397625364221));
#34319=CARTESIAN_POINT('Ctrl Pts',(61.7881520526304,16.2272258855741,12.501389418797));
#34320=CARTESIAN_POINT('Ctrl Pts',(61.5261573533583,17.0029438664577,12.605153473373));
#34321=CARTESIAN_POINT('Ctrl Pts',(61.2497382141963,17.832494589881,12.2700556361696));
#34322=CARTESIAN_POINT('Ctrl Pts',(61.0600503079339,18.3383599455201,11.646143814324));
#34323=CARTESIAN_POINT('Ctrl Pts',(60.8703624016714,18.8442253011592,11.0222319924783));
#34324=CARTESIAN_POINT('Ctrl Pts',(60.7674057283085,19.0264052890141,10.1095061859904));
#34325=CARTESIAN_POINT('Ctrl Pts',(60.7746625458238,18.7972629292321,9.31667252204681));
#34326=CARTESIAN_POINT('Ctrl Pts',(60.7819193633391,18.5681205694502,8.52383885810325));
#34327=CARTESIAN_POINT('Ctrl Pts',(60.8993896717325,17.9276558620313,7.85089733670406));
#34328=CARTESIAN_POINT('Ctrl Pts',(61.0518532638259,17.1565944419206,7.59916807226838));
#34329=CARTESIAN_POINT('Ctrl Pts',(61.2043168559193,16.3855330218099,7.3474388078327));
#34330=CARTESIAN_POINT('Ctrl Pts',(61.3917737317127,15.4838748890073,7.51692180036051));
#34331=CARTESIAN_POINT('Ctrl Pts',(61.5076640106207,14.8493069319055,8.03174648676759));
#34332=CARTESIAN_POINT('Ctrl Pts',(61.6129549313732,14.2727767422054,8.49948515966272));
#34333=CARTESIAN_POINT('Ctrl Pts',(61.6591716047613,13.9167146450877,9.25228420341931));
#34334=CARTESIAN_POINT('Ctrl Pts',(61.614467077582,13.8999750879731,10.0012573013837));
#34335=CARTESIAN_POINT('Ctrl Pts',(61.8799991994799,13.9708704146993,9.99901528063939));
#34336=CARTESIAN_POINT('Ctrl Pts',(61.8836891105328,13.971549239588,9.94007725327275));
#34337=CARTESIAN_POINT('Ctrl Pts',(61.8868114457663,13.9743462862715,9.88115877337008));
#34338=CARTESIAN_POINT('Ctrl Pts',(61.8893500282724,13.9793219277933,9.82239956232278));
#34339=CARTESIAN_POINT('Ctrl Pts',(61.9247219600932,14.0486511901886,9.00366438154032));
#34340=CARTESIAN_POINT('Ctrl Pts',(61.84675892675,14.5409523008496,8.21585107799066));
#34341=CARTESIAN_POINT('Ctrl Pts',(61.712535142454,15.243221392539,7.80941972573588));
#34342=CARTESIAN_POINT('Ctrl Pts',(61.5783113581579,15.9454904842284,7.4029883734811));
#34343=CARTESIAN_POINT('Ctrl Pts',(61.3878268229089,16.8577275569461,7.37793897252118));
#34344=CARTESIAN_POINT('Ctrl Pts',(61.2482107604141,17.5801209048418,7.74541574302332));
#34345=CARTESIAN_POINT('Ctrl Pts',(61.1085946979193,18.3025142527376,8.11289251352547));
#34346=CARTESIAN_POINT('Ctrl Pts',(61.0198471081785,18.8350638758114,8.8728954554897));
#34347=CARTESIAN_POINT('Ctrl Pts',(61.0438394390411,18.9468623871525,9.6873337892666));
#34348=CARTESIAN_POINT('Ctrl Pts',(61.0678317699037,19.0586608984936,10.5017721230435));
#34349=CARTESIAN_POINT('Ctrl Pts',(61.2045640213697,18.749708298102,11.370645848633));
#34350=CARTESIAN_POINT('Ctrl Pts',(61.4156018821482,18.1634433884681,11.9074332417686));
#34351=CARTESIAN_POINT('Ctrl Pts',(61.6266397429268,17.5771784788342,12.4442206349041));
#34352=CARTESIAN_POINT('Ctrl Pts',(61.9119832130179,16.7136012599581,12.6489216955856));
#34353=CARTESIAN_POINT('Ctrl Pts',(62.1670877632026,15.9628772265393,12.4304742338454));
#34354=CARTESIAN_POINT('Ctrl Pts',(62.4221923133873,15.2121531931204,12.2120267721052));
#34355=CARTESIAN_POINT('Ctrl Pts',(62.6470579436654,14.5742823451588,11.5704307879433));
#34356=CARTESIAN_POINT('Ctrl Pts',(62.7640438959386,14.3390239366156,10.7911028658272));
#34357=CARTESIAN_POINT('Ctrl Pts',(62.8020535673526,14.2625865983512,10.537892991755));
#34358=CARTESIAN_POINT('Ctrl Pts',(62.8286748982889,14.2286511253629,10.2701434172214));
#34359=CARTESIAN_POINT('Ctrl Pts',(62.8445369550162,14.2348698103755,10.0018466754434));
#34360=CARTESIAN_POINT('Origin',(63.7511045350785,17.0820569767664,10.));
#34361=CARTESIAN_POINT('',(63.8107147438123,14.4927485186002,9.99793352624083));
#34362=CARTESIAN_POINT('',(63.5459612763502,14.4189472139579,9.9981100037851));
#34363=CARTESIAN_POINT('',(64.4026814811241,14.6503387090836,10.));
#34364=CARTESIAN_POINT('Ctrl Pts',(63.5459612763502,14.4189472139579,9.9981100037851));
#34365=CARTESIAN_POINT('Ctrl Pts',(63.5020657997403,14.4131993125783,10.6909216248416));
#34366=CARTESIAN_POINT('Ctrl Pts',(63.3825723034678,14.6895870615306,11.3881278716997));
#34367=CARTESIAN_POINT('Ctrl Pts',(63.2084966963919,15.1696780211856,11.8560065223221));
#34368=CARTESIAN_POINT('Ctrl Pts',(63.0010658835769,15.7417608055527,12.4135369565263));
#34369=CARTESIAN_POINT('Ctrl Pts',(62.7161316220184,16.6030903983924,12.6454354329572));
#34370=CARTESIAN_POINT('Ctrl Pts',(62.4586624096387,17.3619190322645,12.4478622804133));
#34371=CARTESIAN_POINT('Ctrl Pts',(62.201193197259,18.1207476661366,12.2502891278695));
#34372=CARTESIAN_POINT('Ctrl Pts',(61.9711890340581,18.7770753410411,11.6232443463508));
#34373=CARTESIAN_POINT('Ctrl Pts',(61.8490217755359,19.0309502087539,10.8475065234706));
#34374=CARTESIAN_POINT('Ctrl Pts',(61.7268545170136,19.2848250764668,10.0717687005904));
#34375=CARTESIAN_POINT('Ctrl Pts',(61.7125241631699,19.136247136988,9.14733783634869));
#34376=CARTESIAN_POINT('Ctrl Pts',(61.7898279718489,18.6456858472656,8.48815640829364));
#34377=CARTESIAN_POINT('Ctrl Pts',(61.867131780528,18.1551245575431,7.82897498023858));
#34378=CARTESIAN_POINT('Ctrl Pts',(62.0360697517297,17.3225799175771,7.43504298837021));
#34379=CARTESIAN_POINT('Ctrl Pts',(62.1983751106924,16.5147885234738,7.48275547481141));
#34380=CARTESIAN_POINT('Ctrl Pts',(62.3606804696551,15.7069971293706,7.53046796125261));
#34381=CARTESIAN_POINT('Ctrl Pts',(62.5163532163788,14.9239589811301,8.01982492600339));
#34382=CARTESIAN_POINT('Ctrl Pts',(62.5730664743348,14.5102426728621,8.73170200517146));
#34383=CARTESIAN_POINT('Ctrl Pts',(62.6033893890854,14.2890407035395,9.11232178902007));
#34384=CARTESIAN_POINT('Ctrl Pts',(62.6054224867212,14.1734177690261,9.55655400073804));
#34385=CARTESIAN_POINT('Ctrl Pts',(62.5785998445538,14.1654859215485,10.0004462653845));
#34386=CARTESIAN_POINT('Ctrl Pts',(62.8445369550162,14.2348698103755,10.0018466754434));
#34387=CARTESIAN_POINT('Ctrl Pts',(62.8774950470096,14.2477909590166,9.44438121878217));
#34388=CARTESIAN_POINT('Ctrl Pts',(62.8640028840737,14.4340668190784,8.88455351560662));
#34389=CARTESIAN_POINT('Ctrl Pts',(62.8097033887246,14.7726377170274,8.44788099502234));
#34390=CARTESIAN_POINT('Ctrl Pts',(62.729270654969,15.2741558751071,7.80104690640396));
#34391=CARTESIAN_POINT('Ctrl Pts',(62.5592989131896,16.1098381603915,7.42443858923753));
#34392=CARTESIAN_POINT('Ctrl Pts',(62.3977923938505,16.913927805431,7.48559176785146));
#34393=CARTESIAN_POINT('Ctrl Pts',(62.2362858745114,17.7180174504704,7.5467449464654));
#34394=CARTESIAN_POINT('Ctrl Pts',(62.0832445776126,18.490514455265,8.04565962085973));
#34395=CARTESIAN_POINT('Ctrl Pts',(62.0291411621378,18.8937702597925,8.76039160250516));
#34396=CARTESIAN_POINT('Ctrl Pts',(61.9750377466629,19.2970260643199,9.47512358415059));
#34397=CARTESIAN_POINT('Ctrl Pts',(62.0198722126119,19.3310406685804,10.4056728730471));
#34398=CARTESIAN_POINT('Ctrl Pts',(62.1660913946905,18.9866823611344,11.138080910744));
#34399=CARTESIAN_POINT('Ctrl Pts',(62.312310576769,18.6423240536885,11.8704889484409));
#34400=CARTESIAN_POINT('Ctrl Pts',(62.5599144749771,17.9195928345362,12.4047557349382));
#34401=CARTESIAN_POINT('Ctrl Pts',(62.8211471346509,17.1459983851495,12.5032105584454));
#34402=CARTESIAN_POINT('Ctrl Pts',(63.0823797943247,16.3724039357629,12.6016653819527));
#34403=CARTESIAN_POINT('Ctrl Pts',(63.3572412154642,15.5479462561419,12.2643082424698));
#34404=CARTESIAN_POINT('Ctrl Pts',(63.5458498251155,15.0453884512907,11.6412138093996));
#34405=CARTESIAN_POINT('Ctrl Pts',(63.6819468306564,14.6827506455303,11.1915986689941));
#34406=CARTESIAN_POINT('Ctrl Pts',(63.7731333897311,14.4877209077723,10.5932047327949));
#34407=CARTESIAN_POINT('Ctrl Pts',(63.8107147438123,14.4927485186002,9.99793352624083));
#34408=CARTESIAN_POINT('Origin',(63.7511045350785,17.0820569767664,10.));
#34409=CARTESIAN_POINT('',(64.7775781358098,14.7480685208434,10.0015051238181));
#34410=CARTESIAN_POINT('',(64.511567991272,14.6789571988966,10.0021294030496));
#34411=CARTESIAN_POINT('',(64.4026814811241,14.6503387090836,10.));
#34412=CARTESIAN_POINT('Ctrl Pts',(64.511567991272,14.6789571988966,10.0021294030496));
#34413=CARTESIAN_POINT('Ctrl Pts',(64.5012097288919,14.6745624451438,10.1782532036584));
#34414=CARTESIAN_POINT('Ctrl Pts',(64.4860602506939,14.6880487522533,10.354078307347));
#34415=CARTESIAN_POINT('Ctrl Pts',(64.4658270415774,14.7205078014429,10.5257161206906));
#34416=CARTESIAN_POINT('Ctrl Pts',(64.3708655262953,14.8728494531259,11.3312723100704));
#34417=CARTESIAN_POINT('Ctrl Pts',(64.163921993672,15.4431136830602,12.0445928505661));
#34418=CARTESIAN_POINT('Ctrl Pts',(63.9150421900725,16.1698862069573,12.3462664892695));
#34419=CARTESIAN_POINT('Ctrl Pts',(63.6661623864731,16.8966587308544,12.6479401279729));
#34420=CARTESIAN_POINT('Ctrl Pts',(63.3753463118975,17.7799395487143,12.5379668648842));
#34421=CARTESIAN_POINT('Ctrl Pts',(63.1501962278718,18.4181515535133,12.0655906176062));
#34422=CARTESIAN_POINT('Ctrl Pts',(62.925046143846,19.0563635583122,11.5932143703281));
#34423=CARTESIAN_POINT('Ctrl Pts',(62.76556205037,19.4495067500502,10.7584351388608));
#34424=CARTESIAN_POINT('Ctrl Pts',(62.7205382674991,19.4154782471595,9.93505104704534));
#34425=CARTESIAN_POINT('Ctrl Pts',(62.6755144846283,19.3814497442687,9.11166695522985));
#34426=CARTESIAN_POINT('Ctrl Pts',(62.7449510123626,18.9202495467492,8.2996780030662));
#34427=CARTESIAN_POINT('Ctrl Pts',(62.8751359084421,18.2323333520888,7.8626772661126));
#34428=CARTESIAN_POINT('Ctrl Pts',(63.0053208045215,17.5444171574285,7.425676529159));
#34429=CARTESIAN_POINT('Ctrl Pts',(63.1962540689461,16.6297849656272,7.36366400741544));
#34430=CARTESIAN_POINT('Ctrl Pts',(63.3398198518216,15.8919306215938,7.70440771629217));
#34431=CARTESIAN_POINT('Ctrl Pts',(63.4833856346971,15.1540762775605,8.04515142516891));
#34432=CARTESIAN_POINT('Ctrl Pts',(63.5795839360234,14.592999781295,8.78865136466594));
#34433=CARTESIAN_POINT('Ctrl Pts',(63.5627194046509,14.4538795211095,9.60198253040318));
#34434=CARTESIAN_POINT('Ctrl Pts',(63.5600075610921,14.4315087612499,9.73276747984737));
#34435=CARTESIAN_POINT('Ctrl Pts',(63.5543722345421,14.4200485884486,9.86535806600962));
#34436=CARTESIAN_POINT('Ctrl Pts',(63.5459612763502,14.4189472139579,9.9981100037851));
#34437=CARTESIAN_POINT('Ctrl Pts',(63.8107147438123,14.4927485186002,9.99793352624083));
#34438=CARTESIAN_POINT('Ctrl Pts',(63.8252151156581,14.494688369579,9.7682543660517));
#34439=CARTESIAN_POINT('Ctrl Pts',(63.8317351659301,14.5264111861321,9.53904009330699));
#34440=CARTESIAN_POINT('Ctrl Pts',(63.8297754611263,14.5897808794637,9.3190160464461));
#34441=CARTESIAN_POINT('Ctrl Pts',(63.8227366893229,14.8173890425695,8.52874444322035));
#34442=CARTESIAN_POINT('Ctrl Pts',(63.7063033475529,15.4532632988625,7.85703296342644));
#34443=CARTESIAN_POINT('Ctrl Pts',(63.5546628984882,16.2205322683665,7.60269513736945));
#34444=CARTESIAN_POINT('Ctrl Pts',(63.4030224494236,16.9878012378706,7.34835731131246));
#34445=CARTESIAN_POINT('Ctrl Pts',(63.2161748930644,17.8864649205859,7.51139313899242));
#34446=CARTESIAN_POINT('Ctrl Pts',(63.0996317362701,18.522749012129,8.01927548227232));
#34447=CARTESIAN_POINT('Ctrl Pts',(62.9830885794757,19.1590331036721,8.52715782555223));
#34448=CARTESIAN_POINT('Ctrl Pts',(62.9368498222464,19.5329376040432,9.37988668443209));
#34449=CARTESIAN_POINT('Ctrl Pts',(63.0038765864645,19.4841294236266,10.1981222260488));
#34450=CARTESIAN_POINT('Ctrl Pts',(63.0709033506826,19.43532124321,11.0163577676655));
#34451=CARTESIAN_POINT('Ctrl Pts',(63.2511956363482,18.9638003820057,11.8000999920191));
#34452=CARTESIAN_POINT('Ctrl Pts',(63.4869413276822,18.2853245933941,12.2006980454406));
#34453=CARTESIAN_POINT('Ctrl Pts',(63.7226870190161,17.6068488047825,12.6012960988622));
#34454=CARTESIAN_POINT('Ctrl Pts',(64.0138861160186,16.7214180887636,12.6187499813517));
#34455=CARTESIAN_POINT('Ctrl Pts',(64.253389165651,16.02891964808,12.2452952639449));
#34456=CARTESIAN_POINT('Ctrl Pts',(64.4928922152834,15.3364212073964,11.871840546538));
#34457=CARTESIAN_POINT('Ctrl Pts',(64.6806992175459,14.8368550420482,11.1074772292348));
#34458=CARTESIAN_POINT('Ctrl Pts',(64.755655105023,14.7584549707696,10.2922353809894));
#34459=CARTESIAN_POINT('Ctrl Pts',(64.7645194286933,14.7491833360657,10.195824440425));
#34460=CARTESIAN_POINT('Ctrl Pts',(64.7718054668758,14.7458019429916,10.0987019353608));
#34461=CARTESIAN_POINT('Ctrl Pts',(64.7775781358098,14.7480685208434,10.0015051238181));
#34462=CARTESIAN_POINT('Origin',(63.7511045350785,17.0820569767664,10.));
#34463=CARTESIAN_POINT('',(65.7418454548454,15.0130771992805,9.99981028982562));
#34464=CARTESIAN_POINT('',(65.4764820235065,14.9415523108175,9.99892236192922));
#34465=CARTESIAN_POINT('',(64.4026814811241,14.6503387090836,10.));
#34466=CARTESIAN_POINT('Ctrl Pts',(65.4764820235065,14.9415523108175,9.99892236192922));
#34467=CARTESIAN_POINT('Ctrl Pts',(65.4463344353996,14.9354685130878,10.4860098738008));
#34468=CARTESIAN_POINT('Ctrl Pts',(65.3812875674044,15.0596306010493,10.9740976137645));
#34469=CARTESIAN_POINT('Ctrl Pts',(65.2832167053678,15.3070399126418,11.3788468299413));
#34470=CARTESIAN_POINT('Ctrl Pts',(65.1161273209563,15.7285664365572,12.0684430664547));
#34471=CARTESIAN_POINT('Ctrl Pts',(64.8531757502037,16.5078555104223,12.5161238918082));
#34472=CARTESIAN_POINT('Ctrl Pts',(64.5894870640691,17.2898955363443,12.5214264196761));
#34473=CARTESIAN_POINT('Ctrl Pts',(64.3257983779344,18.0719355622663,12.526728947544));
#34474=CARTESIAN_POINT('Ctrl Pts',(64.0613725764177,18.8567265402451,12.0896531779262));
#34475=CARTESIAN_POINT('Ctrl Pts',(63.8919948632527,19.2867932233327,11.4059132558295));
#34476=CARTESIAN_POINT('Ctrl Pts',(63.7226171500878,19.7168599064204,10.7221733337328));
#34477=CARTESIAN_POINT('Ctrl Pts',(63.6482875252747,19.7922022946169,9.7917692591572));
#34478=CARTESIAN_POINT('Ctrl Pts',(63.6796697714155,19.4730226094499,9.03131812620868));
#34479=CARTESIAN_POINT('Ctrl Pts',(63.7110520175564,19.153842924283,8.27086699326015));
#34480=CARTESIAN_POINT('Ctrl Pts',(63.8481461346512,18.4401411657526,7.68036880193875));
#34481=CARTESIAN_POINT('Ctrl Pts',(64.0069444100312,17.6454383857665,7.524237313639));
#34482=CARTESIAN_POINT('Ctrl Pts',(64.1657426854112,16.8507356057803,7.36810582533925));
#34483=CARTESIAN_POINT('Ctrl Pts',(64.3462451190763,15.9750318043384,7.64634104006116));
#34484=CARTESIAN_POINT('Ctrl Pts',(64.4450065869384,15.4043894403333,8.23435456655407));
#34485=CARTESIAN_POINT('Ctrl Pts',(64.5227251994293,14.9553323969431,8.6970815429164));
#34486=CARTESIAN_POINT('Ctrl Pts',(64.5498246710713,14.6951885590369,9.35164270965612));
#34487=CARTESIAN_POINT('Ctrl Pts',(64.511567991272,14.6789571988966,10.0021294030496));
#34488=CARTESIAN_POINT('Ctrl Pts',(64.7775781358098,14.7480685208434,10.0015051238181));
#34489=CARTESIAN_POINT('Ctrl Pts',(64.8206186125989,14.7649679121881,9.27681483601603));
#34490=CARTESIAN_POINT('Ctrl Pts',(64.7795300848962,15.0958410226864,8.54799381140139));
#34491=CARTESIAN_POINT('Ctrl Pts',(64.6812188924136,15.6402720254874,8.07917134860806));
#34492=CARTESIAN_POINT('Ctrl Pts',(64.5697220196355,16.2577231286926,7.54746954365975));
#34493=CARTESIAN_POINT('Ctrl Pts',(64.3846235013876,17.1498593123119,7.35018631295075));
#34494=CARTESIAN_POINT('Ctrl Pts',(64.23065677798,17.9258100558562,7.57508388624565));
#34495=CARTESIAN_POINT('Ctrl Pts',(64.0766900545725,18.7017607994006,7.79998145954056));
#34496=CARTESIAN_POINT('Ctrl Pts',(63.9538551260052,19.3615261028699,8.44705983683936));
#34497=CARTESIAN_POINT('Ctrl Pts',(63.9391872263039,19.6176065589079,9.22846362604928));
#34498=CARTESIAN_POINT('Ctrl Pts',(63.9245193266025,19.873687014946,10.0098674152592));
#34499=CARTESIAN_POINT('Ctrl Pts',(64.0180184557671,19.7260826235527,10.9255966163803));
#34500=CARTESIAN_POINT('Ctrl Pts',(64.200482779956,19.2464556042235,11.5682854345738));
#34501=CARTESIAN_POINT('Ctrl Pts',(64.3829471041448,18.7668285848942,12.2109742527672));
#34502=CARTESIAN_POINT('Ctrl Pts',(64.654376623358,17.9551789376289,12.5806226880332));
#34503=CARTESIAN_POINT('Ctrl Pts',(64.916416459657,17.1785720640666,12.5127911771402));
#34504=CARTESIAN_POINT('Ctrl Pts',(65.1784562959559,16.4019651905042,12.4449596662473));
#34505=CARTESIAN_POINT('Ctrl Pts',(65.4311064493406,15.6604010906447,11.9396482091956));
#34506=CARTESIAN_POINT('Ctrl Pts',(65.5843661188994,15.2897673262124,11.2216465877776));
#34507=CARTESIAN_POINT('Ctrl Pts',(65.6632851643038,15.0989143577318,10.8519211229877));
#34508=CARTESIAN_POINT('Ctrl Pts',(65.7158498370977,15.0064172468355,10.4257987515067));
#34509=CARTESIAN_POINT('Ctrl Pts',(65.7418454548454,15.0130771992805,9.99981028982562));
#34510=CARTESIAN_POINT('Origin',(63.7511045350785,17.0820569767664,10.));
#34511=CARTESIAN_POINT('',(66.709565290414,15.2652009106025,9.99881345470567));
#34512=CARTESIAN_POINT('',(66.4442667934687,15.1934336836835,9.99943462192776));
#34513=CARTESIAN_POINT('',(64.4026814811241,14.6503387090836,10.));
#34514=CARTESIAN_POINT('Ctrl Pts',(66.4442667934687,15.1934336836835,9.99943462192776));
#34515=CARTESIAN_POINT('Ctrl Pts',(66.3950965524831,15.1827995799555,10.7909504295074));
#34516=CARTESIAN_POINT('Ctrl Pts',(66.242026625676,15.5599243826036,11.5846294221379));
#34517=CARTESIAN_POINT('Ctrl Pts',(66.0272275066145,16.1674256670555,12.0468004663334));
#34518=CARTESIAN_POINT('Ctrl Pts',(65.8036660249293,16.7997089272065,12.5278249876806));
#34519=CARTESIAN_POINT('Ctrl Pts',(65.5132363543,17.6815476659072,12.6497433013673));
#34520=CARTESIAN_POINT('Ctrl Pts',(65.2633677075892,18.4120106025366,12.3579626123137));
#34521=CARTESIAN_POINT('Ctrl Pts',(65.0134990608784,19.1424735391661,12.06618192326));
#34522=CARTESIAN_POINT('Ctrl Pts',(64.8041914380861,19.7215606737244,11.3607022314659));
#34523=CARTESIAN_POINT('Ctrl Pts',(64.7065491918251,19.8839069496221,10.5574238638963));
#34524=CARTESIAN_POINT('Ctrl Pts',(64.608906945564,20.0462532255198,9.75414549632672));
#34525=CARTESIAN_POINT('Ctrl Pts',(64.6229300758342,19.7918586427569,8.85306845298168));
#34526=CARTESIAN_POINT('Ctrl Pts',(64.7197196907436,19.2285753341563,8.2576777189159));
#34527=CARTESIAN_POINT('Ctrl Pts',(64.816509305653,18.6652920255557,7.66228698485014));
#34528=CARTESIAN_POINT('Ctrl Pts',(64.9960654052016,17.7931199911174,7.37258256006362));
#34529=CARTESIAN_POINT('Ctrl Pts',(65.1553666185042,16.9965402212509,7.51828854147109));
#34530=CARTESIAN_POINT('Ctrl Pts',(65.3146678318069,16.1999604513844,7.66399452287857));
#34531=CARTESIAN_POINT('Ctrl Pts',(65.4537141588635,15.4789729460896,8.24511091048004));
#34532=CARTESIAN_POINT('Ctrl Pts',(65.4876237233566,15.1503611804251,9.00142492811739));
#34533=CARTESIAN_POINT('Ctrl Pts',(65.5016305260266,15.0146236613656,9.31383062721454));
#34534=CARTESIAN_POINT('Ctrl Pts',(65.4976987431426,14.9458338550092,9.65612879778036));
#34535=CARTESIAN_POINT('Ctrl Pts',(65.4764820235065,14.9415523108175,9.99892236192922));
#34536=CARTESIAN_POINT('Ctrl Pts',(65.7418454548454,15.0130771992805,9.99981028982562));
#34537=CARTESIAN_POINT('Ctrl Pts',(65.7663329589547,15.0193507802528,9.59853518618479));
#34538=CARTESIAN_POINT('Ctrl Pts',(65.7672447483348,15.1136101264191,9.19737890571013));
#34539=CARTESIAN_POINT('Ctrl Pts',(65.744401378692,15.2965249330007,8.84359325274525));
#34540=CARTESIAN_POINT('Ctrl Pts',(65.6973077831931,15.6736197332262,8.11423332491524));
#34541=CARTESIAN_POINT('Ctrl Pts',(65.5492514064624,16.4275127626822,7.58620525503953));
#34542=CARTESIAN_POINT('Ctrl Pts',(65.3884873478827,17.2288315064447,7.49440429239112));
#34543=CARTESIAN_POINT('Ctrl Pts',(65.2277232893031,18.0301502502071,7.40260332974272));
#34544=CARTESIAN_POINT('Ctrl Pts',(65.0542515488746,18.8788947082761,7.74702947432164));
#34545=CARTESIAN_POINT('Ctrl Pts',(64.9676333413308,19.4034973688025,8.37446367269953));
#34546=CARTESIAN_POINT('Ctrl Pts',(64.8810151337869,19.9281000293289,9.00189787107742));
#34547=CARTESIAN_POINT('Ctrl Pts',(64.8812504591278,20.1285608923127,9.91234012325428));
#34548=CARTESIAN_POINT('Ctrl Pts',(64.9906262726288,19.9217039083204,10.7007759738115));
#34549=CARTESIAN_POINT('Ctrl Pts',(65.1000020861297,19.7148469243281,11.4892118243687));
#34550=CARTESIAN_POINT('Ctrl Pts',(65.3185183877907,19.1006720933596,12.1556412733063));
#34551=CARTESIAN_POINT('Ctrl Pts',(65.5713589268319,18.3583974645568,12.4036017192683));
#34552=CARTESIAN_POINT('Ctrl Pts',(65.8241994658732,17.616122835754,12.6515621652302));
#34553=CARTESIAN_POINT('Ctrl Pts',(66.1113642422948,16.7457484091169,12.4810536082165));
#34554=CARTESIAN_POINT('Ctrl Pts',(66.3274985456645,16.1404633167949,11.9679250313905));
#34555=CARTESIAN_POINT('Ctrl Pts',(66.5245294039924,15.5886775085546,11.5001503082284));
#34556=CARTESIAN_POINT('Ctrl Pts',(66.662531210899,15.2571911193414,10.7476451883995));
#34557=CARTESIAN_POINT('Ctrl Pts',(66.709565290414,15.2652009106025,9.99881345470567));
#34558=CARTESIAN_POINT('Origin',(63.7511045350785,17.0820569767664,10.));
#34559=CARTESIAN_POINT('',(67.6742507328171,15.5286491313886,10.0019962882659));
#34560=CARTESIAN_POINT('',(67.4086397233445,15.458048217099,10.0018117506529));
#34561=CARTESIAN_POINT('',(64.4026814811241,14.6503387090836,10.));
#34562=CARTESIAN_POINT('',(67.0040126136404,20.25986904378,11.1728309286208));
#34563=CARTESIAN_POINT('Ctrl Pts',(67.6742507328171,15.5286491313886,10.0019962882659));
#34564=CARTESIAN_POINT('Ctrl Pts',(67.7079511930089,15.5421457071954,9.43113200366987));
#34565=CARTESIAN_POINT('Ctrl Pts',(67.6927226550025,15.7382477902416,8.8576382151147));
#34566=CARTESIAN_POINT('Ctrl Pts',(67.635211832767,16.0921495062908,8.41584216487544));
#34567=CARTESIAN_POINT('Ctrl Pts',(67.5520689427972,16.6037821050588,7.77714150008993));
#34568=CARTESIAN_POINT('Ctrl Pts',(67.3805551035975,17.4452195762655,7.41369214583754));
#34569=CARTESIAN_POINT('Ctrl Pts',(67.2193238791372,18.2482818068304,7.48861537411896));
#34570=CARTESIAN_POINT('Ctrl Pts',(67.0580926546768,19.0513440373952,7.56353860240038));
#34571=CARTESIAN_POINT('Ctrl Pts',(66.9071440449558,19.8160310273183,8.07683441321561));
#34572=CARTESIAN_POINT('Ctrl Pts',(66.8561932299011,20.2075211669018,8.79681637620264));
#34573=CARTESIAN_POINT('Ctrl Pts',(66.8052424148463,20.5990113064853,9.51679833918967));
#34574=CARTESIAN_POINT('Ctrl Pts',(66.854289394458,20.6173045957293,10.4434664543485));
#34575=CARTESIAN_POINT('Ctrl Pts',(67.0040126136404,20.25986904378,11.1728309286208));
#34576=CARTESIAN_POINT('',(68.0323660008166,16.4802525979518,11.8670505687058));
#34577=CARTESIAN_POINT('Ctrl Pts',(68.0322473001841,16.4806955947433,11.8669181223571));
#34578=CARTESIAN_POINT('Ctrl Pts',(67.9835336336721,16.6817854205938,12.0540417240897));
#34579=CARTESIAN_POINT('Ctrl Pts',(67.9238765324049,16.9239334961962,12.2143044024353));
#34580=CARTESIAN_POINT('Ctrl Pts',(67.7816176378542,17.4856657502708,12.4543153408643));
#34581=CARTESIAN_POINT('Ctrl Pts',(67.6966288605656,17.8119729521746,12.5175));
#34582=CARTESIAN_POINT('Ctrl Pts',(67.5329868199039,18.4226933621783,12.5175));
#34583=CARTESIAN_POINT('Ctrl Pts',(67.4434356591205,18.7477780771091,12.4543153408643));
#34584=CARTESIAN_POINT('Ctrl Pts',(67.274655929957,19.3446857260753,12.1973867613172));
#34585=CARTESIAN_POINT('Ctrl Pts',(67.1955448337828,19.6165425195547,12.003644350162));
#34586=CARTESIAN_POINT('Ctrl Pts',(67.0834304248293,19.9960747381914,11.6080270340044));
#34587=CARTESIAN_POINT('Ctrl Pts',(67.0387983068925,20.1448248140073,11.4009948671634));
#34588=CARTESIAN_POINT('Ctrl Pts',(67.0040126136404,20.25986904378,11.1728309286208));
#34589=CARTESIAN_POINT('Ctrl Pts',(68.0330516124712,16.4776938604227,11.8678155752478));
#34590=CARTESIAN_POINT('Ctrl Pts',(67.8522271893252,16.9785524830602,12.3404055365588));
#34591=CARTESIAN_POINT('Ctrl Pts',(67.6166367512168,17.6838006560656,12.5855412104357));
#34592=CARTESIAN_POINT('Ctrl Pts',(67.3907294446844,18.3529108900531,12.5051234941037));
#34593=CARTESIAN_POINT('Ctrl Pts',(67.1283727946319,19.129979689639,12.4117306641613));
#34594=CARTESIAN_POINT('Ctrl Pts',(66.8790760319582,19.8583083259861,11.879255644893));
#34595=CARTESIAN_POINT('Ctrl Pts',(66.7317311985187,20.2061471825013,11.1455779206959));
#34596=CARTESIAN_POINT('Ctrl Pts',(66.5843863650793,20.5539860390166,10.4119001964987));
#34597=CARTESIAN_POINT('Ctrl Pts',(66.5389934608741,20.5213351156999,9.47701976737268));
#34598=CARTESIAN_POINT('Ctrl Pts',(66.5933174195301,20.1165357938135,8.75982961781548));
#34599=CARTESIAN_POINT('Ctrl Pts',(66.6476413781862,19.7117364719271,8.04263946825828));
#34600=CARTESIAN_POINT('Ctrl Pts',(66.8016821997035,18.934788751471,7.54313959826992));
#34601=CARTESIAN_POINT('Ctrl Pts',(66.9638149498406,18.1276415422747,7.48486270274577));
#34602=CARTESIAN_POINT('Ctrl Pts',(67.1259476999777,17.3204943330785,7.42658580722162));
#34603=CARTESIAN_POINT('Ctrl Pts',(67.2961723787346,16.483147635142,7.80953188616167));
#34604=CARTESIAN_POINT('Ctrl Pts',(67.3756602454435,15.9844353298855,8.46229096311828));
#34605=CARTESIAN_POINT('Ctrl Pts',(67.4285455390929,15.6526293851286,8.89658813193756));
#34606=CARTESIAN_POINT('Ctrl Pts',(67.4412654718215,15.4707226080322,9.45032013874419));
#34607=CARTESIAN_POINT('Ctrl Pts',(67.4086397233445,15.458048217099,10.0018117506529));
#34608=CARTESIAN_POINT('Origin',(69.7479810832458,18.6889152049569,10.));
#34609=CARTESIAN_POINT('',(61.4484819638689,13.2791651259751,10.0015349814512));
#34610=CARTESIAN_POINT('',(61.3659731009889,13.2658134652031,9.99957732584559));
#34611=CARTESIAN_POINT('',(70.5434614183684,15.7201421778575,10.0000000000001));
#34612=CARTESIAN_POINT('',(59.681950857614,16.8135320242448,7.03077704625437));
#34613=CARTESIAN_POINT('Ctrl Pts',(61.3659731009889,13.2658134652031,9.99957732584559));
#34614=CARTESIAN_POINT('Ctrl Pts',(61.3390049028546,13.2594372491749,10.5364470372516));
#34615=CARTESIAN_POINT('Ctrl Pts',(61.1616793186458,13.6128633281576,12.0843271181651));
#34616=CARTESIAN_POINT('Ctrl Pts',(60.4026582657957,15.9358673415302,13.6055385422089));
#34617=CARTESIAN_POINT('Ctrl Pts',(59.447210195013,18.8976307583478,12.2029441264611));
#34618=CARTESIAN_POINT('Ctrl Pts',(59.1533281063616,19.3903963172923,8.83503768583792));
#34619=CARTESIAN_POINT('Ctrl Pts',(59.4806667221929,17.7660737535059,7.2906822312505));
#34620=CARTESIAN_POINT('Ctrl Pts',(59.6819508576139,16.8135320242448,7.03077704625438));
#34621=CARTESIAN_POINT('',(60.0933746109221,15.2780776734582,7.02605498021599));
#34622=CARTESIAN_POINT('Origin',(59.8874012299222,16.0467807963563,10.));
#34623=CARTESIAN_POINT('Ctrl Pts',(61.4484819638689,13.2791651259751,10.0015349814512));
#34624=CARTESIAN_POINT('Ctrl Pts',(61.4440081401684,13.277381239092,10.0935838809865));
#34625=CARTESIAN_POINT('Ctrl Pts',(61.3771948495716,13.3061918618692,11.1915036202383));
#34626=CARTESIAN_POINT('Ctrl Pts',(60.9313710113775,14.5474295567701,13.1842383274677));
#34627=CARTESIAN_POINT('Ctrl Pts',(59.8935459365979,17.8144668208753,13.1913616605739));
#34628=CARTESIAN_POINT('Ctrl Pts',(59.2511484715134,19.6057481548832,10.3395770770156));
#34629=CARTESIAN_POINT('Ctrl Pts',(59.4407261981541,18.3013616530663,7.23382086599183));
#34630=CARTESIAN_POINT('Ctrl Pts',(59.9014396609592,16.1871423562507,6.78116218790437));
#34631=CARTESIAN_POINT('Ctrl Pts',(60.0933772939441,15.2780676602836,7.02603075613026));
#34632=CARTESIAN_POINT('Origin',(69.7479810832458,18.6889152049569,10.));
#34633=CARTESIAN_POINT('',(62.4122187264791,13.5461538679481,10.0005448248896));
#34634=CARTESIAN_POINT('',(62.3341655182897,13.5161734774897,9.99879780140841));
#34635=CARTESIAN_POINT('',(70.5434614183684,15.7201421778575,10.0000000000001));
#34636=CARTESIAN_POINT('Ctrl Pts',(62.3341655182897,13.5161734774897,9.99879780140841));
#34637=CARTESIAN_POINT('Ctrl Pts',(62.286219899295,13.5082196148795,10.9294410660881));
#34638=CARTESIAN_POINT('Ctrl Pts',(61.9458317508115,14.3903370215027,12.870975191806));
#34639=CARTESIAN_POINT('Ctrl Pts',(60.949326866107,17.5197763142875,13.4270461480336));
#34640=CARTESIAN_POINT('Ctrl Pts',(60.1927341524847,19.7394014348252,10.947712313481));
#34641=CARTESIAN_POINT('Ctrl Pts',(60.2392996738452,18.96159921589,7.62511676387808));
#34642=CARTESIAN_POINT('Ctrl Pts',(60.9131915231956,15.8425832679708,6.41562502038855));
#34643=CARTESIAN_POINT('Ctrl Pts',(61.3800631690209,13.6032001394547,8.04417985348944));
#34644=CARTESIAN_POINT('Ctrl Pts',(61.389739398956,13.2714326411404,9.52644947847322));
#34645=CARTESIAN_POINT('Ctrl Pts',(61.3659731009889,13.2658134652031,9.99957732584559));
#34646=CARTESIAN_POINT('Ctrl Pts',(62.4122187264791,13.5461538679481,10.0005448248896));
#34647=CARTESIAN_POINT('Ctrl Pts',(62.3889104933502,13.5391171409457,10.4721900135758));
#34648=CARTESIAN_POINT('Ctrl Pts',(62.231485488278,13.8305514728694,11.9564181322135));
#34649=CARTESIAN_POINT('Ctrl Pts',(61.5138509672066,16.0106566332716,13.5896176377583));
#34650=CARTESIAN_POINT('Ctrl Pts',(60.5349179618126,19.0579057022675,12.3623010109723));
#34651=CARTESIAN_POINT('Ctrl Pts',(60.1913020034494,19.734119272829,9.01938609588907));
#34652=CARTESIAN_POINT('Ctrl Pts',(60.6550135466888,17.3973455890623,6.55469600728483));
#34653=CARTESIAN_POINT('Ctrl Pts',(61.3531034969372,14.2043402063785,7.15651357330655));
#34654=CARTESIAN_POINT('Ctrl Pts',(61.4929236187117,13.2968857360054,9.087148162546));
#34655=CARTESIAN_POINT('Ctrl Pts',(61.4484819638689,13.2791651259751,10.0015349814512));
#34656=CARTESIAN_POINT('Origin',(69.7479810832458,18.6889152049569,10.));
#34657=CARTESIAN_POINT('',(63.3798972175256,13.7984318791273,9.99769259051996));
#34658=CARTESIAN_POINT('',(63.2983967128177,13.7813169744248,10.0022545211423));
#34659=CARTESIAN_POINT('',(70.5434614183684,15.7201421778575,10.0000000000001));
#34660=CARTESIAN_POINT('Ctrl Pts',(63.2983967128177,13.7813169744248,10.0022545211423));
#34661=CARTESIAN_POINT('Ctrl Pts',(63.282643341652,13.7746926693741,10.3298056773904));
#34662=CARTESIAN_POINT('Ctrl Pts',(63.1648404527592,13.9475832402569,11.6627679218546));
#34663=CARTESIAN_POINT('Ctrl Pts',(62.552433017135,15.7650240000834,13.4838568188229));
#34664=CARTESIAN_POINT('Ctrl Pts',(61.540694761931,18.936865245129,12.7341264791949));
#34665=CARTESIAN_POINT('Ctrl Pts',(61.0732543185778,20.0773594018982,9.55182253210507));
#34666=CARTESIAN_POINT('Ctrl Pts',(61.4316477881723,18.1357994369342,6.76826458716723));
#34667=CARTESIAN_POINT('Ctrl Pts',(62.1626591350493,14.8036106221425,6.86000957288757));
#34668=CARTESIAN_POINT('Ctrl Pts',(62.3828842093693,13.5645914770419,8.8526467410516));
#34669=CARTESIAN_POINT('Ctrl Pts',(62.3378725391134,13.5167884478446,9.92684307365804));
#34670=CARTESIAN_POINT('Ctrl Pts',(62.3341655182897,13.5161734774897,9.99879780140841));
#34671=CARTESIAN_POINT('Ctrl Pts',(63.3798972175256,13.7984318791273,9.99769259051996));
#34672=CARTESIAN_POINT('Ctrl Pts',(63.3356696948373,13.7939231905821,10.8435144444691));
#34673=CARTESIAN_POINT('Ctrl Pts',(63.0364669859301,14.5389353035617,12.70898732583));
#34674=CARTESIAN_POINT('Ctrl Pts',(62.080489794707,17.5330036055456,13.5128046754735));
#34675=CARTESIAN_POINT('Ctrl Pts',(61.2715545195409,19.9458125081592,11.2162142452876));
#34676=CARTESIAN_POINT('Ctrl Pts',(61.2525379570576,19.4106046411913,7.83042882970038));
#34677=CARTESIAN_POINT('Ctrl Pts',(61.9047530097005,16.3703262829254,6.38762845988019));
#34678=CARTESIAN_POINT('Ctrl Pts',(62.4147543833102,13.9548208376169,7.90192541386342));
#34679=CARTESIAN_POINT('Ctrl Pts',(62.4390002488206,13.5542391767051,9.45861716832917));
#34680=CARTESIAN_POINT('Ctrl Pts',(62.4122187264791,13.5461538679481,10.0005448248896));
#34681=CARTESIAN_POINT('Origin',(69.7479810832458,18.6889152049569,10.));
#34682=CARTESIAN_POINT('',(64.3454334554184,14.0587048879185,10.0025996902775));
#34683=CARTESIAN_POINT('',(64.2646301485468,14.038988005468,9.99747713720023));
#34684=CARTESIAN_POINT('',(70.5434614183684,15.7201421778575,10.0000000000001));
#34685=CARTESIAN_POINT('Ctrl Pts',(64.2646301485468,14.038988005468,9.99747713720024));
#34686=CARTESIAN_POINT('Ctrl Pts',(64.226770392365,14.0349994054245,10.7242163838114));
#34687=CARTESIAN_POINT('Ctrl Pts',(63.980303897263,14.6082026447201,12.4671953710476));
#34688=CARTESIAN_POINT('Ctrl Pts',(63.0972885120504,17.3556995742977,13.5881174655937));
#34689=CARTESIAN_POINT('Ctrl Pts',(62.2237737811953,20.0116836036718,11.6313322004901));
#34690=CARTESIAN_POINT('Ctrl Pts',(62.0929146809836,19.8960390869576,8.22313767486128));
#34691=CARTESIAN_POINT('Ctrl Pts',(62.686787843468,17.0756569439774,6.3958317144828));
#34692=CARTESIAN_POINT('Ctrl Pts',(63.271636045696,14.3543730978417,7.6257956239861));
#34693=CARTESIAN_POINT('Ctrl Pts',(63.3311289785642,13.7950809180928,9.32167057633655));
#34694=CARTESIAN_POINT('Ctrl Pts',(63.2983967128177,13.7813169744248,10.0022545211423));
#34695=CARTESIAN_POINT('Ctrl Pts',(64.3454334554184,14.0587048879185,10.0025996902775));
#34696=CARTESIAN_POINT('Ctrl Pts',(64.3351645983746,14.0539764689082,10.2176211405936));
#34697=CARTESIAN_POINT('Ctrl Pts',(64.2433978747176,14.1513426806932,11.4397371699227));
#34698=CARTESIAN_POINT('Ctrl Pts',(63.708961052588,15.6987166428558,13.3670096553836));
#34699=CARTESIAN_POINT('Ctrl Pts',(62.6772983776882,18.9427555175133,12.9642257537709));
#34700=CARTESIAN_POINT('Ctrl Pts',(62.1266472347557,20.3916349158421,9.9067950074971));
#34701=CARTESIAN_POINT('Ctrl Pts',(62.4144320750886,18.7114286257305,6.93283507366395));
#34702=CARTESIAN_POINT('Ctrl Pts',(63.1472062543101,15.3704995140598,6.70571036393744));
#34703=CARTESIAN_POINT('Ctrl Pts',(63.425086417853,13.8968260312721,8.66708054183157));
#34704=CARTESIAN_POINT('Ctrl Pts',(63.3883718001703,13.7992958039273,9.83562185337871));
#34705=CARTESIAN_POINT('Ctrl Pts',(63.3798972175256,13.7984318791273,9.99769259051996));
#34706=CARTESIAN_POINT('Origin',(69.7479810832458,18.6889152049569,10.));
#34707=CARTESIAN_POINT('',(65.3101240288667,14.3221339593831,9.99868436122737));
#34708=CARTESIAN_POINT('',(65.2317006057018,14.2935352300231,10.0018375364667));
#34709=CARTESIAN_POINT('',(70.5434614183684,15.7201421778575,10.0000000000001));
#34710=CARTESIAN_POINT('Ctrl Pts',(65.2317006057018,14.2935352300231,10.0018375364667));
#34711=CARTESIAN_POINT('Ctrl Pts',(65.2259676792212,14.2911203313162,10.1205006547493));
#34712=CARTESIAN_POINT('Ctrl Pts',(65.1542869058501,14.333487038742,11.241710128915));
#34713=CARTESIAN_POINT('Ctrl Pts',(64.6921496134354,15.6317182042723,13.2184200895793));
#34714=CARTESIAN_POINT('Ctrl Pts',(63.6589647612363,18.8835992389528,13.1544941616769));
#34715=CARTESIAN_POINT('Ctrl Pts',(63.0319829890499,20.6195097408352,10.2839896215965));
#34716=CARTESIAN_POINT('Ctrl Pts',(63.2346852212378,19.2589973841656,7.16081725087092));
#34717=CARTESIAN_POINT('Ctrl Pts',(63.9523759072002,15.9765219526977,6.56368841308618));
#34718=CARTESIAN_POINT('Ctrl Pts',(64.30157672835,14.2145525524613,8.43212980411671));
#34719=CARTESIAN_POINT('Ctrl Pts',(64.2792379389272,14.0405269650183,9.71707241074883));
#34720=CARTESIAN_POINT('Ctrl Pts',(64.2646301485468,14.038988005468,9.99747713720024));
#34721=CARTESIAN_POINT('Ctrl Pts',(65.3101240288667,14.3221339593831,9.99868436122737));
#34722=CARTESIAN_POINT('Ctrl Pts',(65.2798663326535,14.3164610907008,10.5933471090872));
#34723=CARTESIAN_POINT('Ctrl Pts',(65.0828577529568,14.7310514432719,12.2044751575878));
#34724=CARTESIAN_POINT('Ctrl Pts',(64.2812461473764,17.199991458738,13.6183729089162));
#34725=CARTESIAN_POINT('Ctrl Pts',(63.346239485481,20.0833051820057,12.017555775347));
#34726=CARTESIAN_POINT('Ctrl Pts',(63.1074718691846,20.3682194128848,8.60989310618131));
#34727=CARTESIAN_POINT('Ctrl Pts',(63.6430568297551,17.7632104839249,6.4471568308768));
#34728=CARTESIAN_POINT('Ctrl Pts',(64.2882973111131,14.7920138952888,7.39383484183733));
#34729=CARTESIAN_POINT('Ctrl Pts',(64.3833599300929,14.0761685903618,9.20845039448992));
#34730=CARTESIAN_POINT('Ctrl Pts',(64.3454334554184,14.0587048879185,10.0025996902775));
#34731=CARTESIAN_POINT('Origin',(69.7479810832458,18.6889152049569,10.));
#34732=CARTESIAN_POINT('',(66.2783193540156,14.5724831194333,9.99930975590662));
#34733=CARTESIAN_POINT('',(66.1956016367402,14.559910913876,9.99976839157063));
#34734=CARTESIAN_POINT('',(70.5434614183684,15.7201421778575,10.0000000000001));
#34735=CARTESIAN_POINT('Ctrl Pts',(66.1956016367402,14.559910913876,9.99976839157063));
#34736=CARTESIAN_POINT('Ctrl Pts',(66.1695891483769,14.5533139234257,10.5198381182744));
#34737=CARTESIAN_POINT('Ctrl Pts',(65.9976317638641,14.890051591398,12.0503568643789));
#34738=CARTESIAN_POINT('Ctrl Pts',(65.2498597727098,17.1744195179844,13.6018503664189));
#34739=CARTESIAN_POINT('Ctrl Pts',(64.2890822261735,20.1560728090925,12.2479900298274));
#34740=CARTESIAN_POINT('Ctrl Pts',(63.9799857765362,20.7056191362412,8.89407499549297));
#34741=CARTESIAN_POINT('Ctrl Pts',(64.4632262402319,18.2981238461185,6.52411027736645));
#34742=CARTESIAN_POINT('Ctrl Pts',(65.146471993839,15.1680091238728,7.21818882738257));
#34743=CARTESIAN_POINT('Ctrl Pts',(65.2744447664955,14.3115404877175,9.11709648401003));
#34744=CARTESIAN_POINT('Ctrl Pts',(65.2317006057018,14.2935352300231,10.0018375364667));
#34745=CARTESIAN_POINT('Ctrl Pts',(66.2783193540156,14.5724831194333,9.99930975590662));
#34746=CARTESIAN_POINT('Ctrl Pts',(66.2290088142628,14.5623726178326,10.9656350129457));
#34747=CARTESIAN_POINT('Ctrl Pts',(65.869509017197,15.5078446363722,12.9430947115651));
#34748=CARTESIAN_POINT('Ctrl Pts',(64.852721554462,18.704288070265,13.3837942299379));
#34749=CARTESIAN_POINT('Ctrl Pts',(64.1195886430847,20.8341986998846,10.7999310727631));
#34750=CARTESIAN_POINT('Ctrl Pts',(64.2044184759422,19.9114308093214,7.49968047567758));
#34751=CARTESIAN_POINT('Ctrl Pts',(64.8955230826759,16.7260146593053,6.43862003923501));
#34752=CARTESIAN_POINT('Ctrl Pts',(65.3320744591731,14.6092002260328,8.15058790184904));
#34753=CARTESIAN_POINT('Ctrl Pts',(65.3314182383775,14.3261263074255,9.58018345977288));
#34754=CARTESIAN_POINT('Ctrl Pts',(65.3101240288667,14.3221339593831,9.99868436122737));
#34755=CARTESIAN_POINT('Origin',(69.7479810832458,18.6889152049569,10.));
#34756=CARTESIAN_POINT('',(67.242349320473,14.8383776097513,10.0022118830713));
#34757=CARTESIAN_POINT('',(67.1637176864735,14.810555933805,9.99855140140545));
#34758=CARTESIAN_POINT('',(70.5434614183684,15.7201421778575,10.0000000000001));
#34759=CARTESIAN_POINT('Ctrl Pts',(67.1637176864735,14.810555933805,9.99855140140544));
#34760=CARTESIAN_POINT('Ctrl Pts',(67.1164300139581,14.8034925645055,10.9127656351722));
#34761=CARTESIAN_POINT('Ctrl Pts',(66.7843853462346,15.6578176600211,12.8392373747717));
#34762=CARTESIAN_POINT('Ctrl Pts',(65.795981118425,18.7603708726991,13.4453363911884));
#34763=CARTESIAN_POINT('Ctrl Pts',(65.0290015152611,21.0187603927389,11.00449717215));
#34764=CARTESIAN_POINT('Ctrl Pts',(65.0614895355965,20.2934961228732,7.66994591646111));
#34765=CARTESIAN_POINT('Ctrl Pts',(65.7301904655353,17.1938529499358,6.40846378494576));
#34766=CARTESIAN_POINT('Ctrl Pts',(66.2070041644091,14.9140195913108,8.0104478238207));
#34767=CARTESIAN_POINT('Ctrl Pts',(66.2201050327307,14.5661251855401,9.50987006742361));
#34768=CARTESIAN_POINT('Ctrl Pts',(66.1956016367402,14.559910913876,9.99976839157063));
#34769=CARTESIAN_POINT('Ctrl Pts',(67.242349320473,14.8383776097513,10.0022118830713));
#34770=CARTESIAN_POINT('Ctrl Pts',(67.2260470012181,14.8315944872623,10.3408933046043));
#34771=CARTESIAN_POINT('Ctrl Pts',(67.1051700296205,15.0130297323863,11.6887868410754));
#34772=CARTESIAN_POINT('Ctrl Pts',(66.4816292855382,16.868372167434,13.5013274912989));
#34773=CARTESIAN_POINT('Ctrl Pts',(65.468753391891,20.0422978199459,12.6947822329673));
#34774=CARTESIAN_POINT('Ctrl Pts',(65.0155990043222,21.1273143736846,9.47487431060687));
#34775=CARTESIAN_POINT('Ctrl Pts',(65.3922823621304,19.1153342996381,6.72525821930946));
#34776=CARTESIAN_POINT('Ctrl Pts',(66.1257396929251,15.7718556315866,6.9083705731136));
#34777=CARTESIAN_POINT('Ctrl Pts',(66.3280678631807,14.604717917356,8.91484226317838));
#34778=CARTESIAN_POINT('Ctrl Pts',(66.2803308931335,14.572895560051,9.95989017005526));
#34779=CARTESIAN_POINT('Ctrl Pts',(66.2783193540156,14.5724831194333,9.99930975590662));
#34780=CARTESIAN_POINT('Origin',(69.7479810832458,18.6889152049569,10.));
#34781=CARTESIAN_POINT('',(68.2083503098983,15.0969161422106,9.99673640007591));
#34782=CARTESIAN_POINT('',(68.1281291851066,15.0750265266586,10.0024371765582));
#34783=CARTESIAN_POINT('',(70.5434614183684,15.7201421778575,10.0000000000001));
#34784=CARTESIAN_POINT('',(67.8425423025985,17.2449834421531,7.06170475438605));
#34785=CARTESIAN_POINT('Ctrl Pts',(67.8425423025985,17.244983442153,7.06170475438608));
#34786=CARTESIAN_POINT('Ctrl Pts',(68.0419164156808,16.2988495743024,7.35795147289591));
#34787=CARTESIAN_POINT('Ctrl Pts',(68.2441585752431,15.2831204824219,8.39983158504209));
#34788=CARTESIAN_POINT('Ctrl Pts',(68.2236687995603,15.0986382893443,9.7020767480265));
#34789=CARTESIAN_POINT('Ctrl Pts',(68.2083503098983,15.0969161422106,9.99673640007591));
#34790=CARTESIAN_POINT('',(67.6148078402348,18.1173331571764,6.92649999999998));
#34791=CARTESIAN_POINT('Ctrl Pts',(67.6148078402348,18.1173331571765,6.92649999999999));
#34792=CARTESIAN_POINT('Ctrl Pts',(67.6909584745889,17.8331351207384,6.92649999999999));
#34793=CARTESIAN_POINT('Ctrl Pts',(67.7691522152652,17.5337033543061,6.97030621012384));
#34794=CARTESIAN_POINT('Ctrl Pts',(67.8425423025985,17.2449834421531,7.06170475438605));
#34795=CARTESIAN_POINT('',(67.4240381925641,18.8148375643561,7.01163591529246));
#34796=CARTESIAN_POINT('Ctrl Pts',(67.4238662472344,18.8154792730625,7.01293629783556));
#34797=CARTESIAN_POINT('Ctrl Pts',(67.4888593221927,18.5825814377542,6.95435125823854));
#34798=CARTESIAN_POINT('Ctrl Pts',(67.5537087055993,18.3453582319347,6.92649999999999));
#34799=CARTESIAN_POINT('Ctrl Pts',(67.6148078402348,18.1173331571765,6.92649999999999));
#34800=CARTESIAN_POINT('Ctrl Pts',(67.4242662328515,18.8139865064172,7.00991129962864));
#34801=CARTESIAN_POINT('Ctrl Pts',(67.4544236505276,18.6713424458928,6.97326843816114));
#34802=CARTESIAN_POINT('Ctrl Pts',(67.6913073253836,17.5558463812024,6.77617107551512));
#34803=CARTESIAN_POINT('Ctrl Pts',(68.0973070404756,15.6699322564948,7.59313914445674));
#34804=CARTESIAN_POINT('Ctrl Pts',(68.1615830306033,15.0894434810379,9.30549521878025));
#34805=CARTESIAN_POINT('Ctrl Pts',(68.1281291851066,15.0750265266586,10.0024371765582));
#34806=CARTESIAN_POINT('Origin',(-17.0820569767664,63.7511045350785,10.));
#34807=CARTESIAN_POINT('',(-13.7189801527801,60.9122168113323,9.99965378812947));
#34808=CARTESIAN_POINT('',(-13.6458118873637,60.6472937215209,9.99664393250999));
#34809=CARTESIAN_POINT('',(-14.6503387090836,64.4026814811241,10.));
#34810=CARTESIAN_POINT('',(-14.1985145724512,60.3826426720153,11.6359872033746));
#34811=CARTESIAN_POINT('Ctrl Pts',(-13.6458118873637,60.6472937215209,9.99664393250999));
#34812=CARTESIAN_POINT('Ctrl Pts',(-13.6410407802454,60.6097205320263,10.5892058593234));
#34813=CARTESIAN_POINT('Ctrl Pts',(-13.8356159531907,60.5187326677745,11.184803560304));
#34814=CARTESIAN_POINT('Ctrl Pts',(-14.1985145724512,60.3826426720153,11.6359872033745));
#34815=CARTESIAN_POINT('',(-17.8984305821303,59.3912531651588,11.6380816927072));
#34816=CARTESIAN_POINT('Origin',(-16.0467807963563,59.8874012299222,10.));
#34817=CARTESIAN_POINT('Ctrl Pts',(-17.8984546702661,59.3912467107623,11.6380966037226));
#34818=CARTESIAN_POINT('Ctrl Pts',(-17.4212611177615,59.5701794123024,12.2270179049202));
#34819=CARTESIAN_POINT('Ctrl Pts',(-16.6595160069779,59.8253574740883,12.567422198156));
#34820=CARTESIAN_POINT('Ctrl Pts',(-15.9233267283634,60.0736878712827,12.5157167035403));
#34821=CARTESIAN_POINT('Ctrl Pts',(-15.1456267338051,60.3360206084697,12.4610957466079));
#34822=CARTESIAN_POINT('Ctrl Pts',(-14.3964458015818,60.5907116859352,11.9688993897472));
#34823=CARTESIAN_POINT('Ctrl Pts',(-14.014605944713,60.7469740189126,11.2575578209417));
#34824=CARTESIAN_POINT('Ctrl Pts',(-13.8116368860468,60.8300361143406,10.8794403300265));
#34825=CARTESIAN_POINT('Ctrl Pts',(-13.7124604894775,60.8852870497794,10.4394030962358));
#34826=CARTESIAN_POINT('Ctrl Pts',(-13.7189801527801,60.9122168113323,9.99965378812947));
#34827=CARTESIAN_POINT('Origin',(-17.0820569767664,63.7511045350785,10.));
#34828=CARTESIAN_POINT('',(-13.9708704146993,61.8799991994798,9.9990152806394));
#34829=CARTESIAN_POINT('',(-13.899975087973,61.614467077582,10.0012573013837));
#34830=CARTESIAN_POINT('',(-14.6503387090836,64.4026814811241,10.));
#34831=CARTESIAN_POINT('Ctrl Pts',(-13.899975087973,61.614467077582,10.0012573013837));
#34832=CARTESIAN_POINT('Ctrl Pts',(-13.8982899610888,61.6099667912195,10.0766544396886));
#34833=CARTESIAN_POINT('Ctrl Pts',(-13.900043500223,61.6045451170745,10.1520128061813));
#34834=CARTESIAN_POINT('Ctrl Pts',(-13.9053569552699,61.5981695663354,10.2270376921982));
#34835=CARTESIAN_POINT('Ctrl Pts',(-13.963452717137,61.5284611611194,11.0473378309357));
#34836=CARTESIAN_POINT('Ctrl Pts',(-14.4471220222723,61.3447206686646,11.8277717281243));
#34837=CARTESIAN_POINT('Ctrl Pts',(-15.1337367424346,61.1066011161458,12.2189611289227));
#34838=CARTESIAN_POINT('Ctrl Pts',(-15.8203514625968,60.8684815636269,12.6101505297211));
#34839=CARTESIAN_POINT('Ctrl Pts',(-16.709911597786,60.575982951044,12.6120954341294));
#34840=CARTESIAN_POINT('Ctrl Pts',(-17.3980067606842,60.3374667150896,12.223752356313));
#34841=CARTESIAN_POINT('Ctrl Pts',(-18.0861019235824,60.0989504791352,11.8354092784967));
#34842=CARTESIAN_POINT('Ctrl Pts',(-18.5727321141895,59.9144166198093,11.0567782184557));
#34843=CARTESIAN_POINT('Ctrl Pts',(-18.6339764021912,59.8438645695582,10.2368654679641));
#34844=CARTESIAN_POINT('Ctrl Pts',(-18.695220690193,59.773312519307,9.41695271747245));
#34845=CARTESIAN_POINT('Ctrl Pts',(-18.3310790755893,59.8167422781306,8.55575827653014));
#34846=CARTESIAN_POINT('Ctrl Pts',(-17.6984585141969,59.932110753931,8.03819621078695));
#34847=CARTESIAN_POINT('Ctrl Pts',(-17.0658379528045,60.0474792297313,7.52063414504374));
#34848=CARTESIAN_POINT('Ctrl Pts',(-16.1647384446234,60.2347864225084,7.34670445449967));
#34849=CARTESIAN_POINT('Ctrl Pts',(-15.3927695971153,60.3874931590402,7.59575134544305));
#34850=CARTESIAN_POINT('Ctrl Pts',(-14.6208007496071,60.5401998955719,7.84479823638644));
#34851=CARTESIAN_POINT('Ctrl Pts',(-13.9779625627719,60.6583061758582,8.51682170881728));
#34852=CARTESIAN_POINT('Ctrl Pts',(-13.7459615817214,60.6663289586339,9.30743209219145));
#34853=CARTESIAN_POINT('Ctrl Pts',(-13.6804424696227,60.6685946628634,9.53070739947741));
#34854=CARTESIAN_POINT('Ctrl Pts',(-13.6476895615158,60.6620806891943,9.76344057197133));
#34855=CARTESIAN_POINT('Ctrl Pts',(-13.6458118873637,60.6472937215209,9.99664393250999));
#34856=CARTESIAN_POINT('Ctrl Pts',(-13.7189801527801,60.9122168113323,9.99965378812947));
#34857=CARTESIAN_POINT('Ctrl Pts',(-13.7247257446778,60.9359492362449,9.61211536100735));
#34858=CARTESIAN_POINT('Ctrl Pts',(-13.8125590225005,60.9376863320054,9.2248005482108));
#34859=CARTESIAN_POINT('Ctrl Pts',(-13.9837827281427,60.9170790299751,8.8802861232622));
#34860=CARTESIAN_POINT('Ctrl Pts',(-14.3492981499552,60.8730881195708,8.14484277513853));
#34861=CARTESIAN_POINT('Ctrl Pts',(-15.0948277750946,60.7272727102727,7.60444285964153));
#34862=CARTESIAN_POINT('Ctrl Pts',(-15.8946095193188,60.5669204894781,7.49935843056473));
#34863=CARTESIAN_POINT('Ctrl Pts',(-16.6943912635431,60.4065682686835,7.39427400148794));
#34864=CARTESIAN_POINT('Ctrl Pts',(-17.5484251268522,60.2316792363924,7.72450505883135));
#34865=CARTESIAN_POINT('Ctrl Pts',(-18.0828447847106,60.1424305723414,8.34320956294503));
#34866=CARTESIAN_POINT('Ctrl Pts',(-18.617264442569,60.0531819082903,8.96191406705872));
#34867=CARTESIAN_POINT('Ctrl Pts',(-18.8320698949766,60.0495736124794,9.86909201794267));
#34868=CARTESIAN_POINT('Ctrl Pts',(-18.6376771842086,60.1556096340356,10.6611508664114));
#34869=CARTESIAN_POINT('Ctrl Pts',(-18.4432844734405,60.2616456555919,11.4532097148801));
#34870=CARTESIAN_POINT('Ctrl Pts',(-17.8396935994968,60.4773259945153,12.1301494609335));
#34871=CARTESIAN_POINT('Ctrl Pts',(-17.1014273477892,60.7290924921509,12.3908459426517));
#34872=CARTESIAN_POINT('Ctrl Pts',(-16.3631610960817,60.9808589897866,12.6515424243699));
#34873=CARTESIAN_POINT('Ctrl Pts',(-15.4902194666104,61.2687116461344,12.4959956417528));
#34874=CARTESIAN_POINT('Ctrl Pts',(-14.8769273589395,61.4869914228006,11.9933937214366));
#34875=CARTESIAN_POINT('Ctrl Pts',(-14.3076501674883,61.6896056365773,11.5268626736099));
#34876=CARTESIAN_POINT('Ctrl Pts',(-13.9620906745726,61.8322748736987,10.7613040129743));
#34877=CARTESIAN_POINT('Ctrl Pts',(-13.9708704146993,61.8799991994798,9.9990152806394));
#34878=CARTESIAN_POINT('Origin',(-17.0820569767664,63.7511045350785,10.));
#34879=CARTESIAN_POINT('',(-14.2348698103755,62.8445369550162,10.0018466754434));
#34880=CARTESIAN_POINT('',(-14.1654859215485,62.5785998445538,10.0004462653844));
#34881=CARTESIAN_POINT('',(-14.6503387090836,64.4026814811241,10.));
#34882=CARTESIAN_POINT('Ctrl Pts',(-14.1654859215485,62.5785998445538,10.0004462653844));
#34883=CARTESIAN_POINT('Ctrl Pts',(-14.1585827534688,62.5552558244194,10.3867702486339));
#34884=CARTESIAN_POINT('Ctrl Pts',(-14.2332491130212,62.5100553152291,10.772836742403));
#34885=CARTESIAN_POINT('Ctrl Pts',(-14.3908772813225,62.4426252563818,11.1164878478949));
#34886=CARTESIAN_POINT('Ctrl Pts',(-14.7296226663466,62.2977170112848,11.8549994178653));
#34887=CARTESIAN_POINT('Ctrl Pts',(-15.4515079046903,62.0501467519026,12.3976253642208));
#34888=CARTESIAN_POINT('Ctrl Pts',(-16.2272258855738,61.7881520526305,12.5013894187969));
#34889=CARTESIAN_POINT('Ctrl Pts',(-17.0029438664574,61.5261573533584,12.6051534733731));
#34890=CARTESIAN_POINT('Ctrl Pts',(-17.8324945898807,61.2497382141964,12.2700556361698));
#34891=CARTESIAN_POINT('Ctrl Pts',(-18.3383599455199,61.0600503079339,11.6461438143242));
#34892=CARTESIAN_POINT('Ctrl Pts',(-18.8442253011591,60.8703624016714,11.0222319924786));
#34893=CARTESIAN_POINT('Ctrl Pts',(-19.0264052890141,60.7674057283085,10.1095061859907));
#34894=CARTESIAN_POINT('Ctrl Pts',(-18.7972629292322,60.7746625458238,9.31667252204711));
#34895=CARTESIAN_POINT('Ctrl Pts',(-18.5681205694503,60.781919363339,8.52383885810353));
#34896=CARTESIAN_POINT('Ctrl Pts',(-17.9276558620316,60.8993896717325,7.85089733670426));
#34897=CARTESIAN_POINT('Ctrl Pts',(-17.1565944419209,61.0518532638259,7.59916807226848));
#34898=CARTESIAN_POINT('Ctrl Pts',(-16.3855330218102,61.2043168559192,7.34743880783269));
#34899=CARTESIAN_POINT('Ctrl Pts',(-15.4838748890076,61.3917737317126,7.5169218003604));
#34900=CARTESIAN_POINT('Ctrl Pts',(-14.8493069319057,61.5076640106206,8.03174648676741));
#34901=CARTESIAN_POINT('Ctrl Pts',(-14.2727767422055,61.6129549313731,8.49948515966252));
#34902=CARTESIAN_POINT('Ctrl Pts',(-13.9167146450877,61.6591716047613,9.2522842034192));
#34903=CARTESIAN_POINT('Ctrl Pts',(-13.899975087973,61.614467077582,10.0012573013837));
#34904=CARTESIAN_POINT('Ctrl Pts',(-13.9708704146993,61.8799991994798,9.9990152806394));
#34905=CARTESIAN_POINT('Ctrl Pts',(-13.971549239588,61.8836891105327,9.94007725327275));
#34906=CARTESIAN_POINT('Ctrl Pts',(-13.9743462862715,61.8868114457663,9.88115877337007));
#34907=CARTESIAN_POINT('Ctrl Pts',(-13.9793219277933,61.8893500282724,9.82239956232277));
#34908=CARTESIAN_POINT('Ctrl Pts',(-14.0486511901886,61.9247219600931,9.00366438154032));
#34909=CARTESIAN_POINT('Ctrl Pts',(-14.5409523008496,61.84675892675,8.21585107799066));
#34910=CARTESIAN_POINT('Ctrl Pts',(-15.243221392539,61.712535142454,7.80941972573588));
#34911=CARTESIAN_POINT('Ctrl Pts',(-15.9454904842284,61.5783113581579,7.4029883734811));
#34912=CARTESIAN_POINT('Ctrl Pts',(-16.8577275569461,61.3878268229089,7.37793897252118));
#34913=CARTESIAN_POINT('Ctrl Pts',(-17.5801209048419,61.2482107604141,7.74541574302333));
#34914=CARTESIAN_POINT('Ctrl Pts',(-18.3025142527376,61.1085946979192,8.11289251352548));
#34915=CARTESIAN_POINT('Ctrl Pts',(-18.8350638758114,61.0198471081786,8.8728954554897));
#34916=CARTESIAN_POINT('Ctrl Pts',(-18.9468623871525,61.0438394390412,9.68733378926659));
#34917=CARTESIAN_POINT('Ctrl Pts',(-19.0586608984936,61.0678317699038,10.5017721230435));
#34918=CARTESIAN_POINT('Ctrl Pts',(-18.749708298102,61.2045640213696,11.3706458486331));
#34919=CARTESIAN_POINT('Ctrl Pts',(-18.1634433884681,61.4156018821482,11.9074332417686));
#34920=CARTESIAN_POINT('Ctrl Pts',(-17.5771784788342,61.6266397429268,12.4442206349041));
#34921=CARTESIAN_POINT('Ctrl Pts',(-16.7136012599581,61.911983213018,12.6489216955856));
#34922=CARTESIAN_POINT('Ctrl Pts',(-15.9628772265393,62.1670877632026,12.4304742338454));
#34923=CARTESIAN_POINT('Ctrl Pts',(-15.2121531931204,62.4221923133873,12.2120267721052));
#34924=CARTESIAN_POINT('Ctrl Pts',(-14.5742823451588,62.6470579436654,11.5704307879433));
#34925=CARTESIAN_POINT('Ctrl Pts',(-14.3390239366156,62.7640438959386,10.7911028658272));
#34926=CARTESIAN_POINT('Ctrl Pts',(-14.2625865983512,62.8020535673525,10.5378929917549));
#34927=CARTESIAN_POINT('Ctrl Pts',(-14.2286511253629,62.8286748982889,10.2701434172214));
#34928=CARTESIAN_POINT('Ctrl Pts',(-14.2348698103755,62.8445369550162,10.0018466754434));
#34929=CARTESIAN_POINT('Origin',(-17.0820569767664,63.7511045350785,10.));
#34930=CARTESIAN_POINT('',(-14.4927485186002,63.8107147438123,9.9979335262408));
#34931=CARTESIAN_POINT('',(-14.4189472139579,63.5459612763502,9.99811000378505));
#34932=CARTESIAN_POINT('',(-14.6503387090836,64.4026814811241,10.));
#34933=CARTESIAN_POINT('Ctrl Pts',(-14.4189472139579,63.5459612763502,9.99811000378505));
#34934=CARTESIAN_POINT('Ctrl Pts',(-14.4131993125783,63.5020657997402,10.6909216248415));
#34935=CARTESIAN_POINT('Ctrl Pts',(-14.6895870615305,63.3825723034678,11.3881278716994));
#34936=CARTESIAN_POINT('Ctrl Pts',(-15.1696780211854,63.208496696392,11.8560065223218));
#34937=CARTESIAN_POINT('Ctrl Pts',(-15.7417608055524,63.001065883577,12.4135369565261));
#34938=CARTESIAN_POINT('Ctrl Pts',(-16.6030903983921,62.7161316220186,12.6454354329572));
#34939=CARTESIAN_POINT('Ctrl Pts',(-17.3619190322642,62.4586624096389,12.4478622804134));
#34940=CARTESIAN_POINT('Ctrl Pts',(-18.1207476661363,62.2011931972591,12.2502891278697));
#34941=CARTESIAN_POINT('Ctrl Pts',(-18.7770753410409,61.9711890340582,11.6232443463511));
#34942=CARTESIAN_POINT('Ctrl Pts',(-19.0309502087538,61.8490217755359,10.847506523471));
#34943=CARTESIAN_POINT('Ctrl Pts',(-19.2848250764668,61.7268545170135,10.0717687005908));
#34944=CARTESIAN_POINT('Ctrl Pts',(-19.1362471369881,61.7125241631699,9.14733783634905));
#34945=CARTESIAN_POINT('Ctrl Pts',(-18.6456858472658,61.7898279718489,8.48815640829392));
#34946=CARTESIAN_POINT('Ctrl Pts',(-18.1551245575434,61.8671317805279,7.8289749802388));
#34947=CARTESIAN_POINT('Ctrl Pts',(-17.3225799175774,62.0360697517296,7.4350429883703));
#34948=CARTESIAN_POINT('Ctrl Pts',(-16.5147885234742,62.1983751106923,7.48275547481138));
#34949=CARTESIAN_POINT('Ctrl Pts',(-15.7069971293709,62.360680469655,7.53046796125247));
#34950=CARTESIAN_POINT('Ctrl Pts',(-14.9239589811304,62.5163532163788,8.01982492600314));
#34951=CARTESIAN_POINT('Ctrl Pts',(-14.5102426728623,62.5730664743347,8.73170200517114));
#34952=CARTESIAN_POINT('Ctrl Pts',(-14.2890407035395,62.6033893890854,9.11232178901981));
#34953=CARTESIAN_POINT('Ctrl Pts',(-14.1734177690261,62.6054224867212,9.5565540007379));
#34954=CARTESIAN_POINT('Ctrl Pts',(-14.1654859215485,62.5785998445538,10.0004462653844));
#34955=CARTESIAN_POINT('Ctrl Pts',(-14.2348698103755,62.8445369550162,10.0018466754434));
#34956=CARTESIAN_POINT('Ctrl Pts',(-14.2477909590166,62.8774950470096,9.44438121878215));
#34957=CARTESIAN_POINT('Ctrl Pts',(-14.4340668190784,62.8640028840736,8.88455351560663));
#34958=CARTESIAN_POINT('Ctrl Pts',(-14.7726377170273,62.8097033887246,8.44788099502235));
#34959=CARTESIAN_POINT('Ctrl Pts',(-15.2741558751071,62.7292706549691,7.80104690640396));
#34960=CARTESIAN_POINT('Ctrl Pts',(-16.1098381603915,62.5592989131896,7.42443858923752));
#34961=CARTESIAN_POINT('Ctrl Pts',(-16.913927805431,62.3977923938505,7.48559176785147));
#34962=CARTESIAN_POINT('Ctrl Pts',(-17.7180174504704,62.2362858745114,7.54674494646541));
#34963=CARTESIAN_POINT('Ctrl Pts',(-18.490514455265,62.0832445776126,8.04565962085972));
#34964=CARTESIAN_POINT('Ctrl Pts',(-18.8937702597925,62.0291411621378,8.76039160250515));
#34965=CARTESIAN_POINT('Ctrl Pts',(-19.2970260643199,61.9750377466629,9.47512358415058));
#34966=CARTESIAN_POINT('Ctrl Pts',(-19.3310406685804,62.0198722126119,10.4056728730471));
#34967=CARTESIAN_POINT('Ctrl Pts',(-18.9866823611344,62.1660913946905,11.138080910744));
#34968=CARTESIAN_POINT('Ctrl Pts',(-18.6423240536885,62.312310576769,11.8704889484409));
#34969=CARTESIAN_POINT('Ctrl Pts',(-17.9195928345362,62.5599144749771,12.4047557349382));
#34970=CARTESIAN_POINT('Ctrl Pts',(-17.1459983851495,62.8211471346509,12.5032105584454));
#34971=CARTESIAN_POINT('Ctrl Pts',(-16.3724039357629,63.0823797943247,12.6016653819527));
#34972=CARTESIAN_POINT('Ctrl Pts',(-15.5479462561419,63.3572412154642,12.2643082424698));
#34973=CARTESIAN_POINT('Ctrl Pts',(-15.0453884512907,63.5458498251155,11.6412138093996));
#34974=CARTESIAN_POINT('Ctrl Pts',(-14.6827506455303,63.6819468306564,11.1915986689941));
#34975=CARTESIAN_POINT('Ctrl Pts',(-14.4877209077723,63.7731333897311,10.5932047327948));
#34976=CARTESIAN_POINT('Ctrl Pts',(-14.4927485186002,63.8107147438123,9.9979335262408));
#34977=CARTESIAN_POINT('Origin',(-17.0820569767664,63.7511045350785,10.));
#34978=CARTESIAN_POINT('',(-14.7480685208434,64.7775781358098,10.0015051238181));
#34979=CARTESIAN_POINT('',(-14.6789571988966,64.5115679912719,10.0021294030496));
#34980=CARTESIAN_POINT('',(-14.6503387090836,64.4026814811241,10.));
#34981=CARTESIAN_POINT('Ctrl Pts',(-14.6789571988966,64.5115679912719,10.0021294030496));
#34982=CARTESIAN_POINT('Ctrl Pts',(-14.6745624451438,64.5012097288919,10.1782532036582));
#34983=CARTESIAN_POINT('Ctrl Pts',(-14.6880487522533,64.4860602506939,10.3540783073467));
#34984=CARTESIAN_POINT('Ctrl Pts',(-14.7205078014428,64.4658270415774,10.5257161206902));
#34985=CARTESIAN_POINT('Ctrl Pts',(-14.8728494531256,64.3708655262953,11.33127231007));
#34986=CARTESIAN_POINT('Ctrl Pts',(-15.4431136830598,64.163921993672,12.0445928505658));
#34987=CARTESIAN_POINT('Ctrl Pts',(-16.1698862069569,63.9150421900726,12.3462664892694));
#34988=CARTESIAN_POINT('Ctrl Pts',(-16.896658730854,63.6661623864732,12.6479401279729));
#34989=CARTESIAN_POINT('Ctrl Pts',(-17.7799395487139,63.3753463118977,12.5379668648843));
#34990=CARTESIAN_POINT('Ctrl Pts',(-18.418151553513,63.1501962278719,12.0655906176064));
#34991=CARTESIAN_POINT('Ctrl Pts',(-19.056363558312,62.9250461438461,11.5932143703284));
#34992=CARTESIAN_POINT('Ctrl Pts',(-19.4495067500501,62.76556205037,10.7584351388612));
#34993=CARTESIAN_POINT('Ctrl Pts',(-19.4154782471595,62.7205382674991,9.93505104704572));
#34994=CARTESIAN_POINT('Ctrl Pts',(-19.3814497442688,62.6755144846282,9.11166695523024));
#34995=CARTESIAN_POINT('Ctrl Pts',(-18.9202495467495,62.7449510123625,8.29967800306651));
#34996=CARTESIAN_POINT('Ctrl Pts',(-18.2323333520892,62.875135908442,7.8626772661128));
#34997=CARTESIAN_POINT('Ctrl Pts',(-17.5444171574288,63.0053208045214,7.42567652915909));
#34998=CARTESIAN_POINT('Ctrl Pts',(-16.6297849656276,63.196254068946,7.36366400741539));
#34999=CARTESIAN_POINT('Ctrl Pts',(-15.8919306215942,63.3398198518215,7.70440771629202));
#35000=CARTESIAN_POINT('Ctrl Pts',(-15.1540762775607,63.483385634697,8.04515142516864));
#35001=CARTESIAN_POINT('Ctrl Pts',(-14.5929997812951,63.5795839360234,8.78865136466559));
#35002=CARTESIAN_POINT('Ctrl Pts',(-14.4538795211095,63.5627194046509,9.60198253040281));
#35003=CARTESIAN_POINT('Ctrl Pts',(-14.4315087612499,63.5600075610921,9.73276747984711));
#35004=CARTESIAN_POINT('Ctrl Pts',(-14.4200485884486,63.5543722345421,9.86535806600947));
#35005=CARTESIAN_POINT('Ctrl Pts',(-14.4189472139579,63.5459612763502,9.99811000378505));
#35006=CARTESIAN_POINT('Ctrl Pts',(-14.4927485186002,63.8107147438123,9.9979335262408));
#35007=CARTESIAN_POINT('Ctrl Pts',(-14.494688369579,63.8252151156581,9.76825436605168));
#35008=CARTESIAN_POINT('Ctrl Pts',(-14.5264111861321,63.8317351659301,9.53904009330699));
#35009=CARTESIAN_POINT('Ctrl Pts',(-14.5897808794637,63.8297754611264,9.3190160464461));
#35010=CARTESIAN_POINT('Ctrl Pts',(-14.8173890425695,63.8227366893229,8.52874444322036));
#35011=CARTESIAN_POINT('Ctrl Pts',(-15.4532632988625,63.7063033475529,7.85703296342643));
#35012=CARTESIAN_POINT('Ctrl Pts',(-16.2205322683666,63.5546628984882,7.60269513736945));
#35013=CARTESIAN_POINT('Ctrl Pts',(-16.9878012378706,63.4030224494236,7.34835731131247));
#35014=CARTESIAN_POINT('Ctrl Pts',(-17.8864649205859,63.2161748930643,7.51139313899242));
#35015=CARTESIAN_POINT('Ctrl Pts',(-18.522749012129,63.09963173627,8.01927548227232));
#35016=CARTESIAN_POINT('Ctrl Pts',(-19.1590331036721,62.9830885794757,8.52715782555222));
#35017=CARTESIAN_POINT('Ctrl Pts',(-19.5329376040432,62.9368498222464,9.37988668443207));
#35018=CARTESIAN_POINT('Ctrl Pts',(-19.4841294236266,63.0038765864645,10.1981222260488));
#35019=CARTESIAN_POINT('Ctrl Pts',(-19.43532124321,63.0709033506826,11.0163577676655));
#35020=CARTESIAN_POINT('Ctrl Pts',(-18.9638003820057,63.2511956363482,11.8000999920191));
#35021=CARTESIAN_POINT('Ctrl Pts',(-18.2853245933941,63.4869413276821,12.2006980454407));
#35022=CARTESIAN_POINT('Ctrl Pts',(-17.6068488047825,63.7226870190161,12.6012960988622));
#35023=CARTESIAN_POINT('Ctrl Pts',(-16.7214180887636,64.0138861160186,12.6187499813517));
#35024=CARTESIAN_POINT('Ctrl Pts',(-16.02891964808,64.253389165651,12.2452952639449));
#35025=CARTESIAN_POINT('Ctrl Pts',(-15.3364212073964,64.4928922152834,11.871840546538));
#35026=CARTESIAN_POINT('Ctrl Pts',(-14.8368550420482,64.6806992175459,11.1074772292348));
#35027=CARTESIAN_POINT('Ctrl Pts',(-14.7584549707696,64.755655105023,10.2922353809894));
#35028=CARTESIAN_POINT('Ctrl Pts',(-14.7491833360657,64.7645194286933,10.195824440425));
#35029=CARTESIAN_POINT('Ctrl Pts',(-14.7458019429916,64.7718054668758,10.0987019353608));
#35030=CARTESIAN_POINT('Ctrl Pts',(-14.7480685208434,64.7775781358098,10.0015051238181));
#35031=CARTESIAN_POINT('Origin',(-17.0820569767664,63.7511045350785,10.));
#35032=CARTESIAN_POINT('',(-15.0130771992805,65.7418454548454,9.99981028982561));
#35033=CARTESIAN_POINT('',(-14.9415523108175,65.4764820235065,9.9989223619292));
#35034=CARTESIAN_POINT('',(-14.6503387090836,64.4026814811241,10.));
#35035=CARTESIAN_POINT('Ctrl Pts',(-14.9415523108175,65.4764820235065,9.9989223619292));
#35036=CARTESIAN_POINT('Ctrl Pts',(-14.9354685130878,65.4463344353997,10.4860098738006));
#35037=CARTESIAN_POINT('Ctrl Pts',(-15.0596306010492,65.3812875674045,10.9740976137642));
#35038=CARTESIAN_POINT('Ctrl Pts',(-15.3070399126416,65.283216705368,11.378846829941));
#35039=CARTESIAN_POINT('Ctrl Pts',(-15.7285664365569,65.1161273209565,12.0684430664544));
#35040=CARTESIAN_POINT('Ctrl Pts',(-16.5078555104219,64.8531757502039,12.5161238918081));
#35041=CARTESIAN_POINT('Ctrl Pts',(-17.2898955363439,64.5894870640692,12.5214264196761));
#35042=CARTESIAN_POINT('Ctrl Pts',(-18.0719355622658,64.3257983779345,12.5267289475441));
#35043=CARTESIAN_POINT('Ctrl Pts',(-18.8567265402447,64.0613725764178,12.0896531779265));
#35044=CARTESIAN_POINT('Ctrl Pts',(-19.2867932233325,63.8919948632528,11.4059132558299));
#35045=CARTESIAN_POINT('Ctrl Pts',(-19.7168599064203,63.7226171500879,10.7221733337333));
#35046=CARTESIAN_POINT('Ctrl Pts',(-19.7922022946169,63.6482875252747,9.79176925915765));
#35047=CARTESIAN_POINT('Ctrl Pts',(-19.4730226094501,63.6796697714155,9.03131812620907));
#35048=CARTESIAN_POINT('Ctrl Pts',(-19.1538429242832,63.7110520175563,8.27086699326049));
#35049=CARTESIAN_POINT('Ctrl Pts',(-18.440141165753,63.8481461346511,7.68036880193896));
#35050=CARTESIAN_POINT('Ctrl Pts',(-17.6454383857669,64.0069444100311,7.52423731363907));
#35051=CARTESIAN_POINT('Ctrl Pts',(-16.8507356057808,64.165742685411,7.36810582533919));
#35052=CARTESIAN_POINT('Ctrl Pts',(-15.9750318043388,64.3462451190762,7.64634104006095));
#35053=CARTESIAN_POINT('Ctrl Pts',(-15.4043894403336,64.4450065869383,8.23435456655376));
#35054=CARTESIAN_POINT('Ctrl Pts',(-14.9553323969433,64.5227251994293,8.69708154291612));
#35055=CARTESIAN_POINT('Ctrl Pts',(-14.6951885590369,64.5498246710713,9.35164270965597));
#35056=CARTESIAN_POINT('Ctrl Pts',(-14.6789571988966,64.5115679912719,10.0021294030496));
#35057=CARTESIAN_POINT('Ctrl Pts',(-14.7480685208434,64.7775781358098,10.0015051238181));
#35058=CARTESIAN_POINT('Ctrl Pts',(-14.7649679121881,64.8206186125989,9.27681483601603));
#35059=CARTESIAN_POINT('Ctrl Pts',(-15.0958410226864,64.7795300848962,8.54799381140138));
#35060=CARTESIAN_POINT('Ctrl Pts',(-15.6402720254874,64.6812188924136,8.07917134860805));
#35061=CARTESIAN_POINT('Ctrl Pts',(-16.2577231286926,64.5697220196355,7.54746954365975));
#35062=CARTESIAN_POINT('Ctrl Pts',(-17.1498593123119,64.3846235013876,7.35018631295075));
#35063=CARTESIAN_POINT('Ctrl Pts',(-17.9258100558562,64.23065677798,7.57508388624565));
#35064=CARTESIAN_POINT('Ctrl Pts',(-18.7017607994005,64.0766900545725,7.79998145954055));
#35065=CARTESIAN_POINT('Ctrl Pts',(-19.3615261028699,63.9538551260052,8.44705983683934));
#35066=CARTESIAN_POINT('Ctrl Pts',(-19.6176065589079,63.9391872263039,9.22846362604928));
#35067=CARTESIAN_POINT('Ctrl Pts',(-19.873687014946,63.9245193266025,10.0098674152592));
#35068=CARTESIAN_POINT('Ctrl Pts',(-19.7260826235527,64.0180184557671,10.9255966163803));
#35069=CARTESIAN_POINT('Ctrl Pts',(-19.2464556042234,64.200482779956,11.5682854345738));
#35070=CARTESIAN_POINT('Ctrl Pts',(-18.7668285848942,64.3829471041448,12.2109742527673));
#35071=CARTESIAN_POINT('Ctrl Pts',(-17.9551789376289,64.654376623358,12.5806226880331));
#35072=CARTESIAN_POINT('Ctrl Pts',(-17.1785720640665,64.9164164596569,12.5127911771402));
#35073=CARTESIAN_POINT('Ctrl Pts',(-16.4019651905042,65.1784562959559,12.4449596662473));
#35074=CARTESIAN_POINT('Ctrl Pts',(-15.6604010906447,65.4311064493406,11.9396482091956));
#35075=CARTESIAN_POINT('Ctrl Pts',(-15.2897673262124,65.5843661188994,11.2216465877776));
#35076=CARTESIAN_POINT('Ctrl Pts',(-15.0989143577318,65.6632851643039,10.8519211229877));
#35077=CARTESIAN_POINT('Ctrl Pts',(-15.0064172468355,65.7158498370977,10.4257987515067));
#35078=CARTESIAN_POINT('Ctrl Pts',(-15.0130771992805,65.7418454548454,9.99981028982561));
#35079=CARTESIAN_POINT('Origin',(-17.0820569767664,63.7511045350785,10.));
#35080=CARTESIAN_POINT('',(-15.2652009106025,66.709565290414,9.99881345470565));
#35081=CARTESIAN_POINT('',(-15.1934336836835,66.4442667934687,9.99943462192771));
#35082=CARTESIAN_POINT('',(-14.6503387090836,64.4026814811241,10.));
#35083=CARTESIAN_POINT('Ctrl Pts',(-15.1934336836835,66.4442667934687,9.99943462192771));
#35084=CARTESIAN_POINT('Ctrl Pts',(-15.1827995799555,66.3950965524831,10.7909504295072));
#35085=CARTESIAN_POINT('Ctrl Pts',(-15.5599243826034,66.242026625676,11.5846294221375));
#35086=CARTESIAN_POINT('Ctrl Pts',(-16.1674256670552,66.0272275066146,12.0468004663331));
#35087=CARTESIAN_POINT('Ctrl Pts',(-16.799708927206,65.8036660249294,12.5278249876805));
#35088=CARTESIAN_POINT('Ctrl Pts',(-17.6815476659067,65.5132363543001,12.6497433013674));
#35089=CARTESIAN_POINT('Ctrl Pts',(-18.4120106025362,65.2633677075893,12.3579626123138));
#35090=CARTESIAN_POINT('Ctrl Pts',(-19.1424735391658,65.0134990608785,12.0661819232603));
#35091=CARTESIAN_POINT('Ctrl Pts',(-19.7215606737242,64.8041914380862,11.3607022314663));
#35092=CARTESIAN_POINT('Ctrl Pts',(-19.883906949622,64.7065491918251,10.5574238638967));
#35093=CARTESIAN_POINT('Ctrl Pts',(-20.0462532255198,64.608906945564,9.75414549632719));
#35094=CARTESIAN_POINT('Ctrl Pts',(-19.7918586427571,64.6229300758341,8.85306845298211));
#35095=CARTESIAN_POINT('Ctrl Pts',(-19.2285753341566,64.7197196907435,8.25767771891623));
#35096=CARTESIAN_POINT('Ctrl Pts',(-18.6652920255561,64.8165093056529,7.66228698485035));
#35097=CARTESIAN_POINT('Ctrl Pts',(-17.7931199911179,64.9960654052015,7.37258256006368));
#35098=CARTESIAN_POINT('Ctrl Pts',(-16.9965402212513,65.1553666185042,7.51828854147102));
#35099=CARTESIAN_POINT('Ctrl Pts',(-16.1999604513847,65.3146678318068,7.66399452287836));
#35100=CARTESIAN_POINT('Ctrl Pts',(-15.4789729460898,65.4537141588634,8.2451109104797));
#35101=CARTESIAN_POINT('Ctrl Pts',(-15.1503611804252,65.4876237233566,9.001424928117));
#35102=CARTESIAN_POINT('Ctrl Pts',(-15.0146236613657,65.5016305260265,9.31383062721425));
#35103=CARTESIAN_POINT('Ctrl Pts',(-14.9458338550092,65.4976987431426,9.6561287977802));
#35104=CARTESIAN_POINT('Ctrl Pts',(-14.9415523108175,65.4764820235065,9.9989223619292));
#35105=CARTESIAN_POINT('Ctrl Pts',(-15.0130771992805,65.7418454548454,9.99981028982561));
#35106=CARTESIAN_POINT('Ctrl Pts',(-15.0193507802528,65.7663329589547,9.59853518618478));
#35107=CARTESIAN_POINT('Ctrl Pts',(-15.1136101264191,65.7672447483348,9.19737890571013));
#35108=CARTESIAN_POINT('Ctrl Pts',(-15.2965249330007,65.744401378692,8.84359325274526));
#35109=CARTESIAN_POINT('Ctrl Pts',(-15.6736197332262,65.6973077831931,8.11423332491525));
#35110=CARTESIAN_POINT('Ctrl Pts',(-16.4275127626822,65.5492514064624,7.58620525503953));
#35111=CARTESIAN_POINT('Ctrl Pts',(-17.2288315064447,65.3884873478827,7.49440429239113));
#35112=CARTESIAN_POINT('Ctrl Pts',(-18.0301502502071,65.2277232893031,7.40260332974273));
#35113=CARTESIAN_POINT('Ctrl Pts',(-18.8788947082761,65.0542515488746,7.74702947432164));
#35114=CARTESIAN_POINT('Ctrl Pts',(-19.4034973688025,64.9676333413308,8.37446367269952));
#35115=CARTESIAN_POINT('Ctrl Pts',(-19.9281000293289,64.8810151337869,9.00189787107741));
#35116=CARTESIAN_POINT('Ctrl Pts',(-20.1285608923127,64.8812504591278,9.91234012325427));
#35117=CARTESIAN_POINT('Ctrl Pts',(-19.9217039083204,64.9906262726287,10.7007759738115));
#35118=CARTESIAN_POINT('Ctrl Pts',(-19.7148469243281,65.1000020861297,11.4892118243687));
#35119=CARTESIAN_POINT('Ctrl Pts',(-19.1006720933596,65.3185183877906,12.1556412733063));
#35120=CARTESIAN_POINT('Ctrl Pts',(-18.3583974645568,65.5713589268319,12.4036017192683));
#35121=CARTESIAN_POINT('Ctrl Pts',(-17.616122835754,65.8241994658732,12.6515621652302));
#35122=CARTESIAN_POINT('Ctrl Pts',(-16.745748409117,66.1113642422947,12.4810536082165));
#35123=CARTESIAN_POINT('Ctrl Pts',(-16.1404633167949,66.3274985456644,11.9679250313905));
#35124=CARTESIAN_POINT('Ctrl Pts',(-15.5886775085546,66.5245294039924,11.5001503082284));
#35125=CARTESIAN_POINT('Ctrl Pts',(-15.2571911193414,66.662531210899,10.7476451883995));
#35126=CARTESIAN_POINT('Ctrl Pts',(-15.2652009106025,66.709565290414,9.99881345470565));
#35127=CARTESIAN_POINT('Origin',(-17.0820569767664,63.7511045350785,10.));
#35128=CARTESIAN_POINT('',(-15.5286491313886,67.6742507328171,10.0019962882658));
#35129=CARTESIAN_POINT('',(-15.458048217099,67.4086397233445,10.0018117506529));
#35130=CARTESIAN_POINT('',(-14.6503387090836,64.4026814811241,10.));
#35131=CARTESIAN_POINT('',(-20.2598690437799,67.0040126136404,11.1728309286209));
#35132=CARTESIAN_POINT('Ctrl Pts',(-15.5286491313886,67.6742507328171,10.0019962882658));
#35133=CARTESIAN_POINT('Ctrl Pts',(-15.5421457071955,67.7079511930089,9.43113200366978));
#35134=CARTESIAN_POINT('Ctrl Pts',(-15.7382477902416,67.6927226550025,8.85763821511467));
#35135=CARTESIAN_POINT('Ctrl Pts',(-16.0921495062908,67.635211832767,8.41584216487545));
#35136=CARTESIAN_POINT('Ctrl Pts',(-16.6037821050588,67.5520689427971,7.77714150008994));
#35137=CARTESIAN_POINT('Ctrl Pts',(-17.4452195762655,67.3805551035975,7.41369214583754));
#35138=CARTESIAN_POINT('Ctrl Pts',(-18.2482818068303,67.2193238791371,7.48861537411896));
#35139=CARTESIAN_POINT('Ctrl Pts',(-19.0513440373952,67.0580926546768,7.56353860240037));
#35140=CARTESIAN_POINT('Ctrl Pts',(-19.8160310273183,66.9071440449558,8.07683441321559));
#35141=CARTESIAN_POINT('Ctrl Pts',(-20.2075211669018,66.8561932299011,8.79681637620262));
#35142=CARTESIAN_POINT('Ctrl Pts',(-20.5990113064853,66.8052424148464,9.51679833918964));
#35143=CARTESIAN_POINT('Ctrl Pts',(-20.6173045957293,66.854289394458,10.4434664543485));
#35144=CARTESIAN_POINT('Ctrl Pts',(-20.25986904378,67.0040126136404,11.1728309286208));
#35145=CARTESIAN_POINT('',(-16.4802525979517,68.0323660008167,11.867050568706));
#35146=CARTESIAN_POINT('Ctrl Pts',(-16.4806955947431,68.0322473001842,11.8669181223568));
#35147=CARTESIAN_POINT('Ctrl Pts',(-16.6817854205936,67.9835336336722,12.0540417240895));
#35148=CARTESIAN_POINT('Ctrl Pts',(-16.9239334961961,67.923876532405,12.2143044024353));
#35149=CARTESIAN_POINT('Ctrl Pts',(-17.4856657502708,67.7816176378542,12.4543153408643));
#35150=CARTESIAN_POINT('Ctrl Pts',(-17.8119729521746,67.6966288605656,12.5175));
#35151=CARTESIAN_POINT('Ctrl Pts',(-18.4226933621783,67.5329868199039,12.5175));
#35152=CARTESIAN_POINT('Ctrl Pts',(-18.7477780771091,67.4434356591205,12.4543153408643));
#35153=CARTESIAN_POINT('Ctrl Pts',(-19.3446857260753,67.274655929957,12.1973867613172));
#35154=CARTESIAN_POINT('Ctrl Pts',(-19.6165425195547,67.1955448337828,12.0036443501621));
#35155=CARTESIAN_POINT('Ctrl Pts',(-19.9960747381914,67.0834304248293,11.6080270340045));
#35156=CARTESIAN_POINT('Ctrl Pts',(-20.1448248140072,67.0387983068925,11.4009948671635));
#35157=CARTESIAN_POINT('Ctrl Pts',(-20.2598690437799,67.0040126136404,11.1728309286209));
#35158=CARTESIAN_POINT('Ctrl Pts',(-16.4776938604224,68.0330516124713,11.8678155752476));
#35159=CARTESIAN_POINT('Ctrl Pts',(-16.9785524830599,67.8522271893254,12.3404055365586));
#35160=CARTESIAN_POINT('Ctrl Pts',(-17.6838006560652,67.616636751217,12.5855412104356));
#35161=CARTESIAN_POINT('Ctrl Pts',(-18.3529108900526,67.3907294446846,12.5051234941038));
#35162=CARTESIAN_POINT('Ctrl Pts',(-19.1299796896385,67.1283727946321,12.4117306641615));
#35163=CARTESIAN_POINT('Ctrl Pts',(-19.8583083259858,66.8790760319583,11.8792556448934));
#35164=CARTESIAN_POINT('Ctrl Pts',(-20.2061471825011,66.7317311985188,11.1455779206963));
#35165=CARTESIAN_POINT('Ctrl Pts',(-20.5539860390165,66.5843863650793,10.4119001964992));
#35166=CARTESIAN_POINT('Ctrl Pts',(-20.5213351157,66.538993460874,9.4770197673732));
#35167=CARTESIAN_POINT('Ctrl Pts',(-20.1165357938137,66.5933174195301,8.75982961781592));
#35168=CARTESIAN_POINT('Ctrl Pts',(-19.7117364719275,66.6476413781861,8.04263946825864));
#35169=CARTESIAN_POINT('Ctrl Pts',(-18.9347887514715,66.8016821997034,7.54313959827013));
#35170=CARTESIAN_POINT('Ctrl Pts',(-18.1276415422752,66.9638149498405,7.48486270274581));
#35171=CARTESIAN_POINT('Ctrl Pts',(-17.320494333079,67.1259476999776,7.42658580722149));
#35172=CARTESIAN_POINT('Ctrl Pts',(-16.4831476351424,67.2961723787345,7.80953188616136));
#35173=CARTESIAN_POINT('Ctrl Pts',(-15.9844353298858,67.3756602454434,8.46229096311787));
#35174=CARTESIAN_POINT('Ctrl Pts',(-15.6526293851287,67.4285455390928,8.89658813193721));
#35175=CARTESIAN_POINT('Ctrl Pts',(-15.4707226080323,67.4412654718215,9.450320138744));
#35176=CARTESIAN_POINT('Ctrl Pts',(-15.458048217099,67.4086397233445,10.0018117506529));
#35177=CARTESIAN_POINT('Origin',(-63.7511045350785,-17.0820569767664,10.));
#35178=CARTESIAN_POINT('',(-60.9122168113323,-13.7189801527801,9.99965378812949));
#35179=CARTESIAN_POINT('',(-60.6472937215209,-13.6458118873637,9.99664393251001));
#35180=CARTESIAN_POINT('',(-64.4026814811241,-14.6503387090836,10.));
#35181=CARTESIAN_POINT('',(-60.3826426720153,-14.1985145724515,11.6359872033749));
#35182=CARTESIAN_POINT('Ctrl Pts',(-60.6472937215209,-13.6458118873637,
9.99664393251001));
#35183=CARTESIAN_POINT('Ctrl Pts',(-60.6097205320263,-13.6410407802455,
10.5892058593235));
#35184=CARTESIAN_POINT('Ctrl Pts',(-60.5187326677745,-13.8356159531908,
11.1848035603043));
#35185=CARTESIAN_POINT('Ctrl Pts',(-60.3826426720153,-14.1985145724514,
11.6359872033748));
#35186=CARTESIAN_POINT('',(-59.3912531651587,-17.8984305821306,11.6380816927068));
#35187=CARTESIAN_POINT('Origin',(-59.8874012299222,-16.0467807963563,10.));
#35188=CARTESIAN_POINT('Ctrl Pts',(-59.3912467107622,-17.8984546702664,
11.6380966037222));
#35189=CARTESIAN_POINT('Ctrl Pts',(-59.5701794123022,-17.4212611177619,
12.2270179049199));
#35190=CARTESIAN_POINT('Ctrl Pts',(-59.8253574740882,-16.6595160069785,
12.5674221981558));
#35191=CARTESIAN_POINT('Ctrl Pts',(-60.0736878712825,-15.9233267283639,
12.5157167035403));
#35192=CARTESIAN_POINT('Ctrl Pts',(-60.3360206084695,-15.1456267338057,
12.4610957466082));
#35193=CARTESIAN_POINT('Ctrl Pts',(-60.590711685935,-14.3964458015822,11.9688993897476));
#35194=CARTESIAN_POINT('Ctrl Pts',(-60.7469740189125,-14.0146059447133,
11.2575578209422));
#35195=CARTESIAN_POINT('Ctrl Pts',(-60.8300361143405,-13.8116368860469,
10.8794403300268));
#35196=CARTESIAN_POINT('Ctrl Pts',(-60.8852870497794,-13.7124604894775,
10.439403096236));
#35197=CARTESIAN_POINT('Ctrl Pts',(-60.9122168113323,-13.7189801527801,
9.99965378812949));
#35198=CARTESIAN_POINT('Origin',(-63.7511045350785,-17.0820569767664,10.));
#35199=CARTESIAN_POINT('',(-61.8799991994799,-13.9708704146993,9.99901528063941));
#35200=CARTESIAN_POINT('',(-61.614467077582,-13.8999750879731,10.0012573013837));
#35201=CARTESIAN_POINT('',(-64.4026814811241,-14.6503387090836,10.));
#35202=CARTESIAN_POINT('Ctrl Pts',(-61.614467077582,-13.8999750879731,10.0012573013837));
#35203=CARTESIAN_POINT('Ctrl Pts',(-61.6099667912196,-13.8982899610888,
10.0766544396887));
#35204=CARTESIAN_POINT('Ctrl Pts',(-61.6045451170745,-13.900043500223,10.1520128061816));
#35205=CARTESIAN_POINT('Ctrl Pts',(-61.5981695663354,-13.90535695527,10.2270376921987));
#35206=CARTESIAN_POINT('Ctrl Pts',(-61.5284611611193,-13.9634527171372,
11.0473378309362));
#35207=CARTESIAN_POINT('Ctrl Pts',(-61.3447206686645,-14.4471220222726,
11.8277717281247));
#35208=CARTESIAN_POINT('Ctrl Pts',(-61.1066011161456,-15.1337367424349,
12.218961128923));
#35209=CARTESIAN_POINT('Ctrl Pts',(-60.8684815636268,-15.8203514625973,
12.6101505297213));
#35210=CARTESIAN_POINT('Ctrl Pts',(-60.5759829510438,-16.7099115977865,
12.6120954341293));
#35211=CARTESIAN_POINT('Ctrl Pts',(-60.3374667150895,-17.3980067606846,
12.2237523563128));
#35212=CARTESIAN_POINT('Ctrl Pts',(-60.0989504791351,-18.0861019235828,
11.8354092784963));
#35213=CARTESIAN_POINT('Ctrl Pts',(-59.9144166198093,-18.5727321141897,
11.0567782184552));
#35214=CARTESIAN_POINT('Ctrl Pts',(-59.8438645695582,-18.6339764021913,
10.2368654679636));
#35215=CARTESIAN_POINT('Ctrl Pts',(-59.7733125193071,-18.6952206901928,
9.41695271747191));
#35216=CARTESIAN_POINT('Ctrl Pts',(-59.8167422781307,-18.3310790755889,
8.55575827652964));
#35217=CARTESIAN_POINT('Ctrl Pts',(-59.9321107539311,-17.6984585141965,
8.03819621078659));
#35218=CARTESIAN_POINT('Ctrl Pts',(-60.0474792297314,-17.065837952804,7.52063414504355));
#35219=CARTESIAN_POINT('Ctrl Pts',(-60.2347864225086,-16.1647384446229,
7.34670445449967));
#35220=CARTESIAN_POINT('Ctrl Pts',(-60.3874931590403,-15.3927695971148,
7.5957513454432));
#35221=CARTESIAN_POINT('Ctrl Pts',(-60.540199895572,-14.6208007496067,7.84479823638674));
#35222=CARTESIAN_POINT('Ctrl Pts',(-60.6583061758583,-13.9779625627716,
8.5168217088177));
#35223=CARTESIAN_POINT('Ctrl Pts',(-60.6663289586339,-13.7459615817213,
9.30743209219192));
#35224=CARTESIAN_POINT('Ctrl Pts',(-60.6685946628634,-13.6804424696226,
9.53070739947774));
#35225=CARTESIAN_POINT('Ctrl Pts',(-60.6620806891943,-13.6476895615158,
9.76344057197151));
#35226=CARTESIAN_POINT('Ctrl Pts',(-60.6472937215209,-13.6458118873637,
9.99664393251001));
#35227=CARTESIAN_POINT('Ctrl Pts',(-60.9122168113323,-13.7189801527801,
9.99965378812949));
#35228=CARTESIAN_POINT('Ctrl Pts',(-60.9359492362449,-13.7247257446778,
9.61211536100754));
#35229=CARTESIAN_POINT('Ctrl Pts',(-60.9376863320054,-13.8125590225004,
9.22480054821117));
#35230=CARTESIAN_POINT('Ctrl Pts',(-60.9170790299752,-13.9837827281424,
8.88028612326268));
#35231=CARTESIAN_POINT('Ctrl Pts',(-60.8730881195709,-14.3492981499548,
8.14484277513894));
#35232=CARTESIAN_POINT('Ctrl Pts',(-60.7272727102728,-15.0948277750941,
7.60444285964178));
#35233=CARTESIAN_POINT('Ctrl Pts',(-60.5669204894782,-15.8946095193183,
7.4993584305648));
#35234=CARTESIAN_POINT('Ctrl Pts',(-60.4065682686836,-16.6943912635425,
7.39427400148783));
#35235=CARTESIAN_POINT('Ctrl Pts',(-60.2316792363925,-17.5484251268517,
7.72450505883104));
#35236=CARTESIAN_POINT('Ctrl Pts',(-60.1424305723415,-18.0828447847102,
8.34320956294461));
#35237=CARTESIAN_POINT('Ctrl Pts',(-60.0531819082904,-18.6172644425688,
8.96191406705817));
#35238=CARTESIAN_POINT('Ctrl Pts',(-60.0495736124794,-18.8320698949766,
9.86909201794208));
#35239=CARTESIAN_POINT('Ctrl Pts',(-60.1556096340356,-18.6376771842087,
10.6611508664108));
#35240=CARTESIAN_POINT('Ctrl Pts',(-60.2616456555918,-18.4432844734408,
11.4532097148796));
#35241=CARTESIAN_POINT('Ctrl Pts',(-60.4773259945152,-17.8396935994972,
12.1301494609332));
#35242=CARTESIAN_POINT('Ctrl Pts',(-60.7290924921508,-17.1014273477897,
12.3908459426515));
#35243=CARTESIAN_POINT('Ctrl Pts',(-60.9808589897864,-16.3631610960823,
12.6515424243699));
#35244=CARTESIAN_POINT('Ctrl Pts',(-61.2687116461342,-15.4902194666109,
12.495995641753));
#35245=CARTESIAN_POINT('Ctrl Pts',(-61.4869914228005,-14.8769273589399,
11.993393721437));
#35246=CARTESIAN_POINT('Ctrl Pts',(-61.6896056365772,-14.3076501674885,
11.5268626736103));
#35247=CARTESIAN_POINT('Ctrl Pts',(-61.8322748736988,-13.9620906745725,
10.7613040129745));
#35248=CARTESIAN_POINT('Ctrl Pts',(-61.8799991994799,-13.9708704146993,
9.99901528063941));
#35249=CARTESIAN_POINT('Origin',(-63.7511045350785,-17.0820569767664,10.));
#35250=CARTESIAN_POINT('',(-62.8445369550162,-14.2348698103756,10.0018466754434));
#35251=CARTESIAN_POINT('',(-62.5785998445538,-14.1654859215485,10.0004462653844));
#35252=CARTESIAN_POINT('',(-64.4026814811241,-14.6503387090836,10.));
#35253=CARTESIAN_POINT('Ctrl Pts',(-62.5785998445538,-14.1654859215485,
10.0004462653844));
#35254=CARTESIAN_POINT('Ctrl Pts',(-62.5552558244195,-14.1585827534688,
10.3867702486341));
#35255=CARTESIAN_POINT('Ctrl Pts',(-62.5100553152291,-14.2332491130213,
10.7728367424034));
#35256=CARTESIAN_POINT('Ctrl Pts',(-62.4426252563818,-14.3908772813228,
11.1164878478954));
#35257=CARTESIAN_POINT('Ctrl Pts',(-62.2977170112847,-14.729622666347,11.8549994178658));
#35258=CARTESIAN_POINT('Ctrl Pts',(-62.0501467519025,-15.4515079046908,
12.3976253642211));
#35259=CARTESIAN_POINT('Ctrl Pts',(-61.7881520526304,-16.2272258855744,
12.501389418797));
#35260=CARTESIAN_POINT('Ctrl Pts',(-61.5261573533583,-17.0029438664579,
12.6051534733729));
#35261=CARTESIAN_POINT('Ctrl Pts',(-61.2497382141963,-17.8324945898812,
12.2700556361695));
#35262=CARTESIAN_POINT('Ctrl Pts',(-61.0600503079338,-18.3383599455202,
11.6461438143238));
#35263=CARTESIAN_POINT('Ctrl Pts',(-60.8703624016714,-18.8442253011593,
11.0222319924781));
#35264=CARTESIAN_POINT('Ctrl Pts',(-60.7674057283085,-19.0264052890141,
10.1095061859902));
#35265=CARTESIAN_POINT('Ctrl Pts',(-60.7746625458238,-18.7972629292321,
9.31667252204661));
#35266=CARTESIAN_POINT('Ctrl Pts',(-60.7819193633391,-18.56812056945,8.52383885810307));
#35267=CARTESIAN_POINT('Ctrl Pts',(-60.8993896717326,-17.9276558620312,
7.85089733670394));
#35268=CARTESIAN_POINT('Ctrl Pts',(-61.051853263826,-17.1565944419204,7.59916807226832));
#35269=CARTESIAN_POINT('Ctrl Pts',(-61.2043168559194,-16.3855330218097,
7.3474388078327));
#35270=CARTESIAN_POINT('Ctrl Pts',(-61.3917737317128,-15.4838748890071,
7.51692180036059));
#35271=CARTESIAN_POINT('Ctrl Pts',(-61.5076640106208,-14.8493069319054,
8.03174648676773));
#35272=CARTESIAN_POINT('Ctrl Pts',(-61.6129549313732,-14.2727767422054,
8.49948515966285));
#35273=CARTESIAN_POINT('Ctrl Pts',(-61.6591716047613,-13.9167146450877,
9.25228420341937));
#35274=CARTESIAN_POINT('Ctrl Pts',(-61.614467077582,-13.8999750879731,10.0012573013837));
#35275=CARTESIAN_POINT('Ctrl Pts',(-61.8799991994799,-13.9708704146993,
9.99901528063941));
#35276=CARTESIAN_POINT('Ctrl Pts',(-61.8836891105327,-13.971549239588,9.94007725327294));
#35277=CARTESIAN_POINT('Ctrl Pts',(-61.8868114457663,-13.9743462862715,
9.88115877337042));
#35278=CARTESIAN_POINT('Ctrl Pts',(-61.8893500282723,-13.9793219277933,
9.82239956232329));
#35279=CARTESIAN_POINT('Ctrl Pts',(-61.9247219600932,-14.0486511901884,
9.00366438154083));
#35280=CARTESIAN_POINT('Ctrl Pts',(-61.8467589267501,-14.5409523008493,
8.21585107799109));
#35281=CARTESIAN_POINT('Ctrl Pts',(-61.7125351424541,-15.2432213925386,
7.80941972573615));
#35282=CARTESIAN_POINT('Ctrl Pts',(-61.5783113581581,-15.9454904842279,
7.40298837348122));
#35283=CARTESIAN_POINT('Ctrl Pts',(-61.3878268229091,-16.8577275569455,
7.3779389725211));
#35284=CARTESIAN_POINT('Ctrl Pts',(-61.2482107604142,-17.5801209048414,
7.74541574302308));
#35285=CARTESIAN_POINT('Ctrl Pts',(-61.1085946979193,-18.3025142527372,
8.11289251352506));
#35286=CARTESIAN_POINT('Ctrl Pts',(-61.0198471081786,-18.8350638758112,
8.87289545548915));
#35287=CARTESIAN_POINT('Ctrl Pts',(-61.0438394390412,-18.9468623871524,
9.68733378926602));
#35288=CARTESIAN_POINT('Ctrl Pts',(-61.0678317699037,-19.0586608984937,
10.5017721230429));
#35289=CARTESIAN_POINT('Ctrl Pts',(-61.2045640213696,-18.7497082981023,
11.3706458486326));
#35290=CARTESIAN_POINT('Ctrl Pts',(-61.4156018821481,-18.1634433884685,
11.9074332417682));
#35291=CARTESIAN_POINT('Ctrl Pts',(-61.6266397429266,-17.5771784788347,
12.4442206349039));
#35292=CARTESIAN_POINT('Ctrl Pts',(-61.9119832130178,-16.7136012599587,
12.6489216955855));
#35293=CARTESIAN_POINT('Ctrl Pts',(-62.1670877632025,-15.9628772265398,
12.4304742338455));
#35294=CARTESIAN_POINT('Ctrl Pts',(-62.4221923133871,-15.2121531931209,
12.2120267721055));
#35295=CARTESIAN_POINT('Ctrl Pts',(-62.6470579436653,-14.5742823451591,
11.5704307879438));
#35296=CARTESIAN_POINT('Ctrl Pts',(-62.7640438959386,-14.3390239366158,
10.7911028658277));
#35297=CARTESIAN_POINT('Ctrl Pts',(-62.8020535673525,-14.2625865983513,
10.5378929917554));
#35298=CARTESIAN_POINT('Ctrl Pts',(-62.828674898289,-14.2286511253629,10.2701434172216));
#35299=CARTESIAN_POINT('Ctrl Pts',(-62.8445369550162,-14.2348698103756,
10.0018466754434));
#35300=CARTESIAN_POINT('Origin',(-63.7511045350785,-17.0820569767664,10.));
#35301=CARTESIAN_POINT('',(-63.8107147438124,-14.4927485186002,9.99793352624079));
#35302=CARTESIAN_POINT('',(-63.5459612763503,-14.4189472139579,9.99811000378506));
#35303=CARTESIAN_POINT('',(-64.4026814811241,-14.6503387090836,10.));
#35304=CARTESIAN_POINT('Ctrl Pts',(-63.5459612763503,-14.4189472139579,
9.99811000378506));
#35305=CARTESIAN_POINT('Ctrl Pts',(-63.5020657997403,-14.4131993125783,
10.6909216248416));
#35306=CARTESIAN_POINT('Ctrl Pts',(-63.3825723034678,-14.6895870615306,
11.3881278716998));
#35307=CARTESIAN_POINT('Ctrl Pts',(-63.2084966963919,-15.1696780211858,
11.8560065223222));
#35308=CARTESIAN_POINT('Ctrl Pts',(-63.0010658835769,-15.7417608055529,
12.4135369565264));
#35309=CARTESIAN_POINT('Ctrl Pts',(-62.7161316220184,-16.6030903983926,
12.6454354329572));
#35310=CARTESIAN_POINT('Ctrl Pts',(-62.4586624096387,-17.3619190322647,
12.4478622804133));
#35311=CARTESIAN_POINT('Ctrl Pts',(-62.201193197259,-18.1207476661368,12.2502891278694));
#35312=CARTESIAN_POINT('Ctrl Pts',(-61.9711890340581,-18.7770753410412,
11.6232443463506));
#35313=CARTESIAN_POINT('Ctrl Pts',(-61.8490217755358,-19.030950208754,10.8475065234704));
#35314=CARTESIAN_POINT('Ctrl Pts',(-61.7268545170136,-19.2848250764668,
10.0717687005902));
#35315=CARTESIAN_POINT('Ctrl Pts',(-61.71252416317,-19.1362471369879,9.14733783634849));
#35316=CARTESIAN_POINT('Ctrl Pts',(-61.789827971849,-18.6456858472655,8.48815640829349));
#35317=CARTESIAN_POINT('Ctrl Pts',(-61.867131780528,-18.155124557543,7.82897498023847));
#35318=CARTESIAN_POINT('Ctrl Pts',(-62.0360697517297,-17.3225799175769,
7.43504298837015));
#35319=CARTESIAN_POINT('Ctrl Pts',(-62.1983751106924,-16.5147885234736,
7.48275547481142));
#35320=CARTESIAN_POINT('Ctrl Pts',(-62.3606804696551,-15.7069971293704,
7.53046796125269));
#35321=CARTESIAN_POINT('Ctrl Pts',(-62.5163532163789,-14.9239589811299,
8.01982492600353));
#35322=CARTESIAN_POINT('Ctrl Pts',(-62.5730664743348,-14.510242672862,8.73170200517163));
#35323=CARTESIAN_POINT('Ctrl Pts',(-62.6033893890854,-14.2890407035394,
9.11232178902019));
#35324=CARTESIAN_POINT('Ctrl Pts',(-62.6054224867212,-14.1734177690262,
9.55655400073809));
#35325=CARTESIAN_POINT('Ctrl Pts',(-62.5785998445538,-14.1654859215485,
10.0004462653844));
#35326=CARTESIAN_POINT('Ctrl Pts',(-62.8445369550162,-14.2348698103756,
10.0018466754434));
#35327=CARTESIAN_POINT('Ctrl Pts',(-62.8774950470096,-14.2477909590166,
9.44438121878235));
#35328=CARTESIAN_POINT('Ctrl Pts',(-62.8640028840737,-14.4340668190783,
8.884553515607));
#35329=CARTESIAN_POINT('Ctrl Pts',(-62.8097033887247,-14.772637717027,8.44788099502279));
#35330=CARTESIAN_POINT('Ctrl Pts',(-62.7292706549692,-15.2741558751066,
7.80104690640428));
#35331=CARTESIAN_POINT('Ctrl Pts',(-62.5592989131897,-16.109838160391,7.42443858923766));
#35332=CARTESIAN_POINT('Ctrl Pts',(-62.3977923938506,-16.9139278054305,
7.48559176785143));
#35333=CARTESIAN_POINT('Ctrl Pts',(-62.2362858745115,-17.7180174504699,
7.54674494646519));
#35334=CARTESIAN_POINT('Ctrl Pts',(-62.0832445776127,-18.4905144552645,
8.04565962085933));
#35335=CARTESIAN_POINT('Ctrl Pts',(-62.0291411621378,-18.8937702597922,
8.76039160250466));
#35336=CARTESIAN_POINT('Ctrl Pts',(-61.9750377466629,-19.2970260643198,
9.47512358415));
#35337=CARTESIAN_POINT('Ctrl Pts',(-62.0198722126119,-19.3310406685804,
10.4056728730465));
#35338=CARTESIAN_POINT('Ctrl Pts',(-62.1660913946904,-18.9866823611347,
11.1380809107435));
#35339=CARTESIAN_POINT('Ctrl Pts',(-62.3123105767689,-18.6423240536889,
11.8704889484405));
#35340=CARTESIAN_POINT('Ctrl Pts',(-62.5599144749769,-17.9195928345367,
12.404755734938));
#35341=CARTESIAN_POINT('Ctrl Pts',(-62.8211471346507,-17.1459983851501,
12.5032105584454));
#35342=CARTESIAN_POINT('Ctrl Pts',(-63.0823797943245,-16.3724039357634,
12.6016653819528));
#35343=CARTESIAN_POINT('Ctrl Pts',(-63.3572412154641,-15.5479462561424,
12.2643082424701));
#35344=CARTESIAN_POINT('Ctrl Pts',(-63.5458498251154,-15.045388451291,11.6412138094001));
#35345=CARTESIAN_POINT('Ctrl Pts',(-63.6819468306564,-14.6827506455304,
11.1915986689945));
#35346=CARTESIAN_POINT('Ctrl Pts',(-63.7731333897311,-14.4877209077723,
10.593204732795));
#35347=CARTESIAN_POINT('Ctrl Pts',(-63.8107147438124,-14.4927485186002,
9.99793352624079));
#35348=CARTESIAN_POINT('Origin',(-63.7511045350785,-17.0820569767664,10.));
#35349=CARTESIAN_POINT('',(-64.7775781358098,-14.7480685208434,10.001505123818));
#35350=CARTESIAN_POINT('',(-64.511567991272,-14.6789571988966,10.0021294030496));
#35351=CARTESIAN_POINT('',(-64.4026814811241,-14.6503387090836,10.));
#35352=CARTESIAN_POINT('Ctrl Pts',(-64.511567991272,-14.6789571988966,10.0021294030496));
#35353=CARTESIAN_POINT('Ctrl Pts',(-64.5012097288919,-14.6745624451438,
10.1782532036584));
#35354=CARTESIAN_POINT('Ctrl Pts',(-64.4860602506939,-14.6880487522533,
10.3540783073471));
#35355=CARTESIAN_POINT('Ctrl Pts',(-64.4658270415774,-14.7205078014429,
10.5257161206908));
#35356=CARTESIAN_POINT('Ctrl Pts',(-64.3708655262952,-14.872849453126,11.3312723100706));
#35357=CARTESIAN_POINT('Ctrl Pts',(-64.1639219936719,-15.4431136830603,
12.0445928505662));
#35358=CARTESIAN_POINT('Ctrl Pts',(-63.9150421900725,-16.1698862069574,
12.3462664892696));
#35359=CARTESIAN_POINT('Ctrl Pts',(-63.666162386473,-16.8966587308546,12.6479401279729));
#35360=CARTESIAN_POINT('Ctrl Pts',(-63.3753463118975,-17.7799395487145,
12.5379668648841));
#35361=CARTESIAN_POINT('Ctrl Pts',(-63.1501962278717,-18.4181515535134,
12.065590617606));
#35362=CARTESIAN_POINT('Ctrl Pts',(-62.9250461438459,-19.0563635583123,
11.5932143703279));
#35363=CARTESIAN_POINT('Ctrl Pts',(-62.7655620503699,-19.4495067500503,
10.7584351388606));
#35364=CARTESIAN_POINT('Ctrl Pts',(-62.7205382674991,-19.4154782471594,
9.93505104704512));
#35365=CARTESIAN_POINT('Ctrl Pts',(-62.6755144846283,-19.3814497442686,
9.11166695522964));
#35366=CARTESIAN_POINT('Ctrl Pts',(-62.7449510123627,-18.9202495467491,
8.29967800306603));
#35367=CARTESIAN_POINT('Ctrl Pts',(-62.8751359084421,-18.2323333520887,
7.86267726611249));
#35368=CARTESIAN_POINT('Ctrl Pts',(-63.0053208045216,-17.5444171574283,
7.42567652915895));
#35369=CARTESIAN_POINT('Ctrl Pts',(-63.1962540689462,-16.629784965627,7.36366400741547));
#35370=CARTESIAN_POINT('Ctrl Pts',(-63.3398198518216,-15.8919306215937,
7.70440771629226));
#35371=CARTESIAN_POINT('Ctrl Pts',(-63.4833856346971,-15.1540762775603,
8.04515142516905));
#35372=CARTESIAN_POINT('Ctrl Pts',(-63.5795839360235,-14.5929997812949,
8.78865136466612));
#35373=CARTESIAN_POINT('Ctrl Pts',(-63.5627194046509,-14.4538795211094,
9.60198253040337));
#35374=CARTESIAN_POINT('Ctrl Pts',(-63.5600075610921,-14.4315087612499,
9.73276747984748));
#35375=CARTESIAN_POINT('Ctrl Pts',(-63.5543722345421,-14.4200485884486,
9.86535806600966));
#35376=CARTESIAN_POINT('Ctrl Pts',(-63.5459612763503,-14.4189472139579,
9.99811000378506));
#35377=CARTESIAN_POINT('Ctrl Pts',(-63.8107147438124,-14.4927485186002,
9.99793352624079));
#35378=CARTESIAN_POINT('Ctrl Pts',(-63.8252151156582,-14.494688369579,9.76825436605187));
#35379=CARTESIAN_POINT('Ctrl Pts',(-63.8317351659301,-14.526411186132,9.53904009330736));
#35380=CARTESIAN_POINT('Ctrl Pts',(-63.8297754611264,-14.5897808794636,
9.31901604644665));
#35381=CARTESIAN_POINT('Ctrl Pts',(-63.822736689323,-14.8173890425691,8.52874444322085));
#35382=CARTESIAN_POINT('Ctrl Pts',(-63.706303347553,-15.453263298862,7.85703296342678));
#35383=CARTESIAN_POINT('Ctrl Pts',(-63.5546628984884,-16.220532268366,7.60269513736962));
#35384=CARTESIAN_POINT('Ctrl Pts',(-63.4030224494238,-16.9878012378701,
7.34835731131246));
#35385=CARTESIAN_POINT('Ctrl Pts',(-63.2161748930645,-17.8864649205853,
7.51139313899221));
#35386=CARTESIAN_POINT('Ctrl Pts',(-63.0996317362701,-18.5227490121286,
8.01927548227196));
#35387=CARTESIAN_POINT('Ctrl Pts',(-62.9830885794758,-19.1590331036718,
8.52715782555172));
#35388=CARTESIAN_POINT('Ctrl Pts',(-62.9368498222464,-19.532937604043,9.37988668443149));
#35389=CARTESIAN_POINT('Ctrl Pts',(-63.0038765864645,-19.4841294236266,
10.1981222260482));
#35390=CARTESIAN_POINT('Ctrl Pts',(-63.0709033506825,-19.4353212432102,
11.016357767665));
#35391=CARTESIAN_POINT('Ctrl Pts',(-63.2511956363481,-18.9638003820061,
11.8000999920187));
#35392=CARTESIAN_POINT('Ctrl Pts',(-63.486941327682,-18.2853245933946,12.2006980454404));
#35393=CARTESIAN_POINT('Ctrl Pts',(-63.722687019016,-17.6068488047831,12.6012960988621));
#35394=CARTESIAN_POINT('Ctrl Pts',(-64.0138861160184,-16.7214180887641,
12.6187499813518));
#35395=CARTESIAN_POINT('Ctrl Pts',(-64.2533891656508,-16.0289196480805,
12.2452952639451));
#35396=CARTESIAN_POINT('Ctrl Pts',(-64.4928922152833,-15.3364212073968,
11.8718405465384));
#35397=CARTESIAN_POINT('Ctrl Pts',(-64.6806992175458,-14.8368550420484,
11.1074772292354));
#35398=CARTESIAN_POINT('Ctrl Pts',(-64.7556551050229,-14.7584549707697,
10.29223538099));
#35399=CARTESIAN_POINT('Ctrl Pts',(-64.7645194286933,-14.7491833360657,
10.1958244404253));
#35400=CARTESIAN_POINT('Ctrl Pts',(-64.7718054668758,-14.7458019429916,
10.0987019353609));
#35401=CARTESIAN_POINT('Ctrl Pts',(-64.7775781358098,-14.7480685208434,
10.001505123818));
#35402=CARTESIAN_POINT('Origin',(-63.7511045350785,-17.0820569767664,10.));
#35403=CARTESIAN_POINT('',(-65.7418454548455,-15.0130771992805,9.99981028982562));
#35404=CARTESIAN_POINT('',(-65.4764820235065,-14.9415523108175,9.99892236192921));
#35405=CARTESIAN_POINT('',(-64.4026814811241,-14.6503387090836,10.));
#35406=CARTESIAN_POINT('Ctrl Pts',(-65.4764820235065,-14.9415523108175,
9.99892236192921));
#35407=CARTESIAN_POINT('Ctrl Pts',(-65.4463344353997,-14.9354685130878,
10.4860098738008));
#35408=CARTESIAN_POINT('Ctrl Pts',(-65.3812875674044,-15.0596306010494,
10.9740976137646));
#35409=CARTESIAN_POINT('Ctrl Pts',(-65.2832167053678,-15.3070399126419,
11.3788468299415));
#35410=CARTESIAN_POINT('Ctrl Pts',(-65.1161273209563,-15.7285664365574,
12.0684430664548));
#35411=CARTESIAN_POINT('Ctrl Pts',(-64.8531757502037,-16.5078555104225,
12.5161238918083));
#35412=CARTESIAN_POINT('Ctrl Pts',(-64.589487064069,-17.2898955363445,12.5214264196761));
#35413=CARTESIAN_POINT('Ctrl Pts',(-64.3257983779344,-18.0719355622664,
12.5267289475439));
#35414=CARTESIAN_POINT('Ctrl Pts',(-64.0613725764176,-18.8567265402452,
12.0896531779261));
#35415=CARTESIAN_POINT('Ctrl Pts',(-63.8919948632527,-19.2867932233328,
11.4059132558293));
#35416=CARTESIAN_POINT('Ctrl Pts',(-63.7226171500878,-19.7168599064204,
10.7221733337326));
#35417=CARTESIAN_POINT('Ctrl Pts',(-63.6482875252747,-19.7922022946168,
9.79176925915698));
#35418=CARTESIAN_POINT('Ctrl Pts',(-63.6796697714156,-19.4730226094498,
9.03131812620849));
#35419=CARTESIAN_POINT('Ctrl Pts',(-63.7110520175564,-19.1538429242828,
8.27086699325998));
#35420=CARTESIAN_POINT('Ctrl Pts',(-63.8481461346512,-18.4401411657524,
7.68036880193864));
#35421=CARTESIAN_POINT('Ctrl Pts',(-64.0069444100312,-17.6454383857663,
7.52423731363896));
#35422=CARTESIAN_POINT('Ctrl Pts',(-64.1657426854112,-16.8507356057801,
7.36810582533927));
#35423=CARTESIAN_POINT('Ctrl Pts',(-64.3462451190763,-15.9750318043382,
7.64634104006127));
#35424=CARTESIAN_POINT('Ctrl Pts',(-64.4450065869384,-15.4043894403332,
8.23435456655423));
#35425=CARTESIAN_POINT('Ctrl Pts',(-64.5227251994293,-14.9553323969431,
8.69708154291655));
#35426=CARTESIAN_POINT('Ctrl Pts',(-64.5498246710713,-14.6951885590369,
9.35164270965619));
#35427=CARTESIAN_POINT('Ctrl Pts',(-64.511567991272,-14.6789571988966,10.0021294030496));
#35428=CARTESIAN_POINT('Ctrl Pts',(-64.7775781358098,-14.7480685208434,
10.001505123818));
#35429=CARTESIAN_POINT('Ctrl Pts',(-64.8206186125989,-14.7649679121881,
9.27681483601613));
#35430=CARTESIAN_POINT('Ctrl Pts',(-64.7795300848962,-15.0958410226862,
8.54799381140172));
#35431=CARTESIAN_POINT('Ctrl Pts',(-64.6812188924137,-15.640272025487,8.07917134860842));
#35432=CARTESIAN_POINT('Ctrl Pts',(-64.5697220196357,-16.2577231286921,
7.54746954365997));
#35433=CARTESIAN_POINT('Ctrl Pts',(-64.3846235013878,-17.1498593123113,
7.35018631295078));
#35434=CARTESIAN_POINT('Ctrl Pts',(-64.2306567779802,-17.9258100558557,
7.5750838862455));
#35435=CARTESIAN_POINT('Ctrl Pts',(-64.0766900545726,-18.7017607994001,
7.79998145954022));
#35436=CARTESIAN_POINT('Ctrl Pts',(-63.9538551260053,-19.3615261028695,
8.44705983683885));
#35437=CARTESIAN_POINT('Ctrl Pts',(-63.9391872263039,-19.6176065589078,
9.22846362604872));
#35438=CARTESIAN_POINT('Ctrl Pts',(-63.9245193266025,-19.873687014946,10.0098674152586));
#35439=CARTESIAN_POINT('Ctrl Pts',(-64.018018455767,-19.7260826235529,10.9255966163797));
#35440=CARTESIAN_POINT('Ctrl Pts',(-64.2004827799559,-19.2464556042238,
11.5682854345733));
#35441=CARTESIAN_POINT('Ctrl Pts',(-64.3829471041447,-18.7668285848947,
12.2109742527669));
#35442=CARTESIAN_POINT('Ctrl Pts',(-64.6543766233579,-17.9551789376295,
12.580622688033));
#35443=CARTESIAN_POINT('Ctrl Pts',(-64.9164164596568,-17.1785720640671,
12.5127911771403));
#35444=CARTESIAN_POINT('Ctrl Pts',(-65.1784562959558,-16.4019651905047,
12.4449596662476));
#35445=CARTESIAN_POINT('Ctrl Pts',(-65.4311064493405,-15.6604010906451,
11.939648209196));
#35446=CARTESIAN_POINT('Ctrl Pts',(-65.5843661188993,-15.2897673262127,
11.2216465877781));
#35447=CARTESIAN_POINT('Ctrl Pts',(-65.6632851643038,-15.0989143577319,
10.8519211229881));
#35448=CARTESIAN_POINT('Ctrl Pts',(-65.7158498370977,-15.0064172468355,
10.4257987515069));
#35449=CARTESIAN_POINT('Ctrl Pts',(-65.7418454548455,-15.0130771992805,
9.99981028982562));
#35450=CARTESIAN_POINT('Origin',(-63.7511045350785,-17.0820569767664,10.));
#35451=CARTESIAN_POINT('',(-66.7095652904141,-15.2652009106025,9.99881345470568));
#35452=CARTESIAN_POINT('',(-66.4442667934687,-15.1934336836835,9.99943462192771));
#35453=CARTESIAN_POINT('',(-64.4026814811241,-14.6503387090836,10.));
#35454=CARTESIAN_POINT('Ctrl Pts',(-66.4442667934687,-15.1934336836835,
9.99943462192771));
#35455=CARTESIAN_POINT('Ctrl Pts',(-66.3950965524831,-15.1827995799555,
10.7909504295074));
#35456=CARTESIAN_POINT('Ctrl Pts',(-66.242026625676,-15.5599243826037,11.584629422138));
#35457=CARTESIAN_POINT('Ctrl Pts',(-66.0272275066145,-16.1674256670557,
12.0468004663335));
#35458=CARTESIAN_POINT('Ctrl Pts',(-65.8036660249293,-16.7997089272067,
12.5278249876807));
#35459=CARTESIAN_POINT('Ctrl Pts',(-65.5132363542999,-17.6815476659074,
12.6497433013673));
#35460=CARTESIAN_POINT('Ctrl Pts',(-65.2633677075891,-18.4120106025368,
12.3579626123136));
#35461=CARTESIAN_POINT('Ctrl Pts',(-65.0134990608783,-19.1424735391663,
12.0661819232598));
#35462=CARTESIAN_POINT('Ctrl Pts',(-64.8041914380861,-19.7215606737245,
11.3607022314657));
#35463=CARTESIAN_POINT('Ctrl Pts',(-64.7065491918251,-19.8839069496222,
10.5574238638961));
#35464=CARTESIAN_POINT('Ctrl Pts',(-64.608906945564,-20.0462532255198,9.75414549632649));
#35465=CARTESIAN_POINT('Ctrl Pts',(-64.6229300758342,-19.7918586427568,
8.8530684529815));
#35466=CARTESIAN_POINT('Ctrl Pts',(-64.7197196907436,-19.2285753341561,
8.25767771891577));
#35467=CARTESIAN_POINT('Ctrl Pts',(-64.816509305653,-18.6652920255555,7.66228698485004));
#35468=CARTESIAN_POINT('Ctrl Pts',(-64.9960654052017,-17.7931199911172,
7.37258256006359));
#35469=CARTESIAN_POINT('Ctrl Pts',(-65.1553666185043,-16.9965402212507,
7.51828854147113));
#35470=CARTESIAN_POINT('Ctrl Pts',(-65.314667831807,-16.1999604513842,7.66399452287867));
#35471=CARTESIAN_POINT('Ctrl Pts',(-65.4537141588636,-15.4789729460894,
8.24511091048021));
#35472=CARTESIAN_POINT('Ctrl Pts',(-65.4876237233567,-15.150361180425,9.00142492811759));
#35473=CARTESIAN_POINT('Ctrl Pts',(-65.5016305260266,-15.0146236613656,
9.31383062721468));
#35474=CARTESIAN_POINT('Ctrl Pts',(-65.4976987431426,-14.9458338550092,
9.65612879778042));
#35475=CARTESIAN_POINT('Ctrl Pts',(-65.4764820235065,-14.9415523108175,
9.99892236192921));
#35476=CARTESIAN_POINT('Ctrl Pts',(-65.7418454548455,-15.0130771992805,
9.99981028982562));
#35477=CARTESIAN_POINT('Ctrl Pts',(-65.7663329589547,-15.0193507802528,
9.59853518618498));
#35478=CARTESIAN_POINT('Ctrl Pts',(-65.7672447483349,-15.113610126419,9.19737890571051));
#35479=CARTESIAN_POINT('Ctrl Pts',(-65.7444013786921,-15.2965249330005,
8.84359325274577));
#35480=CARTESIAN_POINT('Ctrl Pts',(-65.6973077831932,-15.6736197332258,
8.11423332491567));
#35481=CARTESIAN_POINT('Ctrl Pts',(-65.5492514064625,-16.4275127626816,
7.58620525503978));
#35482=CARTESIAN_POINT('Ctrl Pts',(-65.3884873478829,-17.2288315064441,
7.49440429239119));
#35483=CARTESIAN_POINT('Ctrl Pts',(-65.2277232893032,-18.0301502502066,
7.4026033297426));
#35484=CARTESIAN_POINT('Ctrl Pts',(-65.0542515488747,-18.8788947082756,
7.74702947432132));
#35485=CARTESIAN_POINT('Ctrl Pts',(-64.9676333413309,-19.4034973688022,
8.3744636726991));
#35486=CARTESIAN_POINT('Ctrl Pts',(-64.881015133787,-19.9281000293287,9.00189787107686));
#35487=CARTESIAN_POINT('Ctrl Pts',(-64.8812504591278,-20.1285608923127,
9.91234012325367));
#35488=CARTESIAN_POINT('Ctrl Pts',(-64.9906262726287,-19.9217039083206,
10.7007759738109));
#35489=CARTESIAN_POINT('Ctrl Pts',(-65.1000020861296,-19.7148469243284,
11.4892118243682));
#35490=CARTESIAN_POINT('Ctrl Pts',(-65.3185183877905,-19.1006720933601,
12.155641273306));
#35491=CARTESIAN_POINT('Ctrl Pts',(-65.5713589268317,-18.3583974645574,
12.4036017192681));
#35492=CARTESIAN_POINT('Ctrl Pts',(-65.824199465873,-17.6161228357546,12.6515621652302));
#35493=CARTESIAN_POINT('Ctrl Pts',(-66.1113642422946,-16.7457484091175,
12.4810536082167));
#35494=CARTESIAN_POINT('Ctrl Pts',(-66.3274985456644,-16.1404633167953,
11.9679250313909));
#35495=CARTESIAN_POINT('Ctrl Pts',(-66.5245294039924,-15.5886775085548,
11.5001503082288));
#35496=CARTESIAN_POINT('Ctrl Pts',(-66.662531210899,-15.2571911193414,10.7476451883997));
#35497=CARTESIAN_POINT('Ctrl Pts',(-66.7095652904141,-15.2652009106025,
9.99881345470568));
#35498=CARTESIAN_POINT('Origin',(-63.7511045350785,-17.0820569767664,10.));
#35499=CARTESIAN_POINT('',(-67.6742507328171,-15.5286491313886,10.0019962882658));
#35500=CARTESIAN_POINT('',(-67.4086397233445,-15.458048217099,10.0018117506529));
#35501=CARTESIAN_POINT('',(-64.4026814811241,-14.6503387090836,10.));
#35502=CARTESIAN_POINT('',(-67.0040126136404,-20.2598690437802,11.1728309286204));
#35503=CARTESIAN_POINT('Ctrl Pts',(-67.6742507328171,-15.5286491313886,
10.0019962882658));
#35504=CARTESIAN_POINT('Ctrl Pts',(-67.707951193009,-15.5421457071955,9.43113200366998));
#35505=CARTESIAN_POINT('Ctrl Pts',(-67.6927226550026,-15.7382477902415,
8.85763821511506));
#35506=CARTESIAN_POINT('Ctrl Pts',(-67.6352118327672,-16.0921495062904,
8.4158421648759));
#35507=CARTESIAN_POINT('Ctrl Pts',(-67.5520689427973,-16.6037821050583,
7.77714150009027));
#35508=CARTESIAN_POINT('Ctrl Pts',(-67.3805551035977,-17.4452195762649,
7.41369214583768));
#35509=CARTESIAN_POINT('Ctrl Pts',(-67.2193238791373,-18.2482818068298,
7.4886153741189));
#35510=CARTESIAN_POINT('Ctrl Pts',(-67.0580926546769,-19.0513440373947,
7.56353860240013));
#35511=CARTESIAN_POINT('Ctrl Pts',(-66.9071440449559,-19.8160310273179,
8.07683441321518));
#35512=CARTESIAN_POINT('Ctrl Pts',(-66.8561932299011,-20.2075211669015,
8.79681637620211));
#35513=CARTESIAN_POINT('Ctrl Pts',(-66.8052424148464,-20.5990113064852,
9.51679833918905));
#35514=CARTESIAN_POINT('Ctrl Pts',(-66.854289394458,-20.6173045957294,10.4434664543479));
#35515=CARTESIAN_POINT('Ctrl Pts',(-67.0040126136403,-20.2598690437802,
11.1728309286203));
#35516=CARTESIAN_POINT('',(-68.0323660008166,-16.4802525979519,11.8670505687061));
#35517=CARTESIAN_POINT('Ctrl Pts',(-68.0322473001841,-16.4806955947434,
11.8669181223572));
#35518=CARTESIAN_POINT('Ctrl Pts',(-67.9835336336721,-16.6817854205938,
12.0540417240897));
#35519=CARTESIAN_POINT('Ctrl Pts',(-67.9238765324049,-16.9239334961962,
12.2143044024353));
#35520=CARTESIAN_POINT('Ctrl Pts',(-67.7816176378542,-17.4856657502708,
12.4543153408643));
#35521=CARTESIAN_POINT('Ctrl Pts',(-67.6966288605656,-17.8119729521746,
12.5175));
#35522=CARTESIAN_POINT('Ctrl Pts',(-67.5329868199039,-18.4226933621783,
12.5175));
#35523=CARTESIAN_POINT('Ctrl Pts',(-67.4434356591205,-18.747778077109,12.4543153408643));
#35524=CARTESIAN_POINT('Ctrl Pts',(-67.2746559299571,-19.3446857260753,
12.1973867613172));
#35525=CARTESIAN_POINT('Ctrl Pts',(-67.1955448337828,-19.6165425195547,
12.0036443501621));
#35526=CARTESIAN_POINT('Ctrl Pts',(-67.0834304248293,-19.9960747381915,
11.6080270340043));
#35527=CARTESIAN_POINT('Ctrl Pts',(-67.0387983068925,-20.1448248140074,
11.4009948671632));
#35528=CARTESIAN_POINT('Ctrl Pts',(-67.0040126136404,-20.2598690437802,
11.1728309286204));
#35529=CARTESIAN_POINT('Ctrl Pts',(-68.0330516124712,-16.4776938604227,
11.8678155752478));
#35530=CARTESIAN_POINT('Ctrl Pts',(-67.8522271893252,-16.9785524830602,
12.3404055365588));
#35531=CARTESIAN_POINT('Ctrl Pts',(-67.6166367512168,-17.6838006560658,
12.5855412104358));
#35532=CARTESIAN_POINT('Ctrl Pts',(-67.3907294446844,-18.3529108900533,
12.5051234941037));
#35533=CARTESIAN_POINT('Ctrl Pts',(-67.1283727946319,-19.1299796896392,
12.4117306641612));
#35534=CARTESIAN_POINT('Ctrl Pts',(-66.8790760319581,-19.8583083259863,
11.8792556448929));
#35535=CARTESIAN_POINT('Ctrl Pts',(-66.7317311985187,-20.2061471825014,
11.1455779206957));
#35536=CARTESIAN_POINT('Ctrl Pts',(-66.5843863650792,-20.5539860390166,
10.4119001964985));
#35537=CARTESIAN_POINT('Ctrl Pts',(-66.5389934608741,-20.5213351156998,
9.47701976737246));
#35538=CARTESIAN_POINT('Ctrl Pts',(-66.5933174195301,-20.1165357938134,
8.7598296178153));
#35539=CARTESIAN_POINT('Ctrl Pts',(-66.6476413781862,-19.7117364719269,
8.04263946825813));
#35540=CARTESIAN_POINT('Ctrl Pts',(-66.8016821997036,-18.9347887514708,
7.54313959826985));
#35541=CARTESIAN_POINT('Ctrl Pts',(-66.9638149498407,-18.1276415422745,
7.48486270274577));
#35542=CARTESIAN_POINT('Ctrl Pts',(-67.1259476999778,-17.3204943330783,
7.42658580722168));
#35543=CARTESIAN_POINT('Ctrl Pts',(-67.2961723787346,-16.4831476351418,
7.80953188616179));
#35544=CARTESIAN_POINT('Ctrl Pts',(-67.3756602454435,-15.9844353298854,
8.46229096311843));
#35545=CARTESIAN_POINT('Ctrl Pts',(-67.4285455390928,-15.6526293851286,
8.89658813193769));
#35546=CARTESIAN_POINT('Ctrl Pts',(-67.4412654718215,-15.4707226080323,
9.45032013874425));
#35547=CARTESIAN_POINT('Ctrl Pts',(-67.4086397233445,-15.458048217099,10.0018117506529));
#35548=CARTESIAN_POINT('Origin',(17.0820569767664,-63.7511045350785,10.));
#35549=CARTESIAN_POINT('',(13.7189801527801,-60.9122168113323,9.99965378812953));
#35550=CARTESIAN_POINT('',(13.6458118873637,-60.6472937215209,9.99664393250996));
#35551=CARTESIAN_POINT('',(14.6503387090836,-64.4026814811241,10.));
#35552=CARTESIAN_POINT('',(14.1985145724514,-60.3826426720153,11.6359872033748));
#35553=CARTESIAN_POINT('Ctrl Pts',(13.6458118873637,-60.6472937215209,9.99664393250996));
#35554=CARTESIAN_POINT('Ctrl Pts',(13.6410407802454,-60.6097205320263,10.5892058593235));
#35555=CARTESIAN_POINT('Ctrl Pts',(13.8356159531907,-60.5187326677745,11.1848035603042));
#35556=CARTESIAN_POINT('Ctrl Pts',(14.1985145724514,-60.3826426720153,11.6359872033748));
#35557=CARTESIAN_POINT('',(17.8984305821305,-59.3912531651587,11.6380816927068));
#35558=CARTESIAN_POINT('Origin',(16.0467807963563,-59.8874012299222,10.));
#35559=CARTESIAN_POINT('Ctrl Pts',(17.8984546702663,-59.3912467107622,11.6380966037224));
#35560=CARTESIAN_POINT('Ctrl Pts',(17.4212611177617,-59.5701794123023,12.2270179049201));
#35561=CARTESIAN_POINT('Ctrl Pts',(16.6595160069781,-59.8253574740882,12.5674221981559));
#35562=CARTESIAN_POINT('Ctrl Pts',(15.9233267283635,-60.0736878712826,12.5157167035403));
#35563=CARTESIAN_POINT('Ctrl Pts',(15.1456267338053,-60.3360206084696,12.461095746608));
#35564=CARTESIAN_POINT('Ctrl Pts',(14.3964458015819,-60.5907116859351,11.9688993897473));
#35565=CARTESIAN_POINT('Ctrl Pts',(14.0146059447131,-60.7469740189126,11.2575578209418));
#35566=CARTESIAN_POINT('Ctrl Pts',(13.8116368860468,-60.8300361143405,10.8794403300266));
#35567=CARTESIAN_POINT('Ctrl Pts',(13.7124604894775,-60.8852870497794,10.4394030962359));
#35568=CARTESIAN_POINT('Ctrl Pts',(13.7189801527801,-60.9122168113323,9.99965378812953));
#35569=CARTESIAN_POINT('Origin',(17.0820569767664,-63.7511045350785,10.));
#35570=CARTESIAN_POINT('',(13.9708704146993,-61.8799991994799,9.99901528063934));
#35571=CARTESIAN_POINT('',(13.899975087973,-61.614467077582,10.0012573013838));
#35572=CARTESIAN_POINT('',(14.6503387090836,-64.4026814811241,10.));
#35573=CARTESIAN_POINT('Ctrl Pts',(13.899975087973,-61.614467077582,10.0012573013838));
#35574=CARTESIAN_POINT('Ctrl Pts',(13.8982899610888,-61.6099667912195,10.0766544396888));
#35575=CARTESIAN_POINT('Ctrl Pts',(13.900043500223,-61.6045451170744,10.1520128061815));
#35576=CARTESIAN_POINT('Ctrl Pts',(13.9053569552699,-61.5981695663354,10.2270376921985));
#35577=CARTESIAN_POINT('Ctrl Pts',(13.9634527171371,-61.5284611611193,11.047337830936));
#35578=CARTESIAN_POINT('Ctrl Pts',(14.4471220222725,-61.3447206686646,11.8277717281245));
#35579=CARTESIAN_POINT('Ctrl Pts',(15.1337367424348,-61.1066011161457,12.2189611289229));
#35580=CARTESIAN_POINT('Ctrl Pts',(15.8203514625971,-60.8684815636268,12.6101505297212));
#35581=CARTESIAN_POINT('Ctrl Pts',(16.7099115977863,-60.5759829510439,12.6120954341293));
#35582=CARTESIAN_POINT('Ctrl Pts',(17.3980067606845,-60.3374667150895,12.2237523563129));
#35583=CARTESIAN_POINT('Ctrl Pts',(18.0861019235826,-60.0989504791351,11.8354092784964));
#35584=CARTESIAN_POINT('Ctrl Pts',(18.5727321141896,-59.9144166198093,11.0567782184554));
#35585=CARTESIAN_POINT('Ctrl Pts',(18.6339764021913,-59.8438645695582,10.2368654679638));
#35586=CARTESIAN_POINT('Ctrl Pts',(18.6952206901929,-59.7733125193071,9.41695271747212));
#35587=CARTESIAN_POINT('Ctrl Pts',(18.3310790755891,-59.8167422781306,8.55575827652985));
#35588=CARTESIAN_POINT('Ctrl Pts',(17.6984585141966,-59.932110753931,8.03819621078674));
#35589=CARTESIAN_POINT('Ctrl Pts',(17.0658379528042,-60.0474792297314,7.52063414504363));
#35590=CARTESIAN_POINT('Ctrl Pts',(16.1647384446231,-60.2347864225085,7.34670445449967));
#35591=CARTESIAN_POINT('Ctrl Pts',(15.392769597115,-60.3874931590403,7.59575134544315));
#35592=CARTESIAN_POINT('Ctrl Pts',(14.6208007496069,-60.540199895572,7.84479823638662));
#35593=CARTESIAN_POINT('Ctrl Pts',(13.9779625627717,-60.6583061758583,8.51682170881753));
#35594=CARTESIAN_POINT('Ctrl Pts',(13.7459615817213,-60.6663289586339,9.30743209219173));
#35595=CARTESIAN_POINT('Ctrl Pts',(13.6804424696227,-60.6685946628634,9.5307073994776));
#35596=CARTESIAN_POINT('Ctrl Pts',(13.6476895615158,-60.6620806891943,9.76344057197141));
#35597=CARTESIAN_POINT('Ctrl Pts',(13.6458118873637,-60.6472937215209,9.99664393250996));
#35598=CARTESIAN_POINT('Ctrl Pts',(13.7189801527801,-60.9122168113323,9.99965378812953));
#35599=CARTESIAN_POINT('Ctrl Pts',(13.7247257446778,-60.9359492362449,9.61211536100744));
#35600=CARTESIAN_POINT('Ctrl Pts',(13.8125590225005,-60.9376863320054,9.22480054821092));
#35601=CARTESIAN_POINT('Ctrl Pts',(13.9837827281426,-60.9170790299751,8.88028612326233));
#35602=CARTESIAN_POINT('Ctrl Pts',(14.3492981499551,-60.8730881195708,8.14484277513865));
#35603=CARTESIAN_POINT('Ctrl Pts',(15.0948277750944,-60.7272727102727,7.60444285964159));
#35604=CARTESIAN_POINT('Ctrl Pts',(15.8946095193187,-60.5669204894781,7.49935843056475));
#35605=CARTESIAN_POINT('Ctrl Pts',(16.6943912635429,-60.4065682686835,7.3942740014879));
#35606=CARTESIAN_POINT('Ctrl Pts',(17.548425126852,-60.2316792363924,7.72450505883126));
#35607=CARTESIAN_POINT('Ctrl Pts',(18.0828447847105,-60.1424305723414,8.3432095629449));
#35608=CARTESIAN_POINT('Ctrl Pts',(18.6172644425689,-60.0531819082903,8.96191406705854));
#35609=CARTESIAN_POINT('Ctrl Pts',(18.8320698949766,-60.0495736124793,9.86909201794247));
#35610=CARTESIAN_POINT('Ctrl Pts',(18.6376771842086,-60.1556096340356,10.6611508664112));
#35611=CARTESIAN_POINT('Ctrl Pts',(18.4432844734406,-60.2616456555918,11.4532097148799));
#35612=CARTESIAN_POINT('Ctrl Pts',(17.8396935994969,-60.4773259945153,12.1301494609334));
#35613=CARTESIAN_POINT('Ctrl Pts',(17.1014273477894,-60.7290924921509,12.3908459426517));
#35614=CARTESIAN_POINT('Ctrl Pts',(16.3631610960819,-60.9808589897865,12.6515424243699));
#35615=CARTESIAN_POINT('Ctrl Pts',(15.4902194666106,-61.2687116461343,12.4959956417529));
#35616=CARTESIAN_POINT('Ctrl Pts',(14.8769273589396,-61.4869914228006,11.9933937214367));
#35617=CARTESIAN_POINT('Ctrl Pts',(14.3076501674883,-61.6896056365772,11.52686267361));
#35618=CARTESIAN_POINT('Ctrl Pts',(13.9620906745725,-61.8322748736988,10.7613040129743));
#35619=CARTESIAN_POINT('Ctrl Pts',(13.9708704146993,-61.8799991994799,9.99901528063934));
#35620=CARTESIAN_POINT('Origin',(17.0820569767664,-63.7511045350785,10.));
#35621=CARTESIAN_POINT('',(14.2348698103755,-62.8445369550162,10.0018466754434));
#35622=CARTESIAN_POINT('',(14.1654859215485,-62.5785998445538,10.0004462653844));
#35623=CARTESIAN_POINT('',(14.6503387090836,-64.4026814811241,10.));
#35624=CARTESIAN_POINT('Ctrl Pts',(14.1654859215485,-62.5785998445538,10.0004462653844));
#35625=CARTESIAN_POINT('Ctrl Pts',(14.1585827534688,-62.5552558244195,10.386770248634));
#35626=CARTESIAN_POINT('Ctrl Pts',(14.2332491130212,-62.5100553152291,10.7728367424032));
#35627=CARTESIAN_POINT('Ctrl Pts',(14.3908772813227,-62.4426252563818,11.1164878478952));
#35628=CARTESIAN_POINT('Ctrl Pts',(14.7296226663468,-62.2977170112848,11.8549994178656));
#35629=CARTESIAN_POINT('Ctrl Pts',(15.4515079046906,-62.0501467519025,12.397625364221));
#35630=CARTESIAN_POINT('Ctrl Pts',(16.2272258855742,-61.7881520526304,12.501389418797));
#35631=CARTESIAN_POINT('Ctrl Pts',(17.0029438664577,-61.5261573533583,12.605153473373));
#35632=CARTESIAN_POINT('Ctrl Pts',(17.832494589881,-61.2497382141963,12.2700556361696));
#35633=CARTESIAN_POINT('Ctrl Pts',(18.3383599455201,-61.0600503079339,11.6461438143239));
#35634=CARTESIAN_POINT('Ctrl Pts',(18.8442253011592,-60.8703624016714,11.0222319924783));
#35635=CARTESIAN_POINT('Ctrl Pts',(19.0264052890141,-60.7674057283086,10.1095061859904));
#35636=CARTESIAN_POINT('Ctrl Pts',(18.7972629292321,-60.7746625458238,9.3166725220468));
#35637=CARTESIAN_POINT('Ctrl Pts',(18.5681205694502,-60.7819193633391,8.52383885810324));
#35638=CARTESIAN_POINT('Ctrl Pts',(17.9276558620313,-60.8993896717325,7.85089733670406));
#35639=CARTESIAN_POINT('Ctrl Pts',(17.1565944419206,-61.0518532638259,7.59916807226838));
#35640=CARTESIAN_POINT('Ctrl Pts',(16.3855330218099,-61.2043168559193,7.3474388078327));
#35641=CARTESIAN_POINT('Ctrl Pts',(15.4838748890073,-61.3917737317127,7.51692180036052));
#35642=CARTESIAN_POINT('Ctrl Pts',(14.8493069319055,-61.5076640106208,8.0317464867676));
#35643=CARTESIAN_POINT('Ctrl Pts',(14.2727767422054,-61.6129549313732,8.49948515966275));
#35644=CARTESIAN_POINT('Ctrl Pts',(13.9167146450877,-61.6591716047613,9.25228420341938));
#35645=CARTESIAN_POINT('Ctrl Pts',(13.899975087973,-61.614467077582,10.0012573013838));
#35646=CARTESIAN_POINT('Ctrl Pts',(13.9708704146993,-61.8799991994799,9.99901528063934));
#35647=CARTESIAN_POINT('Ctrl Pts',(13.971549239588,-61.8836891105328,9.94007725327275));
#35648=CARTESIAN_POINT('Ctrl Pts',(13.9743462862715,-61.8868114457664,9.88115877337014));
#35649=CARTESIAN_POINT('Ctrl Pts',(13.9793219277933,-61.8893500282724,9.8223995623229));
#35650=CARTESIAN_POINT('Ctrl Pts',(14.0486511901885,-61.9247219600932,9.00366438154045));
#35651=CARTESIAN_POINT('Ctrl Pts',(14.5409523008495,-61.8467589267501,8.21585107799077));
#35652=CARTESIAN_POINT('Ctrl Pts',(15.2432213925389,-61.712535142454,7.80941972573595));
#35653=CARTESIAN_POINT('Ctrl Pts',(15.9454904842283,-61.578311358158,7.40298837348113));
#35654=CARTESIAN_POINT('Ctrl Pts',(16.8577275569459,-61.387826822909,7.37793897252116));
#35655=CARTESIAN_POINT('Ctrl Pts',(17.5801209048417,-61.2482107604141,7.74541574302326));
#35656=CARTESIAN_POINT('Ctrl Pts',(18.3025142527375,-61.1085946979193,8.11289251352536));
#35657=CARTESIAN_POINT('Ctrl Pts',(18.8350638758114,-61.0198471081786,8.87289545548955));
#35658=CARTESIAN_POINT('Ctrl Pts',(18.9468623871525,-61.0438394390412,9.68733378926645));
#35659=CARTESIAN_POINT('Ctrl Pts',(19.0586608984936,-61.0678317699038,10.5017721230433));
#35660=CARTESIAN_POINT('Ctrl Pts',(18.749708298102,-61.2045640213696,11.3706458486329));
#35661=CARTESIAN_POINT('Ctrl Pts',(18.1634433884682,-61.4156018821482,11.9074332417685));
#35662=CARTESIAN_POINT('Ctrl Pts',(17.5771784788343,-61.6266397429267,12.444220634904));
#35663=CARTESIAN_POINT('Ctrl Pts',(16.7136012599583,-61.9119832130179,12.6489216955856));
#35664=CARTESIAN_POINT('Ctrl Pts',(15.9628772265394,-62.1670877632026,12.4304742338454));
#35665=CARTESIAN_POINT('Ctrl Pts',(15.2121531931205,-62.4221923133873,12.2120267721052));
#35666=CARTESIAN_POINT('Ctrl Pts',(14.5742823451589,-62.6470579436654,11.5704307879434));
#35667=CARTESIAN_POINT('Ctrl Pts',(14.3390239366156,-62.7640438959386,10.7911028658273));
#35668=CARTESIAN_POINT('Ctrl Pts',(14.2625865983512,-62.8020535673526,10.5378929917551));
#35669=CARTESIAN_POINT('Ctrl Pts',(14.2286511253629,-62.828674898289,10.2701434172215));
#35670=CARTESIAN_POINT('Ctrl Pts',(14.2348698103755,-62.8445369550162,10.0018466754434));
#35671=CARTESIAN_POINT('Origin',(17.0820569767664,-63.7511045350785,10.));
#35672=CARTESIAN_POINT('',(14.4927485186002,-63.8107147438123,9.99793352624086));
#35673=CARTESIAN_POINT('',(14.4189472139579,-63.5459612763503,9.99811000378502));
#35674=CARTESIAN_POINT('',(14.6503387090836,-64.4026814811241,10.));
#35675=CARTESIAN_POINT('Ctrl Pts',(14.4189472139579,-63.5459612763503,9.99811000378502));
#35676=CARTESIAN_POINT('Ctrl Pts',(14.4131993125783,-63.5020657997403,10.6909216248416));
#35677=CARTESIAN_POINT('Ctrl Pts',(14.6895870615306,-63.3825723034678,11.3881278716996));
#35678=CARTESIAN_POINT('Ctrl Pts',(15.1696780211856,-63.2084966963919,11.8560065223221));
#35679=CARTESIAN_POINT('Ctrl Pts',(15.7417608055527,-63.0010658835769,12.4135369565263));
#35680=CARTESIAN_POINT('Ctrl Pts',(16.6030903983924,-62.7161316220184,12.6454354329572));
#35681=CARTESIAN_POINT('Ctrl Pts',(17.3619190322645,-62.4586624096387,12.4478622804133));
#35682=CARTESIAN_POINT('Ctrl Pts',(18.1207476661366,-62.201193197259,12.2502891278695));
#35683=CARTESIAN_POINT('Ctrl Pts',(18.7770753410411,-61.9711890340581,11.6232443463508));
#35684=CARTESIAN_POINT('Ctrl Pts',(19.0309502087539,-61.8490217755358,10.8475065234706));
#35685=CARTESIAN_POINT('Ctrl Pts',(19.2848250764668,-61.7268545170136,10.0717687005904));
#35686=CARTESIAN_POINT('Ctrl Pts',(19.136247136988,-61.7125241631699,9.14733783634868));
#35687=CARTESIAN_POINT('Ctrl Pts',(18.6456858472655,-61.789827971849,8.48815640829363));
#35688=CARTESIAN_POINT('Ctrl Pts',(18.1551245575431,-61.867131780528,7.82897498023858));
#35689=CARTESIAN_POINT('Ctrl Pts',(17.3225799175771,-62.0360697517297,7.43504298837021));
#35690=CARTESIAN_POINT('Ctrl Pts',(16.5147885234738,-62.1983751106924,7.48275547481141));
#35691=CARTESIAN_POINT('Ctrl Pts',(15.7069971293705,-62.3606804696551,7.53046796125262));
#35692=CARTESIAN_POINT('Ctrl Pts',(14.9239589811301,-62.5163532163788,8.0198249260034));
#35693=CARTESIAN_POINT('Ctrl Pts',(14.5102426728621,-62.5730664743348,8.73170200517146));
#35694=CARTESIAN_POINT('Ctrl Pts',(14.2890407035395,-62.6033893890854,9.11232178902005));
#35695=CARTESIAN_POINT('Ctrl Pts',(14.1734177690262,-62.6054224867212,9.55655400073801));
#35696=CARTESIAN_POINT('Ctrl Pts',(14.1654859215485,-62.5785998445538,10.0004462653844));
#35697=CARTESIAN_POINT('Ctrl Pts',(14.2348698103755,-62.8445369550162,10.0018466754434));
#35698=CARTESIAN_POINT('Ctrl Pts',(14.2477909590166,-62.8774950470096,9.44438121878225));
#35699=CARTESIAN_POINT('Ctrl Pts',(14.4340668190784,-62.8640028840737,8.88455351560674));
#35700=CARTESIAN_POINT('Ctrl Pts',(14.7726377170273,-62.8097033887247,8.44788099502246));
#35701=CARTESIAN_POINT('Ctrl Pts',(15.274155875107,-62.7292706549691,7.80104690640403));
#35702=CARTESIAN_POINT('Ctrl Pts',(16.1098381603914,-62.5592989131896,7.42443858923755));
#35703=CARTESIAN_POINT('Ctrl Pts',(16.9139278054309,-62.3977923938505,7.48559176785145));
#35704=CARTESIAN_POINT('Ctrl Pts',(17.7180174504703,-62.2362858745114,7.54674494646536));
#35705=CARTESIAN_POINT('Ctrl Pts',(18.4905144552649,-62.0832445776126,8.04565962085964));
#35706=CARTESIAN_POINT('Ctrl Pts',(18.8937702597924,-62.0291411621378,8.76039160250505));
#35707=CARTESIAN_POINT('Ctrl Pts',(19.2970260643199,-61.9750377466629,9.47512358415046));
#35708=CARTESIAN_POINT('Ctrl Pts',(19.3310406685804,-62.0198722126119,10.405672873047));
#35709=CARTESIAN_POINT('Ctrl Pts',(18.9866823611345,-62.1660913946905,11.1380809107439));
#35710=CARTESIAN_POINT('Ctrl Pts',(18.6423240536885,-62.312310576769,11.8704889484408));
#35711=CARTESIAN_POINT('Ctrl Pts',(17.9195928345363,-62.5599144749771,12.4047557349382));
#35712=CARTESIAN_POINT('Ctrl Pts',(17.1459983851496,-62.8211471346509,12.5032105584454));
#35713=CARTESIAN_POINT('Ctrl Pts',(16.372403935763,-63.0823797943246,12.6016653819527));
#35714=CARTESIAN_POINT('Ctrl Pts',(15.547946256142,-63.3572412154642,12.2643082424699));
#35715=CARTESIAN_POINT('Ctrl Pts',(15.0453884512907,-63.5458498251155,11.6412138093997));
#35716=CARTESIAN_POINT('Ctrl Pts',(14.6827506455303,-63.6819468306564,11.1915986689942));
#35717=CARTESIAN_POINT('Ctrl Pts',(14.4877209077723,-63.7731333897311,10.5932047327949));
#35718=CARTESIAN_POINT('Ctrl Pts',(14.4927485186002,-63.8107147438123,9.99793352624086));
#35719=CARTESIAN_POINT('Origin',(17.0820569767664,-63.7511045350785,10.));
#35720=CARTESIAN_POINT('',(14.7480685208434,-64.7775781358098,10.001505123818));
#35721=CARTESIAN_POINT('',(14.6789571988966,-64.511567991272,10.0021294030496));
#35722=CARTESIAN_POINT('',(14.6503387090836,-64.4026814811241,10.));
#35723=CARTESIAN_POINT('Ctrl Pts',(14.6789571988966,-64.511567991272,10.0021294030496));
#35724=CARTESIAN_POINT('Ctrl Pts',(14.6745624451438,-64.5012097288919,10.1782532036583));
#35725=CARTESIAN_POINT('Ctrl Pts',(14.6880487522533,-64.4860602506939,10.354078307347));
#35726=CARTESIAN_POINT('Ctrl Pts',(14.7205078014429,-64.4658270415774,10.5257161206906));
#35727=CARTESIAN_POINT('Ctrl Pts',(14.8728494531258,-64.3708655262953,11.3312723100704));
#35728=CARTESIAN_POINT('Ctrl Pts',(15.4431136830601,-64.1639219936719,12.0445928505661));
#35729=CARTESIAN_POINT('Ctrl Pts',(16.1698862069573,-63.9150421900725,12.3462664892695));
#35730=CARTESIAN_POINT('Ctrl Pts',(16.8966587308544,-63.6661623864731,12.6479401279729));
#35731=CARTESIAN_POINT('Ctrl Pts',(17.7799395487143,-63.3753463118976,12.5379668648842));
#35732=CARTESIAN_POINT('Ctrl Pts',(18.4181515535132,-63.1501962278718,12.0655906176062));
#35733=CARTESIAN_POINT('Ctrl Pts',(19.0563635583122,-62.925046143846,11.5932143703281));
#35734=CARTESIAN_POINT('Ctrl Pts',(19.4495067500502,-62.7655620503699,10.7584351388608));
#35735=CARTESIAN_POINT('Ctrl Pts',(19.4154782471595,-62.7205382674991,9.93505104704534));
#35736=CARTESIAN_POINT('Ctrl Pts',(19.3814497442687,-62.6755144846282,9.11166695522986));
#35737=CARTESIAN_POINT('Ctrl Pts',(18.9202495467492,-62.7449510123626,8.29967800306621));
#35738=CARTESIAN_POINT('Ctrl Pts',(18.2323333520888,-62.8751359084421,7.8626772661126));
#35739=CARTESIAN_POINT('Ctrl Pts',(17.5444171574285,-63.0053208045216,7.425676529159));
#35740=CARTESIAN_POINT('Ctrl Pts',(16.6297849656272,-63.1962540689461,7.36366400741544));
#35741=CARTESIAN_POINT('Ctrl Pts',(15.8919306215938,-63.3398198518216,7.70440771629217));
#35742=CARTESIAN_POINT('Ctrl Pts',(15.1540762775605,-63.4833856346971,8.04515142516891));
#35743=CARTESIAN_POINT('Ctrl Pts',(14.592999781295,-63.5795839360235,8.78865136466594));
#35744=CARTESIAN_POINT('Ctrl Pts',(14.4538795211095,-63.5627194046509,9.60198253040318));
#35745=CARTESIAN_POINT('Ctrl Pts',(14.4315087612499,-63.5600075610921,9.73276747984734));
#35746=CARTESIAN_POINT('Ctrl Pts',(14.4200485884486,-63.5543722345421,9.86535806600957));
#35747=CARTESIAN_POINT('Ctrl Pts',(14.4189472139579,-63.5459612763503,9.99811000378502));
#35748=CARTESIAN_POINT('Ctrl Pts',(14.4927485186002,-63.8107147438123,9.99793352624086));
#35749=CARTESIAN_POINT('Ctrl Pts',(14.494688369579,-63.8252151156581,9.76825436605176));
#35750=CARTESIAN_POINT('Ctrl Pts',(14.5264111861321,-63.8317351659301,9.53904009330709));
#35751=CARTESIAN_POINT('Ctrl Pts',(14.5897808794637,-63.8297754611264,9.31901604644622));
#35752=CARTESIAN_POINT('Ctrl Pts',(14.8173890425694,-63.8227366893229,8.52874444322046));
#35753=CARTESIAN_POINT('Ctrl Pts',(15.4532632988624,-63.7063033475529,7.85703296342649));
#35754=CARTESIAN_POINT('Ctrl Pts',(16.2205322683665,-63.5546628984883,7.60269513736947));
#35755=CARTESIAN_POINT('Ctrl Pts',(16.9878012378705,-63.4030224494237,7.34835731131246));
#35756=CARTESIAN_POINT('Ctrl Pts',(17.8864649205858,-63.2161748930643,7.51139313899238));
#35757=CARTESIAN_POINT('Ctrl Pts',(18.5227490121289,-63.09963173627,8.01927548227225));
#35758=CARTESIAN_POINT('Ctrl Pts',(19.1590331036721,-62.9830885794757,8.52715782555213));
#35759=CARTESIAN_POINT('Ctrl Pts',(19.5329376040431,-62.9368498222464,9.37988668443198));
#35760=CARTESIAN_POINT('Ctrl Pts',(19.4841294236266,-63.0038765864645,10.1981222260487));
#35761=CARTESIAN_POINT('Ctrl Pts',(19.43532124321,-63.0709033506826,11.0163577676654));
#35762=CARTESIAN_POINT('Ctrl Pts',(18.9638003820058,-63.2511956363481,11.800099992019));
#35763=CARTESIAN_POINT('Ctrl Pts',(18.2853245933942,-63.4869413276821,12.2006980454406));
#35764=CARTESIAN_POINT('Ctrl Pts',(17.6068488047826,-63.7226870190161,12.6012960988622));
#35765=CARTESIAN_POINT('Ctrl Pts',(16.7214180887637,-64.0138861160185,12.6187499813517));
#35766=CARTESIAN_POINT('Ctrl Pts',(16.0289196480801,-64.253389165651,12.2452952639449));
#35767=CARTESIAN_POINT('Ctrl Pts',(15.3364212073965,-64.4928922152834,11.8718405465381));
#35768=CARTESIAN_POINT('Ctrl Pts',(14.8368550420482,-64.6806992175459,11.1074772292349));
#35769=CARTESIAN_POINT('Ctrl Pts',(14.7584549707696,-64.7556551050229,10.2922353809895));
#35770=CARTESIAN_POINT('Ctrl Pts',(14.7491833360657,-64.7645194286933,10.195824440425));
#35771=CARTESIAN_POINT('Ctrl Pts',(14.7458019429916,-64.7718054668758,10.0987019353608));
#35772=CARTESIAN_POINT('Ctrl Pts',(14.7480685208434,-64.7775781358098,10.001505123818));
#35773=CARTESIAN_POINT('Origin',(17.0820569767664,-63.7511045350785,10.));
#35774=CARTESIAN_POINT('',(15.0130771992805,-65.7418454548454,9.99981028982554));
#35775=CARTESIAN_POINT('',(14.9415523108175,-65.4764820235065,9.9989223619293));
#35776=CARTESIAN_POINT('',(14.6503387090836,-64.4026814811241,10.));
#35777=CARTESIAN_POINT('Ctrl Pts',(14.9415523108175,-65.4764820235065,9.9989223619293));
#35778=CARTESIAN_POINT('Ctrl Pts',(14.9354685130879,-65.4463344353997,10.4860098738008));
#35779=CARTESIAN_POINT('Ctrl Pts',(15.0596306010493,-65.3812875674044,10.9740976137645));
#35780=CARTESIAN_POINT('Ctrl Pts',(15.3070399126418,-65.2832167053679,11.3788468299413));
#35781=CARTESIAN_POINT('Ctrl Pts',(15.7285664365572,-65.1161273209564,12.0684430664547));
#35782=CARTESIAN_POINT('Ctrl Pts',(16.5078555104223,-64.8531757502037,12.5161238918082));
#35783=CARTESIAN_POINT('Ctrl Pts',(17.2898955363443,-64.5894870640691,12.5214264196761));
#35784=CARTESIAN_POINT('Ctrl Pts',(18.0719355622662,-64.3257983779344,12.526728947544));
#35785=CARTESIAN_POINT('Ctrl Pts',(18.856726540245,-64.0613725764177,12.0896531779262));
#35786=CARTESIAN_POINT('Ctrl Pts',(19.2867932233327,-63.8919948632527,11.4059132558295));
#35787=CARTESIAN_POINT('Ctrl Pts',(19.7168599064204,-63.7226171500878,10.7221733337328));
#35788=CARTESIAN_POINT('Ctrl Pts',(19.7922022946168,-63.6482875252747,9.7917692591572));
#35789=CARTESIAN_POINT('Ctrl Pts',(19.4730226094499,-63.6796697714155,9.03131812620868));
#35790=CARTESIAN_POINT('Ctrl Pts',(19.153842924283,-63.7110520175564,8.27086699326015));
#35791=CARTESIAN_POINT('Ctrl Pts',(18.4401411657526,-63.8481461346512,7.68036880193875));
#35792=CARTESIAN_POINT('Ctrl Pts',(17.6454383857665,-64.0069444100312,7.524237313639));
#35793=CARTESIAN_POINT('Ctrl Pts',(16.8507356057803,-64.1657426854112,7.36810582533925));
#35794=CARTESIAN_POINT('Ctrl Pts',(15.9750318043384,-64.3462451190763,7.64634104006116));
#35795=CARTESIAN_POINT('Ctrl Pts',(15.4043894403333,-64.4450065869384,8.23435456655407));
#35796=CARTESIAN_POINT('Ctrl Pts',(14.9553323969432,-64.5227251994293,8.69708154291638));
#35797=CARTESIAN_POINT('Ctrl Pts',(14.6951885590369,-64.5498246710713,9.35164270965608));
#35798=CARTESIAN_POINT('Ctrl Pts',(14.6789571988966,-64.511567991272,10.0021294030496));
#35799=CARTESIAN_POINT('Ctrl Pts',(14.7480685208434,-64.7775781358098,10.001505123818));
#35800=CARTESIAN_POINT('Ctrl Pts',(14.7649679121881,-64.8206186125989,9.276814836016));
#35801=CARTESIAN_POINT('Ctrl Pts',(15.0958410226864,-64.7795300848962,8.54799381140143));
#35802=CARTESIAN_POINT('Ctrl Pts',(15.6402720254873,-64.6812188924137,8.07917134860812));
#35803=CARTESIAN_POINT('Ctrl Pts',(16.2577231286925,-64.5697220196356,7.54746954365978));
#35804=CARTESIAN_POINT('Ctrl Pts',(17.1498593123118,-64.3846235013877,7.35018631295075));
#35805=CARTESIAN_POINT('Ctrl Pts',(17.9258100558561,-64.2306567779801,7.57508388624563));
#35806=CARTESIAN_POINT('Ctrl Pts',(18.7017607994005,-64.0766900545725,7.7999814595405));
#35807=CARTESIAN_POINT('Ctrl Pts',(19.3615261028698,-63.9538551260052,8.44705983683928));
#35808=CARTESIAN_POINT('Ctrl Pts',(19.6176065589079,-63.9391872263039,9.22846362604921));
#35809=CARTESIAN_POINT('Ctrl Pts',(19.873687014946,-63.9245193266025,10.0098674152591));
#35810=CARTESIAN_POINT('Ctrl Pts',(19.7260826235527,-64.0180184557671,10.9255966163802));
#35811=CARTESIAN_POINT('Ctrl Pts',(19.2464556042235,-64.200482779956,11.5682854345737));
#35812=CARTESIAN_POINT('Ctrl Pts',(18.7668285848942,-64.3829471041448,12.2109742527672));
#35813=CARTESIAN_POINT('Ctrl Pts',(17.955178937629,-64.654376623358,12.5806226880331));
#35814=CARTESIAN_POINT('Ctrl Pts',(17.1785720640666,-64.9164164596569,12.5127911771402));
#35815=CARTESIAN_POINT('Ctrl Pts',(16.4019651905042,-65.1784562959559,12.4449596662474));
#35816=CARTESIAN_POINT('Ctrl Pts',(15.6604010906447,-65.4311064493406,11.9396482091957));
#35817=CARTESIAN_POINT('Ctrl Pts',(15.2897673262125,-65.5843661188994,11.2216465877777));
#35818=CARTESIAN_POINT('Ctrl Pts',(15.0989143577318,-65.6632851643039,10.8519211229878));
#35819=CARTESIAN_POINT('Ctrl Pts',(15.0064172468355,-65.7158498370977,10.4257987515067));
#35820=CARTESIAN_POINT('Ctrl Pts',(15.0130771992805,-65.7418454548454,9.99981028982554));
#35821=CARTESIAN_POINT('Origin',(17.0820569767664,-63.7511045350785,10.));
#35822=CARTESIAN_POINT('',(15.2652009106025,-66.709565290414,9.99881345470574));
#35823=CARTESIAN_POINT('',(15.1934336836835,-66.4442667934687,9.99943462192768));
#35824=CARTESIAN_POINT('',(14.6503387090836,-64.4026814811241,10.));
#35825=CARTESIAN_POINT('Ctrl Pts',(15.1934336836835,-66.4442667934687,9.99943462192768));
#35826=CARTESIAN_POINT('Ctrl Pts',(15.1827995799554,-66.3950965524831,10.7909504295073));
#35827=CARTESIAN_POINT('Ctrl Pts',(15.5599243826036,-66.2420266256761,11.5846294221378));
#35828=CARTESIAN_POINT('Ctrl Pts',(16.1674256670555,-66.0272275066146,12.0468004663334));
#35829=CARTESIAN_POINT('Ctrl Pts',(16.7997089272064,-65.8036660249294,12.5278249876806));
#35830=CARTESIAN_POINT('Ctrl Pts',(17.6815476659071,-65.5132363543,12.6497433013673));
#35831=CARTESIAN_POINT('Ctrl Pts',(18.4120106025366,-65.2633677075892,12.3579626123137));
#35832=CARTESIAN_POINT('Ctrl Pts',(19.1424735391661,-65.0134990608784,12.06618192326));
#35833=CARTESIAN_POINT('Ctrl Pts',(19.7215606737244,-64.8041914380861,11.3607022314659));
#35834=CARTESIAN_POINT('Ctrl Pts',(19.8839069496221,-64.7065491918251,10.5574238638963));
#35835=CARTESIAN_POINT('Ctrl Pts',(20.0462532255198,-64.608906945564,9.75414549632673));
#35836=CARTESIAN_POINT('Ctrl Pts',(19.7918586427569,-64.6229300758342,8.8530684529817));
#35837=CARTESIAN_POINT('Ctrl Pts',(19.2285753341563,-64.7197196907436,8.25767771891592));
#35838=CARTESIAN_POINT('Ctrl Pts',(18.6652920255557,-64.816509305653,7.66228698485014));
#35839=CARTESIAN_POINT('Ctrl Pts',(17.7931199911174,-64.9960654052016,7.37258256006362));
#35840=CARTESIAN_POINT('Ctrl Pts',(16.9965402212509,-65.1553666185043,7.51828854147109));
#35841=CARTESIAN_POINT('Ctrl Pts',(16.1999604513844,-65.3146678318069,7.66399452287857));
#35842=CARTESIAN_POINT('Ctrl Pts',(15.4789729460896,-65.4537141588635,8.24511091048004));
#35843=CARTESIAN_POINT('Ctrl Pts',(15.1503611804251,-65.4876237233566,9.00142492811739));
#35844=CARTESIAN_POINT('Ctrl Pts',(15.0146236613656,-65.5016305260266,9.31383062721456));
#35845=CARTESIAN_POINT('Ctrl Pts',(14.9458338550092,-65.4976987431426,9.65612879778041));
#35846=CARTESIAN_POINT('Ctrl Pts',(14.9415523108175,-65.4764820235065,9.9989223619293));
#35847=CARTESIAN_POINT('Ctrl Pts',(15.0130771992805,-65.7418454548454,9.99981028982554));
#35848=CARTESIAN_POINT('Ctrl Pts',(15.0193507802528,-65.7663329589547,9.59853518618477));
#35849=CARTESIAN_POINT('Ctrl Pts',(15.1136101264191,-65.7672447483348,9.19737890571016));
#35850=CARTESIAN_POINT('Ctrl Pts',(15.2965249330007,-65.744401378692,8.84359325274533));
#35851=CARTESIAN_POINT('Ctrl Pts',(15.6736197332262,-65.6973077831931,8.1142333249153));
#35852=CARTESIAN_POINT('Ctrl Pts',(16.4275127626821,-65.5492514064624,7.58620525503956));
#35853=CARTESIAN_POINT('Ctrl Pts',(17.2288315064446,-65.3884873478828,7.49440429239113));
#35854=CARTESIAN_POINT('Ctrl Pts',(18.030150250207,-65.2277232893031,7.4026033297427));
#35855=CARTESIAN_POINT('Ctrl Pts',(18.878894708276,-65.0542515488746,7.74702947432161));
#35856=CARTESIAN_POINT('Ctrl Pts',(19.4034973688025,-64.9676333413308,8.37446367269948));
#35857=CARTESIAN_POINT('Ctrl Pts',(19.9281000293289,-64.8810151337869,9.00189787107735));
#35858=CARTESIAN_POINT('Ctrl Pts',(20.1285608923127,-64.8812504591278,9.91234012325419));
#35859=CARTESIAN_POINT('Ctrl Pts',(19.9217039083204,-64.9906262726287,10.7007759738114));
#35860=CARTESIAN_POINT('Ctrl Pts',(19.7148469243281,-65.1000020861296,11.4892118243687));
#35861=CARTESIAN_POINT('Ctrl Pts',(19.1006720933597,-65.3185183877906,12.1556412733063));
#35862=CARTESIAN_POINT('Ctrl Pts',(18.3583974645569,-65.5713589268319,12.4036017192683));
#35863=CARTESIAN_POINT('Ctrl Pts',(17.6161228357541,-65.8241994658732,12.6515621652302));
#35864=CARTESIAN_POINT('Ctrl Pts',(16.745748409117,-66.1113642422947,12.4810536082165));
#35865=CARTESIAN_POINT('Ctrl Pts',(16.1404633167949,-66.3274985456645,11.9679250313906));
#35866=CARTESIAN_POINT('Ctrl Pts',(15.5886775085547,-66.5245294039924,11.5001503082285));
#35867=CARTESIAN_POINT('Ctrl Pts',(15.2571911193414,-66.662531210899,10.7476451883996));
#35868=CARTESIAN_POINT('Ctrl Pts',(15.2652009106025,-66.709565290414,9.99881345470574));
#35869=CARTESIAN_POINT('Origin',(17.0820569767664,-63.7511045350785,10.));
#35870=CARTESIAN_POINT('',(15.5286491313886,-67.6742507328171,10.0019962882658));
#35871=CARTESIAN_POINT('',(15.458048217099,-67.4086397233445,10.0018117506528));
#35872=CARTESIAN_POINT('',(14.6503387090836,-64.4026814811241,10.));
#35873=CARTESIAN_POINT('',(20.2598690437801,-67.0040126136404,11.1728309286207));
#35874=CARTESIAN_POINT('Ctrl Pts',(15.5286491313886,-67.6742507328171,10.0019962882658));
#35875=CARTESIAN_POINT('Ctrl Pts',(15.5421457071955,-67.7079511930089,9.43113200366982));
#35876=CARTESIAN_POINT('Ctrl Pts',(15.7382477902416,-67.6927226550026,8.85763821511471));
#35877=CARTESIAN_POINT('Ctrl Pts',(16.0921495062908,-67.6352118327671,8.41584216487548));
#35878=CARTESIAN_POINT('Ctrl Pts',(16.6037821050588,-67.5520689427972,7.77714150008996));
#35879=CARTESIAN_POINT('Ctrl Pts',(17.4452195762654,-67.3805551035975,7.41369214583755));
#35880=CARTESIAN_POINT('Ctrl Pts',(18.2482818068303,-67.2193238791372,7.48861537411895));
#35881=CARTESIAN_POINT('Ctrl Pts',(19.0513440373952,-67.0580926546768,7.56353860240036));
#35882=CARTESIAN_POINT('Ctrl Pts',(19.8160310273183,-66.9071440449558,8.07683441321558));
#35883=CARTESIAN_POINT('Ctrl Pts',(20.2075211669018,-66.8561932299011,8.7968163762026));
#35884=CARTESIAN_POINT('Ctrl Pts',(20.5990113064853,-66.8052424148464,9.51679833918955));
#35885=CARTESIAN_POINT('Ctrl Pts',(20.6173045957293,-66.854289394458,10.4434664543483));
#35886=CARTESIAN_POINT('Ctrl Pts',(20.2598690437801,-67.0040126136404,11.1728309286206));
#35887=CARTESIAN_POINT('',(16.4802525979518,-68.0323660008166,11.8670505687059));
#35888=CARTESIAN_POINT('Ctrl Pts',(16.4806955947433,-68.0322473001841,11.8669181223571));
#35889=CARTESIAN_POINT('Ctrl Pts',(16.6817854205938,-67.9835336336721,12.0540417240897));
#35890=CARTESIAN_POINT('Ctrl Pts',(16.9239334961962,-67.923876532405,12.2143044024353));
#35891=CARTESIAN_POINT('Ctrl Pts',(17.4856657502708,-67.7816176378542,12.4543153408643));
#35892=CARTESIAN_POINT('Ctrl Pts',(17.8119729521746,-67.6966288605656,12.5175));
#35893=CARTESIAN_POINT('Ctrl Pts',(18.4226933621783,-67.5329868199039,12.5175));
#35894=CARTESIAN_POINT('Ctrl Pts',(18.747778077109,-67.4434356591205,12.4543153408643));
#35895=CARTESIAN_POINT('Ctrl Pts',(19.3446857260753,-67.2746559299571,12.1973867613172));
#35896=CARTESIAN_POINT('Ctrl Pts',(19.6165425195547,-67.1955448337828,12.0036443501621));
#35897=CARTESIAN_POINT('Ctrl Pts',(19.9960747381915,-67.0834304248293,11.6080270340044));
#35898=CARTESIAN_POINT('Ctrl Pts',(20.1448248140073,-67.0387983068925,11.4009948671633));
#35899=CARTESIAN_POINT('Ctrl Pts',(20.2598690437801,-67.0040126136404,11.1728309286206));
#35900=CARTESIAN_POINT('Ctrl Pts',(16.4776938604227,-68.0330516124712,11.8678155752478));
#35901=CARTESIAN_POINT('Ctrl Pts',(16.9785524830602,-67.8522271893252,12.3404055365588));
#35902=CARTESIAN_POINT('Ctrl Pts',(17.6838006560656,-67.6166367512168,12.5855412104357));
#35903=CARTESIAN_POINT('Ctrl Pts',(18.3529108900531,-67.3907294446845,12.5051234941037));
#35904=CARTESIAN_POINT('Ctrl Pts',(19.129979689639,-67.1283727946319,12.4117306641613));
#35905=CARTESIAN_POINT('Ctrl Pts',(19.8583083259861,-66.8790760319582,11.879255644893));
#35906=CARTESIAN_POINT('Ctrl Pts',(20.2061471825013,-66.7317311985187,11.1455779206959));
#35907=CARTESIAN_POINT('Ctrl Pts',(20.5539860390166,-66.5843863650793,10.4119001964987));
#35908=CARTESIAN_POINT('Ctrl Pts',(20.5213351156999,-66.5389934608741,9.47701976737269));
#35909=CARTESIAN_POINT('Ctrl Pts',(20.1165357938135,-66.5933174195301,8.75982961781549));
#35910=CARTESIAN_POINT('Ctrl Pts',(19.7117364719271,-66.6476413781862,8.04263946825829));
#35911=CARTESIAN_POINT('Ctrl Pts',(18.934788751471,-66.8016821997035,7.54313959826994));
#35912=CARTESIAN_POINT('Ctrl Pts',(18.1276415422747,-66.9638149498406,7.48486270274578));
#35913=CARTESIAN_POINT('Ctrl Pts',(17.3204943330785,-67.1259476999777,7.42658580722162));
#35914=CARTESIAN_POINT('Ctrl Pts',(16.483147635142,-67.2961723787346,7.80953188616166));
#35915=CARTESIAN_POINT('Ctrl Pts',(15.9844353298855,-67.3756602454435,8.46229096311826));
#35916=CARTESIAN_POINT('Ctrl Pts',(15.6526293851286,-67.4285455390929,8.89658813193753));
#35917=CARTESIAN_POINT('Ctrl Pts',(15.4707226080323,-67.4412654718215,9.45032013874414));
#35918=CARTESIAN_POINT('Ctrl Pts',(15.458048217099,-67.4086397233445,10.0018117506528));
#35919=CARTESIAN_POINT('Origin',(-18.6889152049569,69.7479810832458,10.));
#35920=CARTESIAN_POINT('',(-13.2791651259751,61.4484819638688,10.0015349814512));
#35921=CARTESIAN_POINT('',(-13.2658134652031,61.3659731009889,9.99957732584554));
#35922=CARTESIAN_POINT('',(-15.7201421778575,70.5434614183684,10.0000000000001));
#35923=CARTESIAN_POINT('',(-16.8135320242448,59.6819508576139,7.03077704625437));
#35924=CARTESIAN_POINT('Ctrl Pts',(-13.2658134652031,61.3659731009889,9.99957732584554));
#35925=CARTESIAN_POINT('Ctrl Pts',(-13.2594372491749,61.3390049028546,10.5364470372516));
#35926=CARTESIAN_POINT('Ctrl Pts',(-13.6128633281576,61.1616793186458,12.0843271181651));
#35927=CARTESIAN_POINT('Ctrl Pts',(-15.9358673415301,60.4026582657957,13.6055385422089));
#35928=CARTESIAN_POINT('Ctrl Pts',(-18.8976307583477,59.447210195013,12.2029441264611));
#35929=CARTESIAN_POINT('Ctrl Pts',(-19.3903963172923,59.1533281063616,8.83503768583798));
#35930=CARTESIAN_POINT('Ctrl Pts',(-17.7660737535059,59.4806667221929,7.29068223125052));
#35931=CARTESIAN_POINT('Ctrl Pts',(-16.8135320242448,59.6819508576139,7.03077704625438));
#35932=CARTESIAN_POINT('',(-15.2780776734586,60.093374610922,7.02605498021586));
#35933=CARTESIAN_POINT('Origin',(-16.0467807963563,59.8874012299222,10.));
#35934=CARTESIAN_POINT('Ctrl Pts',(-13.2791651259751,61.4484819638689,10.0015349814512));
#35935=CARTESIAN_POINT('Ctrl Pts',(-13.2773812390919,61.4440081401684,10.0935838809863));
#35936=CARTESIAN_POINT('Ctrl Pts',(-13.3061918618691,61.3771948495716,11.1915036202381));
#35937=CARTESIAN_POINT('Ctrl Pts',(-14.5474295567697,60.9313710113776,13.1842383274674));
#35938=CARTESIAN_POINT('Ctrl Pts',(-17.8144668208749,59.893545936598,13.1913616605741));
#35939=CARTESIAN_POINT('Ctrl Pts',(-19.6057481548832,59.2511484715134,10.339577077016));
#35940=CARTESIAN_POINT('Ctrl Pts',(-18.3013616530666,59.440726198154,7.2338208659921));
#35941=CARTESIAN_POINT('Ctrl Pts',(-16.187142356251,59.9014396609591,6.78116218790437));
#35942=CARTESIAN_POINT('Ctrl Pts',(-15.2780676602839,60.0933772939441,7.02603075613017));
#35943=CARTESIAN_POINT('Origin',(-18.6889152049569,69.7479810832458,10.));
#35944=CARTESIAN_POINT('',(-13.5461538679481,62.4122187264791,10.0005448248896));
#35945=CARTESIAN_POINT('',(-13.5161734774897,62.3341655182897,9.99879780140835));
#35946=CARTESIAN_POINT('',(-15.7201421778575,70.5434614183684,10.0000000000001));
#35947=CARTESIAN_POINT('Ctrl Pts',(-13.5161734774897,62.3341655182897,9.99879780140835));
#35948=CARTESIAN_POINT('Ctrl Pts',(-13.5082196148794,62.286219899295,10.9294410660881));
#35949=CARTESIAN_POINT('Ctrl Pts',(-14.3903370215027,61.9458317508116,12.870975191806));
#35950=CARTESIAN_POINT('Ctrl Pts',(-17.5197763142875,60.9493268661069,13.4270461480336));
#35951=CARTESIAN_POINT('Ctrl Pts',(-19.7394014348252,60.1927341524848,10.9477123134811));
#35952=CARTESIAN_POINT('Ctrl Pts',(-18.96159921589,60.2392996738452,7.62511676387811));
#35953=CARTESIAN_POINT('Ctrl Pts',(-15.8425832679708,60.9131915231956,6.41562502038854));
#35954=CARTESIAN_POINT('Ctrl Pts',(-13.6032001394547,61.3800631690208,8.04417985348941));
#35955=CARTESIAN_POINT('Ctrl Pts',(-13.2714326411404,61.389739398956,9.52644947847317));
#35956=CARTESIAN_POINT('Ctrl Pts',(-13.2658134652031,61.3659731009889,9.99957732584554));
#35957=CARTESIAN_POINT('Ctrl Pts',(-13.5461538679481,62.4122187264791,10.0005448248896));
#35958=CARTESIAN_POINT('Ctrl Pts',(-13.5391171409456,62.3889104933502,10.4721900135757));
#35959=CARTESIAN_POINT('Ctrl Pts',(-13.8305514728693,62.231485488278,11.9564181322133));
#35960=CARTESIAN_POINT('Ctrl Pts',(-16.0106566332711,61.5138509672068,13.5896176377582));
#35961=CARTESIAN_POINT('Ctrl Pts',(-19.0579057022672,60.5349179618126,12.3623010109727));
#35962=CARTESIAN_POINT('Ctrl Pts',(-19.7341192728292,60.1913020034494,9.0193860958895));
#35963=CARTESIAN_POINT('Ctrl Pts',(-17.3973455890627,60.6550135466887,6.55469600728496));
#35964=CARTESIAN_POINT('Ctrl Pts',(-14.2043402063787,61.3531034969371,7.15651357330629));
#35965=CARTESIAN_POINT('Ctrl Pts',(-13.2968857360054,61.4929236187117,9.08714816254585));
#35966=CARTESIAN_POINT('Ctrl Pts',(-13.2791651259751,61.4484819638689,10.0015349814512));
#35967=CARTESIAN_POINT('Origin',(-18.6889152049569,69.7479810832458,10.));
#35968=CARTESIAN_POINT('',(-13.7984318791272,63.3798972175256,9.9976925905199));
#35969=CARTESIAN_POINT('',(-13.7813169744248,63.2983967128177,10.0022545211422));
#35970=CARTESIAN_POINT('',(-15.7201421778575,70.5434614183684,10.0000000000001));
#35971=CARTESIAN_POINT('Ctrl Pts',(-13.7813169744248,63.2983967128177,10.0022545211422));
#35972=CARTESIAN_POINT('Ctrl Pts',(-13.7746926693741,63.282643341652,10.3298056773904));
#35973=CARTESIAN_POINT('Ctrl Pts',(-13.9475832402569,63.1648404527592,11.6627679218545));
#35974=CARTESIAN_POINT('Ctrl Pts',(-15.7650240000833,62.5524330171351,13.4838568188229));
#35975=CARTESIAN_POINT('Ctrl Pts',(-18.936865245129,61.5406947619309,12.7341264791949));
#35976=CARTESIAN_POINT('Ctrl Pts',(-20.0773594018982,61.0732543185779,9.55182253210509));
#35977=CARTESIAN_POINT('Ctrl Pts',(-18.1357994369342,61.4316477881722,6.76826458716724));
#35978=CARTESIAN_POINT('Ctrl Pts',(-14.8036106221425,62.1626591350494,6.86000957288756));
#35979=CARTESIAN_POINT('Ctrl Pts',(-13.5645914770419,62.3828842093692,8.85264674105157));
#35980=CARTESIAN_POINT('Ctrl Pts',(-13.5167884478445,62.3378725391134,9.926843073658));
#35981=CARTESIAN_POINT('Ctrl Pts',(-13.5161734774897,62.3341655182897,9.99879780140835));
#35982=CARTESIAN_POINT('Ctrl Pts',(-13.7984318791272,63.3798972175256,9.9976925905199));
#35983=CARTESIAN_POINT('Ctrl Pts',(-13.7939231905821,63.3356696948373,10.8435144444689));
#35984=CARTESIAN_POINT('Ctrl Pts',(-14.5389353035615,63.0364669859302,12.7089873258297));
#35985=CARTESIAN_POINT('Ctrl Pts',(-17.5330036055452,62.0804897947072,13.5128046754736));
#35986=CARTESIAN_POINT('Ctrl Pts',(-19.945812508159,61.2715545195409,11.2162142452881));
#35987=CARTESIAN_POINT('Ctrl Pts',(-19.4106046411916,61.2525379570574,7.83042882970079));
#35988=CARTESIAN_POINT('Ctrl Pts',(-16.3703262829259,61.9047530097004,6.38762845988016));
#35989=CARTESIAN_POINT('Ctrl Pts',(-13.9548208376171,62.4147543833102,7.90192541386312));
#35990=CARTESIAN_POINT('Ctrl Pts',(-13.5542391767051,62.4390002488206,9.45861716832901));
#35991=CARTESIAN_POINT('Ctrl Pts',(-13.5461538679481,62.4122187264791,10.0005448248896));
#35992=CARTESIAN_POINT('Origin',(-18.6889152049569,69.7479810832458,10.));
#35993=CARTESIAN_POINT('',(-14.0587048879185,64.3454334554184,10.0025996902774));
#35994=CARTESIAN_POINT('',(-14.038988005468,64.2646301485468,9.99747713720018));
#35995=CARTESIAN_POINT('',(-15.7201421778575,70.5434614183684,10.0000000000001));
#35996=CARTESIAN_POINT('Ctrl Pts',(-14.038988005468,64.2646301485468,9.99747713720018));
#35997=CARTESIAN_POINT('Ctrl Pts',(-14.0349994054244,64.226770392365,10.7242163838114));
#35998=CARTESIAN_POINT('Ctrl Pts',(-14.6082026447201,63.980303897263,12.4671953710476));
#35999=CARTESIAN_POINT('Ctrl Pts',(-17.3556995742977,63.0972885120503,13.5881174655937));
#36000=CARTESIAN_POINT('Ctrl Pts',(-20.0116836036718,62.2237737811954,11.6313322004901));
#36001=CARTESIAN_POINT('Ctrl Pts',(-19.8960390869576,62.0929146809836,8.2231376748613));
#36002=CARTESIAN_POINT('Ctrl Pts',(-17.0756569439774,62.686787843468,6.39583171448279));
#36003=CARTESIAN_POINT('Ctrl Pts',(-14.3543730978417,63.271636045696,7.6257956239861));
#36004=CARTESIAN_POINT('Ctrl Pts',(-13.7950809180928,63.3311289785642,9.32167057633652));
#36005=CARTESIAN_POINT('Ctrl Pts',(-13.7813169744248,63.2983967128177,10.0022545211422));
#36006=CARTESIAN_POINT('Ctrl Pts',(-14.0587048879185,64.3454334554184,10.0025996902774));
#36007=CARTESIAN_POINT('Ctrl Pts',(-14.0539764689082,64.3351645983746,10.2176211405934));
#36008=CARTESIAN_POINT('Ctrl Pts',(-14.1513426806931,64.2433978747177,11.4397371699224));
#36009=CARTESIAN_POINT('Ctrl Pts',(-15.6987166428553,63.7089610525881,13.3670096553834));
#36010=CARTESIAN_POINT('Ctrl Pts',(-18.9427555175128,62.6772983776883,12.9642257537712));
#36011=CARTESIAN_POINT('Ctrl Pts',(-20.3916349158421,62.1266472347557,9.90679500749766));
#36012=CARTESIAN_POINT('Ctrl Pts',(-18.7114286257309,62.4144320750885,6.93283507366423));
#36013=CARTESIAN_POINT('Ctrl Pts',(-15.3704995140603,63.14720625431,6.70571036393722));
#36014=CARTESIAN_POINT('Ctrl Pts',(-13.8968260312722,63.425086417853,8.66708054183125));
#36015=CARTESIAN_POINT('Ctrl Pts',(-13.7992958039273,63.3883718001703,9.83562185337852));
#36016=CARTESIAN_POINT('Ctrl Pts',(-13.7984318791272,63.3798972175256,9.9976925905199));
#36017=CARTESIAN_POINT('Origin',(-18.6889152049569,69.7479810832458,10.));
#36018=CARTESIAN_POINT('',(-14.322133959383,65.3101240288667,9.99868436122735));
#36019=CARTESIAN_POINT('',(-14.2935352300231,65.2317006057018,10.0018375364667));
#36020=CARTESIAN_POINT('',(-15.7201421778575,70.5434614183684,10.0000000000001));
#36021=CARTESIAN_POINT('Ctrl Pts',(-14.2935352300231,65.2317006057018,10.0018375364667));
#36022=CARTESIAN_POINT('Ctrl Pts',(-14.2911203313162,65.2259676792212,10.1205006547493));
#36023=CARTESIAN_POINT('Ctrl Pts',(-14.333487038742,65.1542869058501,11.241710128915));
#36024=CARTESIAN_POINT('Ctrl Pts',(-15.6317182042723,64.6921496134353,13.2184200895793));
#36025=CARTESIAN_POINT('Ctrl Pts',(-18.8835992389528,63.6589647612364,13.1544941616769));
#36026=CARTESIAN_POINT('Ctrl Pts',(-20.6195097408352,63.0319829890498,10.2839896215965));
#36027=CARTESIAN_POINT('Ctrl Pts',(-19.2589973841656,63.2346852212378,7.16081725087092));
#36028=CARTESIAN_POINT('Ctrl Pts',(-15.9765219526977,63.9523759072002,6.56368841308618));
#36029=CARTESIAN_POINT('Ctrl Pts',(-14.2145525524614,64.3015767283499,8.4321298041167));
#36030=CARTESIAN_POINT('Ctrl Pts',(-14.0405269650183,64.2792379389272,9.71707241074879));
#36031=CARTESIAN_POINT('Ctrl Pts',(-14.038988005468,64.2646301485468,9.99747713720018));
#36032=CARTESIAN_POINT('Ctrl Pts',(-14.322133959383,65.3101240288667,9.99868436122735));
#36033=CARTESIAN_POINT('Ctrl Pts',(-14.3164610907008,65.2798663326535,10.593347109087));
#36034=CARTESIAN_POINT('Ctrl Pts',(-14.7310514432717,65.082857752957,12.2044751575874));
#36035=CARTESIAN_POINT('Ctrl Pts',(-17.1999914587374,64.2812461473765,13.6183729089162));
#36036=CARTESIAN_POINT('Ctrl Pts',(-20.0833051820053,63.3462394854811,12.0175557753475));
#36037=CARTESIAN_POINT('Ctrl Pts',(-20.368219412885,63.1074718691845,8.60989310618186));
#36038=CARTESIAN_POINT('Ctrl Pts',(-17.7632104839254,63.6430568297549,6.44715683087691));
#36039=CARTESIAN_POINT('Ctrl Pts',(-14.7920138952891,64.288297311113,7.39383484183699));
#36040=CARTESIAN_POINT('Ctrl Pts',(-14.0761685903618,64.3833599300929,9.20845039448972));
#36041=CARTESIAN_POINT('Ctrl Pts',(-14.0587048879185,64.3454334554184,10.0025996902774));
#36042=CARTESIAN_POINT('Origin',(-18.6889152049569,69.7479810832458,10.));
#36043=CARTESIAN_POINT('',(-14.5724831194333,66.2783193540155,9.99930975590676));
#36044=CARTESIAN_POINT('',(-14.559910913876,66.1956016367402,9.99976839157055));
#36045=CARTESIAN_POINT('',(-15.7201421778575,70.5434614183684,10.0000000000001));
#36046=CARTESIAN_POINT('Ctrl Pts',(-14.559910913876,66.1956016367402,9.99976839157055));
#36047=CARTESIAN_POINT('Ctrl Pts',(-14.5533139234257,66.1695891483769,10.5198381182744));
#36048=CARTESIAN_POINT('Ctrl Pts',(-14.890051591398,65.9976317638641,12.0503568643789));
#36049=CARTESIAN_POINT('Ctrl Pts',(-17.1744195179844,65.2498597727098,13.6018503664189));
#36050=CARTESIAN_POINT('Ctrl Pts',(-20.1560728090925,64.2890822261736,12.2479900298274));
#36051=CARTESIAN_POINT('Ctrl Pts',(-20.7056191362412,63.9799857765361,8.89407499549296));
#36052=CARTESIAN_POINT('Ctrl Pts',(-18.2981238461185,64.4632262402319,6.52411027736645));
#36053=CARTESIAN_POINT('Ctrl Pts',(-15.1680091238728,65.146471993839,7.21818882738257));
#36054=CARTESIAN_POINT('Ctrl Pts',(-14.3115404877175,65.2744447664955,9.11709648401));
#36055=CARTESIAN_POINT('Ctrl Pts',(-14.2935352300231,65.2317006057018,10.0018375364667));
#36056=CARTESIAN_POINT('Ctrl Pts',(-14.5724831194333,66.2783193540155,9.99930975590676));
#36057=CARTESIAN_POINT('Ctrl Pts',(-14.5623726178327,66.2290088142627,10.9656350129456));
#36058=CARTESIAN_POINT('Ctrl Pts',(-15.5078446363719,65.8695090171971,12.9430947115647));
#36059=CARTESIAN_POINT('Ctrl Pts',(-18.7042880702644,64.8527215544621,13.3837942299381));
#36060=CARTESIAN_POINT('Ctrl Pts',(-20.8341986998844,64.1195886430847,10.7999310727637));
#36061=CARTESIAN_POINT('Ctrl Pts',(-19.9114308093218,64.2044184759421,7.49968047567802));
#36062=CARTESIAN_POINT('Ctrl Pts',(-16.7260146593058,64.8955230826759,6.4386200392349));
#36063=CARTESIAN_POINT('Ctrl Pts',(-14.609200226033,65.332074459173,8.15058790184868));
#36064=CARTESIAN_POINT('Ctrl Pts',(-14.3261263074255,65.3314182383775,9.58018345977269));
#36065=CARTESIAN_POINT('Ctrl Pts',(-14.322133959383,65.3101240288667,9.99868436122735));
#36066=CARTESIAN_POINT('Origin',(-18.6889152049569,69.7479810832458,10.));
#36067=CARTESIAN_POINT('',(-14.8383776097513,67.242349320473,10.0022118830713));
#36068=CARTESIAN_POINT('',(-14.810555933805,67.1637176864734,9.9985514014054));
#36069=CARTESIAN_POINT('',(-15.7201421778575,70.5434614183684,10.0000000000001));
#36070=CARTESIAN_POINT('Ctrl Pts',(-14.810555933805,67.1637176864734,9.9985514014054));
#36071=CARTESIAN_POINT('Ctrl Pts',(-14.8034925645054,67.1164300139581,10.9127656351722));
#36072=CARTESIAN_POINT('Ctrl Pts',(-15.6578176600211,66.7843853462346,12.8392373747718));
#36073=CARTESIAN_POINT('Ctrl Pts',(-18.7603708726991,65.795981118425,13.4453363911884));
#36074=CARTESIAN_POINT('Ctrl Pts',(-21.0187603927389,65.0290015152611,11.00449717215));
#36075=CARTESIAN_POINT('Ctrl Pts',(-20.2934961228732,65.0614895355965,7.6699459164611));
#36076=CARTESIAN_POINT('Ctrl Pts',(-17.1938529499358,65.7301904655353,6.40846378494576));
#36077=CARTESIAN_POINT('Ctrl Pts',(-14.9140195913108,66.207004164409,8.01044782382069));
#36078=CARTESIAN_POINT('Ctrl Pts',(-14.5661251855401,66.2201050327307,9.50987006742356));
#36079=CARTESIAN_POINT('Ctrl Pts',(-14.559910913876,66.1956016367402,9.99976839157055));
#36080=CARTESIAN_POINT('Ctrl Pts',(-14.8383776097513,67.242349320473,10.0022118830713));
#36081=CARTESIAN_POINT('Ctrl Pts',(-14.8315944872623,67.2260470012181,10.3408933046041));
#36082=CARTESIAN_POINT('Ctrl Pts',(-15.0130297323862,67.1051700296206,11.688786841075));
#36083=CARTESIAN_POINT('Ctrl Pts',(-16.8683721674333,66.4816292855384,13.5013274912987));
#36084=CARTESIAN_POINT('Ctrl Pts',(-20.0422978199454,65.4687533918912,12.6947822329677));
#36085=CARTESIAN_POINT('Ctrl Pts',(-21.1273143736847,65.0155990043222,9.47487431060756));
#36086=CARTESIAN_POINT('Ctrl Pts',(-19.1153342996386,65.3922823621301,6.72525821930975));
#36087=CARTESIAN_POINT('Ctrl Pts',(-15.7718556315871,66.125739692925,6.90837057311325));
#36088=CARTESIAN_POINT('Ctrl Pts',(-14.6047179173561,66.3280678631807,8.91484226317803));
#36089=CARTESIAN_POINT('Ctrl Pts',(-14.5728955600509,66.2803308931335,9.95989017005515));
#36090=CARTESIAN_POINT('Ctrl Pts',(-14.5724831194333,66.2783193540155,9.99930975590676));
#36091=CARTESIAN_POINT('Origin',(-18.6889152049569,69.7479810832458,10.));
#36092=CARTESIAN_POINT('',(-15.0969161422106,68.2083503098983,9.99673640007589));
#36093=CARTESIAN_POINT('',(-15.0750265266586,68.1281291851066,10.0024371765581));
#36094=CARTESIAN_POINT('',(-15.7201421778575,70.5434614183684,10.0000000000001));
#36095=CARTESIAN_POINT('',(-17.2449834421536,67.8425423025984,7.0617047543859));
#36096=CARTESIAN_POINT('Ctrl Pts',(-17.2449834421536,67.8425423025984,7.06170475438588));
#36097=CARTESIAN_POINT('Ctrl Pts',(-16.2988495743029,68.0419164156806,7.35795147289551));
#36098=CARTESIAN_POINT('Ctrl Pts',(-15.283120482422,68.2441585752431,8.39983158504164));
#36099=CARTESIAN_POINT('Ctrl Pts',(-15.0986382893443,68.2236687995603,9.70207674802626));
#36100=CARTESIAN_POINT('Ctrl Pts',(-15.0969161422106,68.2083503098983,9.99673640007589));
#36101=CARTESIAN_POINT('',(-18.1173331571764,67.6148078402348,6.92649999999998));
#36102=CARTESIAN_POINT('Ctrl Pts',(-18.1173331571765,67.6148078402348,6.92649999999999));
#36103=CARTESIAN_POINT('Ctrl Pts',(-17.8331351207385,67.6909584745888,6.92649999999999));
#36104=CARTESIAN_POINT('Ctrl Pts',(-17.5337033543064,67.7691522152651,6.97030621012379));
#36105=CARTESIAN_POINT('Ctrl Pts',(-17.2449834421535,67.8425423025984,7.06170475438591));
#36106=CARTESIAN_POINT('',(-18.8148375643562,67.424038192564,7.01163591529244));
#36107=CARTESIAN_POINT('Ctrl Pts',(-18.8154792730626,67.4238662472344,7.01293629783559));
#36108=CARTESIAN_POINT('Ctrl Pts',(-18.5825814377542,67.4888593221927,6.95435125823855));
#36109=CARTESIAN_POINT('Ctrl Pts',(-18.3453582319348,67.5537087055992,6.92649999999999));
#36110=CARTESIAN_POINT('Ctrl Pts',(-18.1173331571764,67.6148078402348,6.92649999999999));
#36111=CARTESIAN_POINT('Ctrl Pts',(-18.8139865064172,67.4242662328515,7.00991129962864));
#36112=CARTESIAN_POINT('Ctrl Pts',(-18.6713424458927,67.4544236505276,6.97326843816113));
#36113=CARTESIAN_POINT('Ctrl Pts',(-17.5558463812024,67.6913073253836,6.77617107551512));
#36114=CARTESIAN_POINT('Ctrl Pts',(-15.6699322564948,68.0973070404755,7.59313914445675));
#36115=CARTESIAN_POINT('Ctrl Pts',(-15.0894434810379,68.1615830306032,9.30549521878024));
#36116=CARTESIAN_POINT('Ctrl Pts',(-15.0750265266586,68.1281291851066,10.0024371765581));
#36117=CARTESIAN_POINT('Origin',(-69.7479810832458,-18.6889152049569,10.));
#36118=CARTESIAN_POINT('',(-61.4484819638689,-13.2791651259751,10.0015349814514));
#36119=CARTESIAN_POINT('',(-61.3659731009889,-13.2658134652031,9.99957732584557));
#36120=CARTESIAN_POINT('',(-70.5434614183684,-15.7201421778575,10.0000000000001));
#36121=CARTESIAN_POINT('',(-59.6819508576141,-16.8135320242443,7.03077704625423));
#36122=CARTESIAN_POINT('Ctrl Pts',(-61.3659731009889,-13.2658134652031,
9.99957732584557));
#36123=CARTESIAN_POINT('Ctrl Pts',(-61.3390049028546,-13.2594372491749,
10.5364470372518));
#36124=CARTESIAN_POINT('Ctrl Pts',(-61.1616793186457,-13.6128633281578,
12.0843271181655));
#36125=CARTESIAN_POINT('Ctrl Pts',(-60.4026582657955,-15.9358673415309,
13.605538542209));
#36126=CARTESIAN_POINT('Ctrl Pts',(-59.4472101950129,-18.8976307583482,
12.2029441264605));
#36127=CARTESIAN_POINT('Ctrl Pts',(-59.1533281063617,-19.3903963172921,
8.83503768583721));
#36128=CARTESIAN_POINT('Ctrl Pts',(-59.4806667221931,-17.7660737535053,
7.29068223125013));
#36129=CARTESIAN_POINT('Ctrl Pts',(-59.6819508576141,-16.8135320242442,
7.03077704625421));
#36130=CARTESIAN_POINT('',(-60.0933746109222,-15.2780776734579,7.02605498021606));
#36131=CARTESIAN_POINT('Origin',(-59.8874012299222,-16.0467807963563,10.));
#36132=CARTESIAN_POINT('Ctrl Pts',(-61.4484819638689,-13.2791651259751,
10.0015349814514));
#36133=CARTESIAN_POINT('Ctrl Pts',(-61.4440081401684,-13.2773812390919,
10.0935838809867));
#36134=CARTESIAN_POINT('Ctrl Pts',(-61.3771948495715,-13.3061918618692,
11.1915036202386));
#36135=CARTESIAN_POINT('Ctrl Pts',(-60.9313710113774,-14.5474295567703,
13.1842383274678));
#36136=CARTESIAN_POINT('Ctrl Pts',(-59.8935459365978,-17.8144668208756,
13.1913616605738));
#36137=CARTESIAN_POINT('Ctrl Pts',(-59.2511484715134,-19.6057481548832,
10.3395770770153));
#36138=CARTESIAN_POINT('Ctrl Pts',(-59.4407261981542,-18.301361653066,7.23382086599162));
#36139=CARTESIAN_POINT('Ctrl Pts',(-59.9014396609593,-16.1871423562504,
6.78116218790435));
#36140=CARTESIAN_POINT('Ctrl Pts',(-60.0933772939442,-15.2780676602833,
7.02603075613034));
#36141=CARTESIAN_POINT('Origin',(-69.7479810832458,-18.6889152049569,10.));
#36142=CARTESIAN_POINT('',(-62.4122187264791,-13.5461538679481,10.0005448248896));
#36143=CARTESIAN_POINT('',(-62.3341655182897,-13.5161734774897,9.99879780140837));
#36144=CARTESIAN_POINT('',(-70.5434614183684,-15.7201421778575,10.0000000000001));
#36145=CARTESIAN_POINT('Ctrl Pts',(-62.3341655182897,-13.5161734774897,
9.99879780140837));
#36146=CARTESIAN_POINT('Ctrl Pts',(-62.286219899295,-13.5082196148794,10.9294410660883));
#36147=CARTESIAN_POINT('Ctrl Pts',(-61.9458317508115,-14.3903370215031,
12.8709751918064));
#36148=CARTESIAN_POINT('Ctrl Pts',(-60.9493268661068,-17.5197763142882,
13.4270461480333));
#36149=CARTESIAN_POINT('Ctrl Pts',(-60.1927341524846,-19.7394014348254,
10.9477123134803));
#36150=CARTESIAN_POINT('Ctrl Pts',(-60.2392996738453,-18.9615992158895,
7.62511676387751));
#36151=CARTESIAN_POINT('Ctrl Pts',(-60.9131915231958,-15.84258326797,6.41562502038865));
#36152=CARTESIAN_POINT('Ctrl Pts',(-61.3800631690209,-13.6032001394545,
8.04417985348988));
#36153=CARTESIAN_POINT('Ctrl Pts',(-61.389739398956,-13.2714326411404,9.52644947847341));
#36154=CARTESIAN_POINT('Ctrl Pts',(-61.3659731009889,-13.2658134652031,
9.99957732584557));
#36155=CARTESIAN_POINT('Ctrl Pts',(-62.4122187264791,-13.5461538679481,
10.0005448248896));
#36156=CARTESIAN_POINT('Ctrl Pts',(-62.3889104933502,-13.5391171409457,
10.4721900135759));
#36157=CARTESIAN_POINT('Ctrl Pts',(-62.231485488278,-13.8305514728695,11.9564181322137));
#36158=CARTESIAN_POINT('Ctrl Pts',(-61.5138509672066,-16.0106566332719,
13.5896176377583));
#36159=CARTESIAN_POINT('Ctrl Pts',(-60.5349179618125,-19.0579057022677,
12.362301010972));
#36160=CARTESIAN_POINT('Ctrl Pts',(-60.1913020034495,-19.7341192728289,
9.01938609588879));
#36161=CARTESIAN_POINT('Ctrl Pts',(-60.6550135466889,-17.397345589062,6.55469600728472));
#36162=CARTESIAN_POINT('Ctrl Pts',(-61.3531034969373,-14.2043402063782,
7.15651357330673));
#36163=CARTESIAN_POINT('Ctrl Pts',(-61.4929236187118,-13.2968857360053,
9.08714816254619));
#36164=CARTESIAN_POINT('Ctrl Pts',(-61.4484819638689,-13.2791651259751,
10.0015349814514));
#36165=CARTESIAN_POINT('Origin',(-69.7479810832458,-18.6889152049569,10.));
#36166=CARTESIAN_POINT('',(-63.3798972175256,-13.7984318791272,9.99769259051991));
#36167=CARTESIAN_POINT('',(-63.2983967128177,-13.7813169744248,10.0022545211422));
#36168=CARTESIAN_POINT('',(-70.5434614183684,-15.7201421778575,10.0000000000001));
#36169=CARTESIAN_POINT('Ctrl Pts',(-63.2983967128177,-13.7813169744248,
10.0022545211422));
#36170=CARTESIAN_POINT('Ctrl Pts',(-63.2826433416521,-13.7746926693741,
10.3298056773906));
#36171=CARTESIAN_POINT('Ctrl Pts',(-63.1648404527592,-13.9475832402571,
11.662767921855));
#36172=CARTESIAN_POINT('Ctrl Pts',(-62.5524330171347,-15.7650240000841,
13.4838568188231));
#36173=CARTESIAN_POINT('Ctrl Pts',(-61.5406947619308,-18.9368652451296,
12.7341264791944));
#36174=CARTESIAN_POINT('Ctrl Pts',(-61.0732543185779,-20.0773594018981,
9.5518225321043));
#36175=CARTESIAN_POINT('Ctrl Pts',(-61.4316477881724,-18.1357994369335,
6.76826458716688));
#36176=CARTESIAN_POINT('Ctrl Pts',(-62.1626591350496,-14.8036106221418,
6.86000957288797));
#36177=CARTESIAN_POINT('Ctrl Pts',(-62.3828842093693,-13.5645914770418,
8.85264674105202));
#36178=CARTESIAN_POINT('Ctrl Pts',(-62.3378725391134,-13.5167884478445,
9.92684307365823));
#36179=CARTESIAN_POINT('Ctrl Pts',(-62.3341655182897,-13.5161734774897,
9.99879780140837));
#36180=CARTESIAN_POINT('Ctrl Pts',(-63.3798972175256,-13.7984318791272,
9.99769259051991));
#36181=CARTESIAN_POINT('Ctrl Pts',(-63.3356696948373,-13.7939231905821,
10.8435144444692));
#36182=CARTESIAN_POINT('Ctrl Pts',(-63.0364669859302,-14.5389353035618,
12.7089873258301));
#36183=CARTESIAN_POINT('Ctrl Pts',(-62.0804897947069,-17.5330036055459,
13.5128046754734));
#36184=CARTESIAN_POINT('Ctrl Pts',(-61.271554519541,-19.9458125081593,11.2162142452873));
#36185=CARTESIAN_POINT('Ctrl Pts',(-61.2525379570575,-19.4106046411911,
7.83042882970014));
#36186=CARTESIAN_POINT('Ctrl Pts',(-61.9047530097006,-16.3703262829251,
6.3876284598802));
#36187=CARTESIAN_POINT('Ctrl Pts',(-62.4147543833102,-13.9548208376168,
7.9019254138636));
#36188=CARTESIAN_POINT('Ctrl Pts',(-62.4390002488206,-13.5542391767051,
9.45861716832925));
#36189=CARTESIAN_POINT('Ctrl Pts',(-62.4122187264791,-13.5461538679481,
10.0005448248896));
#36190=CARTESIAN_POINT('Origin',(-69.7479810832458,-18.6889152049569,10.));
#36191=CARTESIAN_POINT('',(-64.3454334554185,-14.0587048879185,10.0025996902775));
#36192=CARTESIAN_POINT('',(-64.2646301485469,-14.038988005468,9.99747713720016));
#36193=CARTESIAN_POINT('',(-70.5434614183684,-15.7201421778575,10.0000000000001));
#36194=CARTESIAN_POINT('Ctrl Pts',(-64.2646301485469,-14.038988005468,9.99747713720016));
#36195=CARTESIAN_POINT('Ctrl Pts',(-64.2267703923651,-14.0349994054244,
10.7242163838116));
#36196=CARTESIAN_POINT('Ctrl Pts',(-63.9803038972629,-14.6082026447204,
12.4671953710481));
#36197=CARTESIAN_POINT('Ctrl Pts',(-63.0972885120501,-17.3556995742985,
13.5881174655936));
#36198=CARTESIAN_POINT('Ctrl Pts',(-62.2237737811953,-20.0116836036721,
11.6313322004894));
#36199=CARTESIAN_POINT('Ctrl Pts',(-62.0929146809836,-19.8960390869572,
8.2231376748606));
#36200=CARTESIAN_POINT('Ctrl Pts',(-62.6867878434683,-17.0756569439767,
6.39583171448275));
#36201=CARTESIAN_POINT('Ctrl Pts',(-63.271636045696,-14.3543730978414,7.62579562398654));
#36202=CARTESIAN_POINT('Ctrl Pts',(-63.3311289785642,-13.7950809180928,
9.32167057633674));
#36203=CARTESIAN_POINT('Ctrl Pts',(-63.2983967128177,-13.7813169744248,
10.0022545211422));
#36204=CARTESIAN_POINT('Ctrl Pts',(-64.3454334554185,-14.0587048879185,
10.0025996902775));
#36205=CARTESIAN_POINT('Ctrl Pts',(-64.3351645983747,-14.0539764689082,
10.2176211405936));
#36206=CARTESIAN_POINT('Ctrl Pts',(-64.2433978747177,-14.1513426806932,
11.4397371699229));
#36207=CARTESIAN_POINT('Ctrl Pts',(-63.7089610525879,-15.6987166428561,
13.3670096553837));
#36208=CARTESIAN_POINT('Ctrl Pts',(-62.6772983776881,-18.9427555175135,
12.9642257537707));
#36209=CARTESIAN_POINT('Ctrl Pts',(-62.1266472347557,-20.391634915842,9.90679500749681));
#36210=CARTESIAN_POINT('Ctrl Pts',(-62.4144320750887,-18.7114286257302,
6.93283507366378));
#36211=CARTESIAN_POINT('Ctrl Pts',(-63.1472062543103,-15.3704995140596,
6.70571036393757));
#36212=CARTESIAN_POINT('Ctrl Pts',(-63.4250864178529,-13.8968260312721,
8.66708054183172));
#36213=CARTESIAN_POINT('Ctrl Pts',(-63.3883718001703,-13.7992958039273,
9.83562185337876));
#36214=CARTESIAN_POINT('Ctrl Pts',(-63.3798972175256,-13.7984318791272,
9.99769259051991));
#36215=CARTESIAN_POINT('Origin',(-69.7479810832458,-18.6889152049569,10.));
#36216=CARTESIAN_POINT('',(-65.3101240288668,-14.322133959383,9.99868436122753));
#36217=CARTESIAN_POINT('',(-65.2317006057018,-14.2935352300231,10.0018375364667));
#36218=CARTESIAN_POINT('',(-70.5434614183684,-15.7201421778575,10.0000000000001));
#36219=CARTESIAN_POINT('Ctrl Pts',(-65.2317006057018,-14.2935352300231,
10.0018375364667));
#36220=CARTESIAN_POINT('Ctrl Pts',(-65.2259676792212,-14.2911203313162,
10.1205006547495));
#36221=CARTESIAN_POINT('Ctrl Pts',(-65.15428690585,-14.3334870387421,11.2417101289155));
#36222=CARTESIAN_POINT('Ctrl Pts',(-64.6921496134352,-15.631718204273,13.2184200895797));
#36223=CARTESIAN_POINT('Ctrl Pts',(-63.6589647612361,-18.8835992389535,
13.1544941616765));
#36224=CARTESIAN_POINT('Ctrl Pts',(-63.0319829890499,-20.6195097408353,
10.2839896215957));
#36225=CARTESIAN_POINT('Ctrl Pts',(-63.2346852212379,-19.2589973841649,
7.16081725087042));
#36226=CARTESIAN_POINT('Ctrl Pts',(-63.9523759072004,-15.9765219526969,
6.56368841308645));
#36227=CARTESIAN_POINT('Ctrl Pts',(-64.30157672835,-14.2145525524612,8.43212980411715));
#36228=CARTESIAN_POINT('Ctrl Pts',(-64.2792379389272,-14.0405269650183,
9.71707241074901));
#36229=CARTESIAN_POINT('Ctrl Pts',(-64.2646301485469,-14.038988005468,9.99747713720016));
#36230=CARTESIAN_POINT('Ctrl Pts',(-65.3101240288668,-14.322133959383,9.99868436122753));
#36231=CARTESIAN_POINT('Ctrl Pts',(-65.2798663326535,-14.3164610907008,
10.5933471090874));
#36232=CARTESIAN_POINT('Ctrl Pts',(-65.0828577529568,-14.7310514432721,
12.204475157588));
#36233=CARTESIAN_POINT('Ctrl Pts',(-64.2812461473762,-17.1999914587382,
13.6183729089162));
#36234=CARTESIAN_POINT('Ctrl Pts',(-63.346239485481,-20.0833051820058,12.0175557753468));
#36235=CARTESIAN_POINT('Ctrl Pts',(-63.1074718691846,-20.3682194128847,
8.60989310618102));
#36236=CARTESIAN_POINT('Ctrl Pts',(-63.6430568297552,-17.7632104839245,
6.44715683087674));
#36237=CARTESIAN_POINT('Ctrl Pts',(-64.2882973111131,-14.7920138952887,
7.3938348418375));
#36238=CARTESIAN_POINT('Ctrl Pts',(-64.3833599300929,-14.0761685903618,
9.20845039449));
#36239=CARTESIAN_POINT('Ctrl Pts',(-64.3454334554185,-14.0587048879185,
10.0025996902775));
#36240=CARTESIAN_POINT('Origin',(-69.7479810832458,-18.6889152049569,10.));
#36241=CARTESIAN_POINT('',(-66.2783193540156,-14.5724831194333,9.99930975590678));
#36242=CARTESIAN_POINT('',(-66.1956016367402,-14.559910913876,9.99976839157072));
#36243=CARTESIAN_POINT('',(-70.5434614183684,-15.7201421778575,10.0000000000001));
#36244=CARTESIAN_POINT('Ctrl Pts',(-66.1956016367402,-14.559910913876,9.99976839157072));
#36245=CARTESIAN_POINT('Ctrl Pts',(-66.1695891483769,-14.5533139234258,
10.5198381182747));
#36246=CARTESIAN_POINT('Ctrl Pts',(-65.9976317638641,-14.8900515913983,
12.0503568643794));
#36247=CARTESIAN_POINT('Ctrl Pts',(-65.2498597727096,-17.1744195179851,
13.601850366419));
#36248=CARTESIAN_POINT('Ctrl Pts',(-64.2890822261733,-20.156072809093,12.2479900298267));
#36249=CARTESIAN_POINT('Ctrl Pts',(-63.9799857765362,-20.705619136241,8.89407499549219));
#36250=CARTESIAN_POINT('Ctrl Pts',(-64.4632262402321,-18.2981238461178,
6.52411027736622));
#36251=CARTESIAN_POINT('Ctrl Pts',(-65.1464719938391,-15.1680091238725,
7.21818882738302));
#36252=CARTESIAN_POINT('Ctrl Pts',(-65.2744447664955,-14.3115404877176,
9.11709648401023));
#36253=CARTESIAN_POINT('Ctrl Pts',(-65.2317006057018,-14.2935352300231,
10.0018375364667));
#36254=CARTESIAN_POINT('Ctrl Pts',(-66.2783193540156,-14.5724831194333,
9.99930975590678));
#36255=CARTESIAN_POINT('Ctrl Pts',(-66.2290088142628,-14.5623726178327,
10.9656350129459));
#36256=CARTESIAN_POINT('Ctrl Pts',(-65.869509017197,-15.5078446363724,12.9430947115652));
#36257=CARTESIAN_POINT('Ctrl Pts',(-64.8527215544619,-18.7042880702652,
13.3837942299378));
#36258=CARTESIAN_POINT('Ctrl Pts',(-64.1195886430846,-20.8341986998846,
10.7999310727628));
#36259=CARTESIAN_POINT('Ctrl Pts',(-64.2044184759423,-19.9114308093211,
7.49968047567736));
#36260=CARTESIAN_POINT('Ctrl Pts',(-64.895523082676,-16.726014659305,6.43862003923507));
#36261=CARTESIAN_POINT('Ctrl Pts',(-65.3320744591731,-14.6092002260327,
8.15058790184925));
#36262=CARTESIAN_POINT('Ctrl Pts',(-65.3314182383775,-14.3261263074255,
9.58018345977307));
#36263=CARTESIAN_POINT('Ctrl Pts',(-65.3101240288668,-14.322133959383,9.99868436122753));
#36264=CARTESIAN_POINT('Origin',(-69.7479810832458,-18.6889152049569,10.));
#36265=CARTESIAN_POINT('',(-67.242349320473,-14.8383776097513,10.0022118830713));
#36266=CARTESIAN_POINT('',(-67.1637176864735,-14.810555933805,9.9985514014054));
#36267=CARTESIAN_POINT('',(-70.5434614183684,-15.7201421778575,10.0000000000001));
#36268=CARTESIAN_POINT('Ctrl Pts',(-67.1637176864735,-14.810555933805,9.9985514014054));
#36269=CARTESIAN_POINT('Ctrl Pts',(-67.1164300139581,-14.8034925645054,
10.9127656351724));
#36270=CARTESIAN_POINT('Ctrl Pts',(-66.7843853462345,-15.6578176600215,
12.8392373747722));
#36271=CARTESIAN_POINT('Ctrl Pts',(-65.7959811184248,-18.7603708726999,
13.4453363911881));
#36272=CARTESIAN_POINT('Ctrl Pts',(-65.0290015152611,-21.0187603927391,
11.0044971721492));
#36273=CARTESIAN_POINT('Ctrl Pts',(-65.0614895355965,-20.2934961228726,
7.66994591646049));
#36274=CARTESIAN_POINT('Ctrl Pts',(-65.7301904655356,-17.193852949935,6.40846378494586));
#36275=CARTESIAN_POINT('Ctrl Pts',(-66.2070041644091,-14.9140195913105,
8.01044782382119));
#36276=CARTESIAN_POINT('Ctrl Pts',(-66.2201050327307,-14.5661251855401,
9.50987006742391));
#36277=CARTESIAN_POINT('Ctrl Pts',(-66.1956016367402,-14.559910913876,9.99976839157072));
#36278=CARTESIAN_POINT('Ctrl Pts',(-67.242349320473,-14.8383776097513,10.0022118830713));
#36279=CARTESIAN_POINT('Ctrl Pts',(-67.2260470012181,-14.8315944872623,
10.3408933046044));
#36280=CARTESIAN_POINT('Ctrl Pts',(-67.1051700296205,-15.0130297323864,
11.6887868410756));
#36281=CARTESIAN_POINT('Ctrl Pts',(-66.4816292855381,-16.8683721674343,
13.501327491299));
#36282=CARTESIAN_POINT('Ctrl Pts',(-65.468753391891,-20.0422978199461,12.6947822329671));
#36283=CARTESIAN_POINT('Ctrl Pts',(-65.0155990043222,-21.1273143736846,
9.47487431060658));
#36284=CARTESIAN_POINT('Ctrl Pts',(-65.3922823621304,-19.1153342996378,
6.72525821930933));
#36285=CARTESIAN_POINT('Ctrl Pts',(-66.1257396929252,-15.7718556315863,
6.90837057311376));
#36286=CARTESIAN_POINT('Ctrl Pts',(-66.3280678631807,-14.604717917356,8.9148422631786));
#36287=CARTESIAN_POINT('Ctrl Pts',(-66.2803308931335,-14.5728955600509,
9.95989017005544));
#36288=CARTESIAN_POINT('Ctrl Pts',(-66.2783193540156,-14.5724831194333,
9.99930975590678));
#36289=CARTESIAN_POINT('Origin',(-69.7479810832458,-18.6889152049569,10.));
#36290=CARTESIAN_POINT('',(-68.2083503098983,-15.0969161422106,9.99673640007589));
#36291=CARTESIAN_POINT('',(-68.1281291851066,-15.0750265266586,10.0024371765581));
#36292=CARTESIAN_POINT('',(-70.5434614183684,-15.7201421778575,10.0000000000001));
#36293=CARTESIAN_POINT('',(-67.8425423025986,-17.2449834421528,7.06170475438615));
#36294=CARTESIAN_POINT('Ctrl Pts',(-67.8425423025986,-17.2449834421528,
7.06170475438615));
#36295=CARTESIAN_POINT('Ctrl Pts',(-68.0419164156808,-16.2988495743022,
7.35795147289606));
#36296=CARTESIAN_POINT('Ctrl Pts',(-68.2441585752431,-15.2831204824218,
8.39983158504225));
#36297=CARTESIAN_POINT('Ctrl Pts',(-68.2236687995604,-15.0986382893443,
9.70207674802657));
#36298=CARTESIAN_POINT('Ctrl Pts',(-68.2083503098983,-15.0969161422106,
9.99673640007589));
#36299=CARTESIAN_POINT('',(-67.6148078402348,-18.1173331571764,6.92649999999999));
#36300=CARTESIAN_POINT('Ctrl Pts',(-67.6148078402348,-18.1173331571764,
6.9265));
#36301=CARTESIAN_POINT('Ctrl Pts',(-67.6909584745889,-17.8331351207383,
6.9265));
#36302=CARTESIAN_POINT('Ctrl Pts',(-67.7691522152653,-17.5337033543059,
6.97030621012388));
#36303=CARTESIAN_POINT('Ctrl Pts',(-67.8425423025986,-17.2449834421528,
7.06170475438616));
#36304=CARTESIAN_POINT('',(-67.4240381925642,-18.8148375643558,7.01163591529236));
#36305=CARTESIAN_POINT('Ctrl Pts',(-67.4238662472345,-18.8154792730621,
7.01293629783548));
#36306=CARTESIAN_POINT('Ctrl Pts',(-67.4888593221928,-18.5825814377539,
6.95435125823852));
#36307=CARTESIAN_POINT('Ctrl Pts',(-67.5537087055993,-18.3453582319346,
6.9265));
#36308=CARTESIAN_POINT('Ctrl Pts',(-67.6148078402348,-18.1173331571764,
6.9265));
#36309=CARTESIAN_POINT('Ctrl Pts',(-67.4242662328516,-18.8139865064169,
7.00991129962856));
#36310=CARTESIAN_POINT('Ctrl Pts',(-67.4544236505277,-18.6713424458923,
6.97326843816105));
#36311=CARTESIAN_POINT('Ctrl Pts',(-67.6913073253837,-17.5558463812018,
6.7761710755152));
#36312=CARTESIAN_POINT('Ctrl Pts',(-68.0973070404756,-15.6699322564945,
7.59313914445722));
#36313=CARTESIAN_POINT('Ctrl Pts',(-68.1615830306033,-15.0894434810379,
9.30549521878046));
#36314=CARTESIAN_POINT('Ctrl Pts',(-68.1281291851067,-15.0750265266586,
10.0024371765581));
#36315=CARTESIAN_POINT('Origin',(18.6889152049569,-69.7479810832458,10.));
#36316=CARTESIAN_POINT('',(13.2791651259751,-61.4484819638689,10.0015349814511));
#36317=CARTESIAN_POINT('',(13.2658134652031,-61.3659731009889,9.99957732584551));
#36318=CARTESIAN_POINT('',(15.7201421778575,-70.5434614183684,10.0000000000001));
#36319=CARTESIAN_POINT('',(16.8135320242446,-59.681950857614,7.03077704625433));
#36320=CARTESIAN_POINT('Ctrl Pts',(13.2658134652031,-61.3659731009889,9.99957732584551));
#36321=CARTESIAN_POINT('Ctrl Pts',(13.2594372491749,-61.3390049028546,10.5364470372516));
#36322=CARTESIAN_POINT('Ctrl Pts',(13.6128633281576,-61.1616793186458,12.0843271181652));
#36323=CARTESIAN_POINT('Ctrl Pts',(15.9358673415304,-60.4026582657957,13.6055385422089));
#36324=CARTESIAN_POINT('Ctrl Pts',(18.8976307583479,-59.4472101950129,12.2029441264609));
#36325=CARTESIAN_POINT('Ctrl Pts',(19.3903963172922,-59.1533281063617,8.83503768583773));
#36326=CARTESIAN_POINT('Ctrl Pts',(17.7660737535057,-59.480666722193,7.29068223125039));
#36327=CARTESIAN_POINT('Ctrl Pts',(16.8135320242446,-59.681950857614,7.03077704625433));
#36328=CARTESIAN_POINT('',(15.2780776734582,-60.0933746109221,7.02605498021597));
#36329=CARTESIAN_POINT('Origin',(16.0467807963563,-59.8874012299222,10.));
#36330=CARTESIAN_POINT('Ctrl Pts',(13.2791651259751,-61.4484819638689,10.0015349814511));
#36331=CARTESIAN_POINT('Ctrl Pts',(13.277381239092,-61.4440081401684,10.0935838809864));
#36332=CARTESIAN_POINT('Ctrl Pts',(13.3061918618692,-61.3771948495716,11.1915036202383));
#36333=CARTESIAN_POINT('Ctrl Pts',(14.5474295567701,-60.9313710113775,13.1842383274677));
#36334=CARTESIAN_POINT('Ctrl Pts',(17.8144668208753,-59.8935459365978,13.1913616605739));
#36335=CARTESIAN_POINT('Ctrl Pts',(19.6057481548832,-59.2511484715134,10.3395770770155));
#36336=CARTESIAN_POINT('Ctrl Pts',(18.3013616530662,-59.4407261981541,7.23382086599181));
#36337=CARTESIAN_POINT('Ctrl Pts',(16.1871423562507,-59.9014396609592,6.78116218790437));
#36338=CARTESIAN_POINT('Ctrl Pts',(15.2780676602835,-60.0933772939442,7.02603075613028));
#36339=CARTESIAN_POINT('Origin',(18.6889152049569,-69.7479810832458,10.));
#36340=CARTESIAN_POINT('',(13.5461538679481,-62.4122187264791,10.0005448248895));
#36341=CARTESIAN_POINT('',(13.5161734774897,-62.3341655182897,9.99879780140832));
#36342=CARTESIAN_POINT('',(15.7201421778575,-70.5434614183684,10.0000000000001));
#36343=CARTESIAN_POINT('Ctrl Pts',(13.5161734774897,-62.3341655182897,9.99879780140832));
#36344=CARTESIAN_POINT('Ctrl Pts',(13.5082196148794,-62.286219899295,10.9294410660881));
#36345=CARTESIAN_POINT('Ctrl Pts',(14.3903370215028,-61.9458317508116,12.8709751918061));
#36346=CARTESIAN_POINT('Ctrl Pts',(17.5197763142877,-60.9493268661069,13.4270461480335));
#36347=CARTESIAN_POINT('Ctrl Pts',(19.7394014348253,-60.1927341524847,10.9477123134808));
#36348=CARTESIAN_POINT('Ctrl Pts',(18.9615992158899,-60.2392996738452,7.62511676387795));
#36349=CARTESIAN_POINT('Ctrl Pts',(15.8425832679706,-60.9131915231956,6.41562502038857));
#36350=CARTESIAN_POINT('Ctrl Pts',(13.6032001394546,-61.3800631690209,8.04417985348955));
#36351=CARTESIAN_POINT('Ctrl Pts',(13.2714326411404,-61.389739398956,9.52644947847322));
#36352=CARTESIAN_POINT('Ctrl Pts',(13.2658134652031,-61.3659731009889,9.99957732584551));
#36353=CARTESIAN_POINT('Ctrl Pts',(13.5461538679481,-62.4122187264791,10.0005448248895));
#36354=CARTESIAN_POINT('Ctrl Pts',(13.5391171409456,-62.3889104933503,10.4721900135758));
#36355=CARTESIAN_POINT('Ctrl Pts',(13.8305514728694,-62.231485488278,11.9564181322135));
#36356=CARTESIAN_POINT('Ctrl Pts',(16.0106566332716,-61.5138509672066,13.5896176377583));
#36357=CARTESIAN_POINT('Ctrl Pts',(19.0579057022675,-60.5349179618126,12.3623010109723));
#36358=CARTESIAN_POINT('Ctrl Pts',(19.734119272829,-60.1913020034494,9.01938609588904));
#36359=CARTESIAN_POINT('Ctrl Pts',(17.3973455890623,-60.6550135466889,6.55469600728483));
#36360=CARTESIAN_POINT('Ctrl Pts',(14.2043402063785,-61.3531034969372,7.15651357330655));
#36361=CARTESIAN_POINT('Ctrl Pts',(13.2968857360054,-61.4929236187117,9.08714816254594));
#36362=CARTESIAN_POINT('Ctrl Pts',(13.2791651259751,-61.4484819638689,10.0015349814511));
#36363=CARTESIAN_POINT('Origin',(18.6889152049569,-69.7479810832458,10.));
#36364=CARTESIAN_POINT('',(13.7984318791273,-63.3798972175256,9.99769259051987));
#36365=CARTESIAN_POINT('',(13.7813169744248,-63.2983967128177,10.0022545211422));
#36366=CARTESIAN_POINT('',(15.7201421778575,-70.5434614183684,10.0000000000001));
#36367=CARTESIAN_POINT('Ctrl Pts',(13.7813169744248,-63.2983967128177,10.0022545211422));
#36368=CARTESIAN_POINT('Ctrl Pts',(13.7746926693741,-63.2826433416521,10.3298056773904));
#36369=CARTESIAN_POINT('Ctrl Pts',(13.9475832402569,-63.1648404527592,11.6627679218547));
#36370=CARTESIAN_POINT('Ctrl Pts',(15.7650240000835,-62.5524330171349,13.483856818823));
#36371=CARTESIAN_POINT('Ctrl Pts',(18.9368652451291,-61.5406947619309,12.7341264791948));
#36372=CARTESIAN_POINT('Ctrl Pts',(20.0773594018982,-61.0732543185779,9.5518225321049));
#36373=CARTESIAN_POINT('Ctrl Pts',(18.135799436934,-61.4316477881723,6.76826458716716));
#36374=CARTESIAN_POINT('Ctrl Pts',(14.8036106221423,-62.1626591350494,6.86000957288767));
#36375=CARTESIAN_POINT('Ctrl Pts',(13.5645914770419,-62.3828842093692,8.85264674105167));
#36376=CARTESIAN_POINT('Ctrl Pts',(13.5167884478445,-62.3378725391134,9.92684307365803));
#36377=CARTESIAN_POINT('Ctrl Pts',(13.5161734774897,-62.3341655182897,9.99879780140832));
#36378=CARTESIAN_POINT('Ctrl Pts',(13.7984318791273,-63.3798972175256,9.99769259051987));
#36379=CARTESIAN_POINT('Ctrl Pts',(13.7939231905821,-63.3356696948374,10.8435144444691));
#36380=CARTESIAN_POINT('Ctrl Pts',(14.5389353035617,-63.0364669859302,12.70898732583));
#36381=CARTESIAN_POINT('Ctrl Pts',(17.5330036055456,-62.080489794707,13.5128046754735));
#36382=CARTESIAN_POINT('Ctrl Pts',(19.9458125081592,-61.2715545195409,11.2162142452876));
#36383=CARTESIAN_POINT('Ctrl Pts',(19.4106046411912,-61.2525379570576,7.83042882970036));
#36384=CARTESIAN_POINT('Ctrl Pts',(16.3703262829254,-61.9047530097005,6.3876284598802));
#36385=CARTESIAN_POINT('Ctrl Pts',(13.9548208376169,-62.4147543833103,7.90192541386342));
#36386=CARTESIAN_POINT('Ctrl Pts',(13.5542391767051,-62.4390002488207,9.45861716832912));
#36387=CARTESIAN_POINT('Ctrl Pts',(13.5461538679481,-62.4122187264791,10.0005448248895));
#36388=CARTESIAN_POINT('Origin',(18.6889152049569,-69.7479810832458,10.));
#36389=CARTESIAN_POINT('',(14.0587048879185,-64.3454334554184,10.0025996902774));
#36390=CARTESIAN_POINT('',(14.038988005468,-64.2646301485468,9.99747713720016));
#36391=CARTESIAN_POINT('',(15.7201421778575,-70.5434614183684,10.0000000000001));
#36392=CARTESIAN_POINT('Ctrl Pts',(14.038988005468,-64.2646301485468,9.99747713720016));
#36393=CARTESIAN_POINT('Ctrl Pts',(14.0349994054244,-64.226770392365,10.7242163838114));
#36394=CARTESIAN_POINT('Ctrl Pts',(14.6082026447201,-63.9803038972629,12.4671953710477));
#36395=CARTESIAN_POINT('Ctrl Pts',(17.3556995742979,-63.0972885120504,13.5881174655936));
#36396=CARTESIAN_POINT('Ctrl Pts',(20.0116836036718,-62.2237737811953,11.6313322004899));
#36397=CARTESIAN_POINT('Ctrl Pts',(19.8960390869576,-62.0929146809836,8.22313767486115));
#36398=CARTESIAN_POINT('Ctrl Pts',(17.0756569439772,-62.6867878434681,6.39583171448279));
#36399=CARTESIAN_POINT('Ctrl Pts',(14.3543730978416,-63.271636045696,7.62579562398619));
#36400=CARTESIAN_POINT('Ctrl Pts',(13.7950809180928,-63.3311289785642,9.32167057633656));
#36401=CARTESIAN_POINT('Ctrl Pts',(13.7813169744248,-63.2983967128177,10.0022545211422));
#36402=CARTESIAN_POINT('Ctrl Pts',(14.0587048879185,-64.3454334554185,10.0025996902774));
#36403=CARTESIAN_POINT('Ctrl Pts',(14.0539764689082,-64.3351645983746,10.2176211405935));
#36404=CARTESIAN_POINT('Ctrl Pts',(14.1513426806932,-64.2433978747176,11.4397371699227));
#36405=CARTESIAN_POINT('Ctrl Pts',(15.6987166428558,-63.708961052588,13.3670096553836));
#36406=CARTESIAN_POINT('Ctrl Pts',(18.9427555175132,-62.6772983776882,12.9642257537709));
#36407=CARTESIAN_POINT('Ctrl Pts',(20.3916349158421,-62.1266472347557,9.9067950074971));
#36408=CARTESIAN_POINT('Ctrl Pts',(18.7114286257305,-62.4144320750886,6.93283507366396));
#36409=CARTESIAN_POINT('Ctrl Pts',(15.3704995140598,-63.1472062543102,6.70571036393745));
#36410=CARTESIAN_POINT('Ctrl Pts',(13.8968260312721,-63.425086417853,8.66708054183155));
#36411=CARTESIAN_POINT('Ctrl Pts',(13.7992958039273,-63.3883718001703,9.83562185337865));
#36412=CARTESIAN_POINT('Ctrl Pts',(13.7984318791273,-63.3798972175256,9.99769259051987));
#36413=CARTESIAN_POINT('Origin',(18.6889152049569,-69.7479810832458,10.));
#36414=CARTESIAN_POINT('',(14.3221339593831,-65.3101240288668,9.99868436122731));
#36415=CARTESIAN_POINT('',(14.2935352300231,-65.2317006057018,10.0018375364666));
#36416=CARTESIAN_POINT('',(15.7201421778575,-70.5434614183684,10.0000000000001));
#36417=CARTESIAN_POINT('Ctrl Pts',(14.2935352300231,-65.2317006057018,10.0018375364666));
#36418=CARTESIAN_POINT('Ctrl Pts',(14.2911203313162,-65.2259676792212,10.1205006547493));
#36419=CARTESIAN_POINT('Ctrl Pts',(14.333487038742,-65.1542869058501,11.2417101289151));
#36420=CARTESIAN_POINT('Ctrl Pts',(15.6317182042724,-64.6921496134353,13.2184200895794));
#36421=CARTESIAN_POINT('Ctrl Pts',(18.8835992389529,-63.6589647612363,13.1544941616768));
#36422=CARTESIAN_POINT('Ctrl Pts',(20.6195097408352,-63.0319829890498,10.2839896215964));
#36423=CARTESIAN_POINT('Ctrl Pts',(19.2589973841654,-63.2346852212378,7.16081725087081));
#36424=CARTESIAN_POINT('Ctrl Pts',(15.9765219526975,-63.9523759072003,6.56368841308624));
#36425=CARTESIAN_POINT('Ctrl Pts',(14.2145525524613,-64.30157672835,8.43212980411679));
#36426=CARTESIAN_POINT('Ctrl Pts',(14.0405269650183,-64.2792379389272,9.71707241074883));
#36427=CARTESIAN_POINT('Ctrl Pts',(14.038988005468,-64.2646301485468,9.99747713720016));
#36428=CARTESIAN_POINT('Ctrl Pts',(14.3221339593831,-65.3101240288668,9.99868436122731));
#36429=CARTESIAN_POINT('Ctrl Pts',(14.3164610907008,-65.2798663326535,10.5933471090872));
#36430=CARTESIAN_POINT('Ctrl Pts',(14.7310514432719,-65.0828577529568,12.2044751575878));
#36431=CARTESIAN_POINT('Ctrl Pts',(17.1999914587379,-64.2812461473763,13.6183729089162));
#36432=CARTESIAN_POINT('Ctrl Pts',(20.0833051820056,-63.346239485481,12.017555775347));
#36433=CARTESIAN_POINT('Ctrl Pts',(20.3682194128848,-63.1074718691846,8.60989310618131));
#36434=CARTESIAN_POINT('Ctrl Pts',(17.7632104839249,-63.6430568297551,6.44715683087681));
#36435=CARTESIAN_POINT('Ctrl Pts',(14.7920138952889,-64.2882973111131,7.39383484183733));
#36436=CARTESIAN_POINT('Ctrl Pts',(14.0761685903618,-64.3833599300929,9.20845039448988));
#36437=CARTESIAN_POINT('Ctrl Pts',(14.0587048879185,-64.3454334554185,10.0025996902774));
#36438=CARTESIAN_POINT('Origin',(18.6889152049569,-69.7479810832458,10.));
#36439=CARTESIAN_POINT('',(14.5724831194333,-66.2783193540155,9.99930975590673));
#36440=CARTESIAN_POINT('',(14.559910913876,-66.1956016367402,9.99976839157072));
#36441=CARTESIAN_POINT('',(15.7201421778575,-70.5434614183684,10.0000000000001));
#36442=CARTESIAN_POINT('Ctrl Pts',(14.559910913876,-66.1956016367402,9.99976839157072));
#36443=CARTESIAN_POINT('Ctrl Pts',(14.5533139234257,-66.1695891483769,10.5198381182745));
#36444=CARTESIAN_POINT('Ctrl Pts',(14.8900515913981,-65.9976317638641,12.050356864379));
#36445=CARTESIAN_POINT('Ctrl Pts',(17.1744195179845,-65.2498597727098,13.6018503664189));
#36446=CARTESIAN_POINT('Ctrl Pts',(20.1560728090925,-64.2890822261735,12.2479900298273));
#36447=CARTESIAN_POINT('Ctrl Pts',(20.7056191362412,-63.9799857765361,8.89407499549286));
#36448=CARTESIAN_POINT('Ctrl Pts',(18.2981238461184,-64.463226240232,6.52411027736642));
#36449=CARTESIAN_POINT('Ctrl Pts',(15.1680091238728,-65.146471993839,7.21818882738264));
#36450=CARTESIAN_POINT('Ctrl Pts',(14.3115404877176,-65.2744447664955,9.11709648401002));
#36451=CARTESIAN_POINT('Ctrl Pts',(14.2935352300231,-65.2317006057018,10.0018375364666));
#36452=CARTESIAN_POINT('Ctrl Pts',(14.5724831194333,-66.2783193540155,9.99930975590673));
#36453=CARTESIAN_POINT('Ctrl Pts',(14.5623726178327,-66.2290088142627,10.9656350129458));
#36454=CARTESIAN_POINT('Ctrl Pts',(15.5078446363722,-65.8695090171971,12.9430947115651));
#36455=CARTESIAN_POINT('Ctrl Pts',(18.7042880702649,-64.8527215544619,13.3837942299379));
#36456=CARTESIAN_POINT('Ctrl Pts',(20.8341986998846,-64.1195886430847,10.7999310727631));
#36457=CARTESIAN_POINT('Ctrl Pts',(19.9114308093213,-64.2044184759422,7.49968047567758));
#36458=CARTESIAN_POINT('Ctrl Pts',(16.7260146593053,-64.895523082676,6.43862003923502));
#36459=CARTESIAN_POINT('Ctrl Pts',(14.6092002260328,-65.3320744591731,8.15058790184903));
#36460=CARTESIAN_POINT('Ctrl Pts',(14.3261263074255,-65.3314182383775,9.58018345977284));
#36461=CARTESIAN_POINT('Ctrl Pts',(14.3221339593831,-65.3101240288668,9.99868436122731));
#36462=CARTESIAN_POINT('Origin',(18.6889152049569,-69.7479810832458,10.));
#36463=CARTESIAN_POINT('',(14.8383776097513,-67.242349320473,10.0022118830713));
#36464=CARTESIAN_POINT('',(14.810555933805,-67.1637176864735,9.99855140140539));
#36465=CARTESIAN_POINT('',(15.7201421778575,-70.5434614183684,10.0000000000001));
#36466=CARTESIAN_POINT('Ctrl Pts',(14.810555933805,-67.1637176864735,9.99855140140538));
#36467=CARTESIAN_POINT('Ctrl Pts',(14.8034925645054,-67.1164300139582,10.9127656351722));
#36468=CARTESIAN_POINT('Ctrl Pts',(15.6578176600211,-66.7843853462345,12.8392373747718));
#36469=CARTESIAN_POINT('Ctrl Pts',(18.7603708726992,-65.795981118425,13.4453363911883));
#36470=CARTESIAN_POINT('Ctrl Pts',(21.0187603927389,-65.0290015152611,11.0044971721499));
#36471=CARTESIAN_POINT('Ctrl Pts',(20.2934961228731,-65.0614895355965,7.66994591646104));
#36472=CARTESIAN_POINT('Ctrl Pts',(17.1938529499357,-65.7301904655353,6.40846378494577));
#36473=CARTESIAN_POINT('Ctrl Pts',(14.9140195913107,-66.2070041644091,8.01044782382078));
#36474=CARTESIAN_POINT('Ctrl Pts',(14.5661251855401,-66.2201050327307,9.50987006742371));
#36475=CARTESIAN_POINT('Ctrl Pts',(14.559910913876,-66.1956016367402,9.99976839157072));
#36476=CARTESIAN_POINT('Ctrl Pts',(14.8383776097513,-67.242349320473,10.0022118830713));
#36477=CARTESIAN_POINT('Ctrl Pts',(14.8315944872623,-67.2260470012181,10.3408933046043));
#36478=CARTESIAN_POINT('Ctrl Pts',(15.0130297323863,-67.1051700296206,11.6887868410754));
#36479=CARTESIAN_POINT('Ctrl Pts',(16.868372167434,-66.4816292855382,13.5013274912989));
#36480=CARTESIAN_POINT('Ctrl Pts',(20.0422978199459,-65.468753391891,12.6947822329673));
#36481=CARTESIAN_POINT('Ctrl Pts',(21.1273143736846,-65.0155990043222,9.47487431060689));
#36482=CARTESIAN_POINT('Ctrl Pts',(19.1153342996381,-65.3922823621302,6.72525821930947));
#36483=CARTESIAN_POINT('Ctrl Pts',(15.7718556315866,-66.1257396929252,6.90837057311361));
#36484=CARTESIAN_POINT('Ctrl Pts',(14.604717917356,-66.3280678631807,8.9148422631784));
#36485=CARTESIAN_POINT('Ctrl Pts',(14.5728955600509,-66.2803308931334,9.95989017005532));
#36486=CARTESIAN_POINT('Ctrl Pts',(14.5724831194333,-66.2783193540155,9.99930975590673));
#36487=CARTESIAN_POINT('Origin',(18.6889152049569,-69.7479810832458,10.));
#36488=CARTESIAN_POINT('',(15.0969161422106,-68.2083503098983,9.99673640007585));
#36489=CARTESIAN_POINT('',(15.0750265266586,-68.1281291851066,10.0024371765581));
#36490=CARTESIAN_POINT('',(15.7201421778575,-70.5434614183684,10.0000000000001));
#36491=CARTESIAN_POINT('',(17.2449834421531,-67.8425423025985,7.06170475438607));
#36492=CARTESIAN_POINT('Ctrl Pts',(17.244983442153,-67.8425423025985,7.06170475438608));
#36493=CARTESIAN_POINT('Ctrl Pts',(16.2988495743024,-68.0419164156808,7.35795147289589));
#36494=CARTESIAN_POINT('Ctrl Pts',(15.2831204824219,-68.2441585752431,8.39983158504204));
#36495=CARTESIAN_POINT('Ctrl Pts',(15.0986382893443,-68.2236687995604,9.70207674802644));
#36496=CARTESIAN_POINT('Ctrl Pts',(15.0969161422106,-68.2083503098983,9.99673640007585));
#36497=CARTESIAN_POINT('',(18.1173331571764,-67.6148078402348,6.92649999999999));
#36498=CARTESIAN_POINT('Ctrl Pts',(18.1173331571764,-67.6148078402348,6.9265));
#36499=CARTESIAN_POINT('Ctrl Pts',(17.8331351207384,-67.6909584745889,6.9265));
#36500=CARTESIAN_POINT('Ctrl Pts',(17.5337033543061,-67.7691522152652,6.97030621012385));
#36501=CARTESIAN_POINT('Ctrl Pts',(17.2449834421531,-67.8425423025985,7.06170475438607));
#36502=CARTESIAN_POINT('',(18.814837564356,-67.4240381925641,7.01163591529248));
#36503=CARTESIAN_POINT('Ctrl Pts',(18.8154792730625,-67.4238662472344,7.01293629783558));
#36504=CARTESIAN_POINT('Ctrl Pts',(18.5825814377542,-67.4888593221927,6.95435125823855));
#36505=CARTESIAN_POINT('Ctrl Pts',(18.3453582319347,-67.5537087055993,6.9265));
#36506=CARTESIAN_POINT('Ctrl Pts',(18.1173331571764,-67.6148078402348,6.9265));
#36507=CARTESIAN_POINT('Ctrl Pts',(18.8139865064172,-67.4242662328515,7.00991129962864));
#36508=CARTESIAN_POINT('Ctrl Pts',(18.6713424458927,-67.4544236505276,6.97326843816114));
#36509=CARTESIAN_POINT('Ctrl Pts',(17.5558463812023,-67.6913073253836,6.77617107551513));
#36510=CARTESIAN_POINT('Ctrl Pts',(15.6699322564948,-68.0973070404755,7.59313914445677));
#36511=CARTESIAN_POINT('Ctrl Pts',(15.0894434810379,-68.1615830306033,9.30549521878023));
#36512=CARTESIAN_POINT('Ctrl Pts',(15.0750265266586,-68.1281291851066,10.0024371765581));
#36513=CARTESIAN_POINT('Ctrl Pts',(20.25986904378,-67.0040126136404,11.1728309286208));
#36514=CARTESIAN_POINT('Ctrl Pts',(20.6173045957293,-66.854289394458,10.4434664543484));
#36515=CARTESIAN_POINT('Ctrl Pts',(20.5807180172414,-66.7561954352348,8.5901302240308));
#36516=CARTESIAN_POINT('Ctrl Pts',(18.2866570474721,-67.2090412643978,7.05024279158514));
#36517=CARTESIAN_POINT('Ctrl Pts',(15.7623446338521,-67.7235827819969,8.14059085434237));
#36518=CARTESIAN_POINT('Ctrl Pts',(15.216861454864,-67.7078986042171,10.8824467802982));
#36519=CARTESIAN_POINT('Ctrl Pts',(17.0999173665986,-67.0414893382909,12.8405694561119));
#36520=CARTESIAN_POINT('Ctrl Pts',(19.6999556621849,-66.1829652216241,12.2707319173769));
#36521=CARTESIAN_POINT('Ctrl Pts',(20.6677950818131,-65.7617874756575,9.68094249642519));
#36522=CARTESIAN_POINT('Ctrl Pts',(19.1062967313386,-66.0183437425752,7.37485535276709));
#36523=CARTESIAN_POINT('Ctrl Pts',(16.3687616678974,-66.5900180970019,7.40446197973339));
#36524=CARTESIAN_POINT('Ctrl Pts',(14.8547867084588,-66.83384050967,9.74329926128826));
#36525=CARTESIAN_POINT('Ctrl Pts',(15.8753739824799,-66.3985290187163,12.3105450512028));
#36526=CARTESIAN_POINT('Ctrl Pts',(18.4864972623912,-65.5370346894516,12.8220707222439));
#36527=CARTESIAN_POINT('Ctrl Pts',(20.3290217552966,-64.8814857844687,10.822782375431));
#36528=CARTESIAN_POINT('Ctrl Pts',(19.727639166345,-64.8807798084461,8.09145561890051));
#36529=CARTESIAN_POINT('Ctrl Pts',(17.1814057921381,-65.4011950297317,7.0581771851638));
#36530=CARTESIAN_POINT('Ctrl Pts',(14.9197267037702,-65.8453641599238,8.64226139479105));
#36531=CARTESIAN_POINT('Ctrl Pts',(14.9188369907852,-65.6837566027253,11.434336752144));
#36532=CARTESIAN_POINT('Ctrl Pts',(17.1435292903638,-64.9258061425711,12.950271123299));
#36533=CARTESIAN_POINT('Ctrl Pts',(19.5784782321595,-64.1115175849317,11.8413258175013));
#36534=CARTESIAN_POINT('Ctrl Pts',(20.0212914063392,-63.831020197438,9.09413821413805));
#36535=CARTESIAN_POINT('Ctrl Pts',(18.0419954959311,-64.1995249831398,7.15290308224172));
#36536=CARTESIAN_POINT('Ctrl Pts',(15.3655869450732,-64.7548205378835,7.74475277436881));
#36537=CARTESIAN_POINT('Ctrl Pts',(14.3372888766999,-64.8685062198083,10.3431139119317));
#36538=CARTESIAN_POINT('Ctrl Pts',(15.8359873727447,-64.305085213021,12.6362038638413));
#36539=CARTESIAN_POINT('Ctrl Pts',(18.4922795208016,-63.4314879220136,12.5838422163726));
#36540=CARTESIAN_POINT('Ctrl Pts',(19.9068421044142,-62.8906110650171,10.2326155433118));
#36541=CARTESIAN_POINT('Ctrl Pts',(18.785128603301,-63.0293273367051,7.67442896667229));
#36542=CARTESIAN_POINT('Ctrl Pts',(16.0891375551553,-63.589870005783,7.18532148363254));
#36543=CARTESIAN_POINT('Ctrl Pts',(14.1815147862765,-63.9391700310929,9.20045592301443));
#36544=CARTESIAN_POINT('Ctrl Pts',(14.723488576521,-63.6321026366037,11.9269511029871));
#36545=CARTESIAN_POINT('Ctrl Pts',(17.196861615384,-62.8075183731851,12.9390225214355));
#36546=CARTESIAN_POINT('Ctrl Pts',(19.3650552728408,-62.064706678561,11.3362221619435));
#36547=CARTESIAN_POINT('Ctrl Pts',(19.2630114600594,-61.9302032807139,8.54457429525393));
#36548=CARTESIAN_POINT('Ctrl Pts',(16.9455204456758,-62.3893271714101,7.04783027207107));
#36549=CARTESIAN_POINT('Ctrl Pts',(14.4384735898226,-62.8992423967486,8.17765522357052));
#36550=CARTESIAN_POINT('Ctrl Pts',(13.9364114971972,-62.8719235739435,10.9288348037816));
#36551=CARTESIAN_POINT('Ctrl Pts',(15.8500240410822,-62.1973266831091,12.8536227562671));
#36552=CARTESIAN_POINT('Ctrl Pts',(18.4407556977104,-61.3412962728355,12.2395195742225));
#36553=CARTESIAN_POINT('Ctrl Pts',(19.3676134988852,-60.9310995184379,9.63289839745374));
#36554=CARTESIAN_POINT('Ctrl Pts',(17.7699646296637,-61.19734228766,7.35288957156119));
#36555=CARTESIAN_POINT('Ctrl Pts',(15.0332534115106,-61.768795893407,7.4280377744411));
#36556=CARTESIAN_POINT('Ctrl Pts',(13.5563500795275,-62.0026849934363,9.79147768509013));
#36557=CARTESIAN_POINT('Ctrl Pts',(14.6172778371392,-61.5565643024821,12.3404488591358));
#36558=CARTESIAN_POINT('Ctrl Pts',(17.2361027255532,-60.6930063334387,12.8070892069869));
#36559=CARTESIAN_POINT('Ctrl Pts',(19.0468753473843,-60.0459653166684,10.7762699688264));
#36560=CARTESIAN_POINT('Ctrl Pts',(18.4024589901612,-60.0567902041013,8.05473611617462));
#36561=CARTESIAN_POINT('Ctrl Pts',(15.8403574002337,-60.5814573009746,7.06404294414454));
#36562=CARTESIAN_POINT('Ctrl Pts',(13.6037685248158,-61.0189035288689,8.6852426906357));
#36563=CARTESIAN_POINT('Ctrl Pts',(13.6472648693585,-60.8454027634006,11.4767030328866));
#36564=CARTESIAN_POINT('Ctrl Pts',(15.8948076660286,-60.0813295310042,12.9532921034687));
#36565=CARTESIAN_POINT('Ctrl Pts',(18.3134648367079,-59.2714063402785,11.8044287744804));
#36566=CARTESIAN_POINT('Ctrl Pts',(18.7097689547776,-59.0033710168103,9.04578082775224));
#36567=CARTESIAN_POINT('Ctrl Pts',(17.3744086881426,-59.2532824184769,7.78080120942667));
#36568=CARTESIAN_POINT('Ctrl Pts',(16.5917431062327,-59.4090483774018,7.56791319796495));
#36569=CARTESIAN_POINT('Ctrl Pts',(20.4459680138347,-67.0649244254632,11.259172404465));
#36570=CARTESIAN_POINT('Ctrl Pts',(20.8307101569087,-66.9078844272409,10.4761135710142));
#36571=CARTESIAN_POINT('Ctrl Pts',(20.7934159435358,-66.8099800782137,8.48633842059632));
#36572=CARTESIAN_POINT('Ctrl Pts',(18.3334494707627,-67.3072801529265,6.83308754393487));
#36573=CARTESIAN_POINT('Ctrl Pts',(15.6262809016687,-67.8708178297157,8.00370485831645));
#36574=CARTESIAN_POINT('Ctrl Pts',(15.0436190322123,-67.8650956520227,10.9474107537966));
#36575=CARTESIAN_POINT('Ctrl Pts',(17.0682804619448,-67.160743301905,13.049686519018));
#36576=CARTESIAN_POINT('Ctrl Pts',(19.8627070898848,-66.2501329885662,12.4378986762067));
#36577=CARTESIAN_POINT('Ctrl Pts',(20.9047756131301,-65.8090656142303,9.65745411880352));
#36578=CARTESIAN_POINT('Ctrl Pts',(19.2313015598939,-66.0956256802751,7.18159743500985));
#36579=CARTESIAN_POINT('Ctrl Pts',(16.2952133143914,-66.7205021994896,7.21338364285578));
#36580=CARTESIAN_POINT('Ctrl Pts',(14.6727612295383,-66.9933909703099,9.72440146443637));
#36581=CARTESIAN_POINT('Ctrl Pts',(15.7714607991054,-66.5371493528456,12.4806427736085));
#36582=CARTESIAN_POINT('Ctrl Pts',(18.5777884658272,-65.6233501657762,13.0298259452254));
#36583=CARTESIAN_POINT('Ctrl Pts',(20.558934634444,-64.9306576947328,10.8833539743373));
#36584=CARTESIAN_POINT('Ctrl Pts',(19.9162581518544,-64.9410163841629,7.95095238475401));
#36585=CARTESIAN_POINT('Ctrl Pts',(17.1855548447373,-65.5108601749996,6.8416060517578));
#36586=CARTESIAN_POINT('Ctrl Pts',(14.7603541429464,-65.9988447894534,8.54230738426523));
#36587=CARTESIAN_POINT('Ctrl Pts',(14.7623776252392,-65.836456643933,11.5399297656087));
#36588=CARTESIAN_POINT('Ctrl Pts',(17.153826032904,-65.033824019284,13.167464204339));
#36589=CARTESIAN_POINT('Ctrl Pts',(19.7710097578038,-64.170705798679,11.9768805549433));
#36590=CARTESIAN_POINT('Ctrl Pts',(20.2494006496399,-63.8806753904707,9.02745047458965));
#36591=CARTESIAN_POINT('Ctrl Pts',(18.1273716126602,-64.2874254021705,6.94330548061662));
#36592=CARTESIAN_POINT('Ctrl Pts',(15.2569098917896,-64.8947173471079,7.57872596768878));
#36593=CARTESIAN_POINT('Ctrl Pts',(14.1558892629051,-65.0278889803931,10.368373274399));
#36594=CARTESIAN_POINT('Ctrl Pts',(15.7678976499206,-64.4341066798257,12.8302759390873));
#36595=CARTESIAN_POINT('Ctrl Pts',(18.622719426852,-63.5073135350879,12.774059531474));
#36596=CARTESIAN_POINT('Ctrl Pts',(20.1443979832212,-62.9377350396947,10.2497402360733));
#36597=CARTESIAN_POINT('Ctrl Pts',(18.9430848635891,-63.0977799648827,7.50322506140514));
#36598=CARTESIAN_POINT('Ctrl Pts',(16.0515990210027,-63.7107053062554,6.97811046011711));
#36599=CARTESIAN_POINT('Ctrl Pts',(14.0065195594074,-64.096836741373,9.14159508133232));
#36600=CARTESIAN_POINT('Ctrl Pts',(14.5913710742638,-63.7782802952007,12.0688094033195));
#36601=CARTESIAN_POINT('Ctrl Pts',(17.2498076016886,-62.9041084194736,13.1553875028215));
#36602=CARTESIAN_POINT('Ctrl Pts',(19.5805980497845,-62.1177290461057,11.4345921747923));
#36603=CARTESIAN_POINT('Ctrl Pts',(19.4740206690255,-61.9844404141372,8.43742875512301));
#36604=CARTESIAN_POINT('Ctrl Pts',(16.9888992784429,-62.4884807287627,6.83049741954164));
#36605=CARTESIAN_POINT('Ctrl Pts',(14.3002673230732,-63.0470515348742,8.04349783254836));
#36606=CARTESIAN_POINT('Ctrl Pts',(13.7642231138315,-63.0288381927736,10.9972137711305));
#36607=CARTESIAN_POINT('Ctrl Pts',(15.8216906940826,-62.3156954611178,13.063700777119));
#36608=CARTESIAN_POINT('Ctrl Pts',(18.60612554685,-61.4077624358673,12.4043885425466));
#36609=CARTESIAN_POINT('Ctrl Pts',(19.6041954665562,-60.9784844518179,9.60587310900414));
#36610=CARTESIAN_POINT('Ctrl Pts',(17.8919095654204,-61.275444121164,7.15801457676317));
#36611=CARTESIAN_POINT('Ctrl Pts',(14.9567058150545,-61.9000836406211,7.23869504058996));
#36612=CARTESIAN_POINT('Ctrl Pts',(13.374054496997,-62.1623078281203,9.77612668779255));
#36613=CARTESIAN_POINT('Ctrl Pts',(14.5160643361694,-61.6944612588913,12.5127480402917));
#36614=CARTESIAN_POINT('Ctrl Pts',(17.3306605884647,-60.7784465109949,13.0137415206691));
#36615=CARTESIAN_POINT('Ctrl Pts',(19.2777173765313,-60.0948882619405,10.8334174170446));
#36616=CARTESIAN_POINT('Ctrl Pts',(18.5888390654041,-60.117626694016,7.91152966540906));
#36617=CARTESIAN_POINT('Ctrl Pts',(15.841099356146,-60.6920353750482,6.84790363622589));
#36618=CARTESIAN_POINT('Ctrl Pts',(13.4428359587848,-61.172802160534,8.58845287746038));
#36619=CARTESIAN_POINT('Ctrl Pts',(13.4925131117116,-60.9976452524506,11.5854149675156));
#36620=CARTESIAN_POINT('Ctrl Pts',(15.9084942245292,-60.188439109268,13.1707075830488));
#36621=CARTESIAN_POINT('Ctrl Pts',(18.5081868105879,-59.33000762519,11.9372672251406));
#36622=CARTESIAN_POINT('Ctrl Pts',(18.9366447422825,-59.0533567133274,8.97553311378072));
#36623=CARTESIAN_POINT('Ctrl Pts',(17.5049637099303,-59.3290771863823,7.61742821670124));
#36624=CARTESIAN_POINT('Ctrl Pts',(16.66567274557,-59.5000158708059,7.38886781406141));
#36625=CARTESIAN_POINT('Ctrl Pts',(20.6320669838895,-67.125836237286,11.3455138803092));
#36626=CARTESIAN_POINT('Ctrl Pts',(21.0441157180881,-66.9614794600238,10.5087606876799));
#36627=CARTESIAN_POINT('Ctrl Pts',(21.0061138698302,-66.8637647211925,8.38254661716184));
#36628=CARTESIAN_POINT('Ctrl Pts',(18.3802418940532,-67.4055190414551,6.6159322962846));
#36629=CARTESIAN_POINT('Ctrl Pts',(15.4902171694852,-68.0180528774347,7.86681886229056));
#36630=CARTESIAN_POINT('Ctrl Pts',(14.8703766095605,-68.0222926998283,11.0123747272948));
#36631=CARTESIAN_POINT('Ctrl Pts',(17.036643557291,-67.2799972655193,13.2588035819241));
#36632=CARTESIAN_POINT('Ctrl Pts',(20.0254585175847,-66.3173007555082,12.6050654350364));
#36633=CARTESIAN_POINT('Ctrl Pts',(21.1417561444472,-65.8563437528032,9.63396574118186));
#36634=CARTESIAN_POINT('Ctrl Pts',(19.3563063884492,-66.1729076179749,6.98833951725262));
#36635=CARTESIAN_POINT('Ctrl Pts',(16.2216649608854,-66.8509863019774,7.02230530597816));
#36636=CARTESIAN_POINT('Ctrl Pts',(14.4907357506179,-67.1529414309498,9.70550366758451));
#36637=CARTESIAN_POINT('Ctrl Pts',(15.667547615731,-66.675769686975,12.6507404960141));
#36638=CARTESIAN_POINT('Ctrl Pts',(18.6690796692632,-65.7096656421006,13.2375811682069));
#36639=CARTESIAN_POINT('Ctrl Pts',(20.7888475135915,-64.979829604997,10.9439255732436));
#36640=CARTESIAN_POINT('Ctrl Pts',(20.1048771373637,-65.0012529598797,7.81044915060753));
#36641=CARTESIAN_POINT('Ctrl Pts',(17.1897038973365,-65.6205253202675,6.62503491835177));
#36642=CARTESIAN_POINT('Ctrl Pts',(14.6009815821227,-66.152325418983,8.44235337373943));
#36643=CARTESIAN_POINT('Ctrl Pts',(14.6059182596933,-65.9891566851404,11.6455227790734));
#36644=CARTESIAN_POINT('Ctrl Pts',(17.1641227754442,-65.1418418959969,13.384657285379));
#36645=CARTESIAN_POINT('Ctrl Pts',(19.9635412834482,-64.2298940124262,12.1124352923853));
#36646=CARTESIAN_POINT('Ctrl Pts',(20.4775098929405,-63.9303305835035,8.96076273504126));
#36647=CARTESIAN_POINT('Ctrl Pts',(18.2127477293893,-64.3753258212012,6.73370787899151));
#36648=CARTESIAN_POINT('Ctrl Pts',(15.1482328385059,-65.0346141563323,7.41269916100874));
#36649=CARTESIAN_POINT('Ctrl Pts',(13.9744896491103,-65.1872717409779,10.3936326368663));
#36650=CARTESIAN_POINT('Ctrl Pts',(15.6998079270965,-64.5631281466306,13.0243480143334));
#36651=CARTESIAN_POINT('Ctrl Pts',(18.7531593329025,-63.5831391481621,12.9642768465754));
#36652=CARTESIAN_POINT('Ctrl Pts',(20.3819538620282,-62.9848590143723,10.2668649288348));
#36653=CARTESIAN_POINT('Ctrl Pts',(19.1010411238773,-63.1662325930602,7.33202115613798));
#36654=CARTESIAN_POINT('Ctrl Pts',(16.0140604868501,-63.8315406067279,6.77089943660167));
#36655=CARTESIAN_POINT('Ctrl Pts',(13.8315243325383,-64.254503451653,9.08273423965024));
#36656=CARTESIAN_POINT('Ctrl Pts',(14.4592535720066,-63.9244579537978,12.210667703652));
#36657=CARTESIAN_POINT('Ctrl Pts',(17.3027535879932,-63.000698465762,13.3717524842076));
#36658=CARTESIAN_POINT('Ctrl Pts',(19.7961408267282,-62.1707514136505,11.5329621876411));
#36659=CARTESIAN_POINT('Ctrl Pts',(19.6850298779915,-62.0386775475604,8.33028321499209));
#36660=CARTESIAN_POINT('Ctrl Pts',(17.0322781112101,-62.5876342861154,6.61316456701221));
#36661=CARTESIAN_POINT('Ctrl Pts',(14.1620610563238,-63.1948606729999,7.90934044152622));
#36662=CARTESIAN_POINT('Ctrl Pts',(13.5920347304658,-63.1857528116036,11.0655927384794));
#36663=CARTESIAN_POINT('Ctrl Pts',(15.7933573470831,-62.4340642391264,13.273778797971));
#36664=CARTESIAN_POINT('Ctrl Pts',(18.7714953959895,-61.4742285988991,12.5692575108707));
#36665=CARTESIAN_POINT('Ctrl Pts',(19.8407774342272,-61.0258693851979,9.57884782055452));
#36666=CARTESIAN_POINT('Ctrl Pts',(18.0138545011772,-61.3535459546681,6.96313958196516));
#36667=CARTESIAN_POINT('Ctrl Pts',(14.8801582185984,-62.0313713878353,7.04935230673882));
#36668=CARTESIAN_POINT('Ctrl Pts',(13.1917589144664,-62.3219306628043,9.76077569049498));
#36669=CARTESIAN_POINT('Ctrl Pts',(14.4148508351996,-61.8323582153005,12.6850472214475));
#36670=CARTESIAN_POINT('Ctrl Pts',(17.4252184513762,-60.8638866885509,13.2203938343513));
#36671=CARTESIAN_POINT('Ctrl Pts',(19.5085594056783,-60.1438112072126,10.8905648652627));
#36672=CARTESIAN_POINT('Ctrl Pts',(18.775219140647,-60.1784631839306,7.7683232146435));
#36673=CARTESIAN_POINT('Ctrl Pts',(15.8418413120583,-60.8026134491219,6.63176432830724));
#36674=CARTESIAN_POINT('Ctrl Pts',(13.2819033927537,-61.3267007921991,8.49166306428506));
#36675=CARTESIAN_POINT('Ctrl Pts',(13.3377613540647,-61.1498877415006,11.6941269021445));
#36676=CARTESIAN_POINT('Ctrl Pts',(15.9221807830298,-60.2955486875318,13.3881230626288));
#36677=CARTESIAN_POINT('Ctrl Pts',(18.7029087844679,-59.3886089101015,12.0701056758008));
#36678=CARTESIAN_POINT('Ctrl Pts',(19.1635205297874,-59.1033424098446,8.90528539980922));
#36679=CARTESIAN_POINT('Ctrl Pts',(17.635518731718,-59.4048719542876,7.45405522397582));
#36680=CARTESIAN_POINT('Ctrl Pts',(16.7396023849073,-59.5909833642099,7.20982243015787));
#36681=CARTESIAN_POINT('Ctrl Pts',(20.8181659539443,-67.1867480491087,11.4318553561533));
#36682=CARTESIAN_POINT('Ctrl Pts',(21.2575212792675,-67.0150744928066,10.5414078043456));
#36683=CARTESIAN_POINT('Ctrl Pts',(21.2188117961245,-66.9175493641713,8.27875481372736));
#36684=CARTESIAN_POINT('Ctrl Pts',(18.4270343173438,-67.5037579299837,6.39877704863433));
#36685=CARTESIAN_POINT('Ctrl Pts',(15.3541534373018,-68.1652879251536,7.72993286626466));
#36686=CARTESIAN_POINT('Ctrl Pts',(14.6971341869088,-68.1794897476338,11.0773387007931));
#36687=CARTESIAN_POINT('Ctrl Pts',(17.0050066526373,-67.3992512291335,13.4679206448302));
#36688=CARTESIAN_POINT('Ctrl Pts',(20.1882099452846,-66.3844685224502,12.7722321938661));
#36689=CARTESIAN_POINT('Ctrl Pts',(21.3787366757643,-65.9036218913761,9.6104773635602));
#36690=CARTESIAN_POINT('Ctrl Pts',(19.4813112170045,-66.2501895556748,6.79508159949539));
#36691=CARTESIAN_POINT('Ctrl Pts',(16.1481166073794,-66.9814704044651,6.83122696910054));
#36692=CARTESIAN_POINT('Ctrl Pts',(14.3087102716975,-67.3124918915897,9.68660587073265));
#36693=CARTESIAN_POINT('Ctrl Pts',(15.5636344323565,-66.8143900211043,12.8208382184198));
#36694=CARTESIAN_POINT('Ctrl Pts',(18.7603708726992,-65.795981118425,13.4453363911883));
#36695=CARTESIAN_POINT('Ctrl Pts',(21.0187603927389,-65.0290015152611,11.0044971721499));
#36696=CARTESIAN_POINT('Ctrl Pts',(20.2934961228731,-65.0614895355965,7.66994591646104));
#36697=CARTESIAN_POINT('Ctrl Pts',(17.1938529499357,-65.7301904655353,6.40846378494577));
#36698=CARTESIAN_POINT('Ctrl Pts',(14.4416090212989,-66.3058060485126,8.34239936321361));
#36699=CARTESIAN_POINT('Ctrl Pts',(14.4494588941473,-66.141856726348,11.7511157925381));
#36700=CARTESIAN_POINT('Ctrl Pts',(17.1744195179845,-65.2498597727098,13.6018503664189));
#36701=CARTESIAN_POINT('Ctrl Pts',(20.1560728090925,-64.2890822261735,12.2479900298273));
#36702=CARTESIAN_POINT('Ctrl Pts',(20.7056191362412,-63.9799857765361,8.89407499549286));
#36703=CARTESIAN_POINT('Ctrl Pts',(18.2981238461184,-64.463226240232,6.52411027736642));
#36704=CARTESIAN_POINT('Ctrl Pts',(15.0395557852222,-65.1745109655565,7.24667235432871));
#36705=CARTESIAN_POINT('Ctrl Pts',(13.7930900353155,-65.3466545015629,10.4188919993335));
#36706=CARTESIAN_POINT('Ctrl Pts',(15.6317182042724,-64.6921496134353,13.2184200895794));
#36707=CARTESIAN_POINT('Ctrl Pts',(18.8835992389529,-63.6589647612363,13.1544941616768));
#36708=CARTESIAN_POINT('Ctrl Pts',(20.6195097408352,-63.0319829890498,10.2839896215964));
#36709=CARTESIAN_POINT('Ctrl Pts',(19.2589973841654,-63.2346852212378,7.16081725087081));
#36710=CARTESIAN_POINT('Ctrl Pts',(15.9765219526975,-63.9523759072003,6.56368841308624));
#36711=CARTESIAN_POINT('Ctrl Pts',(13.6565291056692,-64.4121701619331,9.02387339796815));
#36712=CARTESIAN_POINT('Ctrl Pts',(14.3271360697494,-64.0706356123948,12.3525260039844));
#36713=CARTESIAN_POINT('Ctrl Pts',(17.3556995742979,-63.0972885120504,13.5881174655936));
#36714=CARTESIAN_POINT('Ctrl Pts',(20.0116836036718,-62.2237737811953,11.6313322004899));
#36715=CARTESIAN_POINT('Ctrl Pts',(19.8960390869576,-62.0929146809836,8.22313767486115));
#36716=CARTESIAN_POINT('Ctrl Pts',(17.0756569439772,-62.6867878434681,6.39583171448279));
#36717=CARTESIAN_POINT('Ctrl Pts',(14.0238547895744,-63.3426698111255,7.77518305050405));
#36718=CARTESIAN_POINT('Ctrl Pts',(13.4198463471001,-63.3426674304337,11.1339717058283));
#36719=CARTESIAN_POINT('Ctrl Pts',(15.7650240000835,-62.5524330171349,13.483856818823));
#36720=CARTESIAN_POINT('Ctrl Pts',(18.9368652451291,-61.5406947619309,12.7341264791948));
#36721=CARTESIAN_POINT('Ctrl Pts',(20.0773594018982,-61.0732543185779,9.5518225321049));
#36722=CARTESIAN_POINT('Ctrl Pts',(18.135799436934,-61.4316477881723,6.76826458716716));
#36723=CARTESIAN_POINT('Ctrl Pts',(14.8036106221423,-62.1626591350494,6.86000957288767));
#36724=CARTESIAN_POINT('Ctrl Pts',(13.0094633319359,-62.4815534974883,9.74542469319742));
#36725=CARTESIAN_POINT('Ctrl Pts',(14.3136373342298,-61.9702551717097,12.8573464026033));
#36726=CARTESIAN_POINT('Ctrl Pts',(17.5197763142877,-60.9493268661069,13.4270461480335));
#36727=CARTESIAN_POINT('Ctrl Pts',(19.7394014348253,-60.1927341524847,10.9477123134808));
#36728=CARTESIAN_POINT('Ctrl Pts',(18.9615992158899,-60.2392996738452,7.62511676387795));
#36729=CARTESIAN_POINT('Ctrl Pts',(15.8425832679706,-60.9131915231956,6.41562502038857));
#36730=CARTESIAN_POINT('Ctrl Pts',(13.1209708267227,-61.4805994238643,8.39487325110976));
#36731=CARTESIAN_POINT('Ctrl Pts',(13.1830095964177,-61.3021302305506,11.8028388367734));
#36732=CARTESIAN_POINT('Ctrl Pts',(15.9358673415304,-60.4026582657957,13.6055385422089));
#36733=CARTESIAN_POINT('Ctrl Pts',(18.8976307583479,-59.4472101950129,12.2029441264609));
#36734=CARTESIAN_POINT('Ctrl Pts',(19.3903963172922,-59.1533281063617,8.83503768583773));
#36735=CARTESIAN_POINT('Ctrl Pts',(17.7660737535057,-59.480666722193,7.29068223125039));
#36736=CARTESIAN_POINT('Ctrl Pts',(16.8135320242446,-59.681950857614,7.03077704625433));
#36737=CARTESIAN_POINT('Ctrl Pts',(20.25986904378,-67.0040126136404,11.1728309286208));
#36738=CARTESIAN_POINT('Ctrl Pts',(20.4203000043805,-66.9555034255254,10.9082027524038));
#36739=CARTESIAN_POINT('Ctrl Pts',(20.5332184525385,-66.9207835851305,10.6149904639443));
#36740=CARTESIAN_POINT('Ctrl Pts',(20.6611539455099,-66.8813975908017,9.99178401342259));
#36741=CARTESIAN_POINT('Ctrl Pts',(20.6720025707686,-66.8780249511107,9.66515229429175));
#36742=CARTESIAN_POINT('Ctrl Pts',(20.5855924444283,-66.904675210205,9.0009848649648));
#36743=CARTESIAN_POINT('Ctrl Pts',(20.4815398383751,-66.9367881932439,8.66883374311742));
#36744=CARTESIAN_POINT('Ctrl Pts',(20.1690707048657,-67.0315956493191,8.06423785428596));
#36745=CARTESIAN_POINT('Ctrl Pts',(19.9644265611133,-67.09312085238,7.79496359360541));
#36746=CARTESIAN_POINT('Ctrl Pts',(19.4553169386786,-67.2425937581436,7.32570054462934));
#36747=CARTESIAN_POINT('Ctrl Pts',(19.148781829213,-67.33085397004,7.13688275745718));
#36748=CARTESIAN_POINT('Ctrl Pts',(18.8154792730625,-67.4238662472344,7.01293629783558));
#36749=CARTESIAN_POINT('Ctrl Pts',(15.2652009106025,-66.709565290414,9.99881345470574));
#36750=CARTESIAN_POINT('Ctrl Pts',(15.2659775128488,-66.7141255555458,9.92620926472465));
#36751=CARTESIAN_POINT('Ctrl Pts',(15.2699455778512,-66.7178306708093,9.85363960672275));
#36752=CARTESIAN_POINT('Ctrl Pts',(15.2772137473688,-66.7206515257331,9.78136734601486));
#36753=CARTESIAN_POINT('Ctrl Pts',(15.3594450282717,-66.752566372114,8.9636868341033));
#36754=CARTESIAN_POINT('Ctrl Pts',(15.8641033480846,-66.6712922345579,8.18407440691835));
#36755=CARTESIAN_POINT('Ctrl Pts',(16.5726883518979,-66.5353761067088,7.78933375549815));
#36756=CARTESIAN_POINT('Ctrl Pts',(17.2812733557112,-66.3994599788597,7.39459310407796));
#36757=CARTESIAN_POINT('Ctrl Pts',(18.1937850435249,-66.2089018607175,7.38472422842252));
#36758=CARTESIAN_POINT('Ctrl Pts',(18.9102906125108,-66.0708634238267,7.76413764787115));
#36759=CARTESIAN_POINT('Ctrl Pts',(19.6267961814968,-65.932824986936,8.14355106731979));
#36760=CARTESIAN_POINT('Ctrl Pts',(20.1472956316549,-65.8473062312967,8.91224678187249));
#36761=CARTESIAN_POINT('Ctrl Pts',(20.246238786796,-65.8747431444716,9.72822620930746));
#36762=CARTESIAN_POINT('Ctrl Pts',(20.345181941937,-65.9021800576464,10.5442056367424));
#36763=CARTESIAN_POINT('Ctrl Pts',(20.0225688020609,-66.0425726396352,11.4074687770597));
#36764=CARTESIAN_POINT('Ctrl Pts',(19.4279225161919,-66.2558562834075,11.9340732703408));
#36765=CARTESIAN_POINT('Ctrl Pts',(18.8332762303228,-66.4691399271797,12.4606777636219));
#36766=CARTESIAN_POINT('Ctrl Pts',(17.9665967984607,-66.7553146327353,12.6506236098669));
#36767=CARTESIAN_POINT('Ctrl Pts',(17.2194144305739,-67.0094701965008,12.4192427536872));
#36768=CARTESIAN_POINT('Ctrl Pts',(16.4722320626871,-67.2636257602663,12.1878618975074));
#36769=CARTESIAN_POINT('Ctrl Pts',(15.8445467587756,-67.4857621822417,11.5351543389028));
#36770=CARTESIAN_POINT('Ctrl Pts',(15.6216179699845,-67.5994444228593,10.7518245719412));
#36771=CARTESIAN_POINT('Ctrl Pts',(15.5528913979792,-67.6344914472383,10.5103323450966));
#36772=CARTESIAN_POINT('Ctrl Pts',(15.5226338262371,-67.6592307340631,10.2564254798708));
#36773=CARTESIAN_POINT('Ctrl Pts',(15.5286491313886,-67.6742507328171,10.0019962882658));
#36774=CARTESIAN_POINT('Ctrl Pts',(16.8135320242446,-59.681950857614,7.03077704625433));
#36775=CARTESIAN_POINT('Ctrl Pts',(16.9051481187087,-59.6574023990886,7.06547285383011));
#36776=CARTESIAN_POINT('Ctrl Pts',(16.9947948727223,-59.6333816237466,7.10515219318068));
#36777=CARTESIAN_POINT('Ctrl Pts',(17.082237786682,-59.6099513655673,7.14949694326817));
#36778=CARTESIAN_POINT('Ctrl Pts',(17.1708871306384,-59.5861978454446,7.19445350778722));
#36779=CARTESIAN_POINT('Ctrl Pts',(17.257272050493,-59.5630510759314,7.2442058054096));
#36780=CARTESIAN_POINT('Ctrl Pts',(17.3411153578246,-59.5405853294411,7.29846300340358));
#36781=CARTESIAN_POINT('Ctrl Pts',(17.3650399830487,-59.5341747454331,7.31394525439086));
#36782=CARTESIAN_POINT('Ctrl Pts',(17.3887574233665,-59.5278196764534,7.32979452698956));
#36783=CARTESIAN_POINT('Ctrl Pts',(17.4122606427146,-59.5215220078096,7.34600453500901));
#36784=CARTESIAN_POINT('Ctrl Pts',(17.4307316092674,-59.5165727272383,7.35874383303933));
#36785=CARTESIAN_POINT('Ctrl Pts',(17.4490721037676,-59.5116584065482,7.37170741304488));
#36786=CARTESIAN_POINT('Ctrl Pts',(17.4672605740137,-59.5067848206342,7.38487881928224));
#36787=CARTESIAN_POINT('Ctrl Pts',(17.5471418516652,-59.4853806967971,7.4427258368968));
#36788=CARTESIAN_POINT('Ctrl Pts',(17.6241706060797,-59.4647409042578,7.50463022536142));
#36789=CARTESIAN_POINT('Ctrl Pts',(17.6980879988856,-59.4449347985488,7.57029723839113));
#36790=CARTESIAN_POINT('Ctrl Pts',(17.7541980617666,-59.4299001525126,7.62014450830199));
#36791=CARTESIAN_POINT('Ctrl Pts',(17.808514662402,-59.4153460632368,7.67216077851682));
#36792=CARTESIAN_POINT('Ctrl Pts',(17.8609084969736,-59.4013071775749,7.72622830914027));
#36793=CARTESIAN_POINT('Ctrl Pts',(17.887929214397,-59.3940669981624,7.75411219049193));
#36794=CARTESIAN_POINT('Ctrl Pts',(17.9144382908043,-59.386963912547,7.78254178039818));
#36795=CARTESIAN_POINT('Ctrl Pts',(17.9404163406947,-59.3800031150579,7.81150163987195));
#36796=CARTESIAN_POINT('Ctrl Pts',(17.9513656352696,-59.3770692604189,7.82370771513786));
#36797=CARTESIAN_POINT('Ctrl Pts',(17.9622216783077,-59.3741603924538,7.83600935553802));
#36798=CARTESIAN_POINT('Ctrl Pts',(17.9729722066068,-59.3712797970779,7.84839276276143));
#36799=CARTESIAN_POINT('Ctrl Pts',(18.0365635528686,-59.3542405472014,7.9216428872886));
#36800=CARTESIAN_POINT('Ctrl Pts',(18.0965497610003,-59.3381672911755,7.99784282323338));
#36801=CARTESIAN_POINT('Ctrl Pts',(18.1526942045728,-59.3231234328608,8.07671631116857));
#36802=CARTESIAN_POINT('Ctrl Pts',(18.2078226719183,-59.3083518045556,8.15416252360535));
#36803=CARTESIAN_POINT('Ctrl Pts',(18.2592474979931,-59.2945725639379,8.23418719299189));
#36804=CARTESIAN_POINT('Ctrl Pts',(18.306701932207,-59.281857186613,8.3165506094164));
#36805=CARTESIAN_POINT('Ctrl Pts',(18.3532560644286,-59.2693830444799,8.39735143323749));
#36806=CARTESIAN_POINT('Ctrl Pts',(18.3959893039731,-59.257932707454,8.48040377572554));
#36807=CARTESIAN_POINT('Ctrl Pts',(18.4346037832467,-59.2475859889165,8.56549184002203));
#36808=CARTESIAN_POINT('Ctrl Pts',(18.4539341349641,-59.2424064367844,8.60808680027398));
#36809=CARTESIAN_POINT('Ctrl Pts',(18.4722315774893,-59.2375036518362,8.65119201445444));
#36810=CARTESIAN_POINT('Ctrl Pts',(18.4894539567762,-59.2328889292146,8.69478065000367));
#36811=CARTESIAN_POINT('Ctrl Pts',(18.4977385366612,-59.2306690827247,8.71574834135866));
#36812=CARTESIAN_POINT('Ctrl Pts',(18.5057743024797,-59.2285159057631,8.73682789347791));
#36813=CARTESIAN_POINT('Ctrl Pts',(18.5135562806062,-59.2264307310086,8.75801630574046));
#36814=CARTESIAN_POINT('Ctrl Pts',(18.5185237400553,-59.2250997042608,8.77154147594721));
#36815=CARTESIAN_POINT('Ctrl Pts',(18.5233877588239,-59.2237963943598,8.78511114924033));
#36816=CARTESIAN_POINT('Ctrl Pts',(18.5281423789793,-59.2225223977288,8.79871063662932));
#36817=CARTESIAN_POINT('Ctrl Pts',(18.5587083682319,-59.2143322655927,8.88613755440161));
#36818=CARTESIAN_POINT('Ctrl Pts',(18.5848098578286,-59.207338392534,8.97493705334007));
#36819=CARTESIAN_POINT('Ctrl Pts',(18.6062022975288,-59.2016063055922,9.06488740567675));
#36820=CARTESIAN_POINT('Ctrl Pts',(18.6087806599844,-59.2009154354544,9.07572883445171));
#36821=CARTESIAN_POINT('Ctrl Pts',(18.6112905562915,-59.2002429107659,9.08658699313079));
#36822=CARTESIAN_POINT('Ctrl Pts',(18.6137315088206,-59.199588859507,9.09746150181113));
#36823=CARTESIAN_POINT('Ctrl Pts',(18.6343037125501,-59.1940765541311,9.18911121861902));
#36824=CARTESIAN_POINT('Ctrl Pts',(18.6499830153446,-59.1898752976094,9.28192246232578));
#36825=CARTESIAN_POINT('Ctrl Pts',(18.6608728938762,-59.1869573634512,9.37550443036849));
#36826=CARTESIAN_POINT('Ctrl Pts',(18.672143984606,-59.1839372837923,9.47236233832657));
#36827=CARTESIAN_POINT('Ctrl Pts',(18.678284396888,-59.1822919652802,9.57004704527406));
#36828=CARTESIAN_POINT('Ctrl Pts',(18.6793547107854,-59.1820051755357,9.66811274307749));
#36829=CARTESIAN_POINT('Ctrl Pts',(18.679876498809,-59.1818653628562,9.71592068686325));
#36830=CARTESIAN_POINT('Ctrl Pts',(18.6791925043488,-59.1820486386194,9.76381888086314));
#36831=CARTESIAN_POINT('Ctrl Pts',(18.6773054175282,-59.182554282009,9.81175333277687));
#36832=CARTESIAN_POINT('Ctrl Pts',(18.6767477018728,-59.1827037214685,9.82592003352112));
#36833=CARTESIAN_POINT('Ctrl Pts',(18.6760848075141,-59.1828813434766,9.84008999100378));
#36834=CARTESIAN_POINT('Ctrl Pts',(18.6753177565931,-59.1830868741514,9.85424725645943));
#36835=CARTESIAN_POINT('Ctrl Pts',(18.6702850237357,-59.1844353908563,9.94713513791762));
#36836=CARTESIAN_POINT('Ctrl Pts',(18.660767260643,-59.1869856677907,10.039633649145));
#36837=CARTESIAN_POINT('Ctrl Pts',(18.6468763518991,-59.1907077255708,10.1313703607271));
#36838=CARTESIAN_POINT('Ctrl Pts',(18.633025285787,-59.1944191075498,10.2228439482696));
#36839=CARTESIAN_POINT('Ctrl Pts',(18.6148257395458,-59.1992956612678,10.3135610431858));
#36840=CARTESIAN_POINT('Ctrl Pts',(18.5923417342414,-59.2053202323317,10.4031353906328));
#36841=CARTESIAN_POINT('Ctrl Pts',(18.5702449117701,-59.2112410580682,10.4911672349027));
#36842=CARTESIAN_POINT('Ctrl Pts',(18.544009480218,-59.2182708207657,10.5780961319276));
#36843=CARTESIAN_POINT('Ctrl Pts',(18.5136570926348,-59.2264037185069,10.6635263253263));
#36844=CARTESIAN_POINT('Ctrl Pts',(18.499101256118,-59.2303039431468,10.7044953570147));
#36845=CARTESIAN_POINT('Ctrl Pts',(18.4835980629778,-59.2344580112288,10.7451192119765));
#36846=CARTESIAN_POINT('Ctrl Pts',(18.4671470633348,-59.2388660432978,10.7853510160082));
#36847=CARTESIAN_POINT('Ctrl Pts',(18.4616118760651,-59.2403491922567,10.7988876140478));
#36848=CARTESIAN_POINT('Ctrl Pts',(18.455969374247,-59.2418610960621,10.8123798087171));
#36849=CARTESIAN_POINT('Ctrl Pts',(18.4502194972982,-59.2434017709471,10.8258257522335));
#36850=CARTESIAN_POINT('Ctrl Pts',(18.4447502513563,-59.2448672509805,10.8386154471551));
#36851=CARTESIAN_POINT('Ctrl Pts',(18.4391855696994,-59.2463583029366,10.8513591677142));
#36852=CARTESIAN_POINT('Ctrl Pts',(18.4335294175004,-59.2478738643506,10.864047091407));
#36853=CARTESIAN_POINT('Ctrl Pts',(18.3974943892325,-59.2575294210742,10.9448811412784));
#36854=CARTESIAN_POINT('Ctrl Pts',(18.3577058350311,-59.2681907320404,11.0235565035315));
#36855=CARTESIAN_POINT('Ctrl Pts',(18.3142251103267,-59.2798413571113,11.0997253732369));
#36856=CARTESIAN_POINT('Ctrl Pts',(18.2714642927549,-59.2912990836474,11.1746331206183));
#36857=CARTESIAN_POINT('Ctrl Pts',(18.2251321272566,-59.3037137499762,11.2471173606622));
#36858=CARTESIAN_POINT('Ctrl Pts',(18.1752516289959,-59.3170791892032,11.3168132015522));
#36859=CARTESIAN_POINT('Ctrl Pts',(18.1268143228897,-59.330057926258,11.3844925330993));
#36860=CARTESIAN_POINT('Ctrl Pts',(18.0750306258251,-59.3439333260675,11.4495429414388));
#36861=CARTESIAN_POINT('Ctrl Pts',(18.0198942246886,-59.3587070802256,11.5115898438695));
#36862=CARTESIAN_POINT('Ctrl Pts',(18.0099245352413,-59.3613784504618,11.52280908081));
#36863=CARTESIAN_POINT('Ctrl Pts',(17.9998451629738,-59.364079210121,11.5339299972363));
#36864=CARTESIAN_POINT('Ctrl Pts',(17.9896559870012,-59.3668093915945,11.5449502145346));
#36865=CARTESIAN_POINT('Ctrl Pts',(17.9601614990779,-59.3747124158147,11.576850308015));
#36866=CARTESIAN_POINT('Ctrl Pts',(17.9297469672236,-59.3828619650632,11.6079068412472));
#36867=CARTESIAN_POINT('Ctrl Pts',(17.8984546702662,-59.3912467107622,11.6380966037224));
#36868=CARTESIAN_POINT('Ctrl Pts',(15.0750265266586,-68.1281291851066,10.0024371765581));
#36869=CARTESIAN_POINT('Ctrl Pts',(15.0686010168709,-68.1132191003537,10.3130580784043));
#36870=CARTESIAN_POINT('Ctrl Pts',(15.229260839257,-67.9995899840862,11.6285356953996));
#36871=CARTESIAN_POINT('Ctrl Pts',(17.0050066526373,-67.3992512291335,13.4679206448302));
#36872=CARTESIAN_POINT('Ctrl Pts',(20.1882099452846,-66.3844685224502,12.7722321938661));
#36873=CARTESIAN_POINT('Ctrl Pts',(21.3787366757643,-65.9036218913761,9.6104773635602));
#36874=CARTESIAN_POINT('Ctrl Pts',(19.4813112170045,-66.2501895556748,6.79508159949539));
#36875=CARTESIAN_POINT('Ctrl Pts',(16.1481166073794,-66.9814704044651,6.83122696910054));
#36876=CARTESIAN_POINT('Ctrl Pts',(14.8676525643411,-67.2119040522751,8.81893895087676));
#36877=CARTESIAN_POINT('Ctrl Pts',(14.8112407741816,-67.1683025391241,9.90991228406403));
#36878=CARTESIAN_POINT('Ctrl Pts',(14.810555933805,-67.1637176864735,9.99855140140538));
#36879=CARTESIAN_POINT('Origin',(18.6889152049569,-69.7479810832458,10.));
#36880=CARTESIAN_POINT('Ctrl Pts',(15.0969161422106,-68.2083503098983,9.99673640007585));
#36881=CARTESIAN_POINT('Ctrl Pts',(15.0927295232038,-68.1711103559359,10.7130675867));
#36882=CARTESIAN_POINT('Ctrl Pts',(15.6514186592595,-67.9289066052254,12.4513417391716));
#36883=CARTESIAN_POINT('Ctrl Pts',(18.3902480628713,-67.0483943376965,13.5944453497599));
#36884=CARTESIAN_POINT('Ctrl Pts',(21.0667649555471,-66.1687987195556,11.6442225433397));
#36885=CARTESIAN_POINT('Ctrl Pts',(20.9561469803459,-66.036013638459,8.22016494780579));
#36886=CARTESIAN_POINT('Ctrl Pts',(18.1194957904382,-66.6336669557833,6.39071567224368));
#36887=CARTESIAN_POINT('Ctrl Pts',(15.4027596845032,-67.2173089746449,7.63681194520568));
#36888=CARTESIAN_POINT('Ctrl Pts',(14.8518622987657,-67.2747579502335,9.32892113065756));
#36889=CARTESIAN_POINT('Ctrl Pts',(14.8383776097513,-67.242349320473,10.0022118830713));
#36890=CARTESIAN_POINT('Ctrl Pts',(17.244983442153,-67.8425423025985,7.06170475438608));
#36891=CARTESIAN_POINT('Ctrl Pts',(16.2988495743024,-68.0419164156808,7.35795147289589));
#36892=CARTESIAN_POINT('Ctrl Pts',(14.725851572522,-68.3551165744735,8.97144797270218));
#36893=CARTESIAN_POINT('Ctrl Pts',(15.3567034243025,-68.0236552520251,12.3283366156213));
#36894=CARTESIAN_POINT('Ctrl Pts',(18.3902480628713,-67.0483943376965,13.5944453497599));
#36895=CARTESIAN_POINT('Ctrl Pts',(21.0667649555471,-66.1687987195556,11.6442225433397));
#36896=CARTESIAN_POINT('Ctrl Pts',(20.9561469803459,-66.036013638459,8.22016494780579));
#36897=CARTESIAN_POINT('Ctrl Pts',(18.1194957904382,-66.6336669557833,6.39071567224368));
#36898=CARTESIAN_POINT('Ctrl Pts',(15.0616295968133,-67.2905946547074,7.79327945411719));
#36899=CARTESIAN_POINT('Ctrl Pts',(14.4843023646232,-67.282863942121,11.1722569386416));
#36900=CARTESIAN_POINT('Ctrl Pts',(16.868372167434,-66.4816292855382,13.5013274912989));
#36901=CARTESIAN_POINT('Ctrl Pts',(20.0422978199459,-65.468753391891,12.6947822329673));
#36902=CARTESIAN_POINT('Ctrl Pts',(21.1273143736846,-65.0155990043222,9.47487431060689));
#36903=CARTESIAN_POINT('Ctrl Pts',(19.1153342996381,-65.3922823621302,6.72525821930947));
#36904=CARTESIAN_POINT('Ctrl Pts',(15.7718556315866,-66.1257396929252,6.90837057311361));
#36905=CARTESIAN_POINT('Ctrl Pts',(14.0547985877671,-66.4233986629546,9.86022990097492));
#36906=CARTESIAN_POINT('Ctrl Pts',(15.4655309000317,-65.8829690009266,12.9372608391342));
#36907=CARTESIAN_POINT('Ctrl Pts',(18.7042880702649,-64.8527215544619,13.3837942299379));
#36908=CARTESIAN_POINT('Ctrl Pts',(20.8341986998846,-64.1195886430847,10.7999310727631));
#36909=CARTESIAN_POINT('Ctrl Pts',(19.9114308093213,-64.2044184759422,7.49968047567758));
#36910=CARTESIAN_POINT('Ctrl Pts',(16.7260146593053,-64.895523082676,6.43862003923502));
#36911=CARTESIAN_POINT('Ctrl Pts',(14.0943212306268,-65.4382581333965,8.56699487612852));
#36912=CARTESIAN_POINT('Ctrl Pts',(14.3368288007655,-65.2108533475991,11.9787141005062));
#36913=CARTESIAN_POINT('Ctrl Pts',(17.1999914587379,-64.2812461473763,13.6183729089162));
#36914=CARTESIAN_POINT('Ctrl Pts',(20.0833051820056,-63.346239485481,12.017555775347));
#36915=CARTESIAN_POINT('Ctrl Pts',(20.3682194128848,-63.1074718691846,8.60989310618131));
#36916=CARTESIAN_POINT('Ctrl Pts',(17.7632104839249,-63.6430568297551,6.44715683087681));
#36917=CARTESIAN_POINT('Ctrl Pts',(14.564859018057,-64.3376274439251,7.46621057361502));
#36918=CARTESIAN_POINT('Ctrl Pts',(13.60112044902,-64.4334353369931,10.7544289031929));
#36919=CARTESIAN_POINT('Ctrl Pts',(15.6987166428558,-63.708961052588,13.3670096553836));
#36920=CARTESIAN_POINT('Ctrl Pts',(18.9427555175132,-62.6772983776882,12.9642257537709));
#36921=CARTESIAN_POINT('Ctrl Pts',(20.3916349158421,-62.1266472347557,9.9067950074971));
#36922=CARTESIAN_POINT('Ctrl Pts',(18.7114286257305,-62.4144320750886,6.93283507366396));
#36923=CARTESIAN_POINT('Ctrl Pts',(15.3704995140598,-63.1472062543102,6.70571036393745));
#36924=CARTESIAN_POINT('Ctrl Pts',(13.3244900809145,-63.5330077514078,9.42882503807144));
#36925=CARTESIAN_POINT('Ctrl Pts',(14.3693624549396,-63.090609964374,12.6634621126407));
#36926=CARTESIAN_POINT('Ctrl Pts',(17.5330036055456,-62.080489794707,13.5128046754735));
#36927=CARTESIAN_POINT('Ctrl Pts',(19.9458125081592,-61.2715545195409,11.2162142452876));
#36928=CARTESIAN_POINT('Ctrl Pts',(19.4106046411912,-61.2525379570576,7.83042882970036));
#36929=CARTESIAN_POINT('Ctrl Pts',(16.3703262829254,-61.9047530097005,6.3876284598802));
#36930=CARTESIAN_POINT('Ctrl Pts',(13.5113685232516,-62.5083833543796,8.17992871548479));
#36931=CARTESIAN_POINT('Ctrl Pts',(13.357739085696,-62.3871231598861,11.6022164308586));
#36932=CARTESIAN_POINT('Ctrl Pts',(16.0106566332716,-61.5138509672066,13.5896176377583));
#36933=CARTESIAN_POINT('Ctrl Pts',(19.0579057022675,-60.5349179618126,12.3623010109723));
#36934=CARTESIAN_POINT('Ctrl Pts',(19.734119272829,-60.1913020034494,9.01938609588904));
#36935=CARTESIAN_POINT('Ctrl Pts',(17.3973455890623,-60.6550135466889,6.55469600728483));
#36936=CARTESIAN_POINT('Ctrl Pts',(14.1039347737162,-61.3750552367845,7.17543798647161));
#36937=CARTESIAN_POINT('Ctrl Pts',(12.7669926495712,-61.5708627210562,10.3258507409624));
#36938=CARTESIAN_POINT('Ctrl Pts',(14.5474295567701,-60.9313710113775,13.1842383274677));
#36939=CARTESIAN_POINT('Ctrl Pts',(17.8144668208753,-59.8935459365978,13.1913616605739));
#36940=CARTESIAN_POINT('Ctrl Pts',(19.6057481548832,-59.2511484715134,10.3395770770155));
#36941=CARTESIAN_POINT('Ctrl Pts',(18.2810249486938,-59.4436819065863,7.18539898656541));
#36942=CARTESIAN_POINT('Ctrl Pts',(14.9896601306954,-60.1631753733452,6.54837069990781));
#36943=CARTESIAN_POINT('Ctrl Pts',(12.6441934312551,-60.629216203114,9.00969837718652));
#36944=CARTESIAN_POINT('Ctrl Pts',(13.0868379849885,-60.402326566927,11.2296927240265));
#36945=CARTESIAN_POINT('Ctrl Pts',(13.707234883037,-60.181950026368,11.9973015569304));
#36946=CARTESIAN_POINT('Ctrl Pts',(17.3251900988197,-67.9318278742783,7.23888518457547));
#36947=CARTESIAN_POINT('Ctrl Pts',(16.4352923065869,-68.1161335763132,7.51726810226197));
#36948=CARTESIAN_POINT('Ctrl Pts',(14.9555143577762,-68.4043554971943,9.03347008941793));
#36949=CARTESIAN_POINT('Ctrl Pts',(15.5458770044743,-68.0837432245499,12.1879369455073));
#36950=CARTESIAN_POINT('Ctrl Pts',(18.3940490596781,-67.1581527442329,13.3776987943165));
#36951=CARTESIAN_POINT('Ctrl Pts',(20.9067222911425,-66.3224589027986,11.5450752374347));
#36952=CARTESIAN_POINT('Ctrl Pts',(20.800326051025,-66.1885426111956,8.32748974461941));
#36953=CARTESIAN_POINT('Ctrl Pts',(18.1322775372971,-66.7410189775958,6.60835702425632));
#36954=CARTESIAN_POINT('Ctrl Pts',(15.256353376944,-67.3491954556355,7.92634562444536));
#36955=CARTESIAN_POINT('Ctrl Pts',(14.7113906429075,-67.3327927019053,11.1015693557681));
#36956=CARTESIAN_POINT('Ctrl Pts',(16.9492514661363,-66.5707346233278,13.2901959816018));
#36957=CARTESIAN_POINT('Ctrl Pts',(19.9293395015267,-65.609797362651,12.5322857391188));
#36958=CARTESIAN_POINT('Ctrl Pts',(20.9464805290194,-65.1748301675257,9.5065396089424));
#36959=CARTESIAN_POINT('Ctrl Pts',(19.0533751185266,-65.5196611552341,6.92272651604652));
#36960=CARTESIAN_POINT('Ctrl Pts',(15.9090610352118,-66.1997524963877,7.09479711845809));
#36961=CARTESIAN_POINT('Ctrl Pts',(14.2930946730788,-66.4703242998971,9.86865809630684));
#36962=CARTESIAN_POINT('Ctrl Pts',(15.6163106628564,-65.9533445658039,12.7601427840874));
#36963=CARTESIAN_POINT('Ctrl Pts',(18.6573208483792,-64.9760832641982,13.1797500249766));
#36964=CARTESIAN_POINT('Ctrl Pts',(20.6563484026839,-64.2780203671544,10.751694895066));
#36965=CARTESIAN_POINT('Ctrl Pts',(19.7867752262122,-64.3485967193296,7.65045078699729));
#36966=CARTESIAN_POINT('Ctrl Pts',(16.7909924250965,-64.9888892233674,6.65337273791571));
#36967=CARTESIAN_POINT('Ctrl Pts',(14.3155426340162,-65.489758917571,8.65340568344619));
#36968=CARTESIAN_POINT('Ctrl Pts',(14.5409783214077,-65.2669285289691,11.8593968140379));
#36969=CARTESIAN_POINT('Ctrl Pts',(17.2290425005878,-64.3842388247346,13.4001835116647));
#36970=CARTESIAN_POINT('Ctrl Pts',(19.9360426274117,-63.496475248621,11.8958963196675));
#36971=CARTESIAN_POINT('Ctrl Pts',(20.2013278361943,-63.2629672129436,8.69371713231473));
#36972=CARTESIAN_POINT('Ctrl Pts',(17.7509534583573,-63.7571179704187,6.66139475745698));
#36973=CARTESIAN_POINT('Ctrl Pts',(14.7430153463368,-64.4006674801972,7.61899913400437));
#36974=CARTESIAN_POINT('Ctrl Pts',(13.8349420404105,-64.4815599109683,10.7089365253202));
#36975=CARTESIAN_POINT('Ctrl Pts',(15.803603732902,-63.7916335220748,13.1639775672763));
#36976=CARTESIAN_POINT('Ctrl Pts',(18.8495771338669,-62.8130423308995,12.7854817031124));
#36977=CARTESIAN_POINT('Ctrl Pts',(20.2086399244908,-62.2864574754684,9.91241530746257));
#36978=CARTESIAN_POINT('Ctrl Pts',(18.6273022002302,-62.5477505634248,7.11778639941016));
#36979=CARTESIAN_POINT('Ctrl Pts',(15.4853839339819,-63.2271999473303,6.90435740451559));
#36980=CARTESIAN_POINT('Ctrl Pts',(13.5603011489528,-63.5805992467218,9.46326712676862));
#36981=CARTESIAN_POINT('Ctrl Pts',(14.5397187075307,-63.1557400246277,12.5028542351256));
#36982=CARTESIAN_POINT('Ctrl Pts',(17.5101424007745,-62.1973923166247,13.3009810867784));
#36983=CARTESIAN_POINT('Ctrl Pts',(19.775009344088,-61.4280979699796,11.1428760184691));
#36984=CARTESIAN_POINT('Ctrl Pts',(19.2696261599639,-61.4010899078139,7.96125487716922));
#36985=CARTESIAN_POINT('Ctrl Pts',(16.4102292811539,-62.0048379141108,6.60545597208742));
#36986=CARTESIAN_POINT('Ctrl Pts',(13.721219293131,-62.5629308906206,8.28967977390791));
#36987=CARTESIAN_POINT('Ctrl Pts',(13.5744051997984,-62.4398445301463,11.5056021110758));
#36988=CARTESIAN_POINT('Ctrl Pts',(16.0649021365259,-61.6100928089779,13.3731621953643));
#36989=CARTESIAN_POINT('Ctrl Pts',(18.9259522392798,-60.6810516662198,12.2198532736369));
#36990=CARTESIAN_POINT('Ctrl Pts',(19.5589412741757,-60.3490176872814,9.07851752376016));
#36991=CARTESIAN_POINT('Ctrl Pts',(17.3606274442457,-60.7756290245013,6.76244927662485));
#36992=CARTESIAN_POINT('Ctrl Pts',(14.2633621012124,-61.4431136936917,7.34576025527719));
#36993=CARTESIAN_POINT('Ctrl Pts',(13.0045895703814,-61.6179756985622,10.306201805224));
#36994=CARTESIAN_POINT('Ctrl Pts',(14.6752168136493,-61.0079073996549,12.9922274267495));
#36995=CARTESIAN_POINT('Ctrl Pts',(17.7428017915754,-60.0235254038855,12.9989212198951));
#36996=CARTESIAN_POINT('Ctrl Pts',(19.4236195381877,-59.4107265678368,10.3191004374818));
#36997=CARTESIAN_POINT('Ctrl Pts',(18.1763291194576,-59.5825119500423,7.35512060290615));
#36998=CARTESIAN_POINT('Ctrl Pts',(15.0809863992776,-60.249481453992,6.75650538792377));
#36999=CARTESIAN_POINT('Ctrl Pts',(12.8745037461489,-60.6782816207909,9.06941397854051));
#37000=CARTESIAN_POINT('Ctrl Pts',(13.2888242651274,-60.4589813868428,11.1555417393121));
#37001=CARTESIAN_POINT('Ctrl Pts',(13.8709947795085,-60.2488475749171,11.8768634390786));
#37002=CARTESIAN_POINT('Ctrl Pts',(17.4053967554863,-68.0211134459581,7.41606561476487));
#37003=CARTESIAN_POINT('Ctrl Pts',(16.5717350388713,-68.1903507369457,7.67658473162804));
#37004=CARTESIAN_POINT('Ctrl Pts',(15.1851771430305,-68.4535944199151,9.09549220613369));
#37005=CARTESIAN_POINT('Ctrl Pts',(15.7350505846462,-68.1438311970748,12.0475372753934));
#37006=CARTESIAN_POINT('Ctrl Pts',(18.397850056485,-67.2679111507693,13.160952238873));
#37007=CARTESIAN_POINT('Ctrl Pts',(20.7466796267378,-66.4761190860415,11.4459279315297));
#37008=CARTESIAN_POINT('Ctrl Pts',(20.6445051217041,-66.3410715839322,8.43481454143305));
#37009=CARTESIAN_POINT('Ctrl Pts',(18.145059284156,-66.8483709994082,6.82599837626894));
#37010=CARTESIAN_POINT('Ctrl Pts',(15.4510771570748,-67.4077962565635,8.05941179477353));
#37011=CARTESIAN_POINT('Ctrl Pts',(14.9384789211918,-67.3827214616897,11.0308817728946));
#37012=CARTESIAN_POINT('Ctrl Pts',(17.0301307648387,-66.6598399611173,13.0790644719047));
#37013=CARTESIAN_POINT('Ctrl Pts',(19.8163811831075,-65.7508413334111,12.3697892452703));
#37014=CARTESIAN_POINT('Ctrl Pts',(20.7656466843542,-65.3340613307291,9.53820490727791));
#37015=CARTESIAN_POINT('Ctrl Pts',(18.9914159374152,-65.6470399483378,7.12019481278356));
#37016=CARTESIAN_POINT('Ctrl Pts',(16.0462664388369,-66.2737652998505,7.28122366380257));
#37017=CARTESIAN_POINT('Ctrl Pts',(14.5313907583906,-66.5172499368395,9.87708629163875));
#37018=CARTESIAN_POINT('Ctrl Pts',(15.7670904256811,-66.0237201306814,12.5830247290407));
#37019=CARTESIAN_POINT('Ctrl Pts',(18.6103536264935,-65.0994449739343,12.9757058200154));
#37020=CARTESIAN_POINT('Ctrl Pts',(20.4784981054833,-64.4364520912242,10.7034587173689));
#37021=CARTESIAN_POINT('Ctrl Pts',(19.6621196431031,-64.492774962717,7.80122109831697));
#37022=CARTESIAN_POINT('Ctrl Pts',(16.8559701908879,-65.0822553640589,6.86812543659641));
#37023=CARTESIAN_POINT('Ctrl Pts',(14.5367640374054,-65.5412597017456,8.73981649076384));
#37024=CARTESIAN_POINT('Ctrl Pts',(14.7451278420499,-65.323003710339,11.7400795275695));
#37025=CARTESIAN_POINT('Ctrl Pts',(17.2580935424376,-64.4872315020928,13.1819941144132));
#37026=CARTESIAN_POINT('Ctrl Pts',(19.7887800728178,-63.6467110117609,11.774236863988));
#37027=CARTESIAN_POINT('Ctrl Pts',(20.0344362595038,-63.4184625567026,8.77754115844814));
#37028=CARTESIAN_POINT('Ctrl Pts',(17.7386964327898,-63.8711791110824,6.87563268403716));
#37029=CARTESIAN_POINT('Ctrl Pts',(14.9211716746167,-64.4637075164694,7.77178769439372));
#37030=CARTESIAN_POINT('Ctrl Pts',(14.068763631801,-64.5296844849434,10.6634441474475));
#37031=CARTESIAN_POINT('Ctrl Pts',(15.9084908229482,-63.8743059915618,12.960945479169));
#37032=CARTESIAN_POINT('Ctrl Pts',(18.7563987502206,-62.9487862841108,12.6067376524539));
#37033=CARTESIAN_POINT('Ctrl Pts',(20.0256449331395,-62.4462677161812,9.91803560742804));
#37034=CARTESIAN_POINT('Ctrl Pts',(18.5431757747299,-62.6810690517609,7.30273772515637));
#37035=CARTESIAN_POINT('Ctrl Pts',(15.6002683539039,-63.3071936403505,7.10300444509373));
#37036=CARTESIAN_POINT('Ctrl Pts',(13.7961122169911,-63.6281907420358,9.49770921546579));
#37037=CARTESIAN_POINT('Ctrl Pts',(14.7100749601219,-63.2208700848816,12.3422463576105));
#37038=CARTESIAN_POINT('Ctrl Pts',(17.4872811960032,-62.3142948385424,13.0891574980833));
#37039=CARTESIAN_POINT('Ctrl Pts',(19.6042061800168,-61.5846414204184,11.0695377916506));
#37040=CARTESIAN_POINT('Ctrl Pts',(19.1286476787365,-61.5496418585701,8.09208092463809));
#37041=CARTESIAN_POINT('Ctrl Pts',(16.4501322793825,-62.104922818521,6.82328348429462));
#37042=CARTESIAN_POINT('Ctrl Pts',(13.9310700630103,-62.6174784268616,8.39943083233104));
#37043=CARTESIAN_POINT('Ctrl Pts',(13.7910713139007,-62.4925659004067,11.408987791293));
#37044=CARTESIAN_POINT('Ctrl Pts',(16.1191476397801,-61.7063346507491,13.1567067529703));
#37045=CARTESIAN_POINT('Ctrl Pts',(18.7939987762921,-60.8271853706271,12.0774055363016));
#37046=CARTESIAN_POINT('Ctrl Pts',(19.3837632755223,-60.5067333711136,9.13764895163129));
#37047=CARTESIAN_POINT('Ctrl Pts',(17.3239092994291,-60.8962445023136,6.97020254596486));
#37048=CARTESIAN_POINT('Ctrl Pts',(14.4227894287085,-61.5111721505989,7.51608252408276));
#37049=CARTESIAN_POINT('Ctrl Pts',(13.2421864911916,-61.6650886760682,10.2865528694857));
#37050=CARTESIAN_POINT('Ctrl Pts',(14.8030040705286,-61.0844437879324,12.8002165260313));
#37051=CARTESIAN_POINT('Ctrl Pts',(17.6711367622755,-60.1535048711732,12.8064807792163));
#37052=CARTESIAN_POINT('Ctrl Pts',(19.2414909214922,-59.5703046641601,10.2986237979481));
#37053=CARTESIAN_POINT('Ctrl Pts',(18.0716332902214,-59.7213419934982,7.52484221924687));
#37054=CARTESIAN_POINT('Ctrl Pts',(15.1723126678598,-60.3357875346388,6.96464007593975));
#37055=CARTESIAN_POINT('Ctrl Pts',(13.1048140610427,-60.7273470384677,9.12912957989447));
#37056=CARTESIAN_POINT('Ctrl Pts',(13.4908105452663,-60.5156362067586,11.0813907545978));
#37057=CARTESIAN_POINT('Ctrl Pts',(14.0347546759799,-60.3157451234662,11.7564253212267));
#37058=CARTESIAN_POINT('Ctrl Pts',(17.485603412153,-68.1103990176379,7.59324604495427));
#37059=CARTESIAN_POINT('Ctrl Pts',(16.7081777711558,-68.2645678975782,7.83590136099411));
#37060=CARTESIAN_POINT('Ctrl Pts',(15.4148399282848,-68.502833342636,9.15751432284945));
#37061=CARTESIAN_POINT('Ctrl Pts',(15.924224164818,-68.2039191695996,11.9071376052795));
#37062=CARTESIAN_POINT('Ctrl Pts',(18.4016510532918,-67.3776695573057,12.9442056834295));
#37063=CARTESIAN_POINT('Ctrl Pts',(20.5866369623332,-66.6297792692845,11.3467806256248));
#37064=CARTESIAN_POINT('Ctrl Pts',(20.4886841923832,-66.4936005566688,8.54213933824665));
#37065=CARTESIAN_POINT('Ctrl Pts',(18.1578410310149,-66.9557230212208,7.04363972828159));
#37066=CARTESIAN_POINT('Ctrl Pts',(15.6458009372055,-67.4663970574915,8.19247796510169));
#37067=CARTESIAN_POINT('Ctrl Pts',(15.1655671994761,-67.432650221474,10.9601941900212));
#37068=CARTESIAN_POINT('Ctrl Pts',(17.111010063541,-66.7489452989068,12.8679329622076));
#37069=CARTESIAN_POINT('Ctrl Pts',(19.7034228646883,-65.8918853041711,12.2072927514219));
#37070=CARTESIAN_POINT('Ctrl Pts',(20.584812839689,-65.4932924939326,9.56987020561342));
#37071=CARTESIAN_POINT('Ctrl Pts',(18.9294567563037,-65.7744187414415,7.3176631095206));
#37072=CARTESIAN_POINT('Ctrl Pts',(16.1834718424621,-66.3477781033132,7.46765020914706));
#37073=CARTESIAN_POINT('Ctrl Pts',(14.7696868437023,-66.5641755737819,9.88551448697067));
#37074=CARTESIAN_POINT('Ctrl Pts',(15.9178701885058,-66.0940956955587,12.4059066739939));
#37075=CARTESIAN_POINT('Ctrl Pts',(18.5633864046078,-65.2228066836706,12.7716616150541));
#37076=CARTESIAN_POINT('Ctrl Pts',(20.3006478082827,-64.5948838152939,10.6552225396718));
#37077=CARTESIAN_POINT('Ctrl Pts',(19.5374640599939,-64.6369532061044,7.95199140963667));
#37078=CARTESIAN_POINT('Ctrl Pts',(16.9209479566792,-65.1756215047503,7.08287813527709));
#37079=CARTESIAN_POINT('Ctrl Pts',(14.7579854407948,-65.5927604859202,8.82622729808152));
#37080=CARTESIAN_POINT('Ctrl Pts',(14.9492773626922,-65.379078891709,11.6207622411012));
#37081=CARTESIAN_POINT('Ctrl Pts',(17.2871445842874,-64.5902241794511,12.9638047171617));
#37082=CARTESIAN_POINT('Ctrl Pts',(19.6415175182239,-63.796946774901,11.6525774083085));
#37083=CARTESIAN_POINT('Ctrl Pts',(19.8675446828133,-63.5739579004615,8.86136518458156));
#37084=CARTESIAN_POINT('Ctrl Pts',(17.7264394072222,-63.9852402517461,7.08987061061734));
#37085=CARTESIAN_POINT('Ctrl Pts',(15.0993280028965,-64.5267475527414,7.92457625478306));
#37086=CARTESIAN_POINT('Ctrl Pts',(14.3025852231916,-64.5778090589186,10.6179517695748));
#37087=CARTESIAN_POINT('Ctrl Pts',(16.0133779129944,-63.9569784610486,12.7579133910617));
#37088=CARTESIAN_POINT('Ctrl Pts',(18.6632203665742,-63.0845302373221,12.4279936017954));
#37089=CARTESIAN_POINT('Ctrl Pts',(19.8426499417882,-62.6060779568939,9.92365590739352));
#37090=CARTESIAN_POINT('Ctrl Pts',(18.4590493492297,-62.814387540097,7.48768905090255));
#37091=CARTESIAN_POINT('Ctrl Pts',(15.715152773826,-63.3871873333707,7.30165148567188));
#37092=CARTESIAN_POINT('Ctrl Pts',(14.0319232850294,-63.6757822373498,9.53215130416297));
#37093=CARTESIAN_POINT('Ctrl Pts',(14.8804312127131,-63.2860001451354,12.1816384800953));
#37094=CARTESIAN_POINT('Ctrl Pts',(17.4644199912321,-62.4311973604599,12.8773339093881));
#37095=CARTESIAN_POINT('Ctrl Pts',(19.4334030159456,-61.7411848708572,10.9961995648321));
#37096=CARTESIAN_POINT('Ctrl Pts',(18.9876691975092,-61.6981938093263,8.22290697210694));
#37097=CARTESIAN_POINT('Ctrl Pts',(16.490035277611,-62.2050077229313,7.04111099650184));
#37098=CARTESIAN_POINT('Ctrl Pts',(14.1409208328896,-62.6720259631026,8.50918189075418));
#37099=CARTESIAN_POINT('Ctrl Pts',(14.007737428003,-62.545287270667,11.3123734715102));
#37100=CARTESIAN_POINT('Ctrl Pts',(16.1733931430344,-61.8025764925203,12.9402513105764));
#37101=CARTESIAN_POINT('Ctrl Pts',(18.6620453133043,-60.9733190750343,11.9349577989662));
#37102=CARTESIAN_POINT('Ctrl Pts',(19.208585276869,-60.6644490549457,9.19678037950242));
#37103=CARTESIAN_POINT('Ctrl Pts',(17.2871911546125,-61.016859980126,7.17795581530488));
#37104=CARTESIAN_POINT('Ctrl Pts',(14.5822167562047,-61.5792306075061,7.68640479288833));
#37105=CARTESIAN_POINT('Ctrl Pts',(13.4797834120018,-61.7122016535741,10.2669039337474));
#37106=CARTESIAN_POINT('Ctrl Pts',(14.9307913274079,-61.1609801762098,12.6082056253131));
#37107=CARTESIAN_POINT('Ctrl Pts',(17.5994717329756,-60.2834843384609,12.6140403385374));
#37108=CARTESIAN_POINT('Ctrl Pts',(19.0593623047967,-59.7298827604835,10.2781471584144));
#37109=CARTESIAN_POINT('Ctrl Pts',(17.9669374609853,-59.8601720369542,7.69456383558757));
#37110=CARTESIAN_POINT('Ctrl Pts',(15.263638936442,-60.4220936152857,7.17277476395572));
#37111=CARTESIAN_POINT('Ctrl Pts',(13.3351243759366,-60.7764124561445,9.18884518124844));
#37112=CARTESIAN_POINT('Ctrl Pts',(13.6927968254053,-60.5722910266744,11.0072397698834));
#37113=CARTESIAN_POINT('Ctrl Pts',(14.1985145724514,-60.3826426720153,11.6359872033748));
#37114=CARTESIAN_POINT('Ctrl Pts',(17.244983442153,-67.8425423025985,7.06170475438607));
#37115=CARTESIAN_POINT('Ctrl Pts',(16.875980626074,-67.9363396049609,7.20780006417485));
#37116=CARTESIAN_POINT('Ctrl Pts',(16.5358040823886,-68.0195197262117,7.42431456480016));
#37117=CARTESIAN_POINT('Ctrl Pts',(15.9848167458476,-68.150998080649,7.95780764621775));
#37118=CARTESIAN_POINT('Ctrl Pts',(15.769941108176,-68.2006822338607,8.25968161903173));
#37119=CARTESIAN_POINT('Ctrl Pts',(15.4905619320039,-68.2646302810789,8.88066242679774));
#37120=CARTESIAN_POINT('Ctrl Pts',(15.410358466988,-68.2826595052327,9.184978201574));
#37121=CARTESIAN_POINT('Ctrl Pts',(15.358433741901,-68.2943569622715,9.79677072277292));
#37122=CARTESIAN_POINT('Ctrl Pts',(15.3830449856443,-68.288855628865,10.0982078060305));
#37123=CARTESIAN_POINT('Ctrl Pts',(15.5341550196633,-68.2546420063796,10.6858944634119));
#37124=CARTESIAN_POINT('Ctrl Pts',(15.6614146465391,-68.2257386849337,10.9661810334235));
#37125=CARTESIAN_POINT('Ctrl Pts',(16.0093499903205,-68.1449424659488,11.4722931322537));
#37126=CARTESIAN_POINT('Ctrl Pts',(16.2286900565758,-68.093295210955,11.6926718707977));
#37127=CARTESIAN_POINT('Ctrl Pts',(16.4806955947432,-68.0322473001841,11.8669181223571));
#37128=CARTESIAN_POINT('Ctrl Pts',(14.1985145724514,-60.3826426720153,11.6359872033748));
#37129=CARTESIAN_POINT('Ctrl Pts',(14.1384791309758,-60.3987291200759,11.5775783984678));
#37130=CARTESIAN_POINT('Ctrl Pts',(14.081700362681,-60.4139429451877,11.5159169743213));
#37131=CARTESIAN_POINT('Ctrl Pts',(14.0281914535651,-60.4282806141732,11.451379059159));
#37132=CARTESIAN_POINT('Ctrl Pts',(13.9733764666698,-60.4429682456449,11.3852658635748));
#37133=CARTESIAN_POINT('Ctrl Pts',(13.9219924575766,-60.4567365493853,11.3161335496706));
#37134=CARTESIAN_POINT('Ctrl Pts',(13.8740814492324,-60.4695742653797,11.2443401959101));
#37135=CARTESIAN_POINT('Ctrl Pts',(13.8615442020184,-60.472933610646,11.2255534691112));
#37136=CARTESIAN_POINT('Ctrl Pts',(13.849244935159,-60.4762291892685,11.2065843091216));
#37137=CARTESIAN_POINT('Ctrl Pts',(13.8371847673053,-60.4794607015055,11.1874386951811));
#37138=CARTESIAN_POINT('Ctrl Pts',(13.8274131410429,-60.4820790008712,11.1719261595134));
#37139=CARTESIAN_POINT('Ctrl Pts',(13.8177980990068,-60.48465534362,11.1562969507259));
#37140=CARTESIAN_POINT('Ctrl Pts',(13.8083486578088,-60.4871873137579,11.1405686299001));
#37141=CARTESIAN_POINT('Ctrl Pts',(13.7625022245992,-60.4994718285123,11.0642585714397));
#37142=CARTESIAN_POINT('Ctrl Pts',(13.7205023350773,-60.5107256649919,10.9855425559687));
#37143=CARTESIAN_POINT('Ctrl Pts',(13.6823842420087,-60.5209393772466,10.9048124950817));
#37144=CARTESIAN_POINT('Ctrl Pts',(13.6519560246515,-60.5290925935146,10.8403687718475));
#37145=CARTESIAN_POINT('Ctrl Pts',(13.6240018720623,-60.536582886126,10.7746405673723));
#37146=CARTESIAN_POINT('Ctrl Pts',(13.5985556604601,-60.5434011779752,10.7078100770375));
#37147=CARTESIAN_POINT('Ctrl Pts',(13.5903398047872,-60.5456026098679,10.686232418574));
#37148=CARTESIAN_POINT('Ctrl Pts',(13.5823855107333,-60.547733956536,10.6645397510572));
#37149=CARTESIAN_POINT('Ctrl Pts',(13.5746942691753,-60.5497948185002,10.6427379426545));
#37150=CARTESIAN_POINT('Ctrl Pts',(13.5673646518884,-60.5517587835331,10.6219612045232));
#37151=CARTESIAN_POINT('Ctrl Pts',(13.5602723818286,-60.5536591515681,10.6010802045182));
#37152=CARTESIAN_POINT('Ctrl Pts',(13.5534284149517,-60.5554929869658,10.5801302249954));
#37153=CARTESIAN_POINT('Ctrl Pts',(13.5248766271769,-60.5631434154425,10.4927307124063));
#37154=CARTESIAN_POINT('Ctrl Pts',(13.5006117004043,-60.5696451829756,10.4040498989134));
#37155=CARTESIAN_POINT('Ctrl Pts',(13.4806668323773,-60.5749893942566,10.3144849192065));
#37156=CARTESIAN_POINT('Ctrl Pts',(13.460414058401,-60.5804161086881,10.2235372484701));
#37157=CARTESIAN_POINT('Ctrl Pts',(13.4446152716799,-60.5846493808314,10.1316770970802));
#37158=CARTESIAN_POINT('Ctrl Pts',(13.4333455934662,-60.5876690820077,10.0392871197263));
#37159=CARTESIAN_POINT('Ctrl Pts',(13.4221628859679,-60.5906654794511,9.94761013721475));
#37160=CARTESIAN_POINT('Ctrl Pts',(13.4154393160804,-60.5924670545727,9.85541054684674));
#37161=CARTESIAN_POINT('Ctrl Pts',(13.4132936428739,-60.5930419859756,9.76304299851744));
#37162=CARTESIAN_POINT('Ctrl Pts',(13.4122613686528,-60.5933185830195,9.71860536527655));
#37163=CARTESIAN_POINT('Ctrl Pts',(13.4122893693042,-60.5933110802676,9.67412865780575));
#37164=CARTESIAN_POINT('Ctrl Pts',(13.4133950120097,-60.5930148241975,9.62965173460712));
#37165=CARTESIAN_POINT('Ctrl Pts',(13.4137601235609,-60.5929169928522,9.61496431493879));
#37166=CARTESIAN_POINT('Ctrl Pts',(13.4142427737567,-60.592787667122,9.60027687089771));
#37167=CARTESIAN_POINT('Ctrl Pts',(13.4148436567719,-60.5926266610034,9.585590801596));
#37168=CARTESIAN_POINT('Ctrl Pts',(13.4154511643855,-60.5924638798289,9.57074282172334));
#37169=CARTESIAN_POINT('Ctrl Pts',(13.4161791917241,-60.5922688054914,9.55590504967698));
#37170=CARTESIAN_POINT('Ctrl Pts',(13.4170277181603,-60.5920414435181,9.54108357191584));
#37171=CARTESIAN_POINT('Ctrl Pts',(13.4224967665285,-60.5905760164245,9.44555398638134));
#37172=CARTESIAN_POINT('Ctrl Pts',(13.4329703612531,-60.5877696251762,9.3506422021473));
#37173=CARTESIAN_POINT('Ctrl Pts',(13.4485182643158,-60.5836035771065,9.25674298405853));
#37174=CARTESIAN_POINT('Ctrl Pts',(13.4498478809535,-60.5832473074022,9.24871296469604));
#37175=CARTESIAN_POINT('Ctrl Pts',(13.4512146356353,-60.582881086589,9.24069033920175));
#37176=CARTESIAN_POINT('Ctrl Pts',(13.4526185882087,-60.5825048986307,9.23267534878075));
#37177=CARTESIAN_POINT('Ctrl Pts',(13.4683901533207,-60.5782789204956,9.14263744743655));
#37178=CARTESIAN_POINT('Ctrl Pts',(13.4888516530664,-60.5727962781628,9.05356331283828));
#37179=CARTESIAN_POINT('Ctrl Pts',(13.5137114619786,-60.5661351124408,8.96568771725755));
#37180=CARTESIAN_POINT('Ctrl Pts',(13.5391401674861,-60.5593215113355,8.87580115983445));
#37181=CARTESIAN_POINT('Ctrl Pts',(13.5691709812857,-60.5512747790298,8.78716792582602));
#37182=CARTESIAN_POINT('Ctrl Pts',(13.6035442475271,-60.5420644900992,8.70004212727832));
#37183=CARTESIAN_POINT('Ctrl Pts',(13.6224082878578,-60.5370098857266,8.65222750977575));
#37184=CARTESIAN_POINT('Ctrl Pts',(13.6425810893193,-60.5316045998659,8.60486701428382));
#37185=CARTESIAN_POINT('Ctrl Pts',(13.6640258581899,-60.5258584913652,8.55800419893538));
#37186=CARTESIAN_POINT('Ctrl Pts',(13.6704060167659,-60.5241489330272,8.54406176873024));
#37187=CARTESIAN_POINT('Ctrl Pts',(13.676899765887,-60.5224089381943,8.53016150103107));
#37188=CARTESIAN_POINT('Ctrl Pts',(13.6834982307757,-60.5206408848561,8.51632087094479));
#37189=CARTESIAN_POINT('Ctrl Pts',(13.7247150405699,-60.5095968739572,8.4298664262631));
#37190=CARTESIAN_POINT('Ctrl Pts',(13.7700718775146,-60.4974435461266,8.34560744644018));
#37191=CARTESIAN_POINT('Ctrl Pts',(13.8192407167051,-60.4842687953727,8.26379708587707));
#37192=CARTESIAN_POINT('Ctrl Pts',(13.8693790787445,-60.4708342617545,8.18037356919415));
#37193=CARTESIAN_POINT('Ctrl Pts',(13.9234815558615,-60.4563375467024,8.09949541140026));
#37194=CARTESIAN_POINT('Ctrl Pts',(13.9812533713892,-60.4408576353865,8.02143790704939));
#37195=CARTESIAN_POINT('Ctrl Pts',(14.0394826344362,-60.4252551513772,7.94276232948411));
#37196=CARTESIAN_POINT('Ctrl Pts',(14.1014400133005,-60.4086537217454,7.86695140890492));
#37197=CARTESIAN_POINT('Ctrl Pts',(14.1668712742987,-60.3911214682012,7.79430622909373));
#37198=CARTESIAN_POINT('Ctrl Pts',(14.2014931149696,-60.3818445739529,7.75586726578238));
#37199=CARTESIAN_POINT('Ctrl Pts',(14.2370883363508,-60.3723068631294,7.71831505011915));
#37200=CARTESIAN_POINT('Ctrl Pts',(14.2736239455356,-60.3625171761534,7.68169758973408));
#37201=CARTESIAN_POINT('Ctrl Pts',(14.2866331259749,-60.3590313767605,7.66865926465863));
#37202=CARTESIAN_POINT('Ctrl Pts',(14.2997615607819,-60.3555136232561,7.65573947794386));
#37203=CARTESIAN_POINT('Ctrl Pts',(14.3130078489039,-60.3519642910511,7.64294048656779));
#37204=CARTESIAN_POINT('Ctrl Pts',(14.3231851533472,-60.3492372905443,7.6331068463357));
#37205=CARTESIAN_POINT('Ctrl Pts',(14.3334310228843,-60.3464919180761,7.62334556303852));
#37206=CARTESIAN_POINT('Ctrl Pts',(14.3437359537465,-60.3437307201735,7.61366571160746));
#37207=CARTESIAN_POINT('Ctrl Pts',(14.4166886968569,-60.3241830915715,7.54513815676625));
#37208=CARTESIAN_POINT('Ctrl Pts',(14.4927140802975,-60.3038121514743,7.48057696460985));
#37209=CARTESIAN_POINT('Ctrl Pts',(14.5714997184595,-60.2827016033536,7.42026730037134));
#37210=CARTESIAN_POINT('Ctrl Pts',(14.6503851322383,-60.261564320437,7.35988125883753));
#37211=CARTESIAN_POINT('Ctrl Pts',(14.7320383430701,-60.2396854085352,7.30375667601981));
#37212=CARTESIAN_POINT('Ctrl Pts',(14.8161894528123,-60.2171371866376,7.25220561228357));
#37213=CARTESIAN_POINT('Ctrl Pts',(14.8987454238434,-60.1950163808695,7.20163173230178));
#37214=CARTESIAN_POINT('Ctrl Pts',(14.9837061241246,-60.1722512298408,7.15545893550819));
#37215=CARTESIAN_POINT('Ctrl Pts',(15.0708497996908,-60.1489011523473,7.11401788929066));
#37216=CARTESIAN_POINT('Ctrl Pts',(15.0979686081559,-60.1416346895194,7.10112157997545));
#37217=CARTESIAN_POINT('Ctrl Pts',(15.125299031229,-60.1343115247281,7.08868381627438));
#37218=CARTESIAN_POINT('Ctrl Pts',(15.1528349118068,-60.1269333077644,7.0767154567206));
#37219=CARTESIAN_POINT('Ctrl Pts',(15.1941283917648,-60.115868753157,7.05876741202422));
#37220=CARTESIAN_POINT('Ctrl Pts',(15.2358838838841,-60.1046804027641,7.04187489341864));
#37221=CARTESIAN_POINT('Ctrl Pts',(15.2780676602835,-60.0933772939442,7.02603075613029));
#37222=CARTESIAN_POINT('Ctrl Pts',(15.458048217099,-67.4086397233445,10.0018117506528));
#37223=CARTESIAN_POINT('Ctrl Pts',(15.4516726940089,-67.3922281881599,10.2792252787835));
#37224=CARTESIAN_POINT('Ctrl Pts',(15.488118577317,-67.364342691712,10.5560719127008));
#37225=CARTESIAN_POINT('Ctrl Pts',(15.5698466331085,-67.3243238737158,10.8168646145657));
#37226=CARTESIAN_POINT('Ctrl Pts',(15.8140481541644,-67.2047485806183,11.5961071140833));
#37227=CARTESIAN_POINT('Ctrl Pts',(16.4625291088527,-66.9768469397626,12.2320200381454));
#37228=CARTESIAN_POINT('Ctrl Pts',(17.2188383863881,-66.7200527868787,12.4398697983789));
#37229=CARTESIAN_POINT('Ctrl Pts',(17.9751476639235,-66.4632586339949,12.6477195586123));
#37230=CARTESIAN_POINT('Ctrl Pts',(18.8392852643059,-66.177571969083,12.4275061550171));
#37231=CARTESIAN_POINT('Ctrl Pts',(19.4182523936639,-65.9682965015873,11.8778290289181));
#37232=CARTESIAN_POINT('Ctrl Pts',(19.9972195230219,-65.7590210340916,11.328151902819));
#37233=CARTESIAN_POINT('Ctrl Pts',(20.2910161813555,-65.6261567640121,10.4490110542162));
#37234=CARTESIAN_POINT('Ctrl Pts',(20.162021829958,-65.6065790035572,9.63407278056603));
#37235=CARTESIAN_POINT('Ctrl Pts',(20.0330274785606,-65.5870012431022,8.81913450691582));
#37236=CARTESIAN_POINT('Ctrl Pts',(19.4812421174321,-65.6807099922718,8.06839880821821));
#37237=CARTESIAN_POINT('Ctrl Pts',(18.747685284561,-65.8231242605019,7.71802880880715));
#37238=CARTESIAN_POINT('Ctrl Pts',(18.0141284516898,-65.965538528732,7.36765880939609));
#37239=CARTESIAN_POINT('Ctrl Pts',(17.0988001470759,-66.1566583160226,7.41765450927158));
#37240=CARTESIAN_POINT('Ctrl Pts',(16.4055051616424,-66.288284454746,7.84562973884659));
#37241=CARTESIAN_POINT('Ctrl Pts',(15.7122101762088,-66.4199105934694,8.2736049684216));
#37242=CARTESIAN_POINT('Ctrl Pts',(15.2409485099556,-66.4920430836256,9.07955972769613));
#37243=CARTESIAN_POINT('Ctrl Pts',(15.1966815676295,-66.4497626823332,9.90260247183727));
#37244=CARTESIAN_POINT('Ctrl Pts',(15.1949465504969,-66.4481055265244,9.93486115488332));
#37245=CARTESIAN_POINT('Ctrl Pts',(15.1938674837542,-66.4462726093384,9.96714608853553));
#37246=CARTESIAN_POINT('Ctrl Pts',(15.1934336836835,-66.4442667934687,9.99943462192768));
#37247=CARTESIAN_POINT('Ctrl Pts',(-67.0040126136403,-20.2598690437802,
11.1728309286203));
#37248=CARTESIAN_POINT('Ctrl Pts',(-66.854289394458,-20.6173045957294,10.4434664543479));
#37249=CARTESIAN_POINT('Ctrl Pts',(-66.7561954352348,-20.580718017241,8.59013022403023));
#37250=CARTESIAN_POINT('Ctrl Pts',(-67.209041264398,-18.2866570474715,7.05024279158508));
#37251=CARTESIAN_POINT('Ctrl Pts',(-67.723582781997,-15.7623446338517,8.14059085434287));
#37252=CARTESIAN_POINT('Ctrl Pts',(-67.707898604217,-15.2168614548643,10.8824467802989));
#37253=CARTESIAN_POINT('Ctrl Pts',(-67.0414893382907,-17.0999173665992,
12.8405694561121));
#37254=CARTESIAN_POINT('Ctrl Pts',(-66.182965221624,-19.6999556621853,12.2707319173765));
#37255=CARTESIAN_POINT('Ctrl Pts',(-65.7617874756575,-20.667795081813,9.68094249642456));
#37256=CARTESIAN_POINT('Ctrl Pts',(-66.0183437425753,-19.1062967313381,
7.37485535276681));
#37257=CARTESIAN_POINT('Ctrl Pts',(-66.5900180970021,-16.3687616678969,
7.4044619797337));
#37258=CARTESIAN_POINT('Ctrl Pts',(-66.83384050967,-14.8547867084588,9.74329926128886));
#37259=CARTESIAN_POINT('Ctrl Pts',(-66.3985290187163,-15.8753739824804,
12.3105450512032));
#37260=CARTESIAN_POINT('Ctrl Pts',(-65.5370346894514,-18.4864972623917,
12.8220707222437));
#37261=CARTESIAN_POINT('Ctrl Pts',(-64.8814857844687,-20.3290217552967,
10.8227823754305));
#37262=CARTESIAN_POINT('Ctrl Pts',(-64.8807798084461,-19.7276391663447,
8.09145561890004));
#37263=CARTESIAN_POINT('Ctrl Pts',(-65.4011950297318,-17.1814057921375,
7.05817718516389));
#37264=CARTESIAN_POINT('Ctrl Pts',(-65.8453641599239,-14.91972670377,8.64226139479156));
#37265=CARTESIAN_POINT('Ctrl Pts',(-65.6837566027253,-14.9188369907855,
11.4343367521445));
#37266=CARTESIAN_POINT('Ctrl Pts',(-64.925806142571,-17.1435292903643,12.9502711232991));
#37267=CARTESIAN_POINT('Ctrl Pts',(-64.1115175849316,-19.5784782321599,
11.8413258175008));
#37268=CARTESIAN_POINT('Ctrl Pts',(-63.831020197438,-20.021291406339,9.09413821413749));
#37269=CARTESIAN_POINT('Ctrl Pts',(-64.1995249831399,-18.0419954959306,
7.15290308224158));
#37270=CARTESIAN_POINT('Ctrl Pts',(-64.7548205378836,-15.3655869450728,
7.74475277436916));
#37271=CARTESIAN_POINT('Ctrl Pts',(-64.8685062198083,-14.3372888767,10.3431139119323));
#37272=CARTESIAN_POINT('Ctrl Pts',(-64.3050852130208,-15.8359873727452,
12.6362038638415));
#37273=CARTESIAN_POINT('Ctrl Pts',(-63.4314879220136,-18.4922795208021,
12.5838422163724));
#37274=CARTESIAN_POINT('Ctrl Pts',(-62.890611065017,-19.9068421044143,10.2326155433113));
#37275=CARTESIAN_POINT('Ctrl Pts',(-63.0293273367052,-18.7851286033006,
7.67442896667196));
#37276=CARTESIAN_POINT('Ctrl Pts',(-63.589870005783,-16.0891375551548,7.18532148363271));
#37277=CARTESIAN_POINT('Ctrl Pts',(-63.9391700310929,-14.1815147862763,
9.20045592301492));
#37278=CARTESIAN_POINT('Ctrl Pts',(-63.6321026366036,-14.7234885765213,
11.9269511029875));
#37279=CARTESIAN_POINT('Ctrl Pts',(-62.8075183731849,-17.1968616153845,
12.9390225214354));
#37280=CARTESIAN_POINT('Ctrl Pts',(-62.0647066785609,-19.3650552728411,
11.3362221619431));
#37281=CARTESIAN_POINT('Ctrl Pts',(-61.930203280714,-19.2630114600592,8.54457429525347));
#37282=CARTESIAN_POINT('Ctrl Pts',(-62.3893271714103,-16.9455204456753,
7.04783027207105));
#37283=CARTESIAN_POINT('Ctrl Pts',(-62.8992423967486,-14.4384735898223,
8.1776552235709));
#37284=CARTESIAN_POINT('Ctrl Pts',(-62.8719235739435,-13.9364114971974,
10.9288348037821));
#37285=CARTESIAN_POINT('Ctrl Pts',(-62.197326683109,-15.8500240410826,12.8536227562672));
#37286=CARTESIAN_POINT('Ctrl Pts',(-61.3412962728354,-18.4407556977108,
12.2395195742222));
#37287=CARTESIAN_POINT('Ctrl Pts',(-60.9310995184379,-19.3676134988852,
9.63289839745324));
#37288=CARTESIAN_POINT('Ctrl Pts',(-61.19734228766,-17.7699646296632,7.35288957156097));
#37289=CARTESIAN_POINT('Ctrl Pts',(-61.7687958934071,-15.0332534115102,
7.42803777444134));
#37290=CARTESIAN_POINT('Ctrl Pts',(-62.0026849934362,-13.5563500795274,
9.79147768509061));
#37291=CARTESIAN_POINT('Ctrl Pts',(-61.5565643024821,-14.6172778371396,
12.3404488591361));
#37292=CARTESIAN_POINT('Ctrl Pts',(-60.6930063334386,-17.2361027255536,
12.8070892069868));
#37293=CARTESIAN_POINT('Ctrl Pts',(-60.0459653166684,-19.0468753473845,
10.776269968826));
#37294=CARTESIAN_POINT('Ctrl Pts',(-60.0567902041014,-18.4024589901609,
8.05473611617426));
#37295=CARTESIAN_POINT('Ctrl Pts',(-60.5814573009747,-15.8403574002333,
7.06404294414461));
#37296=CARTESIAN_POINT('Ctrl Pts',(-61.0189035288689,-13.6037685248156,
8.6852426906361));
#37297=CARTESIAN_POINT('Ctrl Pts',(-60.8454027634005,-13.6472648693588,
11.476703032887));
#37298=CARTESIAN_POINT('Ctrl Pts',(-60.081329531004,-15.8948076660291,12.9532921034687));
#37299=CARTESIAN_POINT('Ctrl Pts',(-59.2714063402784,-18.3134648367082,
11.80442877448));
#37300=CARTESIAN_POINT('Ctrl Pts',(-59.0033710168104,-18.7097689547775,
9.0457808277518));
#37301=CARTESIAN_POINT('Ctrl Pts',(-59.253282418477,-17.3744086881423,7.78080120942645));
#37302=CARTESIAN_POINT('Ctrl Pts',(-59.4090483774019,-16.5917431062324,
7.56791319796486));
#37303=CARTESIAN_POINT('Ctrl Pts',(-67.0649244254631,-20.445968013835,11.2591724044644));
#37304=CARTESIAN_POINT('Ctrl Pts',(-66.9078844272408,-20.8307101569088,
10.4761135710135));
#37305=CARTESIAN_POINT('Ctrl Pts',(-66.8099800782137,-20.7934159435354,
8.4863384205957));
#37306=CARTESIAN_POINT('Ctrl Pts',(-67.3072801529266,-18.333449470762,6.83308754393481));
#37307=CARTESIAN_POINT('Ctrl Pts',(-67.8708178297159,-15.6262809016683,
8.003704858317));
#37308=CARTESIAN_POINT('Ctrl Pts',(-67.8650956520226,-15.0436190322125,
10.9474107537972));
#37309=CARTESIAN_POINT('Ctrl Pts',(-67.1607433019049,-17.0682804619454,
13.0496865190182));
#37310=CARTESIAN_POINT('Ctrl Pts',(-66.2501329885661,-19.8627070898853,
12.4378986762062));
#37311=CARTESIAN_POINT('Ctrl Pts',(-65.8090656142303,-20.9047756131301,
9.65745411880286));
#37312=CARTESIAN_POINT('Ctrl Pts',(-66.0956256802753,-19.2313015598933,
7.18159743500955));
#37313=CARTESIAN_POINT('Ctrl Pts',(-66.7205021994898,-16.2952133143909,
7.2133836428561));
#37314=CARTESIAN_POINT('Ctrl Pts',(-66.9933909703099,-14.6727612295383,
9.72440146443704));
#37315=CARTESIAN_POINT('Ctrl Pts',(-66.5371493528455,-15.7714607991059,
12.4806427736089));
#37316=CARTESIAN_POINT('Ctrl Pts',(-65.6233501657759,-18.5777884658278,
13.0298259452252));
#37317=CARTESIAN_POINT('Ctrl Pts',(-64.9306576947329,-20.5589346344442,
10.8833539743367));
#37318=CARTESIAN_POINT('Ctrl Pts',(-64.9410163841629,-19.916258151854,7.95095238475352));
#37319=CARTESIAN_POINT('Ctrl Pts',(-65.5108601749997,-17.1855548447367,
6.84160605175788));
#37320=CARTESIAN_POINT('Ctrl Pts',(-65.9988447894535,-14.7603541429462,
8.54230738426578));
#37321=CARTESIAN_POINT('Ctrl Pts',(-65.8364566439328,-14.7623776252395,
11.5399297656092));
#37322=CARTESIAN_POINT('Ctrl Pts',(-65.0338240192839,-17.1538260329046,
13.167464204339));
#37323=CARTESIAN_POINT('Ctrl Pts',(-64.1707057986788,-19.7710097578042,
11.9768805549428));
#37324=CARTESIAN_POINT('Ctrl Pts',(-63.8806753904707,-20.2494006496397,
9.02745047458906));
#37325=CARTESIAN_POINT('Ctrl Pts',(-64.2874254021706,-18.1273716126596,
6.94330548061646));
#37326=CARTESIAN_POINT('Ctrl Pts',(-64.894717347108,-15.2569098917891,7.57872596768916));
#37327=CARTESIAN_POINT('Ctrl Pts',(-65.0278889803931,-14.1558892629052,
10.3683732743996));
#37328=CARTESIAN_POINT('Ctrl Pts',(-64.4341066798256,-15.7678976499211,
12.8302759390876));
#37329=CARTESIAN_POINT('Ctrl Pts',(-63.5073135350877,-18.6227194268525,
12.7740595314737));
#37330=CARTESIAN_POINT('Ctrl Pts',(-62.9377350396947,-20.1443979832212,
10.2497402360727));
#37331=CARTESIAN_POINT('Ctrl Pts',(-63.0977799648827,-18.9430848635887,
7.50322506140479));
#37332=CARTESIAN_POINT('Ctrl Pts',(-63.7107053062555,-16.0515990210022,
6.97811046011729));
#37333=CARTESIAN_POINT('Ctrl Pts',(-64.096836741373,-14.0065195594072,9.14159508133287));
#37334=CARTESIAN_POINT('Ctrl Pts',(-63.7782802952007,-14.5913710742642,
12.06880940332));
#37335=CARTESIAN_POINT('Ctrl Pts',(-62.9041084194733,-17.2498076016892,
13.1553875028215));
#37336=CARTESIAN_POINT('Ctrl Pts',(-62.1177290461057,-19.5805980497848,
11.4345921747918));
#37337=CARTESIAN_POINT('Ctrl Pts',(-61.9844404141372,-19.4740206690252,
8.43742875512251));
#37338=CARTESIAN_POINT('Ctrl Pts',(-62.4884807287629,-16.9888992784424,
6.83049741954161));
#37339=CARTESIAN_POINT('Ctrl Pts',(-63.0470515348743,-14.3002673230729,
8.04349783254878));
#37340=CARTESIAN_POINT('Ctrl Pts',(-63.0288381927735,-13.7642231138317,
10.997213771131));
#37341=CARTESIAN_POINT('Ctrl Pts',(-62.3156954611176,-15.8216906940831,
13.0637007771192));
#37342=CARTESIAN_POINT('Ctrl Pts',(-61.4077624358672,-18.6061255468504,
12.4043885425463));
#37343=CARTESIAN_POINT('Ctrl Pts',(-60.9784844518179,-19.6041954665562,
9.6058731090036));
#37344=CARTESIAN_POINT('Ctrl Pts',(-61.2754441211642,-17.89190956542,7.15801457676294));
#37345=CARTESIAN_POINT('Ctrl Pts',(-61.9000836406212,-14.9567058150541,
7.23869504059023));
#37346=CARTESIAN_POINT('Ctrl Pts',(-62.1623078281202,-13.3740544969969,
9.77612668779305));
#37347=CARTESIAN_POINT('Ctrl Pts',(-61.6944612588913,-14.5160643361698,
12.512748040292));
#37348=CARTESIAN_POINT('Ctrl Pts',(-60.7784465109946,-17.3306605884652,
13.013741520669));
#37349=CARTESIAN_POINT('Ctrl Pts',(-60.0948882619405,-19.2777173765314,
10.8334174170441));
#37350=CARTESIAN_POINT('Ctrl Pts',(-60.117626694016,-18.5888390654038,7.91152966540869));
#37351=CARTESIAN_POINT('Ctrl Pts',(-60.6920353750484,-15.8410993561455,
6.84790363622595));
#37352=CARTESIAN_POINT('Ctrl Pts',(-61.1728021605341,-13.4428359587846,
8.58845287746082));
#37353=CARTESIAN_POINT('Ctrl Pts',(-60.9976452524506,-13.4925131117118,
11.585414967516));
#37354=CARTESIAN_POINT('Ctrl Pts',(-60.1884391092678,-15.9084942245297,
13.1707075830488));
#37355=CARTESIAN_POINT('Ctrl Pts',(-59.33000762519,-18.5081868105882,11.9372672251402));
#37356=CARTESIAN_POINT('Ctrl Pts',(-59.0533567133275,-18.9366447422823,
8.97553311378027));
#37357=CARTESIAN_POINT('Ctrl Pts',(-59.3290771863823,-17.5049637099299,
7.61742821670101));
#37358=CARTESIAN_POINT('Ctrl Pts',(-59.500015870806,-16.6656727455696,7.38886781406131));
#37359=CARTESIAN_POINT('Ctrl Pts',(-67.1258362372859,-20.6320669838898,
11.3455138803086));
#37360=CARTESIAN_POINT('Ctrl Pts',(-66.9614794600237,-21.0441157180882,
10.5087606876792));
#37361=CARTESIAN_POINT('Ctrl Pts',(-66.8637647211926,-21.0061138698298,
8.38254661716119));
#37362=CARTESIAN_POINT('Ctrl Pts',(-67.4055190414552,-18.3802418940525,
6.61593229628453));
#37363=CARTESIAN_POINT('Ctrl Pts',(-68.0180528774348,-15.4902171694848,
7.86681886229114));
#37364=CARTESIAN_POINT('Ctrl Pts',(-68.0222926998282,-14.8703766095608,
11.0123747272955));
#37365=CARTESIAN_POINT('Ctrl Pts',(-67.2799972655191,-17.0366435572917,
13.2588035819243));
#37366=CARTESIAN_POINT('Ctrl Pts',(-66.317300755508,-20.0254585175853,12.6050654350359));
#37367=CARTESIAN_POINT('Ctrl Pts',(-65.8563437528033,-21.1417561444472,
9.63396574118116));
#37368=CARTESIAN_POINT('Ctrl Pts',(-66.172907617975,-19.3563063884486,6.98833951725229));
#37369=CARTESIAN_POINT('Ctrl Pts',(-66.8509863019776,-16.2216649608848,
7.0223053059785));
#37370=CARTESIAN_POINT('Ctrl Pts',(-67.1529414309497,-14.4907357506179,
9.70550366758521));
#37371=CARTESIAN_POINT('Ctrl Pts',(-66.6757696869749,-15.6675476157315,
12.6507404960146));
#37372=CARTESIAN_POINT('Ctrl Pts',(-65.7096656421003,-18.6690796692638,
13.2375811682066));
#37373=CARTESIAN_POINT('Ctrl Pts',(-64.9798296049969,-20.7888475135917,
10.943925573243));
#37374=CARTESIAN_POINT('Ctrl Pts',(-65.0012529598798,-20.1048771373633,
7.810449150607));
#37375=CARTESIAN_POINT('Ctrl Pts',(-65.6205253202676,-17.1897038973359,
6.62503491835186));
#37376=CARTESIAN_POINT('Ctrl Pts',(-66.1523254189831,-14.6009815821224,
8.44235337374002));
#37377=CARTESIAN_POINT('Ctrl Pts',(-65.9891566851404,-14.6059182596936,
11.6455227790739));
#37378=CARTESIAN_POINT('Ctrl Pts',(-65.1418418959967,-17.1641227754448,
13.384657285379));
#37379=CARTESIAN_POINT('Ctrl Pts',(-64.2298940124261,-19.9635412834486,
12.1124352923848));
#37380=CARTESIAN_POINT('Ctrl Pts',(-63.9303305835035,-20.4775098929403,
8.96076273504062));
#37381=CARTESIAN_POINT('Ctrl Pts',(-64.3753258212014,-18.2127477293887,
6.73370787899134));
#37382=CARTESIAN_POINT('Ctrl Pts',(-65.0346141563324,-15.1482328385054,
7.41269916100916));
#37383=CARTESIAN_POINT('Ctrl Pts',(-65.1872717409779,-13.9744896491104,
10.3936326368669));
#37384=CARTESIAN_POINT('Ctrl Pts',(-64.5631281466304,-15.6998079270971,
13.0243480143336));
#37385=CARTESIAN_POINT('Ctrl Pts',(-63.5831391481619,-18.753159332903,12.9642768465751));
#37386=CARTESIAN_POINT('Ctrl Pts',(-62.9848590143722,-20.3819538620283,
10.2668649288342));
#37387=CARTESIAN_POINT('Ctrl Pts',(-63.1662325930603,-19.1010411238768,
7.33202115613761));
#37388=CARTESIAN_POINT('Ctrl Pts',(-63.831540606728,-16.0140604868496,6.77089943660186));
#37389=CARTESIAN_POINT('Ctrl Pts',(-64.2545034516531,-13.8315243325381,
9.08273423965082));
#37390=CARTESIAN_POINT('Ctrl Pts',(-63.9244579537977,-14.459253572007,12.2106677036524));
#37391=CARTESIAN_POINT('Ctrl Pts',(-63.0006984657617,-17.3027535879938,
13.3717524842075));
#37392=CARTESIAN_POINT('Ctrl Pts',(-62.1707514136505,-19.7961408267284,
11.5329621876406));
#37393=CARTESIAN_POINT('Ctrl Pts',(-62.0386775475603,-19.6850298779912,
8.33028321499155));
#37394=CARTESIAN_POINT('Ctrl Pts',(-62.5876342861156,-17.0322781112095,
6.61316456701218));
#37395=CARTESIAN_POINT('Ctrl Pts',(-63.1948606729999,-14.1620610563234,
7.90934044152666));
#37396=CARTESIAN_POINT('Ctrl Pts',(-63.1857528116036,-13.592034730466,11.06559273848));
#37397=CARTESIAN_POINT('Ctrl Pts',(-62.4340642391261,-15.7933573470836,
13.2737787979711));
#37398=CARTESIAN_POINT('Ctrl Pts',(-61.474228598899,-18.77149539599,12.5692575108704));
#37399=CARTESIAN_POINT('Ctrl Pts',(-61.0258693851979,-19.8407774342271,
9.57884782055393));
#37400=CARTESIAN_POINT('Ctrl Pts',(-61.3535459546682,-18.0138545011767,
6.96313958196492));
#37401=CARTESIAN_POINT('Ctrl Pts',(-62.0313713878355,-14.8801582185979,
7.04935230673909));
#37402=CARTESIAN_POINT('Ctrl Pts',(-62.3219306628042,-13.1917589144664,
9.76077569049554));
#37403=CARTESIAN_POINT('Ctrl Pts',(-61.8323582153005,-14.4148508352001,
12.6850472214478));
#37404=CARTESIAN_POINT('Ctrl Pts',(-60.8638866885507,-17.4252184513767,
13.2203938343511));
#37405=CARTESIAN_POINT('Ctrl Pts',(-60.1438112072126,-19.5085594056784,
10.8905648652622));
#37406=CARTESIAN_POINT('Ctrl Pts',(-60.1784631839307,-18.7752191406467,
7.76832321464309));
#37407=CARTESIAN_POINT('Ctrl Pts',(-60.8026134491221,-15.8418413120578,
6.63176432830731));
#37408=CARTESIAN_POINT('Ctrl Pts',(-61.3267007921992,-13.2819033927535,
8.49166306428554));
#37409=CARTESIAN_POINT('Ctrl Pts',(-61.1498877415005,-13.3377613540649,
11.6941269021449));
#37410=CARTESIAN_POINT('Ctrl Pts',(-60.2955486875317,-15.9221807830303,
13.3881230626289));
#37411=CARTESIAN_POINT('Ctrl Pts',(-59.3886089101014,-18.7029087844682,
12.0701056758003));
#37412=CARTESIAN_POINT('Ctrl Pts',(-59.1033424098446,-19.1635205297872,
8.90528539980874));
#37413=CARTESIAN_POINT('Ctrl Pts',(-59.4048719542877,-17.6355187317176,
7.45405522397557));
#37414=CARTESIAN_POINT('Ctrl Pts',(-59.59098336421,-16.7396023849069,7.20982243015776));
#37415=CARTESIAN_POINT('Ctrl Pts',(-67.1867480491086,-20.8181659539446,
11.4318553561527));
#37416=CARTESIAN_POINT('Ctrl Pts',(-67.0150744928066,-21.2575212792676,
10.5414078043449));
#37417=CARTESIAN_POINT('Ctrl Pts',(-66.9175493641714,-21.2188117961242,
8.27875481372668));
#37418=CARTESIAN_POINT('Ctrl Pts',(-67.5037579299839,-18.4270343173431,
6.39877704863426));
#37419=CARTESIAN_POINT('Ctrl Pts',(-68.1652879251537,-15.3541534373013,
7.72993286626527));
#37420=CARTESIAN_POINT('Ctrl Pts',(-68.1794897476338,-14.697134186909,11.0773387007938));
#37421=CARTESIAN_POINT('Ctrl Pts',(-67.3992512291332,-17.005006652638,13.4679206448304));
#37422=CARTESIAN_POINT('Ctrl Pts',(-66.3844685224501,-20.1882099452852,
12.7722321938656));
#37423=CARTESIAN_POINT('Ctrl Pts',(-65.9036218913761,-21.3787366757643,
9.61047736355945));
#37424=CARTESIAN_POINT('Ctrl Pts',(-66.2501895556749,-19.4813112170038,
6.79508159949504));
#37425=CARTESIAN_POINT('Ctrl Pts',(-66.9814704044654,-16.1481166073788,
6.8312269691009));
#37426=CARTESIAN_POINT('Ctrl Pts',(-67.3124918915896,-14.3087102716974,
9.68660587073339));
#37427=CARTESIAN_POINT('Ctrl Pts',(-66.8143900211042,-15.5636344323571,
12.8208382184203));
#37428=CARTESIAN_POINT('Ctrl Pts',(-65.7959811184248,-18.7603708726999,
13.4453363911881));
#37429=CARTESIAN_POINT('Ctrl Pts',(-65.0290015152611,-21.0187603927391,
11.0044971721492));
#37430=CARTESIAN_POINT('Ctrl Pts',(-65.0614895355965,-20.2934961228726,
7.66994591646049));
#37431=CARTESIAN_POINT('Ctrl Pts',(-65.7301904655356,-17.193852949935,6.40846378494586));
#37432=CARTESIAN_POINT('Ctrl Pts',(-66.3058060485127,-14.4416090212986,
8.34239936321424));
#37433=CARTESIAN_POINT('Ctrl Pts',(-66.1418567263479,-14.4494588941477,
11.7511157925387));
#37434=CARTESIAN_POINT('Ctrl Pts',(-65.2498597727096,-17.1744195179851,
13.601850366419));
#37435=CARTESIAN_POINT('Ctrl Pts',(-64.2890822261733,-20.156072809093,12.2479900298267));
#37436=CARTESIAN_POINT('Ctrl Pts',(-63.9799857765362,-20.705619136241,8.89407499549219));
#37437=CARTESIAN_POINT('Ctrl Pts',(-64.4632262402321,-18.2981238461178,
6.52411027736622));
#37438=CARTESIAN_POINT('Ctrl Pts',(-65.1745109655567,-15.0395557852216,
7.24667235432916));
#37439=CARTESIAN_POINT('Ctrl Pts',(-65.3466545015628,-13.7930900353156,
10.4188919993342));
#37440=CARTESIAN_POINT('Ctrl Pts',(-64.6921496134352,-15.631718204273,13.2184200895797));
#37441=CARTESIAN_POINT('Ctrl Pts',(-63.6589647612361,-18.8835992389535,
13.1544941616765));
#37442=CARTESIAN_POINT('Ctrl Pts',(-63.0319829890499,-20.6195097408353,
10.2839896215957));
#37443=CARTESIAN_POINT('Ctrl Pts',(-63.2346852212379,-19.2589973841649,
7.16081725087042));
#37444=CARTESIAN_POINT('Ctrl Pts',(-63.9523759072004,-15.9765219526969,
6.56368841308645));
#37445=CARTESIAN_POINT('Ctrl Pts',(-64.4121701619332,-13.656529105669,9.02387339796877));
#37446=CARTESIAN_POINT('Ctrl Pts',(-64.0706356123947,-14.3271360697498,
12.3525260039849));
#37447=CARTESIAN_POINT('Ctrl Pts',(-63.0972885120501,-17.3556995742985,
13.5881174655936));
#37448=CARTESIAN_POINT('Ctrl Pts',(-62.2237737811953,-20.0116836036721,
11.6313322004894));
#37449=CARTESIAN_POINT('Ctrl Pts',(-62.0929146809836,-19.8960390869572,
8.2231376748606));
#37450=CARTESIAN_POINT('Ctrl Pts',(-62.6867878434683,-17.0756569439767,
6.39583171448275));
#37451=CARTESIAN_POINT('Ctrl Pts',(-63.3426698111255,-14.023854789574,7.77518305050454));
#37452=CARTESIAN_POINT('Ctrl Pts',(-63.3426674304337,-13.4198463471003,
11.1339717058289));
#37453=CARTESIAN_POINT('Ctrl Pts',(-62.5524330171347,-15.7650240000841,
13.4838568188231));
#37454=CARTESIAN_POINT('Ctrl Pts',(-61.5406947619308,-18.9368652451296,
12.7341264791944));
#37455=CARTESIAN_POINT('Ctrl Pts',(-61.0732543185779,-20.0773594018981,
9.5518225321043));
#37456=CARTESIAN_POINT('Ctrl Pts',(-61.4316477881724,-18.1357994369335,
6.76826458716688));
#37457=CARTESIAN_POINT('Ctrl Pts',(-62.1626591350496,-14.8036106221418,
6.86000957288797));
#37458=CARTESIAN_POINT('Ctrl Pts',(-62.4815534974884,-13.0094633319358,
9.74542469319801));
#37459=CARTESIAN_POINT('Ctrl Pts',(-61.9702551717096,-14.3136373342303,
12.8573464026037));
#37460=CARTESIAN_POINT('Ctrl Pts',(-60.9493268661068,-17.5197763142882,
13.4270461480333));
#37461=CARTESIAN_POINT('Ctrl Pts',(-60.1927341524846,-19.7394014348254,
10.9477123134803));
#37462=CARTESIAN_POINT('Ctrl Pts',(-60.2392996738453,-18.9615992158895,
7.62511676387751));
#37463=CARTESIAN_POINT('Ctrl Pts',(-60.9131915231958,-15.84258326797,6.41562502038865));
#37464=CARTESIAN_POINT('Ctrl Pts',(-61.4805994238643,-13.1209708267224,
8.39487325111026));
#37465=CARTESIAN_POINT('Ctrl Pts',(-61.3021302305505,-13.183009596418,11.8028388367739));
#37466=CARTESIAN_POINT('Ctrl Pts',(-60.4026582657955,-15.9358673415309,
13.605538542209));
#37467=CARTESIAN_POINT('Ctrl Pts',(-59.4472101950129,-18.8976307583482,
12.2029441264605));
#37468=CARTESIAN_POINT('Ctrl Pts',(-59.1533281063617,-19.3903963172921,
8.83503768583721));
#37469=CARTESIAN_POINT('Ctrl Pts',(-59.4806667221931,-17.7660737535053,
7.29068223125013));
#37470=CARTESIAN_POINT('Ctrl Pts',(-59.6819508576141,-16.8135320242442,
7.03077704625421));
#37471=CARTESIAN_POINT('Ctrl Pts',(-67.0040126136403,-20.2598690437802,
11.1728309286203));
#37472=CARTESIAN_POINT('Ctrl Pts',(-66.9555034255254,-20.4203000043806,
10.9082027524034));
#37473=CARTESIAN_POINT('Ctrl Pts',(-66.9207835851305,-20.5332184525386,
10.6149904639439));
#37474=CARTESIAN_POINT('Ctrl Pts',(-66.8813975908017,-20.6611539455099,
9.99178401342212));
#37475=CARTESIAN_POINT('Ctrl Pts',(-66.8780249511107,-20.6720025707685,
9.66515229429124));
#37476=CARTESIAN_POINT('Ctrl Pts',(-66.904675210205,-20.5855924444281,9.00098486496444));
#37477=CARTESIAN_POINT('Ctrl Pts',(-66.9367881932439,-20.4815398383751,
8.66883374311719));
#37478=CARTESIAN_POINT('Ctrl Pts',(-67.0315956493192,-20.1690707048654,
8.06423785428561));
#37479=CARTESIAN_POINT('Ctrl Pts',(-67.0931208523801,-19.964426561113,7.79496359360514));
#37480=CARTESIAN_POINT('Ctrl Pts',(-67.2425937581437,-19.4553169386783,
7.32570054462912));
#37481=CARTESIAN_POINT('Ctrl Pts',(-67.3308539700401,-19.1487818292127,
7.13688275745703));
#37482=CARTESIAN_POINT('Ctrl Pts',(-67.4238662472345,-18.8154792730622,
7.01293629783549));
#37483=CARTESIAN_POINT('Ctrl Pts',(-66.7095652904141,-15.2652009106025,
9.99881345470568));
#37484=CARTESIAN_POINT('Ctrl Pts',(-66.7141255555458,-15.2659775128488,
9.92620926472478));
#37485=CARTESIAN_POINT('Ctrl Pts',(-66.7178306708093,-15.2699455778512,
9.85363960672308));
#37486=CARTESIAN_POINT('Ctrl Pts',(-66.7206515257331,-15.2772137473687,
9.78136734601538));
#37487=CARTESIAN_POINT('Ctrl Pts',(-66.752566372114,-15.3594450282715,8.9636868341038));
#37488=CARTESIAN_POINT('Ctrl Pts',(-66.6712922345581,-15.8641033480842,
8.18407440691875));
#37489=CARTESIAN_POINT('Ctrl Pts',(-66.5353761067089,-16.5726883518974,
7.78933375549841));
#37490=CARTESIAN_POINT('Ctrl Pts',(-66.3994599788598,-17.2812733557106,
7.39459310407807));
#37491=CARTESIAN_POINT('Ctrl Pts',(-66.2089018607176,-18.1937850435244,
7.38472422842244));
#37492=CARTESIAN_POINT('Ctrl Pts',(-66.0708634238268,-18.9102906125104,
7.76413764787091));
#37493=CARTESIAN_POINT('Ctrl Pts',(-65.9328249869361,-19.6267961814964,
8.14355106731939));
#37494=CARTESIAN_POINT('Ctrl Pts',(-65.8473062312968,-20.1472956316547,
8.91224678187198));
#37495=CARTESIAN_POINT('Ctrl Pts',(-65.8747431444716,-20.2462387867959,
9.72822620930693));
#37496=CARTESIAN_POINT('Ctrl Pts',(-65.9021800576463,-20.3451819419371,
10.5442056367419));
#37497=CARTESIAN_POINT('Ctrl Pts',(-66.0425726396352,-20.0225688020612,
11.4074687770592));
#37498=CARTESIAN_POINT('Ctrl Pts',(-66.2558562834074,-19.4279225161922,
11.9340732703405));
#37499=CARTESIAN_POINT('Ctrl Pts',(-66.4691399271796,-18.8332762303233,
12.4606777636217));
#37500=CARTESIAN_POINT('Ctrl Pts',(-66.7553146327352,-17.9665967984612,
12.6506236098669));
#37501=CARTESIAN_POINT('Ctrl Pts',(-67.0094701965007,-17.2194144305744,
12.4192427536873));
#37502=CARTESIAN_POINT('Ctrl Pts',(-67.2636257602662,-16.4722320626875,
12.1878618975077));
#37503=CARTESIAN_POINT('Ctrl Pts',(-67.4857621822416,-15.8445467587759,
11.5351543389033));
#37504=CARTESIAN_POINT('Ctrl Pts',(-67.5994444228593,-15.6216179699846,
10.7518245719417));
#37505=CARTESIAN_POINT('Ctrl Pts',(-67.6344914472383,-15.5528913979793,
10.5103323450969));
#37506=CARTESIAN_POINT('Ctrl Pts',(-67.6592307340631,-15.5226338262371,
10.2564254798709));
#37507=CARTESIAN_POINT('Ctrl Pts',(-67.6742507328171,-15.5286491313886,
10.0019962882658));
#37508=CARTESIAN_POINT('Ctrl Pts',(-59.6819508576141,-16.8135320242443,
7.03077704625424));
#37509=CARTESIAN_POINT('Ctrl Pts',(-59.6574023990845,-16.905148118724,7.06547285383592));
#37510=CARTESIAN_POINT('Ctrl Pts',(-59.6333816237385,-16.9947948727525,
7.10515219319408));
#37511=CARTESIAN_POINT('Ctrl Pts',(-59.6099513655554,-17.0822377867264,
7.1494969432907));
#37512=CARTESIAN_POINT('Ctrl Pts',(-59.5861978454359,-17.1708871306712,
7.19445350780586));
#37513=CARTESIAN_POINT('Ctrl Pts',(-59.5630510759256,-17.2572720505146,
7.24420580542308));
#37514=CARTESIAN_POINT('Ctrl Pts',(-59.5405853294381,-17.3411153578357,
7.29846300341081));
#37515=CARTESIAN_POINT('Ctrl Pts',(-59.5341747454285,-17.3650399830657,
7.31394525440213));
#37516=CARTESIAN_POINT('Ctrl Pts',(-59.5278196764473,-17.3887574233895,
7.32979452700506));
#37517=CARTESIAN_POINT('Ctrl Pts',(-59.5215220078018,-17.4122606427434,
7.3460045350289));
#37518=CARTESIAN_POINT('Ctrl Pts',(-59.5165727272691,-17.4307316091526,
7.35874383296051));
#37519=CARTESIAN_POINT('Ctrl Pts',(-59.5116584066169,-17.4490721035113,
7.37170741286395));
#37520=CARTESIAN_POINT('Ctrl Pts',(-59.5067848207402,-17.4672605736183,
7.38487881899596));
#37521=CARTESIAN_POINT('Ctrl Pts',(-59.4853806969008,-17.5471418512783,
7.44272583659645));
#37522=CARTESIAN_POINT('Ctrl Pts',(-59.464740904359,-17.6241706057018,7.50463022504743));
#37523=CARTESIAN_POINT('Ctrl Pts',(-59.4449347986475,-17.6980879985172,
7.57029723806388));
#37524=CARTESIAN_POINT('Ctrl Pts',(-59.4299001526051,-17.7541980614214,
7.62014450797887));
#37525=CARTESIAN_POINT('Ctrl Pts',(-59.4153460633232,-17.8085146620793,
7.67216077819929));
#37526=CARTESIAN_POINT('Ctrl Pts',(-59.4013071776556,-17.8609084966726,
7.72622830882967));
#37527=CARTESIAN_POINT('Ctrl Pts',(-59.3940669982599,-17.8879292140331,
7.75411219010849));
#37528=CARTESIAN_POINT('Ctrl Pts',(-59.3869639126606,-17.9144382903802,
7.78254177993925));
#37529=CARTESIAN_POINT('Ctrl Pts',(-59.380003115187,-17.940416340213,7.81150163933501));
#37530=CARTESIAN_POINT('Ctrl Pts',(-59.3770692604963,-17.9513656349807,
7.82370771481001));
#37531=CARTESIAN_POINT('Ctrl Pts',(-59.3741603924804,-17.9622216782085,
7.83600935542272));
#37532=CARTESIAN_POINT('Ctrl Pts',(-59.3712797970546,-17.9729722066936,
7.84839276286152));
#37533=CARTESIAN_POINT('Ctrl Pts',(-59.3542405471804,-18.036563552947,7.92164288738543));
#37534=CARTESIAN_POINT('Ctrl Pts',(-59.3381672911566,-18.0965497610707,
7.99784282332634));
#37535=CARTESIAN_POINT('Ctrl Pts',(-59.3231234328439,-18.1526942046358,
8.07671631125713));
#37536=CARTESIAN_POINT('Ctrl Pts',(-59.3083518045395,-18.2078226719783,
8.15416252369557));
#37537=CARTESIAN_POINT('Ctrl Pts',(-59.2945725639227,-18.25924749805,8.23418719308367));
#37538=CARTESIAN_POINT('Ctrl Pts',(-59.2818571865986,-18.3067019322607,
8.31655060950961));
#37539=CARTESIAN_POINT('Ctrl Pts',(-59.2693830444672,-18.3532560644759,
8.39735143332656));
#37540=CARTESIAN_POINT('Ctrl Pts',(-59.2579327074429,-18.3959893040146,
8.48040377581006));
#37541=CARTESIAN_POINT('Ctrl Pts',(-59.2475859889068,-18.4346037832828,
8.56549184010165));
#37542=CARTESIAN_POINT('Ctrl Pts',(-59.2424064367759,-18.4539341349959,
8.60808680034756));
#37543=CARTESIAN_POINT('Ctrl Pts',(-59.2375036518288,-18.4722315775171,
8.65119201452183));
#37544=CARTESIAN_POINT('Ctrl Pts',(-59.2328889292081,-18.4894539568003,
8.6947806500647));
#37545=CARTESIAN_POINT('Ctrl Pts',(-59.2306690827174,-18.4977385366888,
8.71574834142993));
#37546=CARTESIAN_POINT('Ctrl Pts',(-59.2285159057548,-18.5057743025105,
8.73682789355957));
#37547=CARTESIAN_POINT('Ctrl Pts',(-59.2264307309995,-18.51355628064,8.75801630583257));
#37548=CARTESIAN_POINT('Ctrl Pts',(-59.225099704237,-18.5185237401439,8.77154147619001));
#37549=CARTESIAN_POINT('Ctrl Pts',(-59.223796394322,-18.5233877589649,8.78511114963466));
#37550=CARTESIAN_POINT('Ctrl Pts',(-59.2225223976776,-18.5281423791704,
8.79871063717586));
#37551=CARTESIAN_POINT('Ctrl Pts',(-59.2143322655469,-18.5587083684028,
8.88613755494957));
#37552=CARTESIAN_POINT('Ctrl Pts',(-59.2073383924936,-18.5848098579794,
8.9749370538889));
#37553=CARTESIAN_POINT('Ctrl Pts',(-59.2016063055572,-18.6062022976594,
9.06488740622582));
#37554=CARTESIAN_POINT('Ctrl Pts',(-59.2009154354318,-18.6087806600691,
9.07572883481821));
#37555=CARTESIAN_POINT('Ctrl Pts',(-59.2002429107549,-18.6112905563326,
9.08658699331409));
#37556=CARTESIAN_POINT('Ctrl Pts',(-59.199588859507,-18.6137315088204,9.09746150181073));
#37557=CARTESIAN_POINT('Ctrl Pts',(-59.1940765541309,-18.6343037125509,
9.18911121862253));
#37558=CARTESIAN_POINT('Ctrl Pts',(-59.1898752976091,-18.6499830153458,
9.28192246233326));
#37559=CARTESIAN_POINT('Ctrl Pts',(-59.1869573634509,-18.6608728938775,
9.37550443038003));
#37560=CARTESIAN_POINT('Ctrl Pts',(-59.1839372837921,-18.6721439846069,
9.47236233833766));
#37561=CARTESIAN_POINT('Ctrl Pts',(-59.1822919652801,-18.6782843968884,
9.57004704528476));
#37562=CARTESIAN_POINT('Ctrl Pts',(-59.1820051755357,-18.6793547107854,
9.66811274308771));
#37563=CARTESIAN_POINT('Ctrl Pts',(-59.1818653628562,-18.6798764988089,
9.71592068687496));
#37564=CARTESIAN_POINT('Ctrl Pts',(-59.1820486386195,-18.6791925043485,
9.76381888087633));
#37565=CARTESIAN_POINT('Ctrl Pts',(-59.1825542820092,-18.6773054175276,
9.81175333279155));
#37566=CARTESIAN_POINT('Ctrl Pts',(-59.1827037214691,-18.6767477018707,
9.82592003357218));
#37567=CARTESIAN_POINT('Ctrl Pts',(-59.1828813434777,-18.67608480751,9.8400899910912));
#37568=CARTESIAN_POINT('Ctrl Pts',(-59.1830868741532,-18.6753177565863,
9.85424725658315));
#37569=CARTESIAN_POINT('Ctrl Pts',(-59.1844353908592,-18.670285023725,9.94713513804004));
#37570=CARTESIAN_POINT('Ctrl Pts',(-59.1869856677946,-18.6607672606286,
10.039633649266));
#37571=CARTESIAN_POINT('Ctrl Pts',(-59.1907077255756,-18.646876351881,10.1313703608465));
#37572=CARTESIAN_POINT('Ctrl Pts',(-59.1944191075557,-18.6330252857651,
10.2228439483884));
#37573=CARTESIAN_POINT('Ctrl Pts',(-59.1992956612747,-18.6148257395202,
10.3135610433039));
#37574=CARTESIAN_POINT('Ctrl Pts',(-59.2053202323396,-18.592341734212,10.40313539075));
#37575=CARTESIAN_POINT('Ctrl Pts',(-59.2112410580764,-18.5702449117395,
10.4911672350087));
#37576=CARTESIAN_POINT('Ctrl Pts',(-59.2182708207739,-18.5440094801873,
10.5780961320225));
#37577=CARTESIAN_POINT('Ctrl Pts',(-59.2264037185149,-18.513657092605,10.6635263254103));
#37578=CARTESIAN_POINT('Ctrl Pts',(-59.2303039431548,-18.499101256088,10.7044953570947));
#37579=CARTESIAN_POINT('Ctrl Pts',(-59.2344580112368,-18.483598062948,10.7451192120525));
#37580=CARTESIAN_POINT('Ctrl Pts',(-59.2388660433057,-18.4671470633053,
10.7853510160803));
#37581=CARTESIAN_POINT('Ctrl Pts',(-59.2403491922556,-18.4616118760692,
10.7988876140365));
#37582=CARTESIAN_POINT('Ctrl Pts',(-59.2418610960516,-18.4559693742862,
10.8123798086229));
#37583=CARTESIAN_POINT('Ctrl Pts',(-59.2434017709269,-18.4502194973737,
10.8258257520569));
#37584=CARTESIAN_POINT('Ctrl Pts',(-59.2448672509574,-18.4447502514423,
10.8386154469564));
#37585=CARTESIAN_POINT('Ctrl Pts',(-59.2463583029107,-18.4391855697962,
10.8513591674937));
#37586=CARTESIAN_POINT('Ctrl Pts',(-59.2478738643216,-18.4335294176084,
10.8640470911647));
#37587=CARTESIAN_POINT('Ctrl Pts',(-59.2575294210436,-18.3974943893469,
10.9448811410429));
#37588=CARTESIAN_POINT('Ctrl Pts',(-59.2681907320082,-18.3577058351517,
11.0235565033029));
#37589=CARTESIAN_POINT('Ctrl Pts',(-59.2798413570774,-18.3142251104531,
11.0997253730153));
#37590=CARTESIAN_POINT('Ctrl Pts',(-59.2912990836117,-18.271464292888,11.1746331204022));
#37591=CARTESIAN_POINT('Ctrl Pts',(-59.3037137499388,-18.2251321273963,
11.2471173604519));
#37592=CARTESIAN_POINT('Ctrl Pts',(-59.3170791891641,-18.1752516291421,
11.3168132013479));
#37593=CARTESIAN_POINT('Ctrl Pts',(-59.3300579262154,-18.1268143230484,
11.3844925328921));
#37594=CARTESIAN_POINT('Ctrl Pts',(-59.3439333260214,-18.0750306259972,
11.4495429412298));
#37595=CARTESIAN_POINT('Ctrl Pts',(-59.3587070801757,-18.0198942248749,
11.5115898436597));
#37596=CARTESIAN_POINT('Ctrl Pts',(-59.3613784504281,-18.009924535367,11.5228090806713));
#37597=CARTESIAN_POINT('Ctrl Pts',(-59.364079210104,-17.9998451630374,11.5339299971675));
#37598=CARTESIAN_POINT('Ctrl Pts',(-59.3668093915944,-17.9896559870014,
11.5449502145343));
#37599=CARTESIAN_POINT('Ctrl Pts',(-59.3747124158146,-17.9601614990781,
11.5768503080147));
#37600=CARTESIAN_POINT('Ctrl Pts',(-59.3828619650632,-17.9297469672238,
11.6079068412469));
#37601=CARTESIAN_POINT('Ctrl Pts',(-59.3912467107622,-17.8984546702664,
11.6380966037222));
#37602=CARTESIAN_POINT('Ctrl Pts',(-68.1281291851067,-15.0750265266586,
10.0024371765581));
#37603=CARTESIAN_POINT('Ctrl Pts',(-68.1132191003537,-15.0686010168709,
10.3130580784045));
#37604=CARTESIAN_POINT('Ctrl Pts',(-67.9995899840861,-15.2292608392572,
11.6285356954));
#37605=CARTESIAN_POINT('Ctrl Pts',(-67.3992512291332,-17.005006652638,13.4679206448304));
#37606=CARTESIAN_POINT('Ctrl Pts',(-66.3844685224501,-20.1882099452852,
12.7722321938656));
#37607=CARTESIAN_POINT('Ctrl Pts',(-65.9036218913761,-21.3787366757643,
9.61047736355945));
#37608=CARTESIAN_POINT('Ctrl Pts',(-66.2501895556749,-19.4813112170038,
6.79508159949504));
#37609=CARTESIAN_POINT('Ctrl Pts',(-66.9814704044654,-16.1481166073788,
6.8312269691009));
#37610=CARTESIAN_POINT('Ctrl Pts',(-67.2119040522751,-14.867652564341,8.81893895087719));
#37611=CARTESIAN_POINT('Ctrl Pts',(-67.1683025391241,-14.8112407741816,
9.90991228406425));
#37612=CARTESIAN_POINT('Ctrl Pts',(-67.1637176864735,-14.810555933805,9.9985514014054));
#37613=CARTESIAN_POINT('Origin',(-69.7479810832458,-18.6889152049569,10.));
#37614=CARTESIAN_POINT('Ctrl Pts',(-68.2083503098983,-15.0969161422106,
9.99673640007589));
#37615=CARTESIAN_POINT('Ctrl Pts',(-68.1711103559359,-15.0927295232038,
10.7130675867001));
#37616=CARTESIAN_POINT('Ctrl Pts',(-67.9289066052254,-15.6514186592596,
12.4513417391718));
#37617=CARTESIAN_POINT('Ctrl Pts',(-67.0483943376964,-18.3902480628716,
13.5944453497599));
#37618=CARTESIAN_POINT('Ctrl Pts',(-66.1687987195556,-21.0667649555472,
11.6442225433394));
#37619=CARTESIAN_POINT('Ctrl Pts',(-66.0360136384589,-20.9561469803458,
8.22016494780551));
#37620=CARTESIAN_POINT('Ctrl Pts',(-66.6336669557834,-18.1194957904379,
6.39071567224365));
#37621=CARTESIAN_POINT('Ctrl Pts',(-67.2173089746449,-15.4027596845031,
7.63681194520586));
#37622=CARTESIAN_POINT('Ctrl Pts',(-67.2747579502335,-14.8518622987657,
9.32892113065768));
#37623=CARTESIAN_POINT('Ctrl Pts',(-67.242349320473,-14.8383776097513,10.0022118830713));
#37624=CARTESIAN_POINT('Ctrl Pts',(-67.8425423025986,-17.2449834421528,
7.06170475438615));
#37625=CARTESIAN_POINT('Ctrl Pts',(-68.0419164156808,-16.2988495743022,
7.35795147289606));
#37626=CARTESIAN_POINT('Ctrl Pts',(-68.3551165744735,-14.7258515725219,
8.9714479727025));
#37627=CARTESIAN_POINT('Ctrl Pts',(-68.023655252025,-15.3567034243027,12.3283366156215));
#37628=CARTESIAN_POINT('Ctrl Pts',(-67.0483943376964,-18.3902480628716,
13.5944453497599));
#37629=CARTESIAN_POINT('Ctrl Pts',(-66.1687987195556,-21.0667649555472,
11.6442225433394));
#37630=CARTESIAN_POINT('Ctrl Pts',(-66.0360136384589,-20.9561469803458,
8.22016494780551));
#37631=CARTESIAN_POINT('Ctrl Pts',(-66.6336669557834,-18.1194957904379,
6.39071567224365));
#37632=CARTESIAN_POINT('Ctrl Pts',(-67.2905946547074,-15.0616295968131,
7.79327945411745));
#37633=CARTESIAN_POINT('Ctrl Pts',(-67.282863942121,-14.4843023646232,11.1722569386419));
#37634=CARTESIAN_POINT('Ctrl Pts',(-66.4816292855381,-16.8683721674343,
13.501327491299));
#37635=CARTESIAN_POINT('Ctrl Pts',(-65.468753391891,-20.0422978199461,12.6947822329671));
#37636=CARTESIAN_POINT('Ctrl Pts',(-65.0155990043222,-21.1273143736846,
9.47487431060658));
#37637=CARTESIAN_POINT('Ctrl Pts',(-65.3922823621304,-19.1153342996378,
6.72525821930933));
#37638=CARTESIAN_POINT('Ctrl Pts',(-66.1257396929252,-15.7718556315863,
6.90837057311376));
#37639=CARTESIAN_POINT('Ctrl Pts',(-66.4233986629546,-14.054798587767,9.86022990097523));
#37640=CARTESIAN_POINT('Ctrl Pts',(-65.8829690009265,-15.4655309000319,
12.9372608391343));
#37641=CARTESIAN_POINT('Ctrl Pts',(-64.8527215544619,-18.7042880702652,
13.3837942299378));
#37642=CARTESIAN_POINT('Ctrl Pts',(-64.1195886430846,-20.8341986998846,
10.7999310727628));
#37643=CARTESIAN_POINT('Ctrl Pts',(-64.2044184759423,-19.9114308093211,
7.49968047567736));
#37644=CARTESIAN_POINT('Ctrl Pts',(-64.895523082676,-16.726014659305,6.43862003923507));
#37645=CARTESIAN_POINT('Ctrl Pts',(-65.4382581333965,-14.0943212306267,
8.5669948761288));
#37646=CARTESIAN_POINT('Ctrl Pts',(-65.2108533475991,-14.3368288007657,
11.9787141005065));
#37647=CARTESIAN_POINT('Ctrl Pts',(-64.2812461473762,-17.1999914587382,
13.6183729089162));
#37648=CARTESIAN_POINT('Ctrl Pts',(-63.346239485481,-20.0833051820058,12.0175557753468));
#37649=CARTESIAN_POINT('Ctrl Pts',(-63.1074718691846,-20.3682194128847,
8.60989310618102));
#37650=CARTESIAN_POINT('Ctrl Pts',(-63.6430568297552,-17.7632104839245,
6.44715683087674));
#37651=CARTESIAN_POINT('Ctrl Pts',(-64.3376274439251,-14.5648590180568,
7.46621057361522));
#37652=CARTESIAN_POINT('Ctrl Pts',(-64.4334353369931,-13.60112044902,10.7544289031931));
#37653=CARTESIAN_POINT('Ctrl Pts',(-63.7089610525879,-15.6987166428561,
13.3670096553837));
#37654=CARTESIAN_POINT('Ctrl Pts',(-62.6772983776881,-18.9427555175135,
12.9642257537707));
#37655=CARTESIAN_POINT('Ctrl Pts',(-62.1266472347557,-20.391634915842,9.90679500749681));
#37656=CARTESIAN_POINT('Ctrl Pts',(-62.4144320750887,-18.7114286257302,
6.93283507366378));
#37657=CARTESIAN_POINT('Ctrl Pts',(-63.1472062543103,-15.3704995140596,
6.70571036393757));
#37658=CARTESIAN_POINT('Ctrl Pts',(-63.5330077514077,-13.3244900809144,
9.42882503807173));
#37659=CARTESIAN_POINT('Ctrl Pts',(-63.0906099643739,-14.3693624549398,
12.6634621126409));
#37660=CARTESIAN_POINT('Ctrl Pts',(-62.0804897947069,-17.5330036055459,
13.5128046754734));
#37661=CARTESIAN_POINT('Ctrl Pts',(-61.271554519541,-19.9458125081593,11.2162142452873));
#37662=CARTESIAN_POINT('Ctrl Pts',(-61.2525379570575,-19.4106046411911,
7.83042882970014));
#37663=CARTESIAN_POINT('Ctrl Pts',(-61.9047530097006,-16.3703262829251,
6.3876284598802));
#37664=CARTESIAN_POINT('Ctrl Pts',(-62.5083833543796,-13.5113685232515,
8.17992871548504));
#37665=CARTESIAN_POINT('Ctrl Pts',(-62.387123159886,-13.3577390856961,11.6022164308589));
#37666=CARTESIAN_POINT('Ctrl Pts',(-61.5138509672066,-16.0106566332719,
13.5896176377583));
#37667=CARTESIAN_POINT('Ctrl Pts',(-60.5349179618125,-19.0579057022677,
12.362301010972));
#37668=CARTESIAN_POINT('Ctrl Pts',(-60.1913020034495,-19.7341192728289,
9.01938609588879));
#37669=CARTESIAN_POINT('Ctrl Pts',(-60.6550135466889,-17.397345589062,6.55469600728472));
#37670=CARTESIAN_POINT('Ctrl Pts',(-61.3750552367846,-14.103934773716,7.1754379864718));
#37671=CARTESIAN_POINT('Ctrl Pts',(-61.5708627210562,-12.7669926495712,
10.3258507409626));
#37672=CARTESIAN_POINT('Ctrl Pts',(-60.9313710113774,-14.5474295567703,
13.1842383274678));
#37673=CARTESIAN_POINT('Ctrl Pts',(-59.8935459365978,-17.8144668208756,
13.1913616605738));
#37674=CARTESIAN_POINT('Ctrl Pts',(-59.2511484715134,-19.6057481548832,
10.3395770770153));
#37675=CARTESIAN_POINT('Ctrl Pts',(-59.4436819065864,-18.2810249486936,
7.18539898656524));
#37676=CARTESIAN_POINT('Ctrl Pts',(-60.1631753733452,-14.9896601306951,
6.54837069990788));
#37677=CARTESIAN_POINT('Ctrl Pts',(-60.629216203114,-12.644193431255,9.0096983771868));
#37678=CARTESIAN_POINT('Ctrl Pts',(-60.402326566927,-13.0868379849886,11.2296927240267));
#37679=CARTESIAN_POINT('Ctrl Pts',(-60.181950026368,-13.7072348830372,11.9973015569306));
#37680=CARTESIAN_POINT('Ctrl Pts',(-67.9318278742784,-17.3251900988194,
7.23888518457554));
#37681=CARTESIAN_POINT('Ctrl Pts',(-68.1161335763133,-16.4352923065867,
7.51726810226212));
#37682=CARTESIAN_POINT('Ctrl Pts',(-68.4043554971943,-14.9555143577762,
9.03347008941824));
#37683=CARTESIAN_POINT('Ctrl Pts',(-68.0837432245498,-15.5458770044745,
12.1879369455076));
#37684=CARTESIAN_POINT('Ctrl Pts',(-67.1581527442328,-18.3940490596784,
13.3776987943164));
#37685=CARTESIAN_POINT('Ctrl Pts',(-66.3224589027986,-20.9067222911426,
11.5450752374345));
#37686=CARTESIAN_POINT('Ctrl Pts',(-66.1885426111956,-20.8003260510249,
8.32748974461914));
#37687=CARTESIAN_POINT('Ctrl Pts',(-66.7410189775959,-18.1322775372969,
6.60835702425629));
#37688=CARTESIAN_POINT('Ctrl Pts',(-67.3491954556354,-15.2563533769438,
7.92634562444559));
#37689=CARTESIAN_POINT('Ctrl Pts',(-67.3327927019053,-14.7113906429076,
11.1015693557684));
#37690=CARTESIAN_POINT('Ctrl Pts',(-66.5707346233277,-16.9492514661366,
13.2901959816019));
#37691=CARTESIAN_POINT('Ctrl Pts',(-65.609797362651,-19.9293395015269,12.5322857391186));
#37692=CARTESIAN_POINT('Ctrl Pts',(-65.1748301675257,-20.9464805290194,
9.50653960894211));
#37693=CARTESIAN_POINT('Ctrl Pts',(-65.519661155234,-19.0533751185263,6.92272651604638));
#37694=CARTESIAN_POINT('Ctrl Pts',(-66.1997524963879,-15.9090610352115,
7.09479711845824));
#37695=CARTESIAN_POINT('Ctrl Pts',(-66.4703242998971,-14.2930946730788,
9.86865809630714));
#37696=CARTESIAN_POINT('Ctrl Pts',(-65.9533445658038,-15.6163106628566,
12.7601427840876));
#37697=CARTESIAN_POINT('Ctrl Pts',(-64.9760832641981,-18.6573208483795,
13.1797500249765));
#37698=CARTESIAN_POINT('Ctrl Pts',(-64.2780203671544,-20.656348402684,10.7516948950657));
#37699=CARTESIAN_POINT('Ctrl Pts',(-64.3485967193297,-19.786775226212,7.65045078699707));
#37700=CARTESIAN_POINT('Ctrl Pts',(-64.9888892233674,-16.7909924250963,
6.65337273791576));
#37701=CARTESIAN_POINT('Ctrl Pts',(-65.489758917571,-14.315542634016,8.65340568344645));
#37702=CARTESIAN_POINT('Ctrl Pts',(-65.266928528969,-14.5409783214079,11.8593968140381));
#37703=CARTESIAN_POINT('Ctrl Pts',(-64.3842388247345,-17.229042500588,13.4001835116647));
#37704=CARTESIAN_POINT('Ctrl Pts',(-63.496475248621,-19.9360426274119,11.8958963196673));
#37705=CARTESIAN_POINT('Ctrl Pts',(-63.2629672129436,-20.2013278361942,
8.69371713231446));
#37706=CARTESIAN_POINT('Ctrl Pts',(-63.7571179704187,-17.750953458357,6.66139475745692));
#37707=CARTESIAN_POINT('Ctrl Pts',(-64.4006674801973,-14.7430153463366,
7.61899913400456));
#37708=CARTESIAN_POINT('Ctrl Pts',(-64.4815599109683,-13.8349420404106,
10.7089365253204));
#37709=CARTESIAN_POINT('Ctrl Pts',(-63.7916335220747,-15.8036037329023,
13.1639775672764));
#37710=CARTESIAN_POINT('Ctrl Pts',(-62.8130423308995,-18.8495771338671,
12.7854817031123));
#37711=CARTESIAN_POINT('Ctrl Pts',(-62.2864574754684,-20.2086399244908,
9.91241530746228));
#37712=CARTESIAN_POINT('Ctrl Pts',(-62.5477505634248,-18.6273022002299,
7.11778639941));
#37713=CARTESIAN_POINT('Ctrl Pts',(-63.2271999473304,-15.4853839339817,
6.90435740451571));
#37714=CARTESIAN_POINT('Ctrl Pts',(-63.5805992467218,-13.5603011489527,
9.46326712676888));
#37715=CARTESIAN_POINT('Ctrl Pts',(-63.1557400246277,-14.5397187075309,
12.5028542351258));
#37716=CARTESIAN_POINT('Ctrl Pts',(-62.1973923166246,-17.5101424007747,
13.3009810867783));
#37717=CARTESIAN_POINT('Ctrl Pts',(-61.4280979699796,-19.7750093440881,
11.1428760184689));
#37718=CARTESIAN_POINT('Ctrl Pts',(-61.4010899078139,-19.2696261599638,
7.961254877169));
#37719=CARTESIAN_POINT('Ctrl Pts',(-62.0048379141108,-16.4102292811537,
6.60545597208742));
#37720=CARTESIAN_POINT('Ctrl Pts',(-62.5629308906206,-13.7212192931308,
8.28967977390814));
#37721=CARTESIAN_POINT('Ctrl Pts',(-62.4398445301463,-13.5744051997985,
11.5056021110761));
#37722=CARTESIAN_POINT('Ctrl Pts',(-61.6100928089778,-16.0649021365261,
13.3731621953643));
#37723=CARTESIAN_POINT('Ctrl Pts',(-60.6810516662197,-18.9259522392799,
12.2198532736367));
#37724=CARTESIAN_POINT('Ctrl Pts',(-60.3490176872815,-19.5589412741756,
9.07851752375991));
#37725=CARTESIAN_POINT('Ctrl Pts',(-60.7756290245013,-17.3606274442454,
6.76244927662476));
#37726=CARTESIAN_POINT('Ctrl Pts',(-61.4431136936918,-14.2633621012121,
7.34576025527735));
#37727=CARTESIAN_POINT('Ctrl Pts',(-61.6179756985622,-13.0045895703814,
10.3062018052243));
#37728=CARTESIAN_POINT('Ctrl Pts',(-61.0079073996548,-14.6752168136496,
12.9922274267496));
#37729=CARTESIAN_POINT('Ctrl Pts',(-60.0235254038855,-17.7428017915757,
12.9989212198949));
#37730=CARTESIAN_POINT('Ctrl Pts',(-59.4107265678367,-19.4236195381877,
10.3191004374816));
#37731=CARTESIAN_POINT('Ctrl Pts',(-59.5825119500424,-18.1763291194575,
7.35512060290596));
#37732=CARTESIAN_POINT('Ctrl Pts',(-60.249481453992,-15.0809863992773,6.75650538792386));
#37733=CARTESIAN_POINT('Ctrl Pts',(-60.6782816207909,-12.8745037461489,
9.06941397854074));
#37734=CARTESIAN_POINT('Ctrl Pts',(-60.4589813868428,-13.2888242651275,
11.1555417393123));
#37735=CARTESIAN_POINT('Ctrl Pts',(-60.2488475749171,-13.8709947795086,
11.8768634390787));
#37736=CARTESIAN_POINT('Ctrl Pts',(-68.0211134459581,-17.4053967554861,
7.41606561476494));
#37737=CARTESIAN_POINT('Ctrl Pts',(-68.1903507369458,-16.5717350388711,
7.67658473162818));
#37738=CARTESIAN_POINT('Ctrl Pts',(-68.4535944199152,-15.1851771430304,
9.09549220613397));
#37739=CARTESIAN_POINT('Ctrl Pts',(-68.1438311970747,-15.7350505846463,
12.0475372753936));
#37740=CARTESIAN_POINT('Ctrl Pts',(-67.2679111507692,-18.3978500564853,
13.160952238873));
#37741=CARTESIAN_POINT('Ctrl Pts',(-66.4761190860415,-20.746679626738,11.4459279315295));
#37742=CARTESIAN_POINT('Ctrl Pts',(-66.3410715839323,-20.644505121704,8.43481454143279));
#37743=CARTESIAN_POINT('Ctrl Pts',(-66.8483709994084,-18.1450592841558,
6.82599837626892));
#37744=CARTESIAN_POINT('Ctrl Pts',(-67.4077962565635,-15.4510771570746,
8.05941179477375));
#37745=CARTESIAN_POINT('Ctrl Pts',(-67.3827214616897,-14.9384789211918,
11.0308817728949));
#37746=CARTESIAN_POINT('Ctrl Pts',(-66.6598399611172,-17.030130764839,13.0790644719047));
#37747=CARTESIAN_POINT('Ctrl Pts',(-65.750841333411,-19.8163811831077,12.3697892452702));
#37748=CARTESIAN_POINT('Ctrl Pts',(-65.3340613307292,-20.7656466843542,
9.53820490727763));
#37749=CARTESIAN_POINT('Ctrl Pts',(-65.6470399483378,-18.9914159374149,
7.12019481278344));
#37750=CARTESIAN_POINT('Ctrl Pts',(-66.2737652998505,-16.0462664388367,
7.28122366380271));
#37751=CARTESIAN_POINT('Ctrl Pts',(-66.5172499368395,-14.5313907583905,
9.87708629163903));
#37752=CARTESIAN_POINT('Ctrl Pts',(-66.0237201306813,-15.7670904256813,
12.5830247290408));
#37753=CARTESIAN_POINT('Ctrl Pts',(-65.0994449739343,-18.6103536264938,
12.9757058200153));
#37754=CARTESIAN_POINT('Ctrl Pts',(-64.4364520912242,-20.4784981054834,
10.7034587173686));
#37755=CARTESIAN_POINT('Ctrl Pts',(-64.492774962717,-19.6621196431029,7.80122109831677));
#37756=CARTESIAN_POINT('Ctrl Pts',(-65.0822553640589,-16.8559701908876,
6.86812543659645));
#37757=CARTESIAN_POINT('Ctrl Pts',(-65.5412597017456,-14.5367640374053,
8.73981649076409));
#37758=CARTESIAN_POINT('Ctrl Pts',(-65.323003710339,-14.7451278420501,11.7400795275698));
#37759=CARTESIAN_POINT('Ctrl Pts',(-64.4872315020927,-17.2580935424379,
13.1819941144132));
#37760=CARTESIAN_POINT('Ctrl Pts',(-63.6467110117609,-19.7887800728179,
11.7742368639878));
#37761=CARTESIAN_POINT('Ctrl Pts',(-63.4184625567026,-20.0344362595037,
8.7775411584479));
#37762=CARTESIAN_POINT('Ctrl Pts',(-63.8711791110824,-17.7386964327895,
6.87563268403709));
#37763=CARTESIAN_POINT('Ctrl Pts',(-64.4637075164694,-14.9211716746165,
7.7717876943939));
#37764=CARTESIAN_POINT('Ctrl Pts',(-64.5296844849434,-14.0687636318011,
10.6634441474477));
#37765=CARTESIAN_POINT('Ctrl Pts',(-63.8743059915617,-15.9084908229485,
12.9609454791691));
#37766=CARTESIAN_POINT('Ctrl Pts',(-62.9487862841107,-18.7563987502208,
12.6067376524538));
#37767=CARTESIAN_POINT('Ctrl Pts',(-62.4462677161811,-20.0256449331395,
9.91803560742777));
#37768=CARTESIAN_POINT('Ctrl Pts',(-62.6810690517609,-18.5431757747297,
7.30273772515621));
#37769=CARTESIAN_POINT('Ctrl Pts',(-63.3071936403506,-15.6002683539037,
7.10300444509384));
#37770=CARTESIAN_POINT('Ctrl Pts',(-63.6281907420358,-13.7961122169911,
9.49770921546603));
#37771=CARTESIAN_POINT('Ctrl Pts',(-63.2208700848815,-14.7100749601221,
12.3422463576107));
#37772=CARTESIAN_POINT('Ctrl Pts',(-62.3142948385422,-17.4872811960035,
13.0891574980832));
#37773=CARTESIAN_POINT('Ctrl Pts',(-61.5846414204184,-19.6042061800169,
11.0695377916504));
#37774=CARTESIAN_POINT('Ctrl Pts',(-61.5496418585701,-19.1286476787364,
8.09208092463788));
#37775=CARTESIAN_POINT('Ctrl Pts',(-62.1049228185211,-16.4501322793822,
6.82328348429463));
#37776=CARTESIAN_POINT('Ctrl Pts',(-62.6174784268616,-13.9310700630102,
8.39943083233125));
#37777=CARTESIAN_POINT('Ctrl Pts',(-62.4925659004067,-13.7910713139008,
11.4089877912933));
#37778=CARTESIAN_POINT('Ctrl Pts',(-61.706334650749,-16.1191476397804,13.1567067529704));
#37779=CARTESIAN_POINT('Ctrl Pts',(-60.827185370627,-18.7939987762922,12.0774055363014));
#37780=CARTESIAN_POINT('Ctrl Pts',(-60.5067333711136,-19.3837632755223,
9.13764895163106));
#37781=CARTESIAN_POINT('Ctrl Pts',(-60.8962445023137,-17.3239092994289,
6.97020254596478));
#37782=CARTESIAN_POINT('Ctrl Pts',(-61.5111721505989,-14.4227894287083,
7.51608252408292));
#37783=CARTESIAN_POINT('Ctrl Pts',(-61.6650886760682,-13.2421864911916,
10.286552869486));
#37784=CARTESIAN_POINT('Ctrl Pts',(-61.0844437879323,-14.8030040705288,
12.8002165260314));
#37785=CARTESIAN_POINT('Ctrl Pts',(-60.1535048711732,-17.6711367622757,
12.8064807792161));
#37786=CARTESIAN_POINT('Ctrl Pts',(-59.5703046641601,-19.2414909214922,
10.2986237979478));
#37787=CARTESIAN_POINT('Ctrl Pts',(-59.7213419934984,-18.0716332902213,
7.5248422192467));
#37788=CARTESIAN_POINT('Ctrl Pts',(-60.3357875346389,-15.1723126678596,
6.96464007593981));
#37789=CARTESIAN_POINT('Ctrl Pts',(-60.7273470384677,-13.1048140610427,
9.12912957989471));
#37790=CARTESIAN_POINT('Ctrl Pts',(-60.5156362067586,-13.4908105452664,
11.081390754598));
#37791=CARTESIAN_POINT('Ctrl Pts',(-60.3157451234662,-14.0347546759801,
11.7564253212268));
#37792=CARTESIAN_POINT('Ctrl Pts',(-68.1103990176379,-17.4856034121527,
7.59324604495433));
#37793=CARTESIAN_POINT('Ctrl Pts',(-68.2645678975783,-16.7081777711556,
7.83590136099424));
#37794=CARTESIAN_POINT('Ctrl Pts',(-68.5028333426361,-15.4148399282847,
9.1575143228497));
#37795=CARTESIAN_POINT('Ctrl Pts',(-68.2039191695995,-15.9242241648182,
11.9071376052797));
#37796=CARTESIAN_POINT('Ctrl Pts',(-67.3776695573056,-18.4016510532921,
12.9442056834295));
#37797=CARTESIAN_POINT('Ctrl Pts',(-66.6297792692844,-20.5866369623334,
11.3467806256245));
#37798=CARTESIAN_POINT('Ctrl Pts',(-66.4936005566689,-20.4886841923831,
8.54213933824642));
#37799=CARTESIAN_POINT('Ctrl Pts',(-66.9557230212209,-18.1578410310147,
7.04363972828156));
#37800=CARTESIAN_POINT('Ctrl Pts',(-67.4663970574915,-15.6458009372053,
8.19247796510189));
#37801=CARTESIAN_POINT('Ctrl Pts',(-67.4326502214741,-15.1655671994762,
10.9601941900214));
#37802=CARTESIAN_POINT('Ctrl Pts',(-66.7489452989067,-17.1110100635413,
12.8679329622076));
#37803=CARTESIAN_POINT('Ctrl Pts',(-65.891885304171,-19.7034228646885,12.2072927514217));
#37804=CARTESIAN_POINT('Ctrl Pts',(-65.4932924939327,-20.584812839689,9.56987020561317));
#37805=CARTESIAN_POINT('Ctrl Pts',(-65.7744187414414,-18.9294567563035,
7.31766310952049));
#37806=CARTESIAN_POINT('Ctrl Pts',(-66.3477781033132,-16.1834718424619,
7.46765020914719));
#37807=CARTESIAN_POINT('Ctrl Pts',(-66.5641755737819,-14.7696868437023,
9.88551448697093));
#37808=CARTESIAN_POINT('Ctrl Pts',(-66.0940956955586,-15.917870188506,12.4059066739941));
#37809=CARTESIAN_POINT('Ctrl Pts',(-65.2228066836706,-18.5633864046081,
12.771661615054));
#37810=CARTESIAN_POINT('Ctrl Pts',(-64.5948838152939,-20.3006478082828,
10.6552225396715));
#37811=CARTESIAN_POINT('Ctrl Pts',(-64.6369532061044,-19.5374640599938,
7.95199140963649));
#37812=CARTESIAN_POINT('Ctrl Pts',(-65.1756215047503,-16.9209479566789,
7.08287813527712));
#37813=CARTESIAN_POINT('Ctrl Pts',(-65.5927604859202,-14.7579854407947,
8.82622729808175));
#37814=CARTESIAN_POINT('Ctrl Pts',(-65.3790788917089,-14.9492773626923,
11.6207622411014));
#37815=CARTESIAN_POINT('Ctrl Pts',(-64.5902241794511,-17.2871445842876,
12.9638047171617));
#37816=CARTESIAN_POINT('Ctrl Pts',(-63.7969467749009,-19.641517518224,11.6525774083083));
#37817=CARTESIAN_POINT('Ctrl Pts',(-63.5739579004616,-19.8675446828132,
8.86136518458133));
#37818=CARTESIAN_POINT('Ctrl Pts',(-63.985240251746,-17.726439407222,7.08987061061728));
#37819=CARTESIAN_POINT('Ctrl Pts',(-64.5267475527415,-15.0993280028964,
7.92457625478324));
#37820=CARTESIAN_POINT('Ctrl Pts',(-64.5778090589186,-14.3025852231916,
10.617951769575));
#37821=CARTESIAN_POINT('Ctrl Pts',(-63.9569784610485,-16.0133779129947,
12.7579133910618));
#37822=CARTESIAN_POINT('Ctrl Pts',(-63.084530237322,-18.6632203665744,12.4279936017953));
#37823=CARTESIAN_POINT('Ctrl Pts',(-62.6060779568938,-19.8426499417882,
9.92365590739326));
#37824=CARTESIAN_POINT('Ctrl Pts',(-62.8143875400971,-18.4590493492295,
7.48768905090242));
#37825=CARTESIAN_POINT('Ctrl Pts',(-63.3871873333707,-15.7151527738257,
7.30165148567198));
#37826=CARTESIAN_POINT('Ctrl Pts',(-63.6757822373498,-14.0319232850294,
9.53215130416319));
#37827=CARTESIAN_POINT('Ctrl Pts',(-63.2860001451353,-14.8804312127132,
12.1816384800955));
#37828=CARTESIAN_POINT('Ctrl Pts',(-62.4311973604599,-17.4644199912323,
12.8773339093881));
#37829=CARTESIAN_POINT('Ctrl Pts',(-61.7411848708572,-19.4334030159457,
10.9961995648319));
#37830=CARTESIAN_POINT('Ctrl Pts',(-61.6981938093263,-18.987669197509,8.22290697210676));
#37831=CARTESIAN_POINT('Ctrl Pts',(-62.2050077229314,-16.4900352776108,
7.04111099650183));
#37832=CARTESIAN_POINT('Ctrl Pts',(-62.6720259631026,-14.1409208328895,
8.50918189075437));
#37833=CARTESIAN_POINT('Ctrl Pts',(-62.545287270667,-14.0077374280031,11.3123734715104));
#37834=CARTESIAN_POINT('Ctrl Pts',(-61.8025764925202,-16.1733931430346,
12.9402513105764));
#37835=CARTESIAN_POINT('Ctrl Pts',(-60.9733190750343,-18.6620453133045,
11.934957798966));
#37836=CARTESIAN_POINT('Ctrl Pts',(-60.6644490549456,-19.2085852768689,
9.1967803795022));
#37837=CARTESIAN_POINT('Ctrl Pts',(-61.016859980126,-17.2871911546123,7.17795581530479));
#37838=CARTESIAN_POINT('Ctrl Pts',(-61.5792306075061,-14.5822167562045,
7.68640479288848));
#37839=CARTESIAN_POINT('Ctrl Pts',(-61.7122016535742,-13.4797834120018,
10.2669039337477));
#37840=CARTESIAN_POINT('Ctrl Pts',(-61.1609801762097,-14.930791327408,12.6082056253132));
#37841=CARTESIAN_POINT('Ctrl Pts',(-60.2834843384609,-17.5994717329758,
12.6140403385373));
#37842=CARTESIAN_POINT('Ctrl Pts',(-59.7298827604835,-19.0593623047967,
10.2781471584142));
#37843=CARTESIAN_POINT('Ctrl Pts',(-59.8601720369543,-17.9669374609851,
7.69456383558743));
#37844=CARTESIAN_POINT('Ctrl Pts',(-60.4220936152857,-15.2636389364418,
7.17277476395578));
#37845=CARTESIAN_POINT('Ctrl Pts',(-60.7764124561446,-13.3351243759365,
9.18884518124866));
#37846=CARTESIAN_POINT('Ctrl Pts',(-60.5722910266744,-13.6927968254053,
11.0072397698836));
#37847=CARTESIAN_POINT('Ctrl Pts',(-60.3826426720152,-14.1985145724515,
11.6359872033749));
#37848=CARTESIAN_POINT('Ctrl Pts',(-67.8425423025986,-17.2449834421528,
7.06170475438614));
#37849=CARTESIAN_POINT('Ctrl Pts',(-67.936339604961,-16.8759806260738,7.20780006417493));
#37850=CARTESIAN_POINT('Ctrl Pts',(-68.0195197262117,-16.5358040823885,
7.42431456480024));
#37851=CARTESIAN_POINT('Ctrl Pts',(-68.1509980806491,-15.9848167458475,
7.95780764621782));
#37852=CARTESIAN_POINT('Ctrl Pts',(-68.2006822338607,-15.769941108176,8.25968161903171));
#37853=CARTESIAN_POINT('Ctrl Pts',(-68.2646302810789,-15.490561932004,8.88066242679753));
#37854=CARTESIAN_POINT('Ctrl Pts',(-68.2826595052327,-15.410358466988,9.1849782015739));
#37855=CARTESIAN_POINT('Ctrl Pts',(-68.2943569622715,-15.358433741901,9.79677072277298));
#37856=CARTESIAN_POINT('Ctrl Pts',(-68.288855628865,-15.3830449856443,10.0982078060305));
#37857=CARTESIAN_POINT('Ctrl Pts',(-68.2546420063796,-15.5341550196633,
10.6858944634119));
#37858=CARTESIAN_POINT('Ctrl Pts',(-68.2257386849337,-15.661414646539,10.9661810334236));
#37859=CARTESIAN_POINT('Ctrl Pts',(-68.1449424659488,-16.0093499903206,
11.4722931322538));
#37860=CARTESIAN_POINT('Ctrl Pts',(-68.093295210955,-16.2286900565759,11.6926718707978));
#37861=CARTESIAN_POINT('Ctrl Pts',(-68.0322473001841,-16.4806955947434,
11.8669181223572));
#37862=CARTESIAN_POINT('Ctrl Pts',(-60.3826426720152,-14.1985145724515,
11.6359872033749));
#37863=CARTESIAN_POINT('Ctrl Pts',(-60.3987291200758,-14.1384791309761,
11.5775783984681));
#37864=CARTESIAN_POINT('Ctrl Pts',(-60.4139429451876,-14.0817003626815,
11.5159169743219));
#37865=CARTESIAN_POINT('Ctrl Pts',(-60.428280614173,-14.0281914535657,11.4513790591597));
#37866=CARTESIAN_POINT('Ctrl Pts',(-60.4429682456437,-13.9733764666745,
11.3852658635805));
#37867=CARTESIAN_POINT('Ctrl Pts',(-60.4567365493831,-13.9219924575848,
11.3161335496817));
#37868=CARTESIAN_POINT('Ctrl Pts',(-60.4695742653767,-13.8740814492437,
11.244340195927));
#37869=CARTESIAN_POINT('Ctrl Pts',(-60.4729336106422,-13.8615442020328,
11.2255534691331));
#37870=CARTESIAN_POINT('Ctrl Pts',(-60.4762291892638,-13.8492449351765,
11.2065843091488));
#37871=CARTESIAN_POINT('Ctrl Pts',(-60.4794607015,-13.8371847673257,11.1874386952136));
#37872=CARTESIAN_POINT('Ctrl Pts',(-60.4820790008577,-13.8274131410933,
11.1719261595939));
#37873=CARTESIAN_POINT('Ctrl Pts',(-60.4846553435987,-13.8177980990861,
11.156296950855));
#37874=CARTESIAN_POINT('Ctrl Pts',(-60.4871873137292,-13.808348657916,11.1405686300786));
#37875=CARTESIAN_POINT('Ctrl Pts',(-60.4994718284845,-13.7625022247027,
11.0642585716257));
#37876=CARTESIAN_POINT('Ctrl Pts',(-60.5107256649652,-13.7205023351767,
10.9855425561623));
#37877=CARTESIAN_POINT('Ctrl Pts',(-60.5209393772212,-13.6823842421036,
10.9048124952827));
#37878=CARTESIAN_POINT('Ctrl Pts',(-60.5290925934916,-13.6519560247373,
10.8403687720428));
#37879=CARTESIAN_POINT('Ctrl Pts',(-60.5365828861053,-13.6240018721396,
10.7746405675613));
#37880=CARTESIAN_POINT('Ctrl Pts',(-60.5434011779566,-13.5985556605296,
10.7078100772199));
#37881=CARTESIAN_POINT('Ctrl Pts',(-60.5456026098314,-13.5903398049234,
10.6862324189363));
#37882=CARTESIAN_POINT('Ctrl Pts',(-60.5477339564827,-13.582385510932,10.6645397516012));
#37883=CARTESIAN_POINT('Ctrl Pts',(-60.5497948184315,-13.574694269432,10.6427379433821));
#37884=CARTESIAN_POINT('Ctrl Pts',(-60.5517587834915,-13.5673646520437,
10.6219612049815));
#37885=CARTESIAN_POINT('Ctrl Pts',(-60.553659151552,-13.5602723818886,10.6010802047041));
#37886=CARTESIAN_POINT('Ctrl Pts',(-60.5554929869735,-13.5534284149229,
10.5801302249072));
#37887=CARTESIAN_POINT('Ctrl Pts',(-60.5631434154496,-13.5248766271506,
10.4927307123161));
#37888=CARTESIAN_POINT('Ctrl Pts',(-60.569645182982,-13.5006117003807,10.4040498988215));
#37889=CARTESIAN_POINT('Ctrl Pts',(-60.5749893942622,-13.4806668323564,
10.3144849191128));
#37890=CARTESIAN_POINT('Ctrl Pts',(-60.5804161086929,-13.4604140583831,
10.2235372483755));
#37891=CARTESIAN_POINT('Ctrl Pts',(-60.5846493808354,-13.4446152716651,
10.1316770969848));
#37892=CARTESIAN_POINT('Ctrl Pts',(-60.5876690820109,-13.4333455934544,
10.0392871196303));
#37893=CARTESIAN_POINT('Ctrl Pts',(-60.5906654794535,-13.4221628859587,
9.94761013711361));
#37894=CARTESIAN_POINT('Ctrl Pts',(-60.5924670545743,-13.4154393160742,
9.85541054674054));
#37895=CARTESIAN_POINT('Ctrl Pts',(-60.5930419859763,-13.4132936428713,
9.76304299840633));
#37896=CARTESIAN_POINT('Ctrl Pts',(-60.5933185830197,-13.4122613686522,
9.71860536517465));
#37897=CARTESIAN_POINT('Ctrl Pts',(-60.5933110802673,-13.4122893693051,
9.67412865771307));
#37898=CARTESIAN_POINT('Ctrl Pts',(-60.593014824197,-13.4133950120118,9.62965173452372));
#37899=CARTESIAN_POINT('Ctrl Pts',(-60.5929169928494,-13.4137601235713,
9.61496431453743));
#37900=CARTESIAN_POINT('Ctrl Pts',(-60.5927876671156,-13.4142427737806,
9.60027687017834));
#37901=CARTESIAN_POINT('Ctrl Pts',(-60.592626660992,-13.4148436568143,9.58559080055877));
#37902=CARTESIAN_POINT('Ctrl Pts',(-60.5924638798191,-13.4154511644222,
9.57074282096179));
#37903=CARTESIAN_POINT('Ctrl Pts',(-60.5922688054843,-13.4161791917507,
9.55590504919177));
#37904=CARTESIAN_POINT('Ctrl Pts',(-60.5920414435149,-13.4170277181723,
9.5410835717059));
#37905=CARTESIAN_POINT('Ctrl Pts',(-60.5905760164193,-13.4224967665479,
9.44555398617054));
#37906=CARTESIAN_POINT('Ctrl Pts',(-60.5877696251689,-13.4329703612802,
9.35064220193598));
#37907=CARTESIAN_POINT('Ctrl Pts',(-60.5836035770972,-13.4485182643508,
9.256742983847));
#37908=CARTESIAN_POINT('Ctrl Pts',(-60.5832473073958,-13.4498478809775,
9.24871296455522));
#37909=CARTESIAN_POINT('Ctrl Pts',(-60.5828810865857,-13.4512146356476,
9.24069033913143));
#37910=CARTESIAN_POINT('Ctrl Pts',(-60.5825048986307,-13.4526185882087,
9.23267534878088));
#37911=CARTESIAN_POINT('Ctrl Pts',(-60.5782789204955,-13.4683901533212,
9.14263744743344));
#37912=CARTESIAN_POINT('Ctrl Pts',(-60.5727962781624,-13.4888516530677,
9.05356331283212));
#37913=CARTESIAN_POINT('Ctrl Pts',(-60.5661351124401,-13.5137114619812,
8.9656877172483));
#37914=CARTESIAN_POINT('Ctrl Pts',(-60.559321511335,-13.5391401674879,8.87580115982938));
#37915=CARTESIAN_POINT('Ctrl Pts',(-60.5512747790297,-13.5691709812862,
8.78716792582501));
#37916=CARTESIAN_POINT('Ctrl Pts',(-60.5420644900995,-13.6035442475259,
8.70004212728124));
#37917=CARTESIAN_POINT('Ctrl Pts',(-60.5370098857273,-13.6224082878551,
8.65222750978226));
#37918=CARTESIAN_POINT('Ctrl Pts',(-60.5316045998671,-13.642581089315,8.60486701429381));
#37919=CARTESIAN_POINT('Ctrl Pts',(-60.5258584913669,-13.6640258581837,
8.5580041989488));
#37920=CARTESIAN_POINT('Ctrl Pts',(-60.5241489330315,-13.6704060167496,
8.54406176876562));
#37921=CARTESIAN_POINT('Ctrl Pts',(-60.5224089382015,-13.6768997658602,
8.53016150108827));
#37922=CARTESIAN_POINT('Ctrl Pts',(-60.5206408848662,-13.6834982307381,
8.51632087102361));
#37923=CARTESIAN_POINT('Ctrl Pts',(-60.5095968739651,-13.7247150405403,
8.42986642631845));
#37924=CARTESIAN_POINT('Ctrl Pts',(-60.4974435461318,-13.7700718774953,
8.34560744647309));
#37925=CARTESIAN_POINT('Ctrl Pts',(-60.4842687953746,-13.819240716698,8.2637970858888));
#37926=CARTESIAN_POINT('Ctrl Pts',(-60.470834261757,-13.8693790787351,8.18037356920902));
#37927=CARTESIAN_POINT('Ctrl Pts',(-60.4563375467057,-13.9234815558493,
8.09949541141806));
#37928=CARTESIAN_POINT('Ctrl Pts',(-60.4408576353906,-13.981253371374,8.02143790706986));
#37929=CARTESIAN_POINT('Ctrl Pts',(-60.4252551513805,-14.0394826344241,
7.9427623294991));
#37930=CARTESIAN_POINT('Ctrl Pts',(-60.4086537217477,-14.1014400132919,
7.86695140891473));
#37931=CARTESIAN_POINT('Ctrl Pts',(-60.3911214682024,-14.1668712742941,
7.79430622909878));
#37932=CARTESIAN_POINT('Ctrl Pts',(-60.3818445739541,-14.2014931149651,
7.75586726578716));
#37933=CARTESIAN_POINT('Ctrl Pts',(-60.3723068631306,-14.2370883363464,
7.71831505012366));
#37934=CARTESIAN_POINT('Ctrl Pts',(-60.3625171761545,-14.2736239455313,
7.68169758973832));
#37935=CARTESIAN_POINT('Ctrl Pts',(-60.3590313767661,-14.2866331259538,
7.66865926467973));
#37936=CARTESIAN_POINT('Ctrl Pts',(-60.3555136232663,-14.2997615607436,
7.65573947798149));
#37937=CARTESIAN_POINT('Ctrl Pts',(-60.351964291066,-14.3130078488481,7.64294048662165));
#37938=CARTESIAN_POINT('Ctrl Pts',(-60.34923729056,-14.3231851532886,7.63310684639187));
#37939=CARTESIAN_POINT('Ctrl Pts',(-60.3464919180926,-14.3334310228227,
7.6233455630969));
#37940=CARTESIAN_POINT('Ctrl Pts',(-60.3437307201908,-14.343735953682,7.61366571166803));
#37941=CARTESIAN_POINT('Ctrl Pts',(-60.3241830915898,-14.4166886967885,
7.54513815682638));
#37942=CARTESIAN_POINT('Ctrl Pts',(-60.3038121514937,-14.4927140802252,
7.48057696466926));
#37943=CARTESIAN_POINT('Ctrl Pts',(-60.2827016033741,-14.5714997183832,
7.42026730042969));
#37944=CARTESIAN_POINT('Ctrl Pts',(-60.261564320459,-14.650385132156,7.35988125889639));
#37945=CARTESIAN_POINT('Ctrl Pts',(-60.2396854085589,-14.7320383429816,
7.30375667607862));
#37946=CARTESIAN_POINT('Ctrl Pts',(-60.2171371866631,-14.8161894527173,
7.25220561234172));
#37947=CARTESIAN_POINT('Ctrl Pts',(-60.1950163808933,-14.8987454237543,
7.20163173235182));
#37948=CARTESIAN_POINT('Ctrl Pts',(-60.1722512298629,-14.9837061240419,
7.15545893555081));
#37949=CARTESIAN_POINT('Ctrl Pts',(-60.1489011523676,-15.0708497996151,
7.11401788932665));
#37950=CARTESIAN_POINT('Ctrl Pts',(-60.141634689533,-15.0979686081049,7.10112157999862));
#37951=CARTESIAN_POINT('Ctrl Pts',(-60.134311524735,-15.1252990312032,7.08868381628556));
#37952=CARTESIAN_POINT('Ctrl Pts',(-60.1269333077645,-15.1528349118066,
7.07671545672067));
#37953=CARTESIAN_POINT('Ctrl Pts',(-60.1158687531571,-15.1941283917646,
7.05876741202428));
#37954=CARTESIAN_POINT('Ctrl Pts',(-60.1046804027641,-15.2358838838839,
7.04187489341869));
#37955=CARTESIAN_POINT('Ctrl Pts',(-60.0933772939442,-15.2780676602833,
7.02603075613033));
#37956=CARTESIAN_POINT('Ctrl Pts',(-67.4086397233445,-15.458048217099,10.0018117506529));
#37957=CARTESIAN_POINT('Ctrl Pts',(-67.3922281881599,-15.4516726940089,
10.2792252787836));
#37958=CARTESIAN_POINT('Ctrl Pts',(-67.3643426917121,-15.488118577317,10.556071912701));
#37959=CARTESIAN_POINT('Ctrl Pts',(-67.3243238737158,-15.5698466331086,
10.8168646145659));
#37960=CARTESIAN_POINT('Ctrl Pts',(-67.2047485806183,-15.8140481541645,
11.5961071140835));
#37961=CARTESIAN_POINT('Ctrl Pts',(-66.9768469397625,-16.4625291088529,
12.2320200381456));
#37962=CARTESIAN_POINT('Ctrl Pts',(-66.7200527868787,-17.2188383863883,
12.4398697983789));
#37963=CARTESIAN_POINT('Ctrl Pts',(-66.4632586339948,-17.9751476639237,
12.6477195586123));
#37964=CARTESIAN_POINT('Ctrl Pts',(-66.1775719690829,-18.8392852643061,
12.427506155017));
#37965=CARTESIAN_POINT('Ctrl Pts',(-65.9682965015872,-19.4182523936641,
11.8778290289179));
#37966=CARTESIAN_POINT('Ctrl Pts',(-65.7590210340915,-19.997219523022,11.3281519028188));
#37967=CARTESIAN_POINT('Ctrl Pts',(-65.6261567640121,-20.2910161813555,
10.449011054216));
#37968=CARTESIAN_POINT('Ctrl Pts',(-65.6065790035572,-20.162021829958,9.63407278056581));
#37969=CARTESIAN_POINT('Ctrl Pts',(-65.5870012431023,-20.0330274785605,
8.81913450691562));
#37970=CARTESIAN_POINT('Ctrl Pts',(-65.6807099922718,-19.481242117432,8.06839880821806));
#37971=CARTESIAN_POINT('Ctrl Pts',(-65.8231242605019,-18.7476852845608,
7.71802880880706));
#37972=CARTESIAN_POINT('Ctrl Pts',(-65.965538528732,-18.0141284516896,7.36765880939607));
#37973=CARTESIAN_POINT('Ctrl Pts',(-66.1566583160226,-17.0988001470757,
7.41765450927163));
#37974=CARTESIAN_POINT('Ctrl Pts',(-66.288284454746,-16.4055051616422,7.8456297388467));
#37975=CARTESIAN_POINT('Ctrl Pts',(-66.4199105934695,-15.7122101762087,
8.27360496842178));
#37976=CARTESIAN_POINT('Ctrl Pts',(-66.4920430836257,-15.2409485099555,
9.07955972769635));
#37977=CARTESIAN_POINT('Ctrl Pts',(-66.4497626823332,-15.1966815676295,
9.90260247183749));
#37978=CARTESIAN_POINT('Ctrl Pts',(-66.4481055265244,-15.1949465504969,
9.93486115488347));
#37979=CARTESIAN_POINT('Ctrl Pts',(-66.4462726093384,-15.1938674837542,
9.96714608853563));
#37980=CARTESIAN_POINT('Ctrl Pts',(-66.4442667934687,-15.1934336836835,
9.99943462192771));
#37981=CARTESIAN_POINT('Ctrl Pts',(-20.25986904378,67.0040126136404,11.1728309286208));
#37982=CARTESIAN_POINT('Ctrl Pts',(-20.6173045957293,66.854289394458,10.4434664543485));
#37983=CARTESIAN_POINT('Ctrl Pts',(-20.5807180172414,66.7561954352347,8.59013022403081));
#37984=CARTESIAN_POINT('Ctrl Pts',(-18.2866570474721,67.2090412643978,7.05024279158514));
#37985=CARTESIAN_POINT('Ctrl Pts',(-15.7623446338521,67.7235827819969,8.14059085434233));
#37986=CARTESIAN_POINT('Ctrl Pts',(-15.216861454864,67.7078986042171,10.8824467802982));
#37987=CARTESIAN_POINT('Ctrl Pts',(-17.0999173665985,67.0414893382909,12.8405694561119));
#37988=CARTESIAN_POINT('Ctrl Pts',(-19.6999556621849,66.1829652216242,12.270731917377));
#37989=CARTESIAN_POINT('Ctrl Pts',(-20.6677950818131,65.7617874756574,9.68094249642523));
#37990=CARTESIAN_POINT('Ctrl Pts',(-19.1062967313387,66.0183437425753,7.37485535276711));
#37991=CARTESIAN_POINT('Ctrl Pts',(-16.3687616678975,66.5900180970018,7.40446197973337));
#37992=CARTESIAN_POINT('Ctrl Pts',(-14.8547867084588,66.83384050967,9.74329926128818));
#37993=CARTESIAN_POINT('Ctrl Pts',(-15.8753739824799,66.3985290187163,12.3105450512028));
#37994=CARTESIAN_POINT('Ctrl Pts',(-18.4864972623911,65.5370346894516,12.8220707222439));
#37995=CARTESIAN_POINT('Ctrl Pts',(-20.3290217552966,64.8814857844687,10.8227823754311));
#37996=CARTESIAN_POINT('Ctrl Pts',(-19.7276391663451,64.8807798084461,8.09145561890055));
#37997=CARTESIAN_POINT('Ctrl Pts',(-17.1814057921381,65.4011950297316,7.0581771851638));
#37998=CARTESIAN_POINT('Ctrl Pts',(-14.9197267037703,65.8453641599238,8.64226139479096));
#37999=CARTESIAN_POINT('Ctrl Pts',(-14.9188369907852,65.6837566027254,11.4343367521439));
#38000=CARTESIAN_POINT('Ctrl Pts',(-17.1435292903637,64.9258061425711,12.950271123299));
#38001=CARTESIAN_POINT('Ctrl Pts',(-19.5784782321595,64.1115175849317,11.8413258175014));
#38002=CARTESIAN_POINT('Ctrl Pts',(-20.0212914063393,63.8310201974379,9.09413821413813));
#38003=CARTESIAN_POINT('Ctrl Pts',(-18.0419954959312,64.1995249831397,7.15290308224175));
#38004=CARTESIAN_POINT('Ctrl Pts',(-15.3655869450733,64.7548205378834,7.74475277436873));
#38005=CARTESIAN_POINT('Ctrl Pts',(-14.3372888766999,64.8685062198083,10.3431139119316));
#38006=CARTESIAN_POINT('Ctrl Pts',(-15.8359873727446,64.305085213021,12.6362038638412));
#38007=CARTESIAN_POINT('Ctrl Pts',(-18.4922795208015,63.4314879220137,12.5838422163727));
#38008=CARTESIAN_POINT('Ctrl Pts',(-19.9068421044142,62.8906110650171,10.2326155433119));
#38009=CARTESIAN_POINT('Ctrl Pts',(-18.7851286033011,63.029327336705,7.67442896667237));
#38010=CARTESIAN_POINT('Ctrl Pts',(-16.0891375551554,63.5898700057829,7.1853214836325));
#38011=CARTESIAN_POINT('Ctrl Pts',(-14.1815147862765,63.9391700310929,9.20045592301428));
#38012=CARTESIAN_POINT('Ctrl Pts',(-14.7234885765209,63.6321026366037,11.926951102987));
#38013=CARTESIAN_POINT('Ctrl Pts',(-17.1968616153839,62.8075183731852,12.9390225214355));
#38014=CARTESIAN_POINT('Ctrl Pts',(-19.3650552728408,62.0647066785609,11.3362221619437));
#38015=CARTESIAN_POINT('Ctrl Pts',(-19.2630114600595,61.9302032807139,8.54457429525404));
#38016=CARTESIAN_POINT('Ctrl Pts',(-16.9455204456759,62.3893271714101,7.04783027207108));
#38017=CARTESIAN_POINT('Ctrl Pts',(-14.4384735898227,62.8992423967485,8.17765522357039));
#38018=CARTESIAN_POINT('Ctrl Pts',(-13.9364114971972,62.8719235739435,10.9288348037814));
#38019=CARTESIAN_POINT('Ctrl Pts',(-15.850024041082,62.1973266831092,12.853622756267));
#38020=CARTESIAN_POINT('Ctrl Pts',(-18.4407556977103,61.3412962728355,12.2395195742226));
#38021=CARTESIAN_POINT('Ctrl Pts',(-19.3676134988853,60.9310995184379,9.63289839745391));
#38022=CARTESIAN_POINT('Ctrl Pts',(-17.7699646296638,61.1973422876599,7.35288957156125));
#38023=CARTESIAN_POINT('Ctrl Pts',(-15.0332534115107,61.7687958934069,7.42803777444102));
#38024=CARTESIAN_POINT('Ctrl Pts',(-13.5563500795275,62.0026849934362,9.79147768508997));
#38025=CARTESIAN_POINT('Ctrl Pts',(-14.6172778371391,61.5565643024822,12.3404488591357));
#38026=CARTESIAN_POINT('Ctrl Pts',(-17.236102725553,60.6930063334387,12.807089206987));
#38027=CARTESIAN_POINT('Ctrl Pts',(-19.0468753473843,60.0459653166684,10.7762699688266));
#38028=CARTESIAN_POINT('Ctrl Pts',(-18.4024589901613,60.0567902041013,8.05473611617475));
#38029=CARTESIAN_POINT('Ctrl Pts',(-15.8403574002339,60.5814573009745,7.06404294414452));
#38030=CARTESIAN_POINT('Ctrl Pts',(-13.6037685248159,61.0189035288689,8.68524269063552));
#38031=CARTESIAN_POINT('Ctrl Pts',(-13.6472648693584,60.8454027634006,11.4767030328865));
#38032=CARTESIAN_POINT('Ctrl Pts',(-15.8948076660285,60.0813295310042,12.9532921034687));
#38033=CARTESIAN_POINT('Ctrl Pts',(-18.3134648367078,59.2714063402786,11.8044287744805));
#38034=CARTESIAN_POINT('Ctrl Pts',(-18.7097689547777,59.0033710168103,9.04578082775244));
#38035=CARTESIAN_POINT('Ctrl Pts',(-17.3744086881427,59.2532824184768,7.78080120942677));
#38036=CARTESIAN_POINT('Ctrl Pts',(-16.5917431062329,59.4090483774018,7.56791319796499));
#38037=CARTESIAN_POINT('Ctrl Pts',(-20.4459680138347,67.0649244254632,11.259172404465));
#38038=CARTESIAN_POINT('Ctrl Pts',(-20.8307101569087,66.9078844272409,10.4761135710142));
#38039=CARTESIAN_POINT('Ctrl Pts',(-20.7934159435358,66.8099800782136,8.48633842059633));
#38040=CARTESIAN_POINT('Ctrl Pts',(-18.3334494707627,67.3072801529265,6.83308754393487));
#38041=CARTESIAN_POINT('Ctrl Pts',(-15.6262809016687,67.8708178297157,8.00370485831642));
#38042=CARTESIAN_POINT('Ctrl Pts',(-15.0436190322123,67.8650956520227,10.9474107537965));
#38043=CARTESIAN_POINT('Ctrl Pts',(-17.0682804619448,67.1607433019051,13.049686519018));
#38044=CARTESIAN_POINT('Ctrl Pts',(-19.8627070898848,66.2501329885662,12.4378986762067));
#38045=CARTESIAN_POINT('Ctrl Pts',(-20.9047756131302,65.8090656142303,9.65745411880357));
#38046=CARTESIAN_POINT('Ctrl Pts',(-19.231301559894,66.0956256802751,7.18159743500988));
#38047=CARTESIAN_POINT('Ctrl Pts',(-16.2952133143915,66.7205021994896,7.21338364285574));
#38048=CARTESIAN_POINT('Ctrl Pts',(-14.6727612295383,66.9933909703099,9.72440146443631));
#38049=CARTESIAN_POINT('Ctrl Pts',(-15.7714607991054,66.5371493528457,12.4806427736084));
#38050=CARTESIAN_POINT('Ctrl Pts',(-18.5777884658271,65.6233501657761,13.0298259452254));
#38051=CARTESIAN_POINT('Ctrl Pts',(-20.558934634444,64.9306576947329,10.8833539743374));
#38052=CARTESIAN_POINT('Ctrl Pts',(-19.9162581518544,64.9410163841629,7.95095238475407));
#38053=CARTESIAN_POINT('Ctrl Pts',(-17.1855548447374,65.5108601749995,6.84160605175779));
#38054=CARTESIAN_POINT('Ctrl Pts',(-14.7603541429465,65.9988447894534,8.54230738426514));
#38055=CARTESIAN_POINT('Ctrl Pts',(-14.7623776252392,65.8364566439329,11.5399297656086));
#38056=CARTESIAN_POINT('Ctrl Pts',(-17.1538260329039,65.033824019284,13.167464204339));
#38057=CARTESIAN_POINT('Ctrl Pts',(-19.7710097578038,64.170705798679,11.9768805549434));
#38058=CARTESIAN_POINT('Ctrl Pts',(-20.2494006496399,63.8806753904707,9.02745047458974));
#38059=CARTESIAN_POINT('Ctrl Pts',(-18.1273716126603,64.2874254021705,6.94330548061665));
#38060=CARTESIAN_POINT('Ctrl Pts',(-15.2569098917896,64.8947173471078,7.57872596768869));
#38061=CARTESIAN_POINT('Ctrl Pts',(-14.1558892629051,65.0278889803931,10.3683732743989));
#38062=CARTESIAN_POINT('Ctrl Pts',(-15.7678976499205,64.4341066798258,12.8302759390873));
#38063=CARTESIAN_POINT('Ctrl Pts',(-18.6227194268519,63.5073135350879,12.7740595314741));
#38064=CARTESIAN_POINT('Ctrl Pts',(-20.1443979832212,62.9377350396947,10.2497402360734));
#38065=CARTESIAN_POINT('Ctrl Pts',(-18.9430848635892,63.0977799648826,7.50322506140522));
#38066=CARTESIAN_POINT('Ctrl Pts',(-16.0515990210029,63.7107053062553,6.97811046011705));
#38067=CARTESIAN_POINT('Ctrl Pts',(-14.0065195594074,64.096836741373,9.14159508133219));
#38068=CARTESIAN_POINT('Ctrl Pts',(-14.5913710742637,63.7782802952008,12.0688094033194));
#38069=CARTESIAN_POINT('Ctrl Pts',(-17.2498076016885,62.9041084194735,13.1553875028216));
#38070=CARTESIAN_POINT('Ctrl Pts',(-19.5805980497844,62.1177290461058,11.4345921747925));
#38071=CARTESIAN_POINT('Ctrl Pts',(-19.4740206690256,61.9844404141371,8.43742875512314));
#38072=CARTESIAN_POINT('Ctrl Pts',(-16.9888992784431,62.4884807287627,6.83049741954164));
#38073=CARTESIAN_POINT('Ctrl Pts',(-14.3002673230733,63.0470515348742,8.04349783254823));
#38074=CARTESIAN_POINT('Ctrl Pts',(-13.7642231138315,63.0288381927735,10.9972137711303));
#38075=CARTESIAN_POINT('Ctrl Pts',(-15.8216906940824,62.3156954611179,13.063700777119));
#38076=CARTESIAN_POINT('Ctrl Pts',(-18.6061255468499,61.4077624358672,12.4043885425467));
#38077=CARTESIAN_POINT('Ctrl Pts',(-19.6041954665562,60.9784844518179,9.6058731090043));
#38078=CARTESIAN_POINT('Ctrl Pts',(-17.8919095654206,61.275444121164,7.15801457676324));
#38079=CARTESIAN_POINT('Ctrl Pts',(-14.9567058150546,61.900083640621,7.23869504058987));
#38080=CARTESIAN_POINT('Ctrl Pts',(-13.374054496997,62.1623078281203,9.77612668779238));
#38081=CARTESIAN_POINT('Ctrl Pts',(-14.5160643361693,61.6944612588913,12.5127480402915));
#38082=CARTESIAN_POINT('Ctrl Pts',(-17.3306605884645,60.7784465109948,13.0137415206692));
#38083=CARTESIAN_POINT('Ctrl Pts',(-19.2777173765313,60.0948882619406,10.8334174170448));
#38084=CARTESIAN_POINT('Ctrl Pts',(-18.5888390654042,60.1176266940159,7.91152966540921));
#38085=CARTESIAN_POINT('Ctrl Pts',(-15.8410993561462,60.6920353750482,6.84790363622586));
#38086=CARTESIAN_POINT('Ctrl Pts',(-13.4428359587848,61.172802160534,8.58845287746019));
#38087=CARTESIAN_POINT('Ctrl Pts',(-13.4925131117115,60.9976452524507,11.5854149675154));
#38088=CARTESIAN_POINT('Ctrl Pts',(-15.908494224529,60.188439109268,13.1707075830487));
#38089=CARTESIAN_POINT('Ctrl Pts',(-18.5081868105878,59.3300076251901,11.9372672251408));
#38090=CARTESIAN_POINT('Ctrl Pts',(-18.9366447422826,59.0533567133274,8.97553311378094));
#38091=CARTESIAN_POINT('Ctrl Pts',(-17.5049637099305,59.3290771863822,7.61742821670135));
#38092=CARTESIAN_POINT('Ctrl Pts',(-16.6656727455702,59.5000158708058,7.38886781406146));
#38093=CARTESIAN_POINT('Ctrl Pts',(-20.6320669838895,67.125836237286,11.3455138803092));
#38094=CARTESIAN_POINT('Ctrl Pts',(-21.0441157180881,66.9614794600237,10.5087606876799));
#38095=CARTESIAN_POINT('Ctrl Pts',(-21.0061138698302,66.8637647211924,8.38254661716187));
#38096=CARTESIAN_POINT('Ctrl Pts',(-18.3802418940533,67.405519041455,6.61593229628459));
#38097=CARTESIAN_POINT('Ctrl Pts',(-15.4902171694853,68.0180528774347,7.86681886229054));
#38098=CARTESIAN_POINT('Ctrl Pts',(-14.8703766095605,68.0222926998282,11.0123747272948));
#38099=CARTESIAN_POINT('Ctrl Pts',(-17.036643557291,67.2799972655193,13.2588035819241));
#38100=CARTESIAN_POINT('Ctrl Pts',(-20.0254585175847,66.3173007555082,12.6050654350364));
#38101=CARTESIAN_POINT('Ctrl Pts',(-21.1417561444473,65.8563437528032,9.63396574118191));
#38102=CARTESIAN_POINT('Ctrl Pts',(-19.3563063884493,66.172907617975,6.98833951725265));
#38103=CARTESIAN_POINT('Ctrl Pts',(-16.2216649608855,66.8509863019774,7.02230530597812));
#38104=CARTESIAN_POINT('Ctrl Pts',(-14.4907357506179,67.1529414309497,9.70550366758444));
#38105=CARTESIAN_POINT('Ctrl Pts',(-15.6675476157309,66.675769686975,12.6507404960141));
#38106=CARTESIAN_POINT('Ctrl Pts',(-18.6690796692631,65.7096656421006,13.2375811682069));
#38107=CARTESIAN_POINT('Ctrl Pts',(-20.7888475135915,64.9798296049969,10.9439255732437));
#38108=CARTESIAN_POINT('Ctrl Pts',(-20.1048771373638,65.0012529598797,7.81044915060758));
#38109=CARTESIAN_POINT('Ctrl Pts',(-17.1897038973366,65.6205253202674,6.62503491835178));
#38110=CARTESIAN_POINT('Ctrl Pts',(-14.6009815821227,66.1523254189831,8.44235337373933));
#38111=CARTESIAN_POINT('Ctrl Pts',(-14.6059182596932,65.9891566851404,11.6455227790733));
#38112=CARTESIAN_POINT('Ctrl Pts',(-17.1641227754441,65.141841895997,13.3846572853789));
#38113=CARTESIAN_POINT('Ctrl Pts',(-19.9635412834481,64.2298940124263,12.1124352923854));
#38114=CARTESIAN_POINT('Ctrl Pts',(-20.4775098929406,63.9303305835034,8.96076273504135));
#38115=CARTESIAN_POINT('Ctrl Pts',(-18.2127477293894,64.3753258212012,6.73370787899156));
#38116=CARTESIAN_POINT('Ctrl Pts',(-15.1482328385059,65.0346141563322,7.41269916100865));
#38117=CARTESIAN_POINT('Ctrl Pts',(-13.9744896491103,65.1872717409779,10.3936326368661));
#38118=CARTESIAN_POINT('Ctrl Pts',(-15.6998079270964,64.5631281466306,13.0243480143333));
#38119=CARTESIAN_POINT('Ctrl Pts',(-18.7531593329024,63.5831391481621,12.9642768465755));
#38120=CARTESIAN_POINT('Ctrl Pts',(-20.3819538620282,62.9848590143722,10.266864928835));
#38121=CARTESIAN_POINT('Ctrl Pts',(-19.1010411238774,63.1662325930602,7.33202115613807));
#38122=CARTESIAN_POINT('Ctrl Pts',(-16.0140604868503,63.8315406067278,6.77089943660162));
#38123=CARTESIAN_POINT('Ctrl Pts',(-13.8315243325383,64.2545034516531,9.08273423965009));
#38124=CARTESIAN_POINT('Ctrl Pts',(-14.4592535720065,63.9244579537978,12.2106677036518));
#38125=CARTESIAN_POINT('Ctrl Pts',(-17.3027535879931,63.000698465762,13.3717524842076));
#38126=CARTESIAN_POINT('Ctrl Pts',(-19.7961408267281,62.1707514136505,11.5329621876413));
#38127=CARTESIAN_POINT('Ctrl Pts',(-19.6850298779916,62.0386775475604,8.33028321499222));
#38128=CARTESIAN_POINT('Ctrl Pts',(-17.0322781112102,62.5876342861153,6.61316456701222));
#38129=CARTESIAN_POINT('Ctrl Pts',(-14.1620610563239,63.1948606729998,7.90934044152608));
#38130=CARTESIAN_POINT('Ctrl Pts',(-13.5920347304658,63.1857528116036,11.0655927384792));
#38131=CARTESIAN_POINT('Ctrl Pts',(-15.7933573470829,62.4340642391264,13.273778797971));
#38132=CARTESIAN_POINT('Ctrl Pts',(-18.7714953959894,61.4742285988991,12.5692575108708));
#38133=CARTESIAN_POINT('Ctrl Pts',(-19.8407774342272,61.0258693851979,9.5788478205547));
#38134=CARTESIAN_POINT('Ctrl Pts',(-18.0138545011774,61.3535459546681,6.96313958196524));
#38135=CARTESIAN_POINT('Ctrl Pts',(-14.8801582185986,62.0313713878352,7.04935230673872));
#38136=CARTESIAN_POINT('Ctrl Pts',(-13.1917589144664,62.3219306628044,9.7607756904948));
#38137=CARTESIAN_POINT('Ctrl Pts',(-14.4148508351995,61.8323582153006,12.6850472214474));
#38138=CARTESIAN_POINT('Ctrl Pts',(-17.425218451376,60.8638866885509,13.2203938343514));
#38139=CARTESIAN_POINT('Ctrl Pts',(-19.5085594056783,60.1438112072127,10.8905648652629));
#38140=CARTESIAN_POINT('Ctrl Pts',(-18.7752191406471,60.1784631839305,7.76832321464366));
#38141=CARTESIAN_POINT('Ctrl Pts',(-15.8418413120585,60.8026134491219,6.6317643283072));
#38142=CARTESIAN_POINT('Ctrl Pts',(-13.2819033927538,61.326700792199,8.49166306428486));
#38143=CARTESIAN_POINT('Ctrl Pts',(-13.3377613540646,61.1498877415007,11.6941269021443));
#38144=CARTESIAN_POINT('Ctrl Pts',(-15.9221807830296,60.2955486875318,13.3881230626288));
#38145=CARTESIAN_POINT('Ctrl Pts',(-18.7029087844678,59.3886089101016,12.070105675801));
#38146=CARTESIAN_POINT('Ctrl Pts',(-19.1635205297874,59.1033424098445,8.90528539980945));
#38147=CARTESIAN_POINT('Ctrl Pts',(-17.6355187317182,59.4048719542876,7.45405522397594));
#38148=CARTESIAN_POINT('Ctrl Pts',(-16.7396023849075,59.5909833642099,7.20982243015792));
#38149=CARTESIAN_POINT('Ctrl Pts',(-20.8181659539443,67.1867480491087,11.4318553561534));
#38150=CARTESIAN_POINT('Ctrl Pts',(-21.2575212792675,67.0150744928066,10.5414078043456));
#38151=CARTESIAN_POINT('Ctrl Pts',(-21.2188117961246,66.9175493641713,8.2787548137274));
#38152=CARTESIAN_POINT('Ctrl Pts',(-18.4270343173439,67.5037579299837,6.39877704863432));
#38153=CARTESIAN_POINT('Ctrl Pts',(-15.3541534373018,68.1652879251536,7.72993286626462));
#38154=CARTESIAN_POINT('Ctrl Pts',(-14.6971341869088,68.1794897476338,11.0773387007931));
#38155=CARTESIAN_POINT('Ctrl Pts',(-17.0050066526372,67.3992512291335,13.4679206448302));
#38156=CARTESIAN_POINT('Ctrl Pts',(-20.1882099452846,66.3844685224502,12.7722321938662));
#38157=CARTESIAN_POINT('Ctrl Pts',(-21.3787366757643,65.9036218913761,9.61047736356026));
#38158=CARTESIAN_POINT('Ctrl Pts',(-19.4813112170046,66.2501895556747,6.79508159949542));
#38159=CARTESIAN_POINT('Ctrl Pts',(-16.1481166073795,66.9814704044652,6.8312269691005));
#38160=CARTESIAN_POINT('Ctrl Pts',(-14.3087102716975,67.3124918915896,9.68660587073256));
#38161=CARTESIAN_POINT('Ctrl Pts',(-15.5636344323564,66.8143900211043,12.8208382184197));
#38162=CARTESIAN_POINT('Ctrl Pts',(-18.7603708726991,65.795981118425,13.4453363911884));
#38163=CARTESIAN_POINT('Ctrl Pts',(-21.0187603927389,65.0290015152611,11.00449717215));
#38164=CARTESIAN_POINT('Ctrl Pts',(-20.2934961228732,65.0614895355965,7.6699459164611));
#38165=CARTESIAN_POINT('Ctrl Pts',(-17.1938529499358,65.7301904655353,6.40846378494576));
#38166=CARTESIAN_POINT('Ctrl Pts',(-14.441609021299,66.3058060485126,8.34239936321352));
#38167=CARTESIAN_POINT('Ctrl Pts',(-14.4494588941473,66.141856726348,11.7511157925379));
#38168=CARTESIAN_POINT('Ctrl Pts',(-17.1744195179844,65.2498597727098,13.6018503664189));
#38169=CARTESIAN_POINT('Ctrl Pts',(-20.1560728090925,64.2890822261736,12.2479900298274));
#38170=CARTESIAN_POINT('Ctrl Pts',(-20.7056191362412,63.9799857765361,8.89407499549296));
#38171=CARTESIAN_POINT('Ctrl Pts',(-18.2981238461185,64.4632262402319,6.52411027736645));
#38172=CARTESIAN_POINT('Ctrl Pts',(-15.0395557852223,65.1745109655565,7.24667235432862));
#38173=CARTESIAN_POINT('Ctrl Pts',(-13.7930900353155,65.3466545015629,10.4188919993334));
#38174=CARTESIAN_POINT('Ctrl Pts',(-15.6317182042723,64.6921496134353,13.2184200895793));
#38175=CARTESIAN_POINT('Ctrl Pts',(-18.8835992389528,63.6589647612364,13.1544941616769));
#38176=CARTESIAN_POINT('Ctrl Pts',(-20.6195097408352,63.0319829890498,10.2839896215965));
#38177=CARTESIAN_POINT('Ctrl Pts',(-19.2589973841656,63.2346852212378,7.16081725087092));
#38178=CARTESIAN_POINT('Ctrl Pts',(-15.9765219526977,63.9523759072002,6.56368841308618));
#38179=CARTESIAN_POINT('Ctrl Pts',(-13.6565291056693,64.4121701619331,9.023873397968));
#38180=CARTESIAN_POINT('Ctrl Pts',(-14.3271360697493,64.0706356123949,12.3525260039843));
#38181=CARTESIAN_POINT('Ctrl Pts',(-17.3556995742977,63.0972885120503,13.5881174655937));
#38182=CARTESIAN_POINT('Ctrl Pts',(-20.0116836036718,62.2237737811954,11.6313322004901));
#38183=CARTESIAN_POINT('Ctrl Pts',(-19.8960390869576,62.0929146809836,8.2231376748613));
#38184=CARTESIAN_POINT('Ctrl Pts',(-17.0756569439774,62.686787843468,6.39583171448279));
#38185=CARTESIAN_POINT('Ctrl Pts',(-14.0238547895745,63.3426698111255,7.77518305050392));
#38186=CARTESIAN_POINT('Ctrl Pts',(-13.4198463471001,63.3426674304337,11.1339717058281));
#38187=CARTESIAN_POINT('Ctrl Pts',(-15.7650240000833,62.5524330171351,13.4838568188229));
#38188=CARTESIAN_POINT('Ctrl Pts',(-18.936865245129,61.5406947619309,12.7341264791949));
#38189=CARTESIAN_POINT('Ctrl Pts',(-20.0773594018982,61.0732543185779,9.55182253210509));
#38190=CARTESIAN_POINT('Ctrl Pts',(-18.1357994369342,61.4316477881722,6.76826458716724));
#38191=CARTESIAN_POINT('Ctrl Pts',(-14.8036106221425,62.1626591350494,6.86000957288756));
#38192=CARTESIAN_POINT('Ctrl Pts',(-13.0094633319359,62.4815534974883,9.74542469319723));
#38193=CARTESIAN_POINT('Ctrl Pts',(-14.3136373342297,61.9702551717098,12.8573464026032));
#38194=CARTESIAN_POINT('Ctrl Pts',(-17.5197763142875,60.9493268661069,13.4270461480336));
#38195=CARTESIAN_POINT('Ctrl Pts',(-19.7394014348252,60.1927341524848,10.9477123134811));
#38196=CARTESIAN_POINT('Ctrl Pts',(-18.96159921589,60.2392996738452,7.62511676387811));
#38197=CARTESIAN_POINT('Ctrl Pts',(-15.8425832679708,60.9131915231956,6.41562502038854));
#38198=CARTESIAN_POINT('Ctrl Pts',(-13.1209708267228,61.4805994238641,8.39487325110954));
#38199=CARTESIAN_POINT('Ctrl Pts',(-13.1830095964176,61.3021302305506,11.8028388367732));
#38200=CARTESIAN_POINT('Ctrl Pts',(-15.9358673415301,60.4026582657957,13.6055385422089));
#38201=CARTESIAN_POINT('Ctrl Pts',(-18.8976307583477,59.447210195013,12.2029441264611));
#38202=CARTESIAN_POINT('Ctrl Pts',(-19.3903963172923,59.1533281063616,8.83503768583798));
#38203=CARTESIAN_POINT('Ctrl Pts',(-17.7660737535059,59.4806667221929,7.29068223125052));
#38204=CARTESIAN_POINT('Ctrl Pts',(-16.8135320242448,59.6819508576139,7.03077704625438));
#38205=CARTESIAN_POINT('Ctrl Pts',(-20.25986904378,67.0040126136404,11.1728309286207));
#38206=CARTESIAN_POINT('Ctrl Pts',(-20.4203000043805,66.9555034255254,10.9082027524038));
#38207=CARTESIAN_POINT('Ctrl Pts',(-20.5332184525385,66.9207835851305,10.6149904639444));
#38208=CARTESIAN_POINT('Ctrl Pts',(-20.6611539455099,66.8813975908017,9.99178401342257));
#38209=CARTESIAN_POINT('Ctrl Pts',(-20.6720025707686,66.8780249511107,9.66515229429171));
#38210=CARTESIAN_POINT('Ctrl Pts',(-20.5855924444283,66.904675210205,9.00098486496486));
#38211=CARTESIAN_POINT('Ctrl Pts',(-20.4815398383752,66.9367881932439,8.66883374311755));
#38212=CARTESIAN_POINT('Ctrl Pts',(-20.1690707048658,67.0315956493191,8.06423785428621));
#38213=CARTESIAN_POINT('Ctrl Pts',(-19.9644265611135,67.0931208523799,7.79496359360561));
#38214=CARTESIAN_POINT('Ctrl Pts',(-19.4553169386788,67.2425937581436,7.32570054462936));
#38215=CARTESIAN_POINT('Ctrl Pts',(-19.1487818292132,67.3308539700399,7.13688275745722));
#38216=CARTESIAN_POINT('Ctrl Pts',(-18.8154792730627,67.4238662472344,7.01293629783561));
#38217=CARTESIAN_POINT('Ctrl Pts',(-15.2652009106025,66.709565290414,9.99881345470565));
#38218=CARTESIAN_POINT('Ctrl Pts',(-15.2659775128488,66.7141255555457,9.92620926472458));
#38219=CARTESIAN_POINT('Ctrl Pts',(-15.2699455778512,66.7178306708093,9.85363960672269));
#38220=CARTESIAN_POINT('Ctrl Pts',(-15.2772137473688,66.720651525733,9.78136734601481));
#38221=CARTESIAN_POINT('Ctrl Pts',(-15.3594450282717,66.752566372114,8.96368683410325));
#38222=CARTESIAN_POINT('Ctrl Pts',(-15.8641033480846,66.6712922345579,8.18407440691831));
#38223=CARTESIAN_POINT('Ctrl Pts',(-16.5726883518979,66.5353761067088,7.78933375549813));
#38224=CARTESIAN_POINT('Ctrl Pts',(-17.2812733557112,66.3994599788597,7.39459310407796));
#38225=CARTESIAN_POINT('Ctrl Pts',(-18.193785043525,66.2089018607175,7.38472422842254));
#38226=CARTESIAN_POINT('Ctrl Pts',(-18.9102906125109,66.0708634238267,7.76413764787118));
#38227=CARTESIAN_POINT('Ctrl Pts',(-19.6267961814968,65.932824986936,8.14355106731982));
#38228=CARTESIAN_POINT('Ctrl Pts',(-20.1472956316549,65.8473062312967,8.91224678187253));
#38229=CARTESIAN_POINT('Ctrl Pts',(-20.246238786796,65.8747431444715,9.7282262093075));
#38230=CARTESIAN_POINT('Ctrl Pts',(-20.345181941937,65.9021800576463,10.5442056367425));
#38231=CARTESIAN_POINT('Ctrl Pts',(-20.0225688020609,66.0425726396353,11.4074687770597));
#38232=CARTESIAN_POINT('Ctrl Pts',(-19.4279225161918,66.2558562834075,11.9340732703408));
#38233=CARTESIAN_POINT('Ctrl Pts',(-18.8332762303227,66.4691399271797,12.4606777636219));
#38234=CARTESIAN_POINT('Ctrl Pts',(-17.9665967984606,66.7553146327353,12.6506236098669));
#38235=CARTESIAN_POINT('Ctrl Pts',(-17.2194144305738,67.0094701965008,12.4192427536871));
#38236=CARTESIAN_POINT('Ctrl Pts',(-16.472232062687,67.2636257602663,12.1878618975073));
#38237=CARTESIAN_POINT('Ctrl Pts',(-15.8445467587755,67.4857621822417,11.5351543389028));
#38238=CARTESIAN_POINT('Ctrl Pts',(-15.6216179699845,67.5994444228593,10.7518245719412));
#38239=CARTESIAN_POINT('Ctrl Pts',(-15.5528913979792,67.6344914472383,10.5103323450965));
#38240=CARTESIAN_POINT('Ctrl Pts',(-15.5226338262371,67.6592307340631,10.2564254798707));
#38241=CARTESIAN_POINT('Ctrl Pts',(-15.5286491313886,67.6742507328171,10.0019962882658));
#38242=CARTESIAN_POINT('Ctrl Pts',(-16.8135320242449,59.6819508576139,7.0307770462544));
#38243=CARTESIAN_POINT('Ctrl Pts',(-16.9051481187289,59.6574023990832,7.06547285383772));
#38244=CARTESIAN_POINT('Ctrl Pts',(-16.9947948727615,59.6333816237361,7.105152193198));
#38245=CARTESIAN_POINT('Ctrl Pts',(-17.0822377867392,59.609951365552,7.14949694329713));
#38246=CARTESIAN_POINT('Ctrl Pts',(-17.170887130687,59.5861978454316,7.1944535078144));
#38247=CARTESIAN_POINT('Ctrl Pts',(-17.2572720505333,59.5630510759206,7.24420580543408));
#38248=CARTESIAN_POINT('Ctrl Pts',(-17.3411153578571,59.5405853294324,7.29846300342455));
#38249=CARTESIAN_POINT('Ctrl Pts',(-17.3650399830872,59.5341747454228,7.31394525441622));
#38250=CARTESIAN_POINT('Ctrl Pts',(-17.388757423411,59.5278196764415,7.32979452701951));
#38251=CARTESIAN_POINT('Ctrl Pts',(-17.412260642765,59.5215220077961,7.34600453504371));
#38252=CARTESIAN_POINT('Ctrl Pts',(-17.430731609272,59.5165727272371,7.35874383304306));
#38253=CARTESIAN_POINT('Ctrl Pts',(-17.4490721037271,59.5116584065591,7.37170741301654));
#38254=CARTESIAN_POINT('Ctrl Pts',(-17.4672605739288,59.5067848206569,7.38487881922079));
#38255=CARTESIAN_POINT('Ctrl Pts',(-17.5471418515796,59.48538069682,7.44272583683044));
#38256=CARTESIAN_POINT('Ctrl Pts',(-17.6241706059935,59.4647409042809,7.50463022528993));
#38257=CARTESIAN_POINT('Ctrl Pts',(-17.6980879987993,59.4449347985719,7.57029723831441));
#38258=CARTESIAN_POINT('Ctrl Pts',(-17.7541980616857,59.4299001525343,7.62014450822626));
#38259=CARTESIAN_POINT('Ctrl Pts',(-17.8085146623264,59.415346063257,7.67216077844244));
#38260=CARTESIAN_POINT('Ctrl Pts',(-17.8609084969032,59.4013071775938,7.72622830906753));
#38261=CARTESIAN_POINT('Ctrl Pts',(-17.8879292143121,59.3940669981851,7.75411219040241));
#38262=CARTESIAN_POINT('Ctrl Pts',(-17.9144382907055,59.3869639125734,7.78254178029124));
#38263=CARTESIAN_POINT('Ctrl Pts',(-17.9404163405827,59.3800031150879,7.81150163974704));
#38264=CARTESIAN_POINT('Ctrl Pts',(-17.9513656352239,59.3770692604311,7.82370771508563));
#38265=CARTESIAN_POINT('Ctrl Pts',(-17.9622216783274,59.3741603924485,7.83600935555966));
#38266=CARTESIAN_POINT('Ctrl Pts',(-17.9729722066906,59.3712797970554,7.8483927628579));
#38267=CARTESIAN_POINT('Ctrl Pts',(-18.0365635529481,59.3542405471801,7.92164288738644));
#38268=CARTESIAN_POINT('Ctrl Pts',(-18.0965497610756,59.3381672911553,7.99784282333236));
#38269=CARTESIAN_POINT('Ctrl Pts',(-18.152694204644,59.3231234328417,8.0767163112685));
#38270=CARTESIAN_POINT('Ctrl Pts',(-18.2078226719857,59.3083518045375,8.1541625237066));
#38271=CARTESIAN_POINT('Ctrl Pts',(-18.2592474980566,59.2945725639209,8.23418719309428));
#38272=CARTESIAN_POINT('Ctrl Pts',(-18.3067019322666,59.281857186597,8.3165506095198));
#38273=CARTESIAN_POINT('Ctrl Pts',(-18.3532560644872,59.2693830444642,8.3973514333468));
#38274=CARTESIAN_POINT('Ctrl Pts',(-18.3959893040302,59.2579327074387,8.48040377584086));
#38275=CARTESIAN_POINT('Ctrl Pts',(-18.4346037833018,59.2475859889017,8.56549184014349));
#38276=CARTESIAN_POINT('Ctrl Pts',(-18.4539341350127,59.2424064367714,8.60808680038629));
#38277=CARTESIAN_POINT('Ctrl Pts',(-18.4722315775318,59.2375036518248,8.65119201455741));
#38278=CARTESIAN_POINT('Ctrl Pts',(-18.4894539568131,59.2328889292046,8.69478065009698));
#38279=CARTESIAN_POINT('Ctrl Pts',(-18.4977385367033,59.2306690827134,8.71574834146746));
#38280=CARTESIAN_POINT('Ctrl Pts',(-18.5057743025267,59.2285159057505,8.73682789360235));
#38281=CARTESIAN_POINT('Ctrl Pts',(-18.5135562806577,59.2264307309948,8.7580163058807));
#38282=CARTESIAN_POINT('Ctrl Pts',(-18.5185237400942,59.2250997042503,8.77154147605531));
#38283=CARTESIAN_POINT('Ctrl Pts',(-18.5233877588506,59.2237963943526,8.78511114931605));
#38284=CARTESIAN_POINT('Ctrl Pts',(-18.5281423789944,59.2225223977247,8.79871063667249));
#38285=CARTESIAN_POINT('Ctrl Pts',(-18.5587083682407,59.2143322655903,8.88613755443148));
#38286=CARTESIAN_POINT('Ctrl Pts',(-18.5848098578326,59.2073383925329,8.97493705335627));
#38287=CARTESIAN_POINT('Ctrl Pts',(-18.6062022975293,59.2016063055921,9.06488740567881));
#38288=CARTESIAN_POINT('Ctrl Pts',(-18.6087806599848,59.2009154354543,9.07572883445317));
#38289=CARTESIAN_POINT('Ctrl Pts',(-18.6112905562917,59.2002429107658,9.08658699313155));
#38290=CARTESIAN_POINT('Ctrl Pts',(-18.6137315088206,59.1995888595069,9.09746150181129));
#38291=CARTESIAN_POINT('Ctrl Pts',(-18.634303712552,59.1940765541306,9.18911121862735));
#38292=CARTESIAN_POINT('Ctrl Pts',(-18.6499830153474,59.1898752976086,9.28192246234248));
#38293=CARTESIAN_POINT('Ctrl Pts',(-18.6608728938791,59.1869573634504,9.37550443039365));
#38294=CARTESIAN_POINT('Ctrl Pts',(-18.6721439846079,59.1839372837918,9.47236233835083));
#38295=CARTESIAN_POINT('Ctrl Pts',(-18.678284396889,59.1822919652799,9.57004704529739));
#38296=CARTESIAN_POINT('Ctrl Pts',(-18.6793547107856,59.1820051755357,9.66811274309982));
#38297=CARTESIAN_POINT('Ctrl Pts',(-18.6798764988089,59.1818653628562,9.71592068689136));
#38298=CARTESIAN_POINT('Ctrl Pts',(-18.6791925043481,59.1820486386196,9.76381888089709));
#38299=CARTESIAN_POINT('Ctrl Pts',(-18.6773054175267,59.1825542820094,9.81175333281661));
#38300=CARTESIAN_POINT('Ctrl Pts',(-18.6767477018626,59.1827037214712,9.82592003377692));
#38301=CARTESIAN_POINT('Ctrl Pts',(-18.676084807492,59.1828813434825,9.84008999147557));
#38302=CARTESIAN_POINT('Ctrl Pts',(-18.6753177565558,59.1830868741614,9.85424725714683));
#38303=CARTESIAN_POINT('Ctrl Pts',(-18.6702850236762,59.1844353908722,9.94713513860433));
#38304=CARTESIAN_POINT('Ctrl Pts',(-18.6607672605616,59.1869856678125,10.0396336498301));
#38305=CARTESIAN_POINT('Ctrl Pts',(-18.6468763517958,59.1907077255985,10.1313703614097));
#38306=CARTESIAN_POINT('Ctrl Pts',(-18.6330252856618,59.1944191075834,10.2228439489501));
#38307=CARTESIAN_POINT('Ctrl Pts',(-18.6148257393987,59.1992956613072,10.3135610438633));
#38308=CARTESIAN_POINT('Ctrl Pts',(-18.5923417340723,59.205320232377,10.4031353913064));
#38309=CARTESIAN_POINT('Ctrl Pts',(-18.5702449115824,59.2112410581185,10.4911672355606));
#38310=CARTESIAN_POINT('Ctrl Pts',(-18.5440094800128,59.2182708208206,10.5780961325691));
#38311=CARTESIAN_POINT('Ctrl Pts',(-18.513657092413,59.2264037185664,10.6635263259507));
#38312=CARTESIAN_POINT('Ctrl Pts',(-18.4991012558957,59.2303039432063,10.7044953576096));
#38313=CARTESIAN_POINT('Ctrl Pts',(-18.4835980627564,59.2344580112881,10.745119212542));
#38314=CARTESIAN_POINT('Ctrl Pts',(-18.4671470631154,59.2388660433566,10.7853510165448));
#38315=CARTESIAN_POINT('Ctrl Pts',(-18.4616118759027,59.2403491923002,10.7988876144369));
#38316=CARTESIAN_POINT('Ctrl Pts',(-18.4559693741439,59.2418610960897,10.8123798089597));
#38317=CARTESIAN_POINT('Ctrl Pts',(-18.4502194972567,59.2434017709582,10.8258257523306));
#38318=CARTESIAN_POINT('Ctrl Pts',(-18.4447502513313,59.2448672509872,10.8386154472123));
#38319=CARTESIAN_POINT('Ctrl Pts',(-18.4391855696915,59.2463583029387,10.8513591677317));
#38320=CARTESIAN_POINT('Ctrl Pts',(-18.4335294175102,59.2478738643479,10.8640470913851));
#38321=CARTESIAN_POINT('Ctrl Pts',(-18.3974943892406,59.257529421072,10.9448811412621));
#38322=CARTESIAN_POINT('Ctrl Pts',(-18.3577058350372,59.2681907320388,11.0235565035205));
#38323=CARTESIAN_POINT('Ctrl Pts',(-18.3142251103301,59.2798413571104,11.0997253732309));
#38324=CARTESIAN_POINT('Ctrl Pts',(-18.2714642927579,59.2912990836466,11.1746331206135));
#38325=CARTESIAN_POINT('Ctrl Pts',(-18.2251321272591,59.3037137499756,11.2471173606586));
#38326=CARTESIAN_POINT('Ctrl Pts',(-18.1752516289978,59.3170791892027,11.3168132015496));
#38327=CARTESIAN_POINT('Ctrl Pts',(-18.126814322891,59.3300579262576,11.3844925330976));
#38328=CARTESIAN_POINT('Ctrl Pts',(-18.0750306258258,59.3439333260673,11.449542941438));
#38329=CARTESIAN_POINT('Ctrl Pts',(-18.0198942246886,59.3587070802256,11.5115898438694));
#38330=CARTESIAN_POINT('Ctrl Pts',(-18.0099245352413,59.3613784504618,11.5228090808101));
#38331=CARTESIAN_POINT('Ctrl Pts',(-17.9998451629737,59.3640792101211,11.5339299972364));
#38332=CARTESIAN_POINT('Ctrl Pts',(-17.9896559870011,59.3668093915945,11.5449502145347));
#38333=CARTESIAN_POINT('Ctrl Pts',(-17.9601614990778,59.3747124158147,11.5768503080151));
#38334=CARTESIAN_POINT('Ctrl Pts',(-17.9297469672235,59.3828619650632,11.6079068412473));
#38335=CARTESIAN_POINT('Ctrl Pts',(-17.8984546702662,59.3912467107622,11.6380966037225));
#38336=CARTESIAN_POINT('Ctrl Pts',(-15.0750265266586,68.1281291851066,10.0024371765581));
#38337=CARTESIAN_POINT('Ctrl Pts',(-15.0686010168709,68.1132191003536,10.3130580784043));
#38338=CARTESIAN_POINT('Ctrl Pts',(-15.229260839257,67.9995899840861,11.6285356953996));
#38339=CARTESIAN_POINT('Ctrl Pts',(-17.0050066526372,67.3992512291335,13.4679206448302));
#38340=CARTESIAN_POINT('Ctrl Pts',(-20.1882099452846,66.3844685224502,12.7722321938662));
#38341=CARTESIAN_POINT('Ctrl Pts',(-21.3787366757643,65.9036218913761,9.61047736356026));
#38342=CARTESIAN_POINT('Ctrl Pts',(-19.4813112170046,66.2501895556747,6.79508159949542));
#38343=CARTESIAN_POINT('Ctrl Pts',(-16.1481166073795,66.9814704044652,6.8312269691005));
#38344=CARTESIAN_POINT('Ctrl Pts',(-14.8676525643411,67.2119040522751,8.81893895087672));
#38345=CARTESIAN_POINT('Ctrl Pts',(-14.8112407741816,67.168302539124,9.90991228406402));
#38346=CARTESIAN_POINT('Ctrl Pts',(-14.810555933805,67.1637176864734,9.9985514014054));
#38347=CARTESIAN_POINT('Origin',(-18.6889152049569,69.7479810832458,10.));
#38348=CARTESIAN_POINT('Ctrl Pts',(-15.0969161422106,68.2083503098983,9.99673640007589));
#38349=CARTESIAN_POINT('Ctrl Pts',(-15.0927295232038,68.1711103559359,10.7130675866998));
#38350=CARTESIAN_POINT('Ctrl Pts',(-15.6514186592592,67.9289066052255,12.4513417391712));
#38351=CARTESIAN_POINT('Ctrl Pts',(-18.3902480628706,67.0483943376967,13.59444534976));
#38352=CARTESIAN_POINT('Ctrl Pts',(-21.0667649555468,66.1687987195558,11.6442225433404));
#38353=CARTESIAN_POINT('Ctrl Pts',(-20.9561469803463,66.0360136384589,8.2201649478064));
#38354=CARTESIAN_POINT('Ctrl Pts',(-18.1194957904389,66.6336669557831,6.39071567224372));
#38355=CARTESIAN_POINT('Ctrl Pts',(-15.4027596845035,67.2173089746448,7.63681194520529));
#38356=CARTESIAN_POINT('Ctrl Pts',(-14.8518622987657,67.2747579502335,9.32892113065739));
#38357=CARTESIAN_POINT('Ctrl Pts',(-14.8383776097513,67.242349320473,10.0022118830713));
#38358=CARTESIAN_POINT('Ctrl Pts',(-17.2449834421536,67.8425423025984,7.06170475438588));
#38359=CARTESIAN_POINT('Ctrl Pts',(-16.2988495743029,68.0419164156806,7.35795147289551));
#38360=CARTESIAN_POINT('Ctrl Pts',(-14.7258515725222,68.3551165744734,8.97144797270149));
#38361=CARTESIAN_POINT('Ctrl Pts',(-15.356703424302,68.0236552520252,12.3283366156207));
#38362=CARTESIAN_POINT('Ctrl Pts',(-18.3902480628706,67.0483943376967,13.59444534976));
#38363=CARTESIAN_POINT('Ctrl Pts',(-21.0667649555468,66.1687987195558,11.6442225433404));
#38364=CARTESIAN_POINT('Ctrl Pts',(-20.9561469803463,66.0360136384589,8.2201649478064));
#38365=CARTESIAN_POINT('Ctrl Pts',(-18.1194957904389,66.6336669557831,6.39071567224372));
#38366=CARTESIAN_POINT('Ctrl Pts',(-15.0616295968137,67.2905946547072,7.79327945411664));
#38367=CARTESIAN_POINT('Ctrl Pts',(-14.4843023646229,67.2828639421211,11.1722569386409));
#38368=CARTESIAN_POINT('Ctrl Pts',(-16.8683721674333,66.4816292855384,13.5013274912987));
#38369=CARTESIAN_POINT('Ctrl Pts',(-20.0422978199454,65.4687533918912,12.6947822329677));
#38370=CARTESIAN_POINT('Ctrl Pts',(-21.1273143736847,65.0155990043222,9.47487431060756));
#38371=CARTESIAN_POINT('Ctrl Pts',(-19.1153342996386,65.3922823621301,6.72525821930975));
#38372=CARTESIAN_POINT('Ctrl Pts',(-15.7718556315871,66.125739692925,6.90837057311325));
#38373=CARTESIAN_POINT('Ctrl Pts',(-14.0547985877671,66.4233986629546,9.86022990097426));
#38374=CARTESIAN_POINT('Ctrl Pts',(-15.4655309000311,65.8829690009267,12.9372608391338));
#38375=CARTESIAN_POINT('Ctrl Pts',(-18.7042880702644,64.8527215544621,13.3837942299381));
#38376=CARTESIAN_POINT('Ctrl Pts',(-20.8341986998844,64.1195886430847,10.7999310727637));
#38377=CARTESIAN_POINT('Ctrl Pts',(-19.9114308093218,64.2044184759421,7.49968047567802));
#38378=CARTESIAN_POINT('Ctrl Pts',(-16.7260146593058,64.8955230826759,6.4386200392349));
#38379=CARTESIAN_POINT('Ctrl Pts',(-14.0943212306271,65.4382581333963,8.56699487612795));
#38380=CARTESIAN_POINT('Ctrl Pts',(-14.3368288007652,65.2108533475993,11.9787141005057));
#38381=CARTESIAN_POINT('Ctrl Pts',(-17.1999914587374,64.2812461473765,13.6183729089162));
#38382=CARTESIAN_POINT('Ctrl Pts',(-20.0833051820053,63.3462394854811,12.0175557753475));
#38383=CARTESIAN_POINT('Ctrl Pts',(-20.368219412885,63.1074718691845,8.60989310618186));
#38384=CARTESIAN_POINT('Ctrl Pts',(-17.7632104839254,63.6430568297549,6.44715683087691));
#38385=CARTESIAN_POINT('Ctrl Pts',(-14.5648590180574,64.337627443925,7.46621057361457));
#38386=CARTESIAN_POINT('Ctrl Pts',(-13.6011204490198,64.4334353369931,10.7544289031923));
#38387=CARTESIAN_POINT('Ctrl Pts',(-15.6987166428553,63.7089610525881,13.3670096553834));
#38388=CARTESIAN_POINT('Ctrl Pts',(-18.9427555175128,62.6772983776883,12.9642257537712));
#38389=CARTESIAN_POINT('Ctrl Pts',(-20.3916349158421,62.1266472347557,9.90679500749766));
#38390=CARTESIAN_POINT('Ctrl Pts',(-18.7114286257309,62.4144320750885,6.93283507366423));
#38391=CARTESIAN_POINT('Ctrl Pts',(-15.3704995140603,63.14720625431,6.70571036393722));
#38392=CARTESIAN_POINT('Ctrl Pts',(-13.3244900809145,63.5330077514078,9.42882503807092));
#38393=CARTESIAN_POINT('Ctrl Pts',(-14.3693624549392,63.090609964374,12.6634621126404));
#38394=CARTESIAN_POINT('Ctrl Pts',(-17.5330036055452,62.0804897947072,13.5128046754736));
#38395=CARTESIAN_POINT('Ctrl Pts',(-19.945812508159,61.2715545195409,11.2162142452881));
#38396=CARTESIAN_POINT('Ctrl Pts',(-19.4106046411916,61.2525379570574,7.83042882970079));
#38397=CARTESIAN_POINT('Ctrl Pts',(-16.3703262829259,61.9047530097004,6.38762845988016));
#38398=CARTESIAN_POINT('Ctrl Pts',(-13.5113685232519,62.5083833543795,8.17992871548433));
#38399=CARTESIAN_POINT('Ctrl Pts',(-13.3577390856958,62.3871231598862,11.6022164308582));
#38400=CARTESIAN_POINT('Ctrl Pts',(-16.0106566332711,61.5138509672068,13.5896176377582));
#38401=CARTESIAN_POINT('Ctrl Pts',(-19.0579057022672,60.5349179618126,12.3623010109727));
#38402=CARTESIAN_POINT('Ctrl Pts',(-19.7341192728292,60.1913020034494,9.0193860958895));
#38403=CARTESIAN_POINT('Ctrl Pts',(-17.3973455890627,60.6550135466887,6.55469600728496));
#38404=CARTESIAN_POINT('Ctrl Pts',(-14.1039347737165,61.3750552367845,7.17543798647131));
#38405=CARTESIAN_POINT('Ctrl Pts',(-12.7669926495711,61.5708627210561,10.3258507409619));
#38406=CARTESIAN_POINT('Ctrl Pts',(-14.5474295567697,60.9313710113776,13.1842383274674));
#38407=CARTESIAN_POINT('Ctrl Pts',(-17.8144668208749,59.893545936598,13.1913616605741));
#38408=CARTESIAN_POINT('Ctrl Pts',(-19.6057481548832,59.2511484715134,10.339577077016));
#38409=CARTESIAN_POINT('Ctrl Pts',(-18.2810249486942,59.4436819065862,7.1853989865657));
#38410=CARTESIAN_POINT('Ctrl Pts',(-14.9896601306958,60.163175373345,6.54837069990765));
#38411=CARTESIAN_POINT('Ctrl Pts',(-12.6441934312552,60.6292162031139,9.00969837718612));
#38412=CARTESIAN_POINT('Ctrl Pts',(-13.0868379849883,60.402326566927,11.2296927240261));
#38413=CARTESIAN_POINT('Ctrl Pts',(-13.7072348830368,60.1819500263681,11.9973015569302));
#38414=CARTESIAN_POINT('Ctrl Pts',(-17.3251900988202,67.9318278742782,7.23888518457529));
#38415=CARTESIAN_POINT('Ctrl Pts',(-16.4352923065874,68.1161335763131,7.5172681022616));
#38416=CARTESIAN_POINT('Ctrl Pts',(-14.9555143577764,68.4043554971942,9.03347008941727));
#38417=CARTESIAN_POINT('Ctrl Pts',(-15.5458770044739,68.0837432245501,12.1879369455068));
#38418=CARTESIAN_POINT('Ctrl Pts',(-18.3940490596775,67.158152744233,13.3776987943165));
#38419=CARTESIAN_POINT('Ctrl Pts',(-20.9067222911422,66.3224589027987,11.5450752374354));
#38420=CARTESIAN_POINT('Ctrl Pts',(-20.8003260510253,66.1885426111955,8.32748974461997));
#38421=CARTESIAN_POINT('Ctrl Pts',(-18.1322775372978,66.7410189775957,6.60835702425636));
#38422=CARTESIAN_POINT('Ctrl Pts',(-15.2563533769444,67.3491954556353,7.92634562444483));
#38423=CARTESIAN_POINT('Ctrl Pts',(-14.7113906429073,67.3327927019054,11.1015693557675));
#38424=CARTESIAN_POINT('Ctrl Pts',(-16.9492514661357,66.5707346233279,13.2901959816016));
#38425=CARTESIAN_POINT('Ctrl Pts',(-19.9293395015263,65.6097973626512,12.5322857391193));
#38426=CARTESIAN_POINT('Ctrl Pts',(-20.9464805290196,65.1748301675256,9.50653960894302));
#38427=CARTESIAN_POINT('Ctrl Pts',(-19.0533751185271,65.5196611552339,6.92272651604678));
#38428=CARTESIAN_POINT('Ctrl Pts',(-15.9090610352123,66.1997524963876,7.09479711845775));
#38429=CARTESIAN_POINT('Ctrl Pts',(-14.2930946730788,66.4703242998971,9.86865809630622));
#38430=CARTESIAN_POINT('Ctrl Pts',(-15.6163106628559,65.9533445658041,12.7601427840871));
#38431=CARTESIAN_POINT('Ctrl Pts',(-18.6573208483787,64.9760832641984,13.1797500249769));
#38432=CARTESIAN_POINT('Ctrl Pts',(-20.6563484026838,64.2780203671544,10.7516948950666));
#38433=CARTESIAN_POINT('Ctrl Pts',(-19.7867752262126,64.3485967193295,7.65045078699769));
#38434=CARTESIAN_POINT('Ctrl Pts',(-16.7909924250971,64.9888892233673,6.65337273791561));
#38435=CARTESIAN_POINT('Ctrl Pts',(-14.3155426340163,65.4897589175709,8.65340568344564));
#38436=CARTESIAN_POINT('Ctrl Pts',(-14.5409783214074,65.2669285289692,11.8593968140374));
#38437=CARTESIAN_POINT('Ctrl Pts',(-17.2290425005872,64.3842388247347,13.4001835116647));
#38438=CARTESIAN_POINT('Ctrl Pts',(-19.9360426274114,63.4964752486211,11.895896319668));
#38439=CARTESIAN_POINT('Ctrl Pts',(-20.2013278361945,63.2629672129435,8.69371713231524));
#38440=CARTESIAN_POINT('Ctrl Pts',(-17.7509534583579,63.7571179704186,6.66139475745709));
#38441=CARTESIAN_POINT('Ctrl Pts',(-14.7430153463372,64.4006674801971,7.61899913400395));
#38442=CARTESIAN_POINT('Ctrl Pts',(-13.8349420404104,64.4815599109683,10.7089365253196));
#38443=CARTESIAN_POINT('Ctrl Pts',(-15.8036037329016,63.791633522075,13.1639775672761));
#38444=CARTESIAN_POINT('Ctrl Pts',(-18.8495771338665,62.8130423308996,12.7854817031127));
#38445=CARTESIAN_POINT('Ctrl Pts',(-20.2086399244908,62.2864574754684,9.9124153074631));
#38446=CARTESIAN_POINT('Ctrl Pts',(-18.6273022002306,62.5477505634246,7.11778639941041));
#38447=CARTESIAN_POINT('Ctrl Pts',(-15.4853839339823,63.2271999473302,6.90435740451538));
#38448=CARTESIAN_POINT('Ctrl Pts',(-13.5603011489528,63.5805992467218,9.46326712676812));
#38449=CARTESIAN_POINT('Ctrl Pts',(-14.5397187075304,63.1557400246278,12.5028542351253));
#38450=CARTESIAN_POINT('Ctrl Pts',(-17.510142400774,62.1973923166248,13.3009810867785));
#38451=CARTESIAN_POINT('Ctrl Pts',(-19.7750093440878,61.4280979699797,11.1428760184696));
#38452=CARTESIAN_POINT('Ctrl Pts',(-19.2696261599642,61.4010899078137,7.96125487716962));
#38453=CARTESIAN_POINT('Ctrl Pts',(-16.4102292811544,62.0048379141107,6.60545597208737));
#38454=CARTESIAN_POINT('Ctrl Pts',(-13.7212192931312,62.5629308906205,8.28967977390748));
#38455=CARTESIAN_POINT('Ctrl Pts',(-13.5744051997982,62.4398445301464,11.5056021110754));
#38456=CARTESIAN_POINT('Ctrl Pts',(-16.0649021365254,61.610092808978,13.3731621953642));
#38457=CARTESIAN_POINT('Ctrl Pts',(-18.9259522392795,60.6810516662199,12.2198532736373));
#38458=CARTESIAN_POINT('Ctrl Pts',(-19.5589412741758,60.3490176872815,9.0785175237606));
#38459=CARTESIAN_POINT('Ctrl Pts',(-17.3606274442461,60.7756290245011,6.76244927662497));
#38460=CARTESIAN_POINT('Ctrl Pts',(-14.2633621012127,61.4431136936916,7.34576025527691));
#38461=CARTESIAN_POINT('Ctrl Pts',(-13.0045895703813,61.6179756985622,10.3062018052236));
#38462=CARTESIAN_POINT('Ctrl Pts',(-14.675216813649,61.007907399655,12.9922274267493));
#38463=CARTESIAN_POINT('Ctrl Pts',(-17.7428017915751,60.0235254038857,12.9989212198953));
#38464=CARTESIAN_POINT('Ctrl Pts',(-19.4236195381877,59.4107265678367,10.3191004374823));
#38465=CARTESIAN_POINT('Ctrl Pts',(-18.176329119458,59.5825119500423,7.3551206029064));
#38466=CARTESIAN_POINT('Ctrl Pts',(-15.080986399278,60.2494814539918,6.75650538792364));
#38467=CARTESIAN_POINT('Ctrl Pts',(-12.874503746149,60.6782816207908,9.06941397854012));
#38468=CARTESIAN_POINT('Ctrl Pts',(-13.2888242651273,60.4589813868428,11.1555417393118));
#38469=CARTESIAN_POINT('Ctrl Pts',(-13.8709947795083,60.2488475749172,11.8768634390783));
#38470=CARTESIAN_POINT('Ctrl Pts',(-17.4053967554868,68.021113445958,7.4160656147647));
#38471=CARTESIAN_POINT('Ctrl Pts',(-16.5717350388718,68.1903507369456,7.6765847316277));
#38472=CARTESIAN_POINT('Ctrl Pts',(-15.1851771430307,68.4535944199151,9.09549220613307));
#38473=CARTESIAN_POINT('Ctrl Pts',(-15.7350505846458,68.1438311970748,12.0475372753929));
#38474=CARTESIAN_POINT('Ctrl Pts',(-18.3978500564844,67.2679111507695,13.1609522388731));
#38475=CARTESIAN_POINT('Ctrl Pts',(-20.7466796267376,66.4761190860416,11.4459279315303));
#38476=CARTESIAN_POINT('Ctrl Pts',(-20.6445051217044,66.3410715839321,8.43481454143356));
#38477=CARTESIAN_POINT('Ctrl Pts',(-18.1450592841567,66.8483709994082,6.82599837626898));
#38478=CARTESIAN_POINT('Ctrl Pts',(-15.4510771570751,67.4077962565634,8.05941179477303));
#38479=CARTESIAN_POINT('Ctrl Pts',(-14.9384789211916,67.3827214616898,11.0308817728941));
#38480=CARTESIAN_POINT('Ctrl Pts',(-17.0301307648381,66.6598399611174,13.0790644719045));
#38481=CARTESIAN_POINT('Ctrl Pts',(-19.8163811831071,65.7508413334112,12.3697892452708));
#38482=CARTESIAN_POINT('Ctrl Pts',(-20.7656466843543,65.3340613307291,9.53820490727848));
#38483=CARTESIAN_POINT('Ctrl Pts',(-18.9914159374157,65.6470399483376,7.12019481278381));
#38484=CARTESIAN_POINT('Ctrl Pts',(-16.0462664388374,66.2737652998504,7.28122366380225));
#38485=CARTESIAN_POINT('Ctrl Pts',(-14.5313907583906,66.5172499368395,9.87708629163818));
#38486=CARTESIAN_POINT('Ctrl Pts',(-15.7670904256806,66.0237201306815,12.5830247290403));
#38487=CARTESIAN_POINT('Ctrl Pts',(-18.610353626493,65.0994449739345,12.9757058200156));
#38488=CARTESIAN_POINT('Ctrl Pts',(-20.4784981054832,64.4364520912243,10.7034587173694));
#38489=CARTESIAN_POINT('Ctrl Pts',(-19.6621196431034,64.4927749627168,7.80122109831736));
#38490=CARTESIAN_POINT('Ctrl Pts',(-16.8559701908884,65.0822553640587,6.86812543659629));
#38491=CARTESIAN_POINT('Ctrl Pts',(-14.5367640374057,65.5412597017455,8.73981649076335));
#38492=CARTESIAN_POINT('Ctrl Pts',(-14.7451278420497,65.3230037103391,11.7400795275691));
#38493=CARTESIAN_POINT('Ctrl Pts',(-17.2580935424371,64.487231502093,13.1819941144132));
#38494=CARTESIAN_POINT('Ctrl Pts',(-19.7887800728175,63.6467110117611,11.7742368639884));
#38495=CARTESIAN_POINT('Ctrl Pts',(-20.034436259504,63.4184625567025,8.77754115844864));
#38496=CARTESIAN_POINT('Ctrl Pts',(-17.7386964327903,63.8711791110823,6.87563268403724));
#38497=CARTESIAN_POINT('Ctrl Pts',(-14.921171674617,64.4637075164693,7.77178769439333));
#38498=CARTESIAN_POINT('Ctrl Pts',(-14.0687636318009,64.5296844849434,10.663444147447));
#38499=CARTESIAN_POINT('Ctrl Pts',(-15.9084908229478,63.8743059915619,12.9609454791688));
#38500=CARTESIAN_POINT('Ctrl Pts',(-18.7563987502202,62.9487862841109,12.6067376524542));
#38501=CARTESIAN_POINT('Ctrl Pts',(-20.0256449331395,62.4462677161811,9.91803560742851));
#38502=CARTESIAN_POINT('Ctrl Pts',(-18.5431757747304,62.6810690517608,7.3027377251566));
#38503=CARTESIAN_POINT('Ctrl Pts',(-15.6002683539043,63.3071936403504,7.10300444509352));
#38504=CARTESIAN_POINT('Ctrl Pts',(-13.7961122169912,63.6281907420357,9.49770921546533));
#38505=CARTESIAN_POINT('Ctrl Pts',(-14.7100749601216,63.2208700848817,12.3422463576102));
#38506=CARTESIAN_POINT('Ctrl Pts',(-17.4872811960028,62.3142948385424,13.0891574980834));
#38507=CARTESIAN_POINT('Ctrl Pts',(-19.6042061800167,61.5846414204185,11.0695377916511));
#38508=CARTESIAN_POINT('Ctrl Pts',(-19.1286476787368,61.54964185857,8.09208092463846));
#38509=CARTESIAN_POINT('Ctrl Pts',(-16.4501322793829,62.104922818521,6.82328348429458));
#38510=CARTESIAN_POINT('Ctrl Pts',(-13.9310700630105,62.6174784268615,8.39943083233065));
#38511=CARTESIAN_POINT('Ctrl Pts',(-13.7910713139005,62.4925659004067,11.4089877912926));
#38512=CARTESIAN_POINT('Ctrl Pts',(-16.1191476397797,61.7063346507492,13.1567067529703));
#38513=CARTESIAN_POINT('Ctrl Pts',(-18.7939987762918,60.8271853706271,12.0774055363019));
#38514=CARTESIAN_POINT('Ctrl Pts',(-19.3837632755225,60.5067333711136,9.13764895163169));
#38515=CARTESIAN_POINT('Ctrl Pts',(-17.3239092994295,60.8962445023135,6.97020254596497));
#38516=CARTESIAN_POINT('Ctrl Pts',(-14.4227894287088,61.5111721505988,7.5160825240825));
#38517=CARTESIAN_POINT('Ctrl Pts',(-13.2421864911915,61.6650886760681,10.2865528694853));
#38518=CARTESIAN_POINT('Ctrl Pts',(-14.8030040705283,61.0844437879325,12.8002165260311));
#38519=CARTESIAN_POINT('Ctrl Pts',(-17.6711367622752,60.1535048711733,12.8064807792164));
#38520=CARTESIAN_POINT('Ctrl Pts',(-19.2414909214921,59.5703046641601,10.2986237979485));
#38521=CARTESIAN_POINT('Ctrl Pts',(-18.0716332902218,59.7213419934982,7.5248422192471));
#38522=CARTESIAN_POINT('Ctrl Pts',(-15.1723126678601,60.3357875346387,6.96464007593962));
#38523=CARTESIAN_POINT('Ctrl Pts',(-13.1048140610428,60.7273470384677,9.12912957989411));
#38524=CARTESIAN_POINT('Ctrl Pts',(-13.4908105452662,60.5156362067586,11.0813907545975));
#38525=CARTESIAN_POINT('Ctrl Pts',(-14.0347546759797,60.3157451234663,11.7564253212264));
#38526=CARTESIAN_POINT('Ctrl Pts',(-17.4856034121534,68.1103990176377,7.59324604495411));
#38527=CARTESIAN_POINT('Ctrl Pts',(-16.7081777711562,68.2645678975781,7.83590136099379));
#38528=CARTESIAN_POINT('Ctrl Pts',(-15.414839928285,68.5028333426359,9.15751432284886));
#38529=CARTESIAN_POINT('Ctrl Pts',(-15.9242241648176,68.2039191695997,11.907137605279));
#38530=CARTESIAN_POINT('Ctrl Pts',(-18.4016510532913,67.3776695573058,12.9442056834296));
#38531=CARTESIAN_POINT('Ctrl Pts',(-20.586636962333,66.6297792692846,11.3467806256253));
#38532=CARTESIAN_POINT('Ctrl Pts',(-20.4886841923835,66.4936005566688,8.54213933824715));
#38533=CARTESIAN_POINT('Ctrl Pts',(-18.1578410310155,66.9557230212207,7.04363972828162));
#38534=CARTESIAN_POINT('Ctrl Pts',(-15.6458009372058,67.4663970574914,8.19247796510122));
#38535=CARTESIAN_POINT('Ctrl Pts',(-15.1655671994759,67.4326502214742,10.9601941900207));
#38536=CARTESIAN_POINT('Ctrl Pts',(-17.1110100635405,66.7489452989069,12.8679329622074));
#38537=CARTESIAN_POINT('Ctrl Pts',(-19.703422864688,65.8918853041712,12.2072927514223));
#38538=CARTESIAN_POINT('Ctrl Pts',(-20.5848128396891,65.4932924939326,9.56987020561395));
#38539=CARTESIAN_POINT('Ctrl Pts',(-18.9294567563042,65.7744187414414,7.31766310952083));
#38540=CARTESIAN_POINT('Ctrl Pts',(-16.1834718424625,66.3477781033129,7.46765020914676));
#38541=CARTESIAN_POINT('Ctrl Pts',(-14.7696868437023,66.564175573782,9.88551448697013));
#38542=CARTESIAN_POINT('Ctrl Pts',(-15.9178701885053,66.0940956955587,12.4059066739936));
#38543=CARTESIAN_POINT('Ctrl Pts',(-18.5633864046074,65.2228066836708,12.7716616150543));
#38544=CARTESIAN_POINT('Ctrl Pts',(-20.3006478082826,64.5948838152939,10.6552225396723));
#38545=CARTESIAN_POINT('Ctrl Pts',(-19.5374640599943,64.6369532061042,7.95199140963702));
#38546=CARTESIAN_POINT('Ctrl Pts',(-16.9209479566796,65.1756215047502,7.082878135277));
#38547=CARTESIAN_POINT('Ctrl Pts',(-14.757985440795,65.5927604859201,8.82622729808104));
#38548=CARTESIAN_POINT('Ctrl Pts',(-14.9492773626919,65.3790788917091,11.6207622411008));
#38549=CARTESIAN_POINT('Ctrl Pts',(-17.2871445842869,64.5902241794512,12.9638047171617));
#38550=CARTESIAN_POINT('Ctrl Pts',(-19.6415175182236,63.796946774901,11.6525774083089));
#38551=CARTESIAN_POINT('Ctrl Pts',(-19.8675446828135,63.5739579004615,8.86136518458202));
#38552=CARTESIAN_POINT('Ctrl Pts',(-17.7264394072227,63.9852402517459,7.08987061061742));
#38553=CARTESIAN_POINT('Ctrl Pts',(-15.0993280028969,64.5267475527414,7.92457625478271));
#38554=CARTESIAN_POINT('Ctrl Pts',(-14.3025852231914,64.5778090589186,10.6179517695743));
#38555=CARTESIAN_POINT('Ctrl Pts',(-16.013377912994,63.9569784610488,12.7579133910615));
#38556=CARTESIAN_POINT('Ctrl Pts',(-18.6632203665739,63.0845302373222,12.4279936017957));
#38557=CARTESIAN_POINT('Ctrl Pts',(-19.8426499417882,62.6060779568938,9.92365590739396));
#38558=CARTESIAN_POINT('Ctrl Pts',(-18.4590493492301,62.8143875400969,7.48768905090278));
#38559=CARTESIAN_POINT('Ctrl Pts',(-15.7151527738263,63.3871873333706,7.30165148567168));
#38560=CARTESIAN_POINT('Ctrl Pts',(-14.0319232850295,63.6757822373498,9.53215130416253));
#38561=CARTESIAN_POINT('Ctrl Pts',(-14.8804312127128,63.2860001451355,12.1816384800951));
#38562=CARTESIAN_POINT('Ctrl Pts',(-17.4644199912317,62.4311973604601,12.8773339093883));
#38563=CARTESIAN_POINT('Ctrl Pts',(-19.4334030159455,61.7411848708572,10.9961995648325));
#38564=CARTESIAN_POINT('Ctrl Pts',(-18.9876691975094,61.6981938093263,8.22290697210729));
#38565=CARTESIAN_POINT('Ctrl Pts',(-16.4900352776115,62.2050077229312,7.04111099650179));
#38566=CARTESIAN_POINT('Ctrl Pts',(-14.1409208328898,62.6720259631026,8.50918189075381));
#38567=CARTESIAN_POINT('Ctrl Pts',(-14.0077374280029,62.545287270667,11.3123734715098));
#38568=CARTESIAN_POINT('Ctrl Pts',(-16.173393143034,61.8025764925204,12.9402513105763));
#38569=CARTESIAN_POINT('Ctrl Pts',(-18.6620453133041,60.9733190750344,11.9349577989665));
#38570=CARTESIAN_POINT('Ctrl Pts',(-19.2085852768691,60.6644490549456,9.19678037950279));
#38571=CARTESIAN_POINT('Ctrl Pts',(-17.2871911546129,61.0168599801259,7.17795581530498));
#38572=CARTESIAN_POINT('Ctrl Pts',(-14.582216756205,61.5792306075059,7.68640479288809));
#38573=CARTESIAN_POINT('Ctrl Pts',(-13.4797834120017,61.7122016535742,10.2669039337471));
#38574=CARTESIAN_POINT('Ctrl Pts',(-14.9307913274076,61.1609801762098,12.6082056253129));
#38575=CARTESIAN_POINT('Ctrl Pts',(-17.5994717329753,60.2834843384611,12.6140403385376));
#38576=CARTESIAN_POINT('Ctrl Pts',(-19.0593623047967,59.7298827604834,10.2781471584148));
#38577=CARTESIAN_POINT('Ctrl Pts',(-17.9669374609856,59.8601720369542,7.6945638355878));
#38578=CARTESIAN_POINT('Ctrl Pts',(-15.2636389364423,60.4220936152855,7.17277476395559));
#38579=CARTESIAN_POINT('Ctrl Pts',(-13.3351243759366,60.7764124561446,9.18884518124811));
#38580=CARTESIAN_POINT('Ctrl Pts',(-13.6927968254052,60.5722910266745,11.0072397698831));
#38581=CARTESIAN_POINT('Ctrl Pts',(-14.1985145724512,60.3826426720153,11.6359872033746));
#38582=CARTESIAN_POINT('Ctrl Pts',(-17.2449834421534,67.8425423025984,7.06170475438596));
#38583=CARTESIAN_POINT('Ctrl Pts',(-16.8759806260743,67.9363396049608,7.20780006417468));
#38584=CARTESIAN_POINT('Ctrl Pts',(-16.535804082389,68.0195197262116,7.42431456479993));
#38585=CARTESIAN_POINT('Ctrl Pts',(-15.9848167458479,68.150998080649,7.95780764621744));
#38586=CARTESIAN_POINT('Ctrl Pts',(-15.7699411081763,68.2006822338607,8.25968161903134));
#38587=CARTESIAN_POINT('Ctrl Pts',(-15.4905619320041,68.2646302810789,8.88066242679718));
#38588=CARTESIAN_POINT('Ctrl Pts',(-15.4103584669881,68.2826595052327,9.18497820157355));
#38589=CARTESIAN_POINT('Ctrl Pts',(-15.3584337419011,68.2943569622715,9.79677072277262));
#38590=CARTESIAN_POINT('Ctrl Pts',(-15.3830449856443,68.288855628865,10.0982078060301));
#38591=CARTESIAN_POINT('Ctrl Pts',(-15.5341550196632,68.2546420063796,10.6858944634116));
#38592=CARTESIAN_POINT('Ctrl Pts',(-15.6614146465389,68.2257386849337,10.9661810334232));
#38593=CARTESIAN_POINT('Ctrl Pts',(-16.0093499903202,68.1449424659489,11.4722931322534));
#38594=CARTESIAN_POINT('Ctrl Pts',(-16.2286900565756,68.0932952109551,11.6926718707975));
#38595=CARTESIAN_POINT('Ctrl Pts',(-16.4806955947431,68.0322473001842,11.8669181223569));
#38596=CARTESIAN_POINT('Ctrl Pts',(-14.1985145724512,60.3826426720153,11.6359872033746));
#38597=CARTESIAN_POINT('Ctrl Pts',(-14.1384791309752,60.3987291200761,11.5775783984672));
#38598=CARTESIAN_POINT('Ctrl Pts',(-14.0817003626801,60.413942945188,11.5159169743203));
#38599=CARTESIAN_POINT('Ctrl Pts',(-14.0281914535639,60.4282806141735,11.4513790591575));
#38600=CARTESIAN_POINT('Ctrl Pts',(-13.973376466664,60.4429682456465,11.3852658635676));
#38601=CARTESIAN_POINT('Ctrl Pts',(-13.9219924575667,60.456736549388,11.3161335496572));
#38602=CARTESIAN_POINT('Ctrl Pts',(-13.8740814492191,60.4695742653833,11.24434019589));
#38603=CARTESIAN_POINT('Ctrl Pts',(-13.8615442019958,60.4729336106521,11.225553469077));
#38604=CARTESIAN_POINT('Ctrl Pts',(-13.8492449351277,60.4762291892769,11.2065843090731));
#38605=CARTESIAN_POINT('Ctrl Pts',(-13.8371847672655,60.4794607015161,11.1874386951179));
#38606=CARTESIAN_POINT('Ctrl Pts',(-13.8274131410566,60.4820790008676,11.1719261595341));
#38607=CARTESIAN_POINT('Ctrl Pts',(-13.8177980990722,60.4846553436025,11.1562969508317));
#38608=CARTESIAN_POINT('Ctrl Pts',(-13.8083486579241,60.487187313727,11.140568630092));
#38609=CARTESIAN_POINT('Ctrl Pts',(-13.7625022247112,60.4994718284823,11.0642585716409));
#38610=CARTESIAN_POINT('Ctrl Pts',(-13.7205023351854,60.5107256649629,10.9855425561791));
#38611=CARTESIAN_POINT('Ctrl Pts',(-13.6823842421124,60.5209393772188,10.9048124953012));
#38612=CARTESIAN_POINT('Ctrl Pts',(-13.6519560247452,60.5290925934895,10.8403687720607));
#38613=CARTESIAN_POINT('Ctrl Pts',(-13.6240018721467,60.5365828861033,10.7746405675787));
#38614=CARTESIAN_POINT('Ctrl Pts',(-13.598555660536,60.5434011779549,10.7078100772367));
#38615=CARTESIAN_POINT('Ctrl Pts',(-13.5903398049439,60.5456026098259,10.6862324189903));
#38616=CARTESIAN_POINT('Ctrl Pts',(-13.5823855109655,60.5477339564738,10.6645397516926));
#38617=CARTESIAN_POINT('Ctrl Pts',(-13.5746942694777,60.5497948184192,10.6427379435114));
#38618=CARTESIAN_POINT('Ctrl Pts',(-13.5673646520995,60.5517587834765,10.6219612051427));
#38619=CARTESIAN_POINT('Ctrl Pts',(-13.5602723819539,60.5536591515346,10.6010802048978));
#38620=CARTESIAN_POINT('Ctrl Pts',(-13.5534284149968,60.5554929869537,10.5801302251332));
#38621=CARTESIAN_POINT('Ctrl Pts',(-13.5248766272142,60.5631434154325,10.4927307125355));
#38622=CARTESIAN_POINT('Ctrl Pts',(-13.5006117004349,60.5696451829675,10.4040498990336));
#38623=CARTESIAN_POINT('Ctrl Pts',(-13.480666832402,60.57498939425,10.3144849193173));
#38624=CARTESIAN_POINT('Ctrl Pts',(-13.460414058422,60.5804161086824,10.2235372485817));
#38625=CARTESIAN_POINT('Ctrl Pts',(-13.4446152716974,60.5846493808267,10.1316770971923));
#38626=CARTESIAN_POINT('Ctrl Pts',(-13.4333455934799,60.587669082004,10.0392871198388));
#38627=CARTESIAN_POINT('Ctrl Pts',(-13.4221628859774,60.5906654794485,9.94761013732271));
#38628=CARTESIAN_POINT('Ctrl Pts',(-13.4154393160861,60.5924670545712,9.85541054694995));
#38629=CARTESIAN_POINT('Ctrl Pts',(-13.4132936428762,60.593041985975,9.76304299861578));
#38630=CARTESIAN_POINT('Ctrl Pts',(-13.4122613686534,60.5933185830193,9.71860536536672));
#38631=CARTESIAN_POINT('Ctrl Pts',(-13.4122893693034,60.5933110802678,9.67412865788773));
#38632=CARTESIAN_POINT('Ctrl Pts',(-13.4133950120079,60.593014824198,9.62965173468087));
#38633=CARTESIAN_POINT('Ctrl Pts',(-13.4137601235553,60.5929169928537,9.61496431514677));
#38634=CARTESIAN_POINT('Ctrl Pts',(-13.4142427737453,60.5927876671251,9.60027687123983));
#38635=CARTESIAN_POINT('Ctrl Pts',(-13.4148436567524,60.5926266610086,9.58559080207231));
#38636=CARTESIAN_POINT('Ctrl Pts',(-13.4154511643685,60.5924638798335,9.57074282207608));
#38637=CARTESIAN_POINT('Ctrl Pts',(-13.4161791917116,60.5922688054948,9.55590504990595));
#38638=CARTESIAN_POINT('Ctrl Pts',(-13.4170277181543,60.5920414435197,9.54108357202142));
#38639=CARTESIAN_POINT('Ctrl Pts',(-13.4224967665196,60.5905760164269,9.44555398647223));
#38640=CARTESIAN_POINT('Ctrl Pts',(-13.4329703612428,60.5877696251789,9.35064220222354));
#38641=CARTESIAN_POINT('Ctrl Pts',(-13.4485182643056,60.5836035771093,9.25674298412033));
#38642=CARTESIAN_POINT('Ctrl Pts',(-13.4498478809465,60.5832473074041,9.24871296473712));
#38643=CARTESIAN_POINT('Ctrl Pts',(-13.4512146356318,60.5828810865899,9.24069033922208));
#38644=CARTESIAN_POINT('Ctrl Pts',(-13.4526185882088,60.5825048986307,9.23267534878043));
#38645=CARTESIAN_POINT('Ctrl Pts',(-13.4683901533204,60.5782789204957,9.14263744743809));
#38646=CARTESIAN_POINT('Ctrl Pts',(-13.4888516530656,60.572796278163,9.05356331284174));
#38647=CARTESIAN_POINT('Ctrl Pts',(-13.5137114619772,60.5661351124412,8.96568771726277));
#38648=CARTESIAN_POINT('Ctrl Pts',(-13.5391401674804,60.559321511337,8.8758011598541));
#38649=CARTESIAN_POINT('Ctrl Pts',(-13.5691709812742,60.5512747790329,8.78716792585963));
#38650=CARTESIAN_POINT('Ctrl Pts',(-13.6035442475085,60.5420644901042,8.70004212732541));
#38651=CARTESIAN_POINT('Ctrl Pts',(-13.6224082878329,60.5370098857333,8.65222750983641));
#38652=CARTESIAN_POINT('Ctrl Pts',(-13.6425810892874,60.5316045998745,8.60486701435782));
#38653=CARTESIAN_POINT('Ctrl Pts',(-13.6640258581501,60.5258584913759,8.55800419902235));
#38654=CARTESIAN_POINT('Ctrl Pts',(-13.6704060167119,60.5241489330416,8.54406176884704));
#38655=CARTESIAN_POINT('Ctrl Pts',(-13.6768997658184,60.5224089382127,8.53016150117742));
#38656=CARTESIAN_POINT('Ctrl Pts',(-13.6834982306919,60.5206408848786,8.51632087112045));
#38657=CARTESIAN_POINT('Ctrl Pts',(-13.7247150404844,60.5095968739801,8.42986642642761));
#38658=CARTESIAN_POINT('Ctrl Pts',(-13.7700718774285,60.4974435461497,8.3456074465938));
#38659=CARTESIAN_POINT('Ctrl Pts',(-13.8192407166192,60.4842687953957,8.2637970860201));
#38660=CARTESIAN_POINT('Ctrl Pts',(-13.869379078653,60.470834261779,8.18037356933611));
#38661=CARTESIAN_POINT('Ctrl Pts',(-13.9234815557643,60.4563375467285,8.09949541154091));
#38662=CARTESIAN_POINT('Ctrl Pts',(-13.9812533712864,60.4408576354141,8.02143790718841));
#38663=CARTESIAN_POINT('Ctrl Pts',(-14.039482634331,60.4252551514054,7.94276232961702));
#38664=CARTESIAN_POINT('Ctrl Pts',(-14.1014400131933,60.4086537217741,7.86695140903171));
#38665=CARTESIAN_POINT('Ctrl Pts',(-14.16687127419,60.3911214682303,7.79430622921448));
#38666=CARTESIAN_POINT('Ctrl Pts',(-14.2014931148633,60.3818445739814,7.75586726589624));
#38667=CARTESIAN_POINT('Ctrl Pts',(-14.2370883362474,60.3723068631571,7.71831505022628));
#38668=CARTESIAN_POINT('Ctrl Pts',(-14.2736239454352,60.3625171761803,7.68169758983469));
#38669=CARTESIAN_POINT('Ctrl Pts',(-14.2866331258705,60.3590313767884,7.66865926476215));
#38670=CARTESIAN_POINT('Ctrl Pts',(-14.2997615606732,60.3555136232852,7.65573947805022));
#38671=CARTESIAN_POINT('Ctrl Pts',(-14.313007848791,60.3519642910813,7.64294048667691));
#38672=CARTESIAN_POINT('Ctrl Pts',(-14.323185153228,60.3492372905763,7.63310684644997));
#38673=CARTESIAN_POINT('Ctrl Pts',(-14.3334310227586,60.3464919181098,7.62334556315778));
#38674=CARTESIAN_POINT('Ctrl Pts',(-14.3437359536144,60.3437307202089,7.61366571173162));
#38675=CARTESIAN_POINT('Ctrl Pts',(-14.4166886967228,60.3241830916074,7.545138156884));
#38676=CARTESIAN_POINT('Ctrl Pts',(-14.4927140801617,60.3038121515107,7.48057696472124));
#38677=CARTESIAN_POINT('Ctrl Pts',(-14.5714997183224,60.2827016033904,7.42026730047636));
#38678=CARTESIAN_POINT('Ctrl Pts',(-14.6503851320848,60.2615643204781,7.35988125894772));
#38679=CARTESIAN_POINT('Ctrl Pts',(-14.7320383428994,60.239685408581,7.30375667613358));
#38680=CARTESIAN_POINT('Ctrl Pts',(-14.8161894526237,60.2171371866881,7.25220561239913));
#38681=CARTESIAN_POINT('Ctrl Pts',(-14.8987454236577,60.1950163809192,7.20163173240665));
#38682=CARTESIAN_POINT('Ctrl Pts',(-14.9837061239422,60.1722512298896,7.15545893560281));
#38683=CARTESIAN_POINT('Ctrl Pts',(-15.0708497995124,60.1489011523951,7.11401788937555));
#38684=CARTESIAN_POINT('Ctrl Pts',(-15.0979686080361,60.1416346895515,7.10112158002999));
#38685=CARTESIAN_POINT('Ctrl Pts',(-15.1252990311688,60.1343115247443,7.08868381630056));
#38686=CARTESIAN_POINT('Ctrl Pts',(-15.1528349118071,60.1269333077643,7.07671545672048));
#38687=CARTESIAN_POINT('Ctrl Pts',(-15.1941283917652,60.1158687531569,7.05876741202411));
#38688=CARTESIAN_POINT('Ctrl Pts',(-15.2358838838844,60.104680402764,7.04187489341853));
#38689=CARTESIAN_POINT('Ctrl Pts',(-15.2780676602838,60.0933772939441,7.02603075613018));
#38690=CARTESIAN_POINT('Ctrl Pts',(-15.458048217099,67.4086397233445,10.0018117506529));
#38691=CARTESIAN_POINT('Ctrl Pts',(-15.4516726940089,67.3922281881599,10.2792252787833));
#38692=CARTESIAN_POINT('Ctrl Pts',(-15.4881185773169,67.3643426917121,10.5560719127005));
#38693=CARTESIAN_POINT('Ctrl Pts',(-15.5698466331083,67.3243238737159,10.8168646145652));
#38694=CARTESIAN_POINT('Ctrl Pts',(-15.8140481541641,67.2047485806184,11.5961071140829));
#38695=CARTESIAN_POINT('Ctrl Pts',(-16.4625291088523,66.9768469397627,12.2320200381452));
#38696=CARTESIAN_POINT('Ctrl Pts',(-17.2188383863877,66.7200527868788,12.4398697983788));
#38697=CARTESIAN_POINT('Ctrl Pts',(-17.975147663923,66.463258633995,12.6477195586124));
#38698=CARTESIAN_POINT('Ctrl Pts',(-18.8392852643055,66.1775719690831,12.4275061550173));
#38699=CARTESIAN_POINT('Ctrl Pts',(-19.4182523936636,65.9682965015874,11.8778290289184));
#38700=CARTESIAN_POINT('Ctrl Pts',(-19.9972195230217,65.7590210340917,11.3281519028195));
#38701=CARTESIAN_POINT('Ctrl Pts',(-20.2910161813554,65.6261567640121,10.4490110542167));
#38702=CARTESIAN_POINT('Ctrl Pts',(-20.1620218299581,65.6065790035572,9.63407278056648));
#38703=CARTESIAN_POINT('Ctrl Pts',(-20.0330274785608,65.5870012431022,8.81913450691625));
#38704=CARTESIAN_POINT('Ctrl Pts',(-19.4812421174325,65.6807099922718,8.06839880821855));
#38705=CARTESIAN_POINT('Ctrl Pts',(-18.7476852845614,65.8231242605018,7.71802880880736));
#38706=CARTESIAN_POINT('Ctrl Pts',(-18.0141284516903,65.9655385287319,7.36765880939615));
#38707=CARTESIAN_POINT('Ctrl Pts',(-17.0988001470764,66.1566583160224,7.41765450927146));
#38708=CARTESIAN_POINT('Ctrl Pts',(-16.4055051616428,66.2882844547459,7.84562973884635));
#38709=CARTESIAN_POINT('Ctrl Pts',(-15.7122101762091,66.4199105934693,8.27360496842124));
#38710=CARTESIAN_POINT('Ctrl Pts',(-15.2409485099557,66.4920430836257,9.07955972769568));
#38711=CARTESIAN_POINT('Ctrl Pts',(-15.1966815676295,66.4497626823333,9.90260247183681));
#38712=CARTESIAN_POINT('Ctrl Pts',(-15.194946550497,66.4481055265245,9.93486115488302));
#38713=CARTESIAN_POINT('Ctrl Pts',(-15.1938674837542,66.4462726093384,9.9671460885354));
#38714=CARTESIAN_POINT('Ctrl Pts',(-15.1934336836835,66.4442667934687,9.99943462192771));
#38715=CARTESIAN_POINT('Origin',(17.0820569767664,-63.7511045350785,10.));
#38716=CARTESIAN_POINT('Origin',(16.0467807963563,-59.8874012299222,10.));
#38717=CARTESIAN_POINT('Origin',(-63.7511045350785,-17.0820569767664,10.));
#38718=CARTESIAN_POINT('Origin',(-59.8874012299222,-16.0467807963563,10.));
#38719=CARTESIAN_POINT('Origin',(-17.0820569767664,63.7511045350785,10.));
#38720=CARTESIAN_POINT('Origin',(-16.0467807963563,59.8874012299222,10.));
#38721=CARTESIAN_POINT('Ctrl Pts',(67.0040126136404,20.25986904378,11.1728309286208));
#38722=CARTESIAN_POINT('Ctrl Pts',(66.854289394458,20.6173045957293,10.4434664543485));
#38723=CARTESIAN_POINT('Ctrl Pts',(66.7561954352347,20.5807180172414,8.59013022403084));
#38724=CARTESIAN_POINT('Ctrl Pts',(67.2090412643979,18.2866570474722,7.05024279158514));
#38725=CARTESIAN_POINT('Ctrl Pts',(67.7235827819968,15.7623446338521,8.14059085434232));
#38726=CARTESIAN_POINT('Ctrl Pts',(67.7078986042172,15.216861454864,10.8824467802982));
#38727=CARTESIAN_POINT('Ctrl Pts',(67.0414893382908,17.0999173665985,12.8405694561119));
#38728=CARTESIAN_POINT('Ctrl Pts',(66.1829652216242,19.6999556621848,12.270731917377));
#38729=CARTESIAN_POINT('Ctrl Pts',(65.7617874756575,20.6677950818131,9.68094249642526));
#38730=CARTESIAN_POINT('Ctrl Pts',(66.0183437425752,19.1062967313387,7.37485535276711));
#38731=CARTESIAN_POINT('Ctrl Pts',(66.5900180970019,16.3687616678975,7.40446197973336));
#38732=CARTESIAN_POINT('Ctrl Pts',(66.8338405096701,14.8547867084588,9.74329926128817));
#38733=CARTESIAN_POINT('Ctrl Pts',(66.3985290187163,15.8753739824799,12.3105450512028));
#38734=CARTESIAN_POINT('Ctrl Pts',(65.5370346894516,18.4864972623911,12.8220707222439));
#38735=CARTESIAN_POINT('Ctrl Pts',(64.8814857844687,20.3290217552966,10.8227823754311));
#38736=CARTESIAN_POINT('Ctrl Pts',(64.8807798084461,19.7276391663451,8.09145561890055));
#38737=CARTESIAN_POINT('Ctrl Pts',(65.4011950297316,17.1814057921382,7.0581771851638));
#38738=CARTESIAN_POINT('Ctrl Pts',(65.8453641599238,14.9197267037703,8.64226139479096));
#38739=CARTESIAN_POINT('Ctrl Pts',(65.6837566027253,14.9188369907852,11.4343367521439));
#38740=CARTESIAN_POINT('Ctrl Pts',(64.9258061425712,17.1435292903637,12.9502711232991));
#38741=CARTESIAN_POINT('Ctrl Pts',(64.1115175849317,19.5784782321595,11.8413258175013));
#38742=CARTESIAN_POINT('Ctrl Pts',(63.831020197438,20.0212914063393,9.09413821413814));
#38743=CARTESIAN_POINT('Ctrl Pts',(64.1995249831397,18.0419954959312,7.15290308224174));
#38744=CARTESIAN_POINT('Ctrl Pts',(64.7548205378835,15.3655869450733,7.74475277436874));
#38745=CARTESIAN_POINT('Ctrl Pts',(64.8685062198083,14.3372888766999,10.3431139119316));
#38746=CARTESIAN_POINT('Ctrl Pts',(64.305085213021,15.8359873727446,12.6362038638412));
#38747=CARTESIAN_POINT('Ctrl Pts',(63.4314879220137,18.4922795208015,12.5838422163727));
#38748=CARTESIAN_POINT('Ctrl Pts',(62.8906110650171,19.9068421044142,10.2326155433119));
#38749=CARTESIAN_POINT('Ctrl Pts',(63.0293273367051,18.7851286033011,7.67442896667236));
#38750=CARTESIAN_POINT('Ctrl Pts',(63.5898700057829,16.0891375551554,7.18532148363251));
#38751=CARTESIAN_POINT('Ctrl Pts',(63.9391700310929,14.1815147862765,9.20045592301428));
#38752=CARTESIAN_POINT('Ctrl Pts',(63.6321026366037,14.7234885765209,11.926951102987));
#38753=CARTESIAN_POINT('Ctrl Pts',(62.8075183731852,17.1968616153839,12.9390225214355));
#38754=CARTESIAN_POINT('Ctrl Pts',(62.0647066785609,19.3650552728408,11.3362221619436));
#38755=CARTESIAN_POINT('Ctrl Pts',(61.9302032807139,19.2630114600595,8.54457429525403));
#38756=CARTESIAN_POINT('Ctrl Pts',(62.3893271714101,16.9455204456759,7.04783027207108));
#38757=CARTESIAN_POINT('Ctrl Pts',(62.8992423967485,14.4384735898227,8.1776552235704));
#38758=CARTESIAN_POINT('Ctrl Pts',(62.8719235739435,13.9364114971972,10.9288348037815));
#38759=CARTESIAN_POINT('Ctrl Pts',(62.1973266831092,15.850024041082,12.853622756267));
#38760=CARTESIAN_POINT('Ctrl Pts',(61.3412962728356,18.4407556977103,12.2395195742226));
#38761=CARTESIAN_POINT('Ctrl Pts',(60.9310995184378,19.3676134988853,9.63289839745389));
#38762=CARTESIAN_POINT('Ctrl Pts',(61.19734228766,17.7699646296638,7.35288957156125));
#38763=CARTESIAN_POINT('Ctrl Pts',(61.7687958934069,15.0332534115107,7.42803777444101));
#38764=CARTESIAN_POINT('Ctrl Pts',(62.0026849934363,13.5563500795275,9.79147768508998));
#38765=CARTESIAN_POINT('Ctrl Pts',(61.5565643024821,14.6172778371391,12.3404488591357));
#38766=CARTESIAN_POINT('Ctrl Pts',(60.6930063334388,17.236102725553,12.807089206987));
#38767=CARTESIAN_POINT('Ctrl Pts',(60.0459653166684,19.0468753473843,10.7762699688266));
#38768=CARTESIAN_POINT('Ctrl Pts',(60.0567902041013,18.4024589901613,8.05473611617474));
#38769=CARTESIAN_POINT('Ctrl Pts',(60.5814573009746,15.8403574002339,7.06404294414452));
#38770=CARTESIAN_POINT('Ctrl Pts',(61.0189035288689,13.6037685248159,8.68524269063554));
#38771=CARTESIAN_POINT('Ctrl Pts',(60.8454027634006,13.6472648693585,11.4767030328865));
#38772=CARTESIAN_POINT('Ctrl Pts',(60.0813295310042,15.8948076660285,12.9532921034687));
#38773=CARTESIAN_POINT('Ctrl Pts',(59.2714063402786,18.3134648367079,11.8044287744805));
#38774=CARTESIAN_POINT('Ctrl Pts',(59.0033710168103,18.7097689547777,9.04578082775238));
#38775=CARTESIAN_POINT('Ctrl Pts',(59.2532824184769,17.3744086881427,7.78080120942675));
#38776=CARTESIAN_POINT('Ctrl Pts',(59.4090483774018,16.5917431062329,7.56791319796499));
#38777=CARTESIAN_POINT('Ctrl Pts',(67.0649244254632,20.4459680138347,11.259172404465));
#38778=CARTESIAN_POINT('Ctrl Pts',(66.9078844272409,20.8307101569087,10.4761135710142));
#38779=CARTESIAN_POINT('Ctrl Pts',(66.8099800782135,20.7934159435358,8.48633842059636));
#38780=CARTESIAN_POINT('Ctrl Pts',(67.3072801529265,18.3334494707627,6.83308754393488));
#38781=CARTESIAN_POINT('Ctrl Pts',(67.8708178297157,15.6262809016687,8.0037048583164));
#38782=CARTESIAN_POINT('Ctrl Pts',(67.8650956520228,15.0436190322123,10.9474107537965));
#38783=CARTESIAN_POINT('Ctrl Pts',(67.160743301905,17.0682804619447,13.049686519018));
#38784=CARTESIAN_POINT('Ctrl Pts',(66.2501329885663,19.8627070898848,12.4378986762067));
#38785=CARTESIAN_POINT('Ctrl Pts',(65.8090656142303,20.9047756131302,9.65745411880361));
#38786=CARTESIAN_POINT('Ctrl Pts',(66.0956256802751,19.231301559894,7.18159743500988));
#38787=CARTESIAN_POINT('Ctrl Pts',(66.7205021994896,16.2952133143915,7.21338364285575));
#38788=CARTESIAN_POINT('Ctrl Pts',(66.9933909703099,14.6727612295384,9.72440146443628));
#38789=CARTESIAN_POINT('Ctrl Pts',(66.5371493528457,15.7714607991054,12.4806427736084));
#38790=CARTESIAN_POINT('Ctrl Pts',(65.6233501657761,18.5777884658271,13.0298259452254));
#38791=CARTESIAN_POINT('Ctrl Pts',(64.9306576947328,20.558934634444,10.8833539743374));
#38792=CARTESIAN_POINT('Ctrl Pts',(64.9410163841629,19.9162581518544,7.95095238475408));
#38793=CARTESIAN_POINT('Ctrl Pts',(65.5108601749995,17.1855548447374,6.84160605175778));
#38794=CARTESIAN_POINT('Ctrl Pts',(65.9988447894534,14.7603541429465,8.54230738426514));
#38795=CARTESIAN_POINT('Ctrl Pts',(65.8364566439329,14.7623776252392,11.5399297656086));
#38796=CARTESIAN_POINT('Ctrl Pts',(65.0338240192841,17.1538260329039,13.167464204339));
#38797=CARTESIAN_POINT('Ctrl Pts',(64.1707057986789,19.7710097578038,11.9768805549434));
#38798=CARTESIAN_POINT('Ctrl Pts',(63.8806753904707,20.2494006496399,9.02745047458975));
#38799=CARTESIAN_POINT('Ctrl Pts',(64.2874254021705,18.1273716126603,6.94330548061664));
#38800=CARTESIAN_POINT('Ctrl Pts',(64.8947173471079,15.2569098917896,7.5787259676887));
#38801=CARTESIAN_POINT('Ctrl Pts',(65.0278889803931,14.1558892629051,10.3683732743989));
#38802=CARTESIAN_POINT('Ctrl Pts',(64.4341066798258,15.7678976499205,12.8302759390873));
#38803=CARTESIAN_POINT('Ctrl Pts',(63.5073135350879,18.6227194268519,12.7740595314741));
#38804=CARTESIAN_POINT('Ctrl Pts',(62.9377350396946,20.1443979832212,10.2497402360735));
#38805=CARTESIAN_POINT('Ctrl Pts',(63.0977799648827,18.9430848635892,7.50322506140521));
#38806=CARTESIAN_POINT('Ctrl Pts',(63.7107053062553,16.0515990210029,6.97811046011707));
#38807=CARTESIAN_POINT('Ctrl Pts',(64.096836741373,14.0065195594074,9.14159508133219));
#38808=CARTESIAN_POINT('Ctrl Pts',(63.7782802952008,14.5913710742637,12.0688094033194));
#38809=CARTESIAN_POINT('Ctrl Pts',(62.9041084194735,17.2498076016885,13.1553875028215));
#38810=CARTESIAN_POINT('Ctrl Pts',(62.1177290461058,19.5805980497845,11.4345921747925));
#38811=CARTESIAN_POINT('Ctrl Pts',(61.9844404141371,19.4740206690255,8.43742875512311));
#38812=CARTESIAN_POINT('Ctrl Pts',(62.4884807287628,16.9888992784431,6.83049741954166));
#38813=CARTESIAN_POINT('Ctrl Pts',(63.0470515348742,14.3002673230733,8.04349783254823));
#38814=CARTESIAN_POINT('Ctrl Pts',(63.0288381927736,13.7642231138315,10.9972137711304));
#38815=CARTESIAN_POINT('Ctrl Pts',(62.3156954611178,15.8216906940825,13.063700777119));
#38816=CARTESIAN_POINT('Ctrl Pts',(61.4077624358673,18.6061255468499,12.4043885425467));
#38817=CARTESIAN_POINT('Ctrl Pts',(60.9784844518179,19.6041954665562,9.60587310900428));
#38818=CARTESIAN_POINT('Ctrl Pts',(61.275444121164,17.8919095654206,7.15801457676324));
#38819=CARTESIAN_POINT('Ctrl Pts',(61.9000836406211,14.9567058150546,7.23869504058986));
#38820=CARTESIAN_POINT('Ctrl Pts',(62.1623078281203,13.374054496997,9.77612668779241));
#38821=CARTESIAN_POINT('Ctrl Pts',(61.6944612588913,14.5160643361693,12.5127480402915));
#38822=CARTESIAN_POINT('Ctrl Pts',(60.7784465109949,17.3306605884645,13.0137415206692));
#38823=CARTESIAN_POINT('Ctrl Pts',(60.0948882619405,19.2777173765313,10.8334174170447));
#38824=CARTESIAN_POINT('Ctrl Pts',(60.117626694016,18.5888390654042,7.91152966540919));
#38825=CARTESIAN_POINT('Ctrl Pts',(60.6920353750482,15.8410993561462,6.84790363622586));
#38826=CARTESIAN_POINT('Ctrl Pts',(61.172802160534,13.4428359587848,8.58845287746021));
#38827=CARTESIAN_POINT('Ctrl Pts',(60.9976452524506,13.4925131117115,11.5854149675154));
#38828=CARTESIAN_POINT('Ctrl Pts',(60.1884391092681,15.908494224529,13.1707075830487));
#38829=CARTESIAN_POINT('Ctrl Pts',(59.3300076251901,18.5081868105878,11.9372672251407));
#38830=CARTESIAN_POINT('Ctrl Pts',(59.0533567133274,18.9366447422826,8.97553311378089));
#38831=CARTESIAN_POINT('Ctrl Pts',(59.3290771863822,17.5049637099304,7.61742821670134));
#38832=CARTESIAN_POINT('Ctrl Pts',(59.5000158708058,16.6656727455702,7.38886781406145));
#38833=CARTESIAN_POINT('Ctrl Pts',(67.125836237286,20.6320669838895,11.3455138803092));
#38834=CARTESIAN_POINT('Ctrl Pts',(66.9614794600237,21.0441157180881,10.5087606876799));
#38835=CARTESIAN_POINT('Ctrl Pts',(66.8637647211924,21.0061138698302,8.38254661716189));
#38836=CARTESIAN_POINT('Ctrl Pts',(67.4055190414551,18.3802418940533,6.6159322962846));
#38837=CARTESIAN_POINT('Ctrl Pts',(68.0180528774347,15.4902171694853,7.8668188622905));
#38838=CARTESIAN_POINT('Ctrl Pts',(68.0222926998282,14.8703766095605,11.0123747272948));
#38839=CARTESIAN_POINT('Ctrl Pts',(67.2799972655193,17.036643557291,13.2588035819241));
#38840=CARTESIAN_POINT('Ctrl Pts',(66.3173007555082,20.0254585175847,12.6050654350364));
#38841=CARTESIAN_POINT('Ctrl Pts',(65.8563437528032,21.1417561444473,9.63396574118195));
#38842=CARTESIAN_POINT('Ctrl Pts',(66.1729076179749,19.3563063884493,6.98833951725265));
#38843=CARTESIAN_POINT('Ctrl Pts',(66.8509863019774,16.2216649608855,7.02230530597812));
#38844=CARTESIAN_POINT('Ctrl Pts',(67.1529414309498,14.4907357506179,9.70550366758441));
#38845=CARTESIAN_POINT('Ctrl Pts',(66.675769686975,15.6675476157309,12.6507404960141));
#38846=CARTESIAN_POINT('Ctrl Pts',(65.7096656421006,18.6690796692631,13.2375811682069));
#38847=CARTESIAN_POINT('Ctrl Pts',(64.979829604997,20.7888475135915,10.9439255732437));
#38848=CARTESIAN_POINT('Ctrl Pts',(65.0012529598797,20.1048771373638,7.81044915060759));
#38849=CARTESIAN_POINT('Ctrl Pts',(65.6205253202674,17.1897038973366,6.62503491835178));
#38850=CARTESIAN_POINT('Ctrl Pts',(66.1523254189831,14.6009815821227,8.44235337373932));
#38851=CARTESIAN_POINT('Ctrl Pts',(65.9891566851404,14.6059182596932,11.6455227790733));
#38852=CARTESIAN_POINT('Ctrl Pts',(65.141841895997,17.1641227754441,13.384657285379));
#38853=CARTESIAN_POINT('Ctrl Pts',(64.2298940124262,19.9635412834481,12.1124352923854));
#38854=CARTESIAN_POINT('Ctrl Pts',(63.9303305835034,20.4775098929406,8.96076273504136));
#38855=CARTESIAN_POINT('Ctrl Pts',(64.3753258212011,18.2127477293894,6.73370787899155));
#38856=CARTESIAN_POINT('Ctrl Pts',(65.0346141563323,15.148232838506,7.41269916100866));
#38857=CARTESIAN_POINT('Ctrl Pts',(65.1872717409779,13.9744896491103,10.3936326368662));
#38858=CARTESIAN_POINT('Ctrl Pts',(64.5631281466306,15.6998079270964,13.0243480143333));
#38859=CARTESIAN_POINT('Ctrl Pts',(63.5831391481621,18.7531593329024,12.9642768465755));
#38860=CARTESIAN_POINT('Ctrl Pts',(62.9848590143723,20.3819538620282,10.266864928835));
#38861=CARTESIAN_POINT('Ctrl Pts',(63.1662325930602,19.1010411238774,7.33202115613807));
#38862=CARTESIAN_POINT('Ctrl Pts',(63.8315406067278,16.0140604868503,6.77089943660162));
#38863=CARTESIAN_POINT('Ctrl Pts',(64.254503451653,13.8315243325383,9.08273423965009));
#38864=CARTESIAN_POINT('Ctrl Pts',(63.9244579537979,14.4592535720065,12.2106677036519));
#38865=CARTESIAN_POINT('Ctrl Pts',(63.000698465762,17.3027535879931,13.3717524842076));
#38866=CARTESIAN_POINT('Ctrl Pts',(62.1707514136505,19.7961408267281,11.5329621876413));
#38867=CARTESIAN_POINT('Ctrl Pts',(62.0386775475604,19.6850298779916,8.3302832149922));
#38868=CARTESIAN_POINT('Ctrl Pts',(62.5876342861153,17.0322781112102,6.61316456701223));
#38869=CARTESIAN_POINT('Ctrl Pts',(63.1948606729998,14.1620610563239,7.90934044152608));
#38870=CARTESIAN_POINT('Ctrl Pts',(63.1857528116037,13.5920347304658,11.0655927384792));
#38871=CARTESIAN_POINT('Ctrl Pts',(62.4340642391263,15.7933573470829,13.273778797971));
#38872=CARTESIAN_POINT('Ctrl Pts',(61.4742285988992,18.7714953959895,12.5692575108708));
#38873=CARTESIAN_POINT('Ctrl Pts',(61.0258693851979,19.8407774342272,9.57884782055468));
#38874=CARTESIAN_POINT('Ctrl Pts',(61.3535459546682,18.0138545011774,6.96313958196523));
#38875=CARTESIAN_POINT('Ctrl Pts',(62.0313713878352,14.8801582185986,7.04935230673873));
#38876=CARTESIAN_POINT('Ctrl Pts',(62.3219306628043,13.1917589144664,9.76077569049482));
#38877=CARTESIAN_POINT('Ctrl Pts',(61.8323582153006,14.4148508351995,12.6850472214474));
#38878=CARTESIAN_POINT('Ctrl Pts',(60.8638866885509,17.425218451376,13.2203938343514));
#38879=CARTESIAN_POINT('Ctrl Pts',(60.1438112072126,19.5085594056783,10.8905648652629));
#38880=CARTESIAN_POINT('Ctrl Pts',(60.1784631839306,18.7752191406471,7.76832321464364));
#38881=CARTESIAN_POINT('Ctrl Pts',(60.8026134491219,15.8418413120585,6.6317643283072));
#38882=CARTESIAN_POINT('Ctrl Pts',(61.3267007921991,13.2819033927538,8.49166306428489));
#38883=CARTESIAN_POINT('Ctrl Pts',(61.1498877415007,13.3377613540646,11.6941269021443));
#38884=CARTESIAN_POINT('Ctrl Pts',(60.2955486875319,15.9221807830296,13.3881230626288));
#38885=CARTESIAN_POINT('Ctrl Pts',(59.3886089101015,18.7029087844678,12.0701056758009));
#38886=CARTESIAN_POINT('Ctrl Pts',(59.1033424098445,19.1635205297874,8.9052853998094));
#38887=CARTESIAN_POINT('Ctrl Pts',(59.4048719542876,17.6355187317182,7.45405522397592));
#38888=CARTESIAN_POINT('Ctrl Pts',(59.5909833642099,16.7396023849075,7.20982243015791));
#38889=CARTESIAN_POINT('Ctrl Pts',(67.1867480491087,20.8181659539443,11.4318553561534));
#38890=CARTESIAN_POINT('Ctrl Pts',(67.0150744928066,21.2575212792675,10.5414078043456));
#38891=CARTESIAN_POINT('Ctrl Pts',(66.9175493641713,21.2188117961246,8.27875481372742));
#38892=CARTESIAN_POINT('Ctrl Pts',(67.5037579299836,18.4270343173439,6.39877704863433));
#38893=CARTESIAN_POINT('Ctrl Pts',(68.1652879251536,15.3541534373019,7.72993286626459));
#38894=CARTESIAN_POINT('Ctrl Pts',(68.1794897476338,14.6971341869088,11.0773387007931));
#38895=CARTESIAN_POINT('Ctrl Pts',(67.3992512291335,17.0050066526372,13.4679206448302));
#38896=CARTESIAN_POINT('Ctrl Pts',(66.3844685224502,20.1882099452846,12.7722321938662));
#38897=CARTESIAN_POINT('Ctrl Pts',(65.9036218913761,21.3787366757644,9.61047736356028));
#38898=CARTESIAN_POINT('Ctrl Pts',(66.2501895556748,19.4813112170046,6.79508159949543));
#38899=CARTESIAN_POINT('Ctrl Pts',(66.9814704044652,16.1481166073795,6.83122696910049));
#38900=CARTESIAN_POINT('Ctrl Pts',(67.3124918915896,14.3087102716975,9.68660587073254));
#38901=CARTESIAN_POINT('Ctrl Pts',(66.8143900211043,15.5636344323564,12.8208382184197));
#38902=CARTESIAN_POINT('Ctrl Pts',(65.795981118425,18.7603708726991,13.4453363911884));
#38903=CARTESIAN_POINT('Ctrl Pts',(65.0290015152611,21.0187603927389,11.00449717215));
#38904=CARTESIAN_POINT('Ctrl Pts',(65.0614895355965,20.2934961228732,7.66994591646111));
#38905=CARTESIAN_POINT('Ctrl Pts',(65.7301904655353,17.1938529499358,6.40846378494576));
#38906=CARTESIAN_POINT('Ctrl Pts',(66.3058060485126,14.441609021299,8.34239936321351));
#38907=CARTESIAN_POINT('Ctrl Pts',(66.141856726348,14.4494588941473,11.7511157925379));
#38908=CARTESIAN_POINT('Ctrl Pts',(65.2498597727098,17.1744195179844,13.6018503664189));
#38909=CARTESIAN_POINT('Ctrl Pts',(64.2890822261735,20.1560728090925,12.2479900298274));
#38910=CARTESIAN_POINT('Ctrl Pts',(63.9799857765362,20.7056191362412,8.89407499549297));
#38911=CARTESIAN_POINT('Ctrl Pts',(64.4632262402319,18.2981238461185,6.52411027736645));
#38912=CARTESIAN_POINT('Ctrl Pts',(65.1745109655566,15.0395557852223,7.24667235432862));
#38913=CARTESIAN_POINT('Ctrl Pts',(65.3466545015629,13.7930900353155,10.4188919993334));
#38914=CARTESIAN_POINT('Ctrl Pts',(64.6921496134354,15.6317182042723,13.2184200895793));
#38915=CARTESIAN_POINT('Ctrl Pts',(63.6589647612363,18.8835992389528,13.1544941616769));
#38916=CARTESIAN_POINT('Ctrl Pts',(63.0319829890499,20.6195097408352,10.2839896215965));
#38917=CARTESIAN_POINT('Ctrl Pts',(63.2346852212378,19.2589973841656,7.16081725087092));
#38918=CARTESIAN_POINT('Ctrl Pts',(63.9523759072002,15.9765219526977,6.56368841308618));
#38919=CARTESIAN_POINT('Ctrl Pts',(64.4121701619331,13.6565291056693,9.023873397968));
#38920=CARTESIAN_POINT('Ctrl Pts',(64.0706356123949,14.3271360697493,12.3525260039843));
#38921=CARTESIAN_POINT('Ctrl Pts',(63.0972885120504,17.3556995742977,13.5881174655937));
#38922=CARTESIAN_POINT('Ctrl Pts',(62.2237737811953,20.0116836036718,11.6313322004901));
#38923=CARTESIAN_POINT('Ctrl Pts',(62.0929146809836,19.8960390869576,8.22313767486128));
#38924=CARTESIAN_POINT('Ctrl Pts',(62.686787843468,17.0756569439774,6.3958317144828));
#38925=CARTESIAN_POINT('Ctrl Pts',(63.3426698111255,14.0238547895745,7.77518305050392));
#38926=CARTESIAN_POINT('Ctrl Pts',(63.3426674304337,13.4198463471001,11.1339717058281));
#38927=CARTESIAN_POINT('Ctrl Pts',(62.552433017135,15.7650240000834,13.4838568188229));
#38928=CARTESIAN_POINT('Ctrl Pts',(61.540694761931,18.936865245129,12.7341264791949));
#38929=CARTESIAN_POINT('Ctrl Pts',(61.0732543185778,20.0773594018982,9.55182253210507));
#38930=CARTESIAN_POINT('Ctrl Pts',(61.4316477881723,18.1357994369342,6.76826458716723));
#38931=CARTESIAN_POINT('Ctrl Pts',(62.1626591350493,14.8036106221425,6.86000957288757));
#38932=CARTESIAN_POINT('Ctrl Pts',(62.4815534974884,13.0094633319359,9.74542469319725));
#38933=CARTESIAN_POINT('Ctrl Pts',(61.9702551717097,14.3136373342297,12.8573464026032));
#38934=CARTESIAN_POINT('Ctrl Pts',(60.949326866107,17.5197763142875,13.4270461480336));
#38935=CARTESIAN_POINT('Ctrl Pts',(60.1927341524847,19.7394014348252,10.947712313481));
#38936=CARTESIAN_POINT('Ctrl Pts',(60.2392996738452,18.96159921589,7.62511676387808));
#38937=CARTESIAN_POINT('Ctrl Pts',(60.9131915231956,15.8425832679708,6.41562502038855));
#38938=CARTESIAN_POINT('Ctrl Pts',(61.4805994238642,13.1209708267227,8.39487325110957));
#38939=CARTESIAN_POINT('Ctrl Pts',(61.3021302305506,13.1830095964177,11.8028388367732));
#38940=CARTESIAN_POINT('Ctrl Pts',(60.4026582657957,15.9358673415302,13.6055385422089));
#38941=CARTESIAN_POINT('Ctrl Pts',(59.447210195013,18.8976307583478,12.2029441264611));
#38942=CARTESIAN_POINT('Ctrl Pts',(59.1533281063616,19.3903963172923,8.83503768583792));
#38943=CARTESIAN_POINT('Ctrl Pts',(59.4806667221929,17.7660737535059,7.2906822312505));
#38944=CARTESIAN_POINT('Ctrl Pts',(59.6819508576139,16.8135320242448,7.03077704625438));
#38945=CARTESIAN_POINT('Ctrl Pts',(67.0040126136404,20.2598690437801,11.1728309286207));
#38946=CARTESIAN_POINT('Ctrl Pts',(66.9555034255254,20.4203000043805,10.9082027524038));
#38947=CARTESIAN_POINT('Ctrl Pts',(66.9207835851305,20.5332184525385,10.6149904639444));
#38948=CARTESIAN_POINT('Ctrl Pts',(66.8813975908017,20.6611539455099,9.99178401342255));
#38949=CARTESIAN_POINT('Ctrl Pts',(66.8780249511107,20.6720025707686,9.66515229429171));
#38950=CARTESIAN_POINT('Ctrl Pts',(66.904675210205,20.5855924444283,9.00098486496477));
#38951=CARTESIAN_POINT('Ctrl Pts',(66.9367881932439,20.4815398383751,8.66883374311739));
#38952=CARTESIAN_POINT('Ctrl Pts',(67.0315956493191,20.1690707048657,8.06423785428611));
#38953=CARTESIAN_POINT('Ctrl Pts',(67.09312085238,19.9644265611134,7.79496359360553));
#38954=CARTESIAN_POINT('Ctrl Pts',(67.2425937581436,19.4553169386786,7.32570054462924));
#38955=CARTESIAN_POINT('Ctrl Pts',(67.33085397004,19.148781829213,7.13688275745713));
#38956=CARTESIAN_POINT('Ctrl Pts',(67.4238662472344,18.8154792730625,7.01293629783555));
#38957=CARTESIAN_POINT('Ctrl Pts',(66.709565290414,15.2652009106025,9.99881345470567));
#38958=CARTESIAN_POINT('Ctrl Pts',(66.7141255555458,15.2659775128488,9.92620926472459));
#38959=CARTESIAN_POINT('Ctrl Pts',(66.7178306708093,15.2699455778512,9.85363960672269));
#38960=CARTESIAN_POINT('Ctrl Pts',(66.7206515257331,15.2772137473688,9.78136734601481));
#38961=CARTESIAN_POINT('Ctrl Pts',(66.752566372114,15.3594450282717,8.96368683410324));
#38962=CARTESIAN_POINT('Ctrl Pts',(66.6712922345579,15.8641033480846,8.1840744069183));
#38963=CARTESIAN_POINT('Ctrl Pts',(66.5353761067088,16.5726883518979,7.78933375549813));
#38964=CARTESIAN_POINT('Ctrl Pts',(66.3994599788597,17.2812733557112,7.39459310407795));
#38965=CARTESIAN_POINT('Ctrl Pts',(66.2089018607174,18.193785043525,7.38472422842254));
#38966=CARTESIAN_POINT('Ctrl Pts',(66.0708634238267,18.9102906125109,7.76413764787119));
#38967=CARTESIAN_POINT('Ctrl Pts',(65.932824986936,19.6267961814968,8.14355106731984));
#38968=CARTESIAN_POINT('Ctrl Pts',(65.8473062312967,20.147295631655,8.91224678187255));
#38969=CARTESIAN_POINT('Ctrl Pts',(65.8747431444716,20.246238786796,9.72822620930753));
#38970=CARTESIAN_POINT('Ctrl Pts',(65.9021800576464,20.345181941937,10.5442056367425));
#38971=CARTESIAN_POINT('Ctrl Pts',(66.0425726396353,20.0225688020609,11.4074687770597));
#38972=CARTESIAN_POINT('Ctrl Pts',(66.2558562834075,19.4279225161918,11.9340732703408));
#38973=CARTESIAN_POINT('Ctrl Pts',(66.4691399271798,18.8332762303227,12.4606777636219));
#38974=CARTESIAN_POINT('Ctrl Pts',(66.7553146327353,17.9665967984606,12.6506236098669));
#38975=CARTESIAN_POINT('Ctrl Pts',(67.0094701965008,17.2194144305738,12.4192427536871));
#38976=CARTESIAN_POINT('Ctrl Pts',(67.2636257602663,16.472232062687,12.1878618975073));
#38977=CARTESIAN_POINT('Ctrl Pts',(67.4857621822417,15.8445467587755,11.5351543389028));
#38978=CARTESIAN_POINT('Ctrl Pts',(67.5994444228594,15.6216179699845,10.7518245719412));
#38979=CARTESIAN_POINT('Ctrl Pts',(67.6344914472383,15.5528913979793,10.5103323450966));
#38980=CARTESIAN_POINT('Ctrl Pts',(67.6592307340631,15.5226338262371,10.2564254798708));
#38981=CARTESIAN_POINT('Ctrl Pts',(67.6742507328171,15.5286491313886,10.0019962882659));
#38982=CARTESIAN_POINT('Ctrl Pts',(59.6819508576139,16.8135320242449,7.0307770462544));
#38983=CARTESIAN_POINT('Ctrl Pts',(59.6574023990872,16.905148118714,7.06547285383208));
#38984=CARTESIAN_POINT('Ctrl Pts',(59.633381623744,16.9947948727323,7.10515219318508));
#38985=CARTESIAN_POINT('Ctrl Pts',(59.6099513655634,17.0822377866965,7.14949694327549));
#38986=CARTESIAN_POINT('Ctrl Pts',(59.5861978454406,17.1708871306533,7.1944535077954));
#38987=CARTESIAN_POINT('Ctrl Pts',(59.5630510759273,17.2572720505083,7.24420580541868));
#38988=CARTESIAN_POINT('Ctrl Pts',(59.540585329437,17.3411153578402,7.2984630034136));
#38989=CARTESIAN_POINT('Ctrl Pts',(59.5341747454294,17.3650399830626,7.31394525440008));
#38990=CARTESIAN_POINT('Ctrl Pts',(59.5278196764501,17.3887574233789,7.32979452699793));
#38991=CARTESIAN_POINT('Ctrl Pts',(59.5215220078066,17.4122606427255,7.34600453501649));
#38992=CARTESIAN_POINT('Ctrl Pts',(59.5165727272894,17.4307316090769,7.358743832908));
#38993=CARTESIAN_POINT('Ctrl Pts',(59.5116584066524,17.4490721033785,7.37170741276992));
#38994=CARTESIAN_POINT('Ctrl Pts',(59.5067848207907,17.4672605734295,7.38487881885917));
#38995=CARTESIAN_POINT('Ctrl Pts',(59.4853806969507,17.547141851092,7.44272583645177));
#38996=CARTESIAN_POINT('Ctrl Pts',(59.4647409044082,17.6241706055182,7.50463022489488));
#38997=CARTESIAN_POINT('Ctrl Pts',(59.4449347986959,17.6980879983368,7.57029723790349));
#38998=CARTESIAN_POINT('Ctrl Pts',(59.4299001526504,17.7541980612524,7.62014450782053));
#38999=CARTESIAN_POINT('Ctrl Pts',(59.4153460633656,17.8085146619212,7.6721607780437));
#39000=CARTESIAN_POINT('Ctrl Pts',(59.401307177695,17.8609084965252,7.7262283086775));
#39001=CARTESIAN_POINT('Ctrl Pts',(59.3940669983074,17.8879292138559,7.75411218992159));
#39002=CARTESIAN_POINT('Ctrl Pts',(59.3869639127158,17.9144382901743,7.78254177971635));
#39003=CARTESIAN_POINT('Ctrl Pts',(59.3800031152495,17.9404163399798,7.81150163907493));
#39004=CARTESIAN_POINT('Ctrl Pts',(59.377069260484,17.9513656350265,7.82370771485813));
#39005=CARTESIAN_POINT('Ctrl Pts',(59.3741603923946,17.9622216785285,7.83600935578381));
#39006=CARTESIAN_POINT('Ctrl Pts',(59.3712797968968,17.9729722072825,7.84839276353972));
#39007=CARTESIAN_POINT('Ctrl Pts',(59.3542405470275,18.0365635535174,7.92164288808634));
#39008=CARTESIAN_POINT('Ctrl Pts',(59.338167291009,18.0965497616217,7.99784282404939));
#39009=CARTESIAN_POINT('Ctrl Pts',(59.3231234327018,18.152694205166,8.07671631200185));
#39010=CARTESIAN_POINT('Ctrl Pts',(59.3083518044045,18.2078226724821,8.15416252445319));
#39011=CARTESIAN_POINT('Ctrl Pts',(59.2945725637949,18.259247498527,8.23418719385315));
#39012=CARTESIAN_POINT('Ctrl Pts',(59.2818571864781,18.3067019327104,8.31655061029));
#39013=CARTESIAN_POINT('Ctrl Pts',(59.2693830443537,18.3532560648998,8.39735143411931));
#39014=CARTESIAN_POINT('Ctrl Pts',(59.2579327073364,18.3959893044119,8.48040377661436));
#39015=CARTESIAN_POINT('Ctrl Pts',(59.2475859888077,18.4346037836527,8.56549184091671));
#39016=CARTESIAN_POINT('Ctrl Pts',(59.2424064366885,18.4539341353218,8.60808680110125));
#39017=CARTESIAN_POINT('Ctrl Pts',(59.2375036517524,18.4722315778021,8.6511920152124));
#39018=CARTESIAN_POINT('Ctrl Pts',(59.2328889291418,18.4894539570476,8.69478065069042));
#39019=CARTESIAN_POINT('Ctrl Pts',(59.2306690826426,18.4977385369678,8.71574834215067));
#39020=CARTESIAN_POINT('Ctrl Pts',(59.2285159056722,18.505774302819,8.73682789437621));
#39021=CARTESIAN_POINT('Ctrl Pts',(59.2264307309096,18.5135562809755,8.75801630674609));
#39022=CARTESIAN_POINT('Ctrl Pts',(59.2250997041795,18.5185237403585,8.77154147678875));
#39023=CARTESIAN_POINT('Ctrl Pts',(59.2237963942956,18.5233877590632,8.78511114991627));
#39024=CARTESIAN_POINT('Ctrl Pts',(59.222522397681,18.5281423791575,8.79871063713888));
#39025=CARTESIAN_POINT('Ctrl Pts',(59.2143322655506,18.5587083683889,8.88613755490554));
#39026=CARTESIAN_POINT('Ctrl Pts',(59.2073383924974,18.5848098579651,8.97493705383762));
#39027=CARTESIAN_POINT('Ctrl Pts',(59.2016063055609,18.6062022976455,9.06488740616719));
#39028=CARTESIAN_POINT('Ctrl Pts',(59.2009154354341,18.6087806600602,9.07572883477923));
#39029=CARTESIAN_POINT('Ctrl Pts',(59.200242910756,18.6112905563283,9.08658699329483));
#39030=CARTESIAN_POINT('Ctrl Pts',(59.1995888595069,18.6137315088206,9.09746150181125));
#39031=CARTESIAN_POINT('Ctrl Pts',(59.1940765541311,18.63430371255,9.18911121861839));
#39032=CARTESIAN_POINT('Ctrl Pts',(59.1898752976095,18.6499830153444,9.28192246232436));
#39033=CARTESIAN_POINT('Ctrl Pts',(59.1869573634513,18.660872893876,9.37550443036629));
#39034=CARTESIAN_POINT('Ctrl Pts',(59.1839372837924,18.6721439846059,9.47236233832445));
#39035=CARTESIAN_POINT('Ctrl Pts',(59.1822919652802,18.6782843968879,9.57004704527203));
#39036=CARTESIAN_POINT('Ctrl Pts',(59.1820051755357,18.6793547107854,9.66811274307554));
#39037=CARTESIAN_POINT('Ctrl Pts',(59.1818653628562,18.679876498809,9.7159206868577));
#39038=CARTESIAN_POINT('Ctrl Pts',(59.1820486386194,18.6791925043489,9.76381888085402));
#39039=CARTESIAN_POINT('Ctrl Pts',(59.1825542820089,18.6773054175288,9.81175333276414));
#39040=CARTESIAN_POINT('Ctrl Pts',(59.1827037214712,18.6767477018626,9.82592003378259));
#39041=CARTESIAN_POINT('Ctrl Pts',(59.1828813434833,18.6760848074891,9.84008999153942));
#39042=CARTESIAN_POINT('Ctrl Pts',(59.1830868741632,18.6753177565492,9.85424725726874));
#39043=CARTESIAN_POINT('Ctrl Pts',(59.1844353908751,18.6702850236656,9.94713513872897));
#39044=CARTESIAN_POINT('Ctrl Pts',(59.1869856678166,18.6607672605466,10.0396336499573));
#39045=CARTESIAN_POINT('Ctrl Pts',(59.1907077256037,18.6468763517762,10.1313703615392));
#39046=CARTESIAN_POINT('Ctrl Pts',(59.1944191075896,18.6330252856387,10.2228439490746));
#39047=CARTESIAN_POINT('Ctrl Pts',(59.1992956613142,18.6148257393727,10.3135610439828));
#39048=CARTESIAN_POINT('Ctrl Pts',(59.2053202323847,18.5923417340437,10.4031353914207));
#39049=CARTESIAN_POINT('Ctrl Pts',(59.2112410581269,18.570244911551,10.4911672356704));
#39050=CARTESIAN_POINT('Ctrl Pts',(59.2182708208297,18.544009479979,10.5780961326744));
#39051=CARTESIAN_POINT('Ctrl Pts',(59.2264037185759,18.5136570923772,10.6635263260514));
#39052=CARTESIAN_POINT('Ctrl Pts',(59.2303039432159,18.4991012558599,10.7044953577056));
#39053=CARTESIAN_POINT('Ctrl Pts',(59.2344580112977,18.4835980627207,10.7451192126333));
#39054=CARTESIAN_POINT('Ctrl Pts',(59.2388660433661,18.4671470630801,10.7853510166313));
#39055=CARTESIAN_POINT('Ctrl Pts',(59.2403491923144,18.4616118758496,10.7988876145655));
#39056=CARTESIAN_POINT('Ctrl Pts',(59.2418610961089,18.4559693740725,10.81237980913));
#39057=CARTESIAN_POINT('Ctrl Pts',(59.2434017709825,18.4502194971662,10.8258257525424));
#39058=CARTESIAN_POINT('Ctrl Pts',(59.2448672510403,18.4447502511329,10.8386154476733));
#39059=CARTESIAN_POINT('Ctrl Pts',(59.2463583030217,18.4391855693816,10.8513591684399));
#39060=CARTESIAN_POINT('Ctrl Pts',(59.2478738644618,18.4335294170853,10.8640470923383));
#39061=CARTESIAN_POINT('Ctrl Pts',(59.2575294211935,18.3974943887873,10.9448811421958));
#39062=CARTESIAN_POINT('Ctrl Pts',(59.2681907321678,18.357705834556,11.0235565044334));
#39063=CARTESIAN_POINT('Ctrl Pts',(59.2798413572467,18.3142251098216,11.0997253741218));
#39064=CARTESIAN_POINT('Ctrl Pts',(59.2912990837899,18.271464292223,11.1746331214818));
#39065=CARTESIAN_POINT('Ctrl Pts',(59.3037137501258,18.2251321266983,11.247117361503));
#39066=CARTESIAN_POINT('Ctrl Pts',(59.3170791893599,18.1752516284115,11.3168132023689));
#39067=CARTESIAN_POINT('Ctrl Pts',(59.3300579264205,18.1268143222831,11.384492533888));
#39068=CARTESIAN_POINT('Ctrl Pts',(59.3439333262358,18.0750306251971,11.4495429421988));
#39069=CARTESIAN_POINT('Ctrl Pts',(59.3587070803994,18.0198942240399,11.5115898445996));
#39070=CARTESIAN_POINT('Ctrl Pts',(59.361378450579,18.009924534804,11.5228090812926));
#39071=CARTESIAN_POINT('Ctrl Pts',(59.3640792101803,17.9998451627528,11.5339299974755));
#39072=CARTESIAN_POINT('Ctrl Pts',(59.3668093915945,17.9896559870011,11.5449502145347));
#39073=CARTESIAN_POINT('Ctrl Pts',(59.3747124158147,17.9601614990778,11.5768503080151));
#39074=CARTESIAN_POINT('Ctrl Pts',(59.3828619650632,17.9297469672235,11.6079068412473));
#39075=CARTESIAN_POINT('Ctrl Pts',(59.3912467107623,17.8984546702662,11.6380966037226));
#39076=CARTESIAN_POINT('Ctrl Pts',(68.1281291851066,15.0750265266586,10.0024371765582));
#39077=CARTESIAN_POINT('Ctrl Pts',(68.1132191003536,15.0686010168709,10.3130580784043));
#39078=CARTESIAN_POINT('Ctrl Pts',(67.9995899840861,15.229260839257,11.6285356953996));
#39079=CARTESIAN_POINT('Ctrl Pts',(67.3992512291335,17.0050066526372,13.4679206448302));
#39080=CARTESIAN_POINT('Ctrl Pts',(66.3844685224502,20.1882099452846,12.7722321938662));
#39081=CARTESIAN_POINT('Ctrl Pts',(65.9036218913761,21.3787366757644,9.61047736356028));
#39082=CARTESIAN_POINT('Ctrl Pts',(66.2501895556748,19.4813112170046,6.79508159949543));
#39083=CARTESIAN_POINT('Ctrl Pts',(66.9814704044652,16.1481166073795,6.83122696910049));
#39084=CARTESIAN_POINT('Ctrl Pts',(67.2119040522751,14.8676525643411,8.81893895087672));
#39085=CARTESIAN_POINT('Ctrl Pts',(67.1683025391241,14.8112407741816,9.90991228406404));
#39086=CARTESIAN_POINT('Ctrl Pts',(67.1637176864735,14.810555933805,9.99855140140544));
#39087=CARTESIAN_POINT('Origin',(69.7479810832458,18.6889152049569,10.));
#39088=CARTESIAN_POINT('Ctrl Pts',(68.2083503098983,15.0969161422106,9.99673640007591));
#39089=CARTESIAN_POINT('Ctrl Pts',(68.1711103559359,15.0927295232038,10.7130675867));
#39090=CARTESIAN_POINT('Ctrl Pts',(67.9289066052253,15.6514186592595,12.4513417391717));
#39091=CARTESIAN_POINT('Ctrl Pts',(67.0483943376965,18.3902480628713,13.5944453497599));
#39092=CARTESIAN_POINT('Ctrl Pts',(66.1687987195556,21.0667649555471,11.6442225433397));
#39093=CARTESIAN_POINT('Ctrl Pts',(66.036013638459,20.9561469803459,8.22016494780576));
#39094=CARTESIAN_POINT('Ctrl Pts',(66.6336669557833,18.1194957904382,6.39071567224367));
#39095=CARTESIAN_POINT('Ctrl Pts',(67.2173089746449,15.4027596845032,7.6368119452057));
#39096=CARTESIAN_POINT('Ctrl Pts',(67.2747579502335,14.8518622987657,9.32892113065761));
#39097=CARTESIAN_POINT('Ctrl Pts',(67.242349320473,14.8383776097513,10.0022118830713));
#39098=CARTESIAN_POINT('Ctrl Pts',(67.8425423025985,17.244983442153,7.06170475438608));
#39099=CARTESIAN_POINT('Ctrl Pts',(68.0419164156808,16.2988495743024,7.35795147289591));
#39100=CARTESIAN_POINT('Ctrl Pts',(68.3551165744735,14.725851572522,8.97144797270223));
#39101=CARTESIAN_POINT('Ctrl Pts',(68.023655252025,15.3567034243025,12.3283366156213));
#39102=CARTESIAN_POINT('Ctrl Pts',(67.0483943376965,18.3902480628713,13.5944453497599));
#39103=CARTESIAN_POINT('Ctrl Pts',(66.1687987195556,21.0667649555471,11.6442225433397));
#39104=CARTESIAN_POINT('Ctrl Pts',(66.036013638459,20.9561469803459,8.22016494780576));
#39105=CARTESIAN_POINT('Ctrl Pts',(66.6336669557833,18.1194957904382,6.39071567224367));
#39106=CARTESIAN_POINT('Ctrl Pts',(67.2905946547074,15.0616295968133,7.79327945411721));
#39107=CARTESIAN_POINT('Ctrl Pts',(67.282863942121,14.4843023646231,11.1722569386416));
#39108=CARTESIAN_POINT('Ctrl Pts',(66.4816292855382,16.868372167434,13.5013274912989));
#39109=CARTESIAN_POINT('Ctrl Pts',(65.468753391891,20.0422978199459,12.6947822329673));
#39110=CARTESIAN_POINT('Ctrl Pts',(65.0155990043222,21.1273143736846,9.47487431060687));
#39111=CARTESIAN_POINT('Ctrl Pts',(65.3922823621304,19.1153342996381,6.72525821930946));
#39112=CARTESIAN_POINT('Ctrl Pts',(66.1257396929251,15.7718556315866,6.9083705731136));
#39113=CARTESIAN_POINT('Ctrl Pts',(66.4233986629547,14.0547985877671,9.86022990097494));
#39114=CARTESIAN_POINT('Ctrl Pts',(65.8829690009265,15.4655309000317,12.9372608391342));
#39115=CARTESIAN_POINT('Ctrl Pts',(64.852721554462,18.704288070265,13.3837942299379));
#39116=CARTESIAN_POINT('Ctrl Pts',(64.1195886430847,20.8341986998846,10.7999310727631));
#39117=CARTESIAN_POINT('Ctrl Pts',(64.2044184759422,19.9114308093214,7.49968047567758));
#39118=CARTESIAN_POINT('Ctrl Pts',(64.8955230826759,16.7260146593053,6.43862003923501));
#39119=CARTESIAN_POINT('Ctrl Pts',(65.4382581333965,14.0943212306268,8.56699487612852));
#39120=CARTESIAN_POINT('Ctrl Pts',(65.2108533475991,14.3368288007655,11.9787141005062));
#39121=CARTESIAN_POINT('Ctrl Pts',(64.2812461473764,17.199991458738,13.6183729089162));
#39122=CARTESIAN_POINT('Ctrl Pts',(63.346239485481,20.0833051820057,12.017555775347));
#39123=CARTESIAN_POINT('Ctrl Pts',(63.1074718691846,20.3682194128848,8.60989310618131));
#39124=CARTESIAN_POINT('Ctrl Pts',(63.6430568297551,17.7632104839249,6.4471568308768));
#39125=CARTESIAN_POINT('Ctrl Pts',(64.3376274439251,14.564859018057,7.46621057361501));
#39126=CARTESIAN_POINT('Ctrl Pts',(64.4334353369931,13.60112044902,10.7544289031929));
#39127=CARTESIAN_POINT('Ctrl Pts',(63.708961052588,15.6987166428558,13.3670096553836));
#39128=CARTESIAN_POINT('Ctrl Pts',(62.6772983776882,18.9427555175133,12.9642257537709));
#39129=CARTESIAN_POINT('Ctrl Pts',(62.1266472347557,20.3916349158421,9.9067950074971));
#39130=CARTESIAN_POINT('Ctrl Pts',(62.4144320750886,18.7114286257305,6.93283507366395));
#39131=CARTESIAN_POINT('Ctrl Pts',(63.1472062543101,15.3704995140598,6.70571036393744));
#39132=CARTESIAN_POINT('Ctrl Pts',(63.5330077514078,13.3244900809145,9.42882503807144));
#39133=CARTESIAN_POINT('Ctrl Pts',(63.0906099643739,14.3693624549396,12.6634621126407));
#39134=CARTESIAN_POINT('Ctrl Pts',(62.080489794707,17.5330036055456,13.5128046754735));
#39135=CARTESIAN_POINT('Ctrl Pts',(61.2715545195409,19.9458125081592,11.2162142452876));
#39136=CARTESIAN_POINT('Ctrl Pts',(61.2525379570576,19.4106046411913,7.83042882970038));
#39137=CARTESIAN_POINT('Ctrl Pts',(61.9047530097005,16.3703262829254,6.38762845988019));
#39138=CARTESIAN_POINT('Ctrl Pts',(62.5083833543796,13.5113685232517,8.17992871548476));
#39139=CARTESIAN_POINT('Ctrl Pts',(62.3871231598861,13.357739085696,11.6022164308586));
#39140=CARTESIAN_POINT('Ctrl Pts',(61.5138509672066,16.0106566332716,13.5896176377583));
#39141=CARTESIAN_POINT('Ctrl Pts',(60.5349179618126,19.0579057022675,12.3623010109723));
#39142=CARTESIAN_POINT('Ctrl Pts',(60.1913020034494,19.734119272829,9.01938609588907));
#39143=CARTESIAN_POINT('Ctrl Pts',(60.6550135466888,17.3973455890623,6.55469600728483));
#39144=CARTESIAN_POINT('Ctrl Pts',(61.3750552367845,14.1039347737162,7.1754379864716));
#39145=CARTESIAN_POINT('Ctrl Pts',(61.5708627210562,12.7669926495712,10.3258507409623));
#39146=CARTESIAN_POINT('Ctrl Pts',(60.9313710113775,14.5474295567701,13.1842383274677));
#39147=CARTESIAN_POINT('Ctrl Pts',(59.8935459365979,17.8144668208753,13.1913616605739));
#39148=CARTESIAN_POINT('Ctrl Pts',(59.2511484715134,19.6057481548832,10.3395770770156));
#39149=CARTESIAN_POINT('Ctrl Pts',(59.4436819065863,18.2810249486939,7.18539898656543));
#39150=CARTESIAN_POINT('Ctrl Pts',(60.1631753733451,14.9896601306954,6.54837069990779));
#39151=CARTESIAN_POINT('Ctrl Pts',(60.629216203114,12.6441934312551,9.0096983771865));
#39152=CARTESIAN_POINT('Ctrl Pts',(60.402326566927,13.0868379849885,11.2296927240265));
#39153=CARTESIAN_POINT('Ctrl Pts',(60.181950026368,13.707234883037,11.9973015569304));
#39154=CARTESIAN_POINT('Ctrl Pts',(67.9318278742783,17.3251900988197,7.23888518457547));
#39155=CARTESIAN_POINT('Ctrl Pts',(68.1161335763132,16.4352923065869,7.51726810226198));
#39156=CARTESIAN_POINT('Ctrl Pts',(68.4043554971943,14.9555143577762,9.03347008941797));
#39157=CARTESIAN_POINT('Ctrl Pts',(68.0837432245498,15.5458770044744,12.1879369455074));
#39158=CARTESIAN_POINT('Ctrl Pts',(67.1581527442329,18.3940490596782,13.3776987943165));
#39159=CARTESIAN_POINT('Ctrl Pts',(66.3224589027986,20.9067222911425,11.5450752374347));
#39160=CARTESIAN_POINT('Ctrl Pts',(66.1885426111956,20.800326051025,8.32748974461938));
#39161=CARTESIAN_POINT('Ctrl Pts',(66.7410189775958,18.1322775372971,6.60835702425631));
#39162=CARTESIAN_POINT('Ctrl Pts',(67.3491954556354,15.256353376944,7.92634562444538));
#39163=CARTESIAN_POINT('Ctrl Pts',(67.3327927019053,14.7113906429075,11.1015693557681));
#39164=CARTESIAN_POINT('Ctrl Pts',(66.5707346233278,16.9492514661364,13.2901959816018));
#39165=CARTESIAN_POINT('Ctrl Pts',(65.609797362651,19.9293395015267,12.5322857391188));
#39166=CARTESIAN_POINT('Ctrl Pts',(65.1748301675256,20.9464805290195,9.50653960894237));
#39167=CARTESIAN_POINT('Ctrl Pts',(65.5196611552341,19.0533751185266,6.92272651604651));
#39168=CARTESIAN_POINT('Ctrl Pts',(66.1997524963878,15.9090610352117,7.09479711845808));
#39169=CARTESIAN_POINT('Ctrl Pts',(66.470324299897,14.2930946730788,9.86865809630686));
#39170=CARTESIAN_POINT('Ctrl Pts',(65.953344565804,15.6163106628564,12.7601427840874));
#39171=CARTESIAN_POINT('Ctrl Pts',(64.9760832641982,18.6573208483792,13.1797500249766));
#39172=CARTESIAN_POINT('Ctrl Pts',(64.2780203671544,20.656348402684,10.751694895066));
#39173=CARTESIAN_POINT('Ctrl Pts',(64.3485967193296,19.7867752262122,7.65045078699728));
#39174=CARTESIAN_POINT('Ctrl Pts',(64.9888892233674,16.7909924250966,6.6533727379157));
#39175=CARTESIAN_POINT('Ctrl Pts',(65.489758917571,14.3155426340161,8.65340568344619));
#39176=CARTESIAN_POINT('Ctrl Pts',(65.2669285289691,14.5409783214077,11.8593968140379));
#39177=CARTESIAN_POINT('Ctrl Pts',(64.3842388247346,17.2290425005878,13.4001835116647));
#39178=CARTESIAN_POINT('Ctrl Pts',(63.4964752486209,19.9360426274117,11.8958963196675));
#39179=CARTESIAN_POINT('Ctrl Pts',(63.2629672129437,20.2013278361943,8.69371713231472));
#39180=CARTESIAN_POINT('Ctrl Pts',(63.7571179704186,17.7509534583573,6.66139475745697));
#39181=CARTESIAN_POINT('Ctrl Pts',(64.4006674801973,14.7430153463369,7.61899913400436));
#39182=CARTESIAN_POINT('Ctrl Pts',(64.4815599109682,13.8349420404105,10.7089365253202));
#39183=CARTESIAN_POINT('Ctrl Pts',(63.7916335220749,15.8036037329021,13.1639775672763));
#39184=CARTESIAN_POINT('Ctrl Pts',(62.8130423308994,18.8495771338669,12.7854817031124));
#39185=CARTESIAN_POINT('Ctrl Pts',(62.2864574754684,20.2086399244908,9.91241530746257));
#39186=CARTESIAN_POINT('Ctrl Pts',(62.5477505634247,18.6273022002302,7.11778639941015));
#39187=CARTESIAN_POINT('Ctrl Pts',(63.2271999473304,15.4853839339819,6.90435740451559));
#39188=CARTESIAN_POINT('Ctrl Pts',(63.5805992467218,13.5603011489528,9.46326712676861));
#39189=CARTESIAN_POINT('Ctrl Pts',(63.1557400246278,14.5397187075307,12.5028542351256));
#39190=CARTESIAN_POINT('Ctrl Pts',(62.1973923166246,17.5101424007745,13.3009810867784));
#39191=CARTESIAN_POINT('Ctrl Pts',(61.4280979699796,19.775009344088,11.1428760184691));
#39192=CARTESIAN_POINT('Ctrl Pts',(61.4010899078139,19.2696261599639,7.96125487716923));
#39193=CARTESIAN_POINT('Ctrl Pts',(62.0048379141107,16.4102292811539,6.60545597208741));
#39194=CARTESIAN_POINT('Ctrl Pts',(62.5629308906206,13.721219293131,8.28967977390788));
#39195=CARTESIAN_POINT('Ctrl Pts',(62.4398445301463,13.5744051997983,11.5056021110758));
#39196=CARTESIAN_POINT('Ctrl Pts',(61.6100928089779,16.0649021365259,13.3731621953643));
#39197=CARTESIAN_POINT('Ctrl Pts',(60.6810516662198,18.9259522392798,12.219853273637));
#39198=CARTESIAN_POINT('Ctrl Pts',(60.3490176872815,19.5589412741757,9.07851752376018));
#39199=CARTESIAN_POINT('Ctrl Pts',(60.7756290245012,17.3606274442457,6.76244927662485));
#39200=CARTESIAN_POINT('Ctrl Pts',(61.4431136936917,14.2633621012124,7.34576025527717));
#39201=CARTESIAN_POINT('Ctrl Pts',(61.6179756985622,13.0045895703814,10.306201805224));
#39202=CARTESIAN_POINT('Ctrl Pts',(61.007907399655,14.6752168136493,12.9922274267495));
#39203=CARTESIAN_POINT('Ctrl Pts',(60.0235254038855,17.7428017915754,12.9989212198951));
#39204=CARTESIAN_POINT('Ctrl Pts',(59.4107265678368,19.4236195381877,10.3191004374818));
#39205=CARTESIAN_POINT('Ctrl Pts',(59.5825119500423,18.1763291194577,7.35512060290615));
#39206=CARTESIAN_POINT('Ctrl Pts',(60.249481453992,15.0809863992776,6.75650538792376));
#39207=CARTESIAN_POINT('Ctrl Pts',(60.6782816207908,12.8745037461489,9.06941397854048));
#39208=CARTESIAN_POINT('Ctrl Pts',(60.4589813868428,13.2888242651274,11.1555417393121));
#39209=CARTESIAN_POINT('Ctrl Pts',(60.2488475749171,13.8709947795085,11.8768634390785));
#39210=CARTESIAN_POINT('Ctrl Pts',(68.0211134459581,17.4053967554863,7.41606561476487));
#39211=CARTESIAN_POINT('Ctrl Pts',(68.1903507369457,16.5717350388713,7.67658473162805));
#39212=CARTESIAN_POINT('Ctrl Pts',(68.4535944199152,15.1851771430305,9.09549220613371));
#39213=CARTESIAN_POINT('Ctrl Pts',(68.1438311970747,15.7350505846462,12.0475372753934));
#39214=CARTESIAN_POINT('Ctrl Pts',(67.2679111507693,18.397850056485,13.160952238873));
#39215=CARTESIAN_POINT('Ctrl Pts',(66.4761190860415,20.7466796267379,11.4459279315297));
#39216=CARTESIAN_POINT('Ctrl Pts',(66.3410715839322,20.6445051217041,8.43481454143301));
#39217=CARTESIAN_POINT('Ctrl Pts',(66.8483709994082,18.145059284156,6.82599837626894));
#39218=CARTESIAN_POINT('Ctrl Pts',(67.4077962565635,15.4510771570748,8.05941179477355));
#39219=CARTESIAN_POINT('Ctrl Pts',(67.3827214616896,14.9384789211918,11.0308817728947));
#39220=CARTESIAN_POINT('Ctrl Pts',(66.6598399611173,17.0301307648387,13.0790644719047));
#39221=CARTESIAN_POINT('Ctrl Pts',(65.7508413334111,19.8163811831076,12.3697892452703));
#39222=CARTESIAN_POINT('Ctrl Pts',(65.3340613307291,20.7656466843542,9.53820490727789));
#39223=CARTESIAN_POINT('Ctrl Pts',(65.6470399483378,18.9914159374152,7.12019481278355));
#39224=CARTESIAN_POINT('Ctrl Pts',(66.2737652998504,16.0462664388369,7.28122366380258));
#39225=CARTESIAN_POINT('Ctrl Pts',(66.5172499368395,14.5313907583906,9.87708629163876));
#39226=CARTESIAN_POINT('Ctrl Pts',(66.0237201306813,15.767090425681,12.5830247290407));
#39227=CARTESIAN_POINT('Ctrl Pts',(65.0994449739345,18.6103536264936,12.9757058200153));
#39228=CARTESIAN_POINT('Ctrl Pts',(64.4364520912241,20.4784981054833,10.7034587173689));
#39229=CARTESIAN_POINT('Ctrl Pts',(64.492774962717,19.6621196431031,7.80122109831696));
#39230=CARTESIAN_POINT('Ctrl Pts',(65.0822553640588,16.8559701908878,6.8681254365964));
#39231=CARTESIAN_POINT('Ctrl Pts',(65.5412597017456,14.5367640374055,8.73981649076384));
#39232=CARTESIAN_POINT('Ctrl Pts',(65.323003710339,14.7451278420499,11.7400795275695));
#39233=CARTESIAN_POINT('Ctrl Pts',(64.4872315020929,17.2580935424376,13.1819941144132));
#39234=CARTESIAN_POINT('Ctrl Pts',(63.6467110117609,19.7887800728178,11.774236863988));
#39235=CARTESIAN_POINT('Ctrl Pts',(63.4184625567026,20.0344362595038,8.77754115844814));
#39236=CARTESIAN_POINT('Ctrl Pts',(63.8711791110823,17.7386964327898,6.87563268403714));
#39237=CARTESIAN_POINT('Ctrl Pts',(64.4637075164693,14.9211716746167,7.77178769439372));
#39238=CARTESIAN_POINT('Ctrl Pts',(64.5296844849434,14.068763631801,10.6634441474475));
#39239=CARTESIAN_POINT('Ctrl Pts',(63.8743059915617,15.9084908229483,12.960945479169));
#39240=CARTESIAN_POINT('Ctrl Pts',(62.9487862841108,18.7563987502206,12.6067376524539));
#39241=CARTESIAN_POINT('Ctrl Pts',(62.4462677161811,20.0256449331395,9.91803560742804));
#39242=CARTESIAN_POINT('Ctrl Pts',(62.6810690517609,18.5431757747299,7.30273772515635));
#39243=CARTESIAN_POINT('Ctrl Pts',(63.3071936403504,15.6002683539039,7.10300444509373));
#39244=CARTESIAN_POINT('Ctrl Pts',(63.6281907420359,13.7961122169911,9.49770921546578));
#39245=CARTESIAN_POINT('Ctrl Pts',(63.2208700848815,14.7100749601219,12.3422463576105));
#39246=CARTESIAN_POINT('Ctrl Pts',(62.3142948385424,17.4872811960033,13.0891574980833));
#39247=CARTESIAN_POINT('Ctrl Pts',(61.5846414204184,19.6042061800168,11.0695377916506));
#39248=CARTESIAN_POINT('Ctrl Pts',(61.5496418585701,19.1286476787366,8.0920809246381));
#39249=CARTESIAN_POINT('Ctrl Pts',(62.1049228185211,16.4501322793825,6.82328348429461));
#39250=CARTESIAN_POINT('Ctrl Pts',(62.6174784268616,13.9310700630103,8.39943083233102));
#39251=CARTESIAN_POINT('Ctrl Pts',(62.4925659004067,13.7910713139007,11.408987791293));
#39252=CARTESIAN_POINT('Ctrl Pts',(61.7063346507491,16.1191476397801,13.1567067529703));
#39253=CARTESIAN_POINT('Ctrl Pts',(60.8271853706271,18.7939987762921,12.0774055363016));
#39254=CARTESIAN_POINT('Ctrl Pts',(60.5067333711135,19.3837632755223,9.13764895163131));
#39255=CARTESIAN_POINT('Ctrl Pts',(60.8962445023137,17.3239092994291,6.97020254596486));
#39256=CARTESIAN_POINT('Ctrl Pts',(61.5111721505988,14.4227894287085,7.51608252408274));
#39257=CARTESIAN_POINT('Ctrl Pts',(61.6650886760682,13.2421864911916,10.2865528694857));
#39258=CARTESIAN_POINT('Ctrl Pts',(61.0844437879323,14.8030040705286,12.8002165260313));
#39259=CARTESIAN_POINT('Ctrl Pts',(60.1535048711732,17.6711367622755,12.8064807792163));
#39260=CARTESIAN_POINT('Ctrl Pts',(59.5703046641601,19.2414909214922,10.2986237979481));
#39261=CARTESIAN_POINT('Ctrl Pts',(59.7213419934983,18.0716332902215,7.52484221924688));
#39262=CARTESIAN_POINT('Ctrl Pts',(60.3357875346389,15.1723126678598,6.96464007593973));
#39263=CARTESIAN_POINT('Ctrl Pts',(60.7273470384677,13.1048140610428,9.12912957989445));
#39264=CARTESIAN_POINT('Ctrl Pts',(60.5156362067586,13.4908105452663,11.0813907545978));
#39265=CARTESIAN_POINT('Ctrl Pts',(60.3157451234662,14.0347546759799,11.7564253212267));
#39266=CARTESIAN_POINT('Ctrl Pts',(68.1103990176379,17.4856034121529,7.59324604495427));
#39267=CARTESIAN_POINT('Ctrl Pts',(68.2645678975782,16.7081777711558,7.83590136099412));
#39268=CARTESIAN_POINT('Ctrl Pts',(68.502833342636,15.4148399282848,9.15751432284947));
#39269=CARTESIAN_POINT('Ctrl Pts',(68.2039191695996,15.924224164818,11.9071376052795));
#39270=CARTESIAN_POINT('Ctrl Pts',(67.3776695573056,18.4016510532919,12.9442056834295));
#39271=CARTESIAN_POINT('Ctrl Pts',(66.6297792692845,20.5866369623332,11.3467806256248));
#39272=CARTESIAN_POINT('Ctrl Pts',(66.4936005566688,20.4886841923832,8.54213933824664));
#39273=CARTESIAN_POINT('Ctrl Pts',(66.9557230212208,18.1578410310149,7.04363972828156));
#39274=CARTESIAN_POINT('Ctrl Pts',(67.4663970574915,15.6458009372055,8.19247796510172));
#39275=CARTESIAN_POINT('Ctrl Pts',(67.432650221474,15.1655671994761,10.9601941900212));
#39276=CARTESIAN_POINT('Ctrl Pts',(66.7489452989068,17.1110100635411,12.8679329622076));
#39277=CARTESIAN_POINT('Ctrl Pts',(65.8918853041711,19.7034228646884,12.2072927514219));
#39278=CARTESIAN_POINT('Ctrl Pts',(65.4932924939326,20.5848128396891,9.5698702056134));
#39279=CARTESIAN_POINT('Ctrl Pts',(65.7744187414415,18.9294567563037,7.3176631095206));
#39280=CARTESIAN_POINT('Ctrl Pts',(66.3477781033131,16.1834718424621,7.46765020914705));
#39281=CARTESIAN_POINT('Ctrl Pts',(66.564175573782,14.7696868437023,9.8855144869707));
#39282=CARTESIAN_POINT('Ctrl Pts',(66.0940956955586,15.9178701885058,12.4059066739939));
#39283=CARTESIAN_POINT('Ctrl Pts',(65.2228066836707,18.5633864046078,12.7716616150541));
#39284=CARTESIAN_POINT('Ctrl Pts',(64.5948838152938,20.3006478082827,10.6552225396717));
#39285=CARTESIAN_POINT('Ctrl Pts',(64.6369532061044,19.537464059994,7.95199140963666));
#39286=CARTESIAN_POINT('Ctrl Pts',(65.1756215047502,16.9209479566792,7.08287813527709));
#39287=CARTESIAN_POINT('Ctrl Pts',(65.5927604859202,14.7579854407948,8.82622729808151));
#39288=CARTESIAN_POINT('Ctrl Pts',(65.3790788917089,14.9492773626922,11.6207622411012));
#39289=CARTESIAN_POINT('Ctrl Pts',(64.5902241794512,17.2871445842874,12.9638047171617));
#39290=CARTESIAN_POINT('Ctrl Pts',(63.7969467749009,19.6415175182239,11.6525774083085));
#39291=CARTESIAN_POINT('Ctrl Pts',(63.5739579004615,19.8675446828134,8.86136518458155));
#39292=CARTESIAN_POINT('Ctrl Pts',(63.985240251746,17.7264394072222,7.08987061061733));
#39293=CARTESIAN_POINT('Ctrl Pts',(64.5267475527414,15.0993280028965,7.92457625478306));
#39294=CARTESIAN_POINT('Ctrl Pts',(64.5778090589186,14.3025852231916,10.6179517695748));
#39295=CARTESIAN_POINT('Ctrl Pts',(63.9569784610487,16.0133779129945,12.7579133910617));
#39296=CARTESIAN_POINT('Ctrl Pts',(63.084530237322,18.6632203665742,12.4279936017954));
#39297=CARTESIAN_POINT('Ctrl Pts',(62.6060779568939,19.8426499417882,9.92365590739351));
#39298=CARTESIAN_POINT('Ctrl Pts',(62.8143875400969,18.4590493492297,7.48768905090255));
#39299=CARTESIAN_POINT('Ctrl Pts',(63.3871873333707,15.715152773826,7.30165148567187));
#39300=CARTESIAN_POINT('Ctrl Pts',(63.6757822373498,14.0319232850294,9.53215130416296));
#39301=CARTESIAN_POINT('Ctrl Pts',(63.2860001451354,14.8804312127131,12.1816384800953));
#39302=CARTESIAN_POINT('Ctrl Pts',(62.4311973604599,17.4644199912321,12.8773339093882));
#39303=CARTESIAN_POINT('Ctrl Pts',(61.7411848708572,19.4334030159456,10.9961995648321));
#39304=CARTESIAN_POINT('Ctrl Pts',(61.6981938093262,18.9876691975092,8.22290697210695));
#39305=CARTESIAN_POINT('Ctrl Pts',(62.2050077229314,16.490035277611,7.04111099650182));
#39306=CARTESIAN_POINT('Ctrl Pts',(62.6720259631025,14.1409208328896,8.50918189075416));
#39307=CARTESIAN_POINT('Ctrl Pts',(62.545287270667,14.007737428003,11.3123734715102));
#39308=CARTESIAN_POINT('Ctrl Pts',(61.8025764925203,16.1733931430344,12.9402513105764));
#39309=CARTESIAN_POINT('Ctrl Pts',(60.9733190750344,18.6620453133043,11.9349577989662));
#39310=CARTESIAN_POINT('Ctrl Pts',(60.6644490549456,19.208585276869,9.19678037950243));
#39311=CARTESIAN_POINT('Ctrl Pts',(61.016859980126,17.2871911546125,7.17795581530488));
#39312=CARTESIAN_POINT('Ctrl Pts',(61.579230607506,14.5822167562047,7.68640479288831));
#39313=CARTESIAN_POINT('Ctrl Pts',(61.7122016535742,13.4797834120018,10.2669039337474));
#39314=CARTESIAN_POINT('Ctrl Pts',(61.1609801762097,14.9307913274078,12.6082056253131));
#39315=CARTESIAN_POINT('Ctrl Pts',(60.283484338461,17.5994717329756,12.6140403385374));
#39316=CARTESIAN_POINT('Ctrl Pts',(59.7298827604835,19.0593623047967,10.2781471584144));
#39317=CARTESIAN_POINT('Ctrl Pts',(59.8601720369542,17.9669374609853,7.69456383558759));
#39318=CARTESIAN_POINT('Ctrl Pts',(60.4220936152857,15.263638936442,7.1727747639557));
#39319=CARTESIAN_POINT('Ctrl Pts',(60.7764124561445,13.3351243759366,9.18884518124842));
#39320=CARTESIAN_POINT('Ctrl Pts',(60.5722910266744,13.6927968254053,11.0072397698834));
#39321=CARTESIAN_POINT('Ctrl Pts',(60.3826426720153,14.1985145724514,11.6359872033748));
#39322=CARTESIAN_POINT('Ctrl Pts',(67.8425423025985,17.244983442153,7.06170475438608));
#39323=CARTESIAN_POINT('Ctrl Pts',(67.9363396049609,16.875980626074,7.20780006417486));
#39324=CARTESIAN_POINT('Ctrl Pts',(68.0195197262116,16.5358040823887,7.42431456480013));
#39325=CARTESIAN_POINT('Ctrl Pts',(68.150998080649,15.9848167458477,7.95780764621763));
#39326=CARTESIAN_POINT('Ctrl Pts',(68.2006822338607,15.7699411081761,8.25968161903159));
#39327=CARTESIAN_POINT('Ctrl Pts',(68.2646302810789,15.490561932004,8.88066242679754));
#39328=CARTESIAN_POINT('Ctrl Pts',(68.2826595052327,15.4103584669881,9.1849782015738));
#39329=CARTESIAN_POINT('Ctrl Pts',(68.2943569622715,15.3584337419011,9.79677072277276));
#39330=CARTESIAN_POINT('Ctrl Pts',(68.288855628865,15.3830449856443,10.0982078060303));
#39331=CARTESIAN_POINT('Ctrl Pts',(68.2546420063796,15.5341550196633,10.6858944634116));
#39332=CARTESIAN_POINT('Ctrl Pts',(68.2257386849337,15.661414646539,10.9661810334233));
#39333=CARTESIAN_POINT('Ctrl Pts',(68.1449424659489,16.0093499903205,11.4722931322537));
#39334=CARTESIAN_POINT('Ctrl Pts',(68.093295210955,16.2286900565758,11.6926718707977));
#39335=CARTESIAN_POINT('Ctrl Pts',(68.0322473001841,16.4806955947432,11.866918122357));
#39336=CARTESIAN_POINT('Ctrl Pts',(60.3826426720153,14.1985145724513,11.6359872033747));
#39337=CARTESIAN_POINT('Ctrl Pts',(60.3987291200773,14.1384791309705,11.5775783984626));
#39338=CARTESIAN_POINT('Ctrl Pts',(60.4139429451904,14.0817003626712,11.5159169743106));
#39339=CARTESIAN_POINT('Ctrl Pts',(60.4282806141769,14.0281914535512,11.4513790591422));
#39340=CARTESIAN_POINT('Ctrl Pts',(60.4429682456479,13.9733764666589,11.3852658635604));
#39341=CARTESIAN_POINT('Ctrl Pts',(60.4567365493875,13.9219924575684,11.3161335496589));
#39342=CARTESIAN_POINT('Ctrl Pts',(60.4695742653813,13.8740814492266,11.2443401959014));
#39343=CARTESIAN_POINT('Ctrl Pts',(60.4729336106476,13.8615442020125,11.2255534691022));
#39344=CARTESIAN_POINT('Ctrl Pts',(60.47622918927,13.8492449351532,11.2065843091125));
#39345=CARTESIAN_POINT('Ctrl Pts',(60.4794607015071,13.8371847672994,11.1874386951717));
#39346=CARTESIAN_POINT('Ctrl Pts',(60.482079000826,13.8274131412115,11.1719261597808));
#39347=CARTESIAN_POINT('Ctrl Pts',(60.4846553435296,13.8177980993441,11.1562969512741));
#39348=CARTESIAN_POINT('Ctrl Pts',(60.4871873136239,13.808348658309,11.1405686307327));
#39349=CARTESIAN_POINT('Ctrl Pts',(60.4994718283844,13.7625022250763,11.0642585722979));
#39350=CARTESIAN_POINT('Ctrl Pts',(60.5107256648705,13.7205023355303,10.9855425568516));
#39351=CARTESIAN_POINT('Ctrl Pts',(60.5209393771319,13.6823842424367,10.9048124959882));
#39352=CARTESIAN_POINT('Ctrl Pts',(60.5290925934109,13.6519560250385,10.8403687727283));
#39353=CARTESIAN_POINT('Ctrl Pts',(60.5365828860325,13.624001872411,10.774640568225));
#39354=CARTESIAN_POINT('Ctrl Pts',(60.5434011778913,13.5985556607734,10.7078100778602));
#39355=CARTESIAN_POINT('Ctrl Pts',(60.5456026096946,13.5903398054339,10.6862324202928));
#39356=CARTESIAN_POINT('Ctrl Pts',(60.5477339562792,13.5823855116918,10.6645397536815));
#39357=CARTESIAN_POINT('Ctrl Pts',(60.5497948181657,13.5746942704238,10.6427379461932));
#39358=CARTESIAN_POINT('Ctrl Pts',(60.5517587833252,13.5673646526643,10.6219612068108));
#39359=CARTESIAN_POINT('Ctrl Pts',(60.5536591514791,13.5602723821607,10.6010802055411));
#39360=CARTESIAN_POINT('Ctrl Pts',(60.5554929869877,13.5534284148699,10.5801302247449));
#39361=CARTESIAN_POINT('Ctrl Pts',(60.5631434154612,13.5248766271072,10.4927307121652));
#39362=CARTESIAN_POINT('Ctrl Pts',(60.5696451829914,13.5006117003455,10.4040498986825));
#39363=CARTESIAN_POINT('Ctrl Pts',(60.5749893942698,13.4806668323283,10.3144849189863));
#39364=CARTESIAN_POINT('Ctrl Pts',(60.5804161086993,13.4604140583591,10.2235372482481));
#39365=CARTESIAN_POINT('Ctrl Pts',(60.5846493808407,13.4446152716452,10.1316770968566));
#39366=CARTESIAN_POINT('Ctrl Pts',(60.5876690820151,13.4333455934388,10.0392871195015));
#39367=CARTESIAN_POINT('Ctrl Pts',(60.5906654794564,13.4221628859479,9.94761013698967));
#39368=CARTESIAN_POINT('Ctrl Pts',(60.5924670545761,13.4154393160677,9.85541054662176));
#39369=CARTESIAN_POINT('Ctrl Pts',(60.593041985977,13.4132936428687,9.76304299829284));
#39370=CARTESIAN_POINT('Ctrl Pts',(60.5933185830198,13.4122613686516,9.71860536507053));
#39371=CARTESIAN_POINT('Ctrl Pts',(60.593311080267,13.4122893693062,9.67412865761842));
#39372=CARTESIAN_POINT('Ctrl Pts',(60.5930148241964,13.4133950120139,9.62965173443852));
#39373=CARTESIAN_POINT('Ctrl Pts',(60.5929169928498,13.4137601235697,9.61496431461915));
#39374=CARTESIAN_POINT('Ctrl Pts',(60.5927876671177,13.4142427737727,9.60027687042694));
#39375=CARTESIAN_POINT('Ctrl Pts',(60.5926266609965,13.4148436567973,9.58559080097424));
#39376=CARTESIAN_POINT('Ctrl Pts',(60.592463879823,13.4154511644075,9.57074282126799));
#39377=CARTESIAN_POINT('Ctrl Pts',(60.5922688054872,13.41617919174,9.55590504938851));
#39378=CARTESIAN_POINT('Ctrl Pts',(60.5920414435162,13.4170277181673,9.54108357179352));
#39379=CARTESIAN_POINT('Ctrl Pts',(60.5905760164217,13.4224967665389,9.44555398627452));
#39380=CARTESIAN_POINT('Ctrl Pts',(60.5877696251729,13.4329703612654,9.35064220205595));
#39381=CARTESIAN_POINT('Ctrl Pts',(60.5836035771031,13.4485182643284,9.25674298398244));
#39382=CARTESIAN_POINT('Ctrl Pts',(60.5832473073999,13.4498478809622,9.24871296464536));
#39383=CARTESIAN_POINT('Ctrl Pts',(60.5828810865878,13.4512146356398,9.24069033917638));
#39384=CARTESIAN_POINT('Ctrl Pts',(60.5825048986307,13.4526185882087,9.2326753487807));
#39385=CARTESIAN_POINT('Ctrl Pts',(60.5782789204955,13.4683901533211,9.14263744743419));
#39386=CARTESIAN_POINT('Ctrl Pts',(60.5727962781625,13.4888516530674,9.05356331283375));
#39387=CARTESIAN_POINT('Ctrl Pts',(60.5661351124403,13.5137114619805,8.96568771725081));
#39388=CARTESIAN_POINT('Ctrl Pts',(60.559321511336,13.5391401674843,8.8758011598418));
#39389=CARTESIAN_POINT('Ctrl Pts',(60.5512747790317,13.5691709812787,8.78716792584701));
#39390=CARTESIAN_POINT('Ctrl Pts',(60.5420644901028,13.6035442475136,8.7000421273125));
#39391=CARTESIAN_POINT('Ctrl Pts',(60.5370098857317,13.6224082878388,8.65222750982204));
#39392=CARTESIAN_POINT('Ctrl Pts',(60.5316045998727,13.6425810892942,8.60486701434196));
#39393=CARTESIAN_POINT('Ctrl Pts',(60.5258584913738,13.664025858158,8.55800419900509));
#39394=CARTESIAN_POINT('Ctrl Pts',(60.524148933004,13.6704060168522,8.54406176854061));
#39395=CARTESIAN_POINT('Ctrl Pts',(60.5224089381384,13.6768997660958,8.53016150058375));
#39396=CARTESIAN_POINT('Ctrl Pts',(60.5206408847664,13.6834982311107,8.51632087024207));
#39397=CARTESIAN_POINT('Ctrl Pts',(60.5095968738589,13.7247150409368,8.42986642555251));
#39398=CARTESIAN_POINT('Ctrl Pts',(60.4974435460195,13.7700718779143,8.34560744572339));
#39399=CARTESIAN_POINT('Ctrl Pts',(60.4842687952566,13.8192407171385,8.26379708515597));
#39400=CARTESIAN_POINT('Ctrl Pts',(60.4708342616313,13.869379079204,8.1803735684824));
#39401=CARTESIAN_POINT('Ctrl Pts',(60.4563375465724,13.9234815563466,8.09949541069896));
#39402=CARTESIAN_POINT('Ctrl Pts',(60.4408576352497,13.9812533718997,8.02143790635972));
#39403=CARTESIAN_POINT('Ctrl Pts',(60.4252551512339,14.0394826349709,7.94276232880787));
#39404=CARTESIAN_POINT('Ctrl Pts',(60.4086537215957,14.101440013859,7.86695140824316));
#39405=CARTESIAN_POINT('Ctrl Pts',(60.3911214680452,14.1668712748806,7.79430622844769));
#39406=CARTESIAN_POINT('Ctrl Pts',(60.3818445738006,14.2014931155381,7.7558672651732));
#39407=CARTESIAN_POINT('Ctrl Pts',(60.3723068629811,14.2370883369045,7.71831504954584));
#39408=CARTESIAN_POINT('Ctrl Pts',(60.3625171760094,14.2736239460729,7.68169758919558));
#39409=CARTESIAN_POINT('Ctrl Pts',(60.3590313766341,14.2866331264466,7.66865926419253));
#39410=CARTESIAN_POINT('Ctrl Pts',(60.3555136231476,14.2997615611866,7.65573947754891));
#39411=CARTESIAN_POINT('Ctrl Pts',(60.3519642909609,14.3130078492403,7.64294048624275));
#39412=CARTESIAN_POINT('Ctrl Pts',(60.3492372904052,14.3231851538666,7.63310684583699));
#39413=CARTESIAN_POINT('Ctrl Pts',(60.3464919178874,14.3334310235887,7.62334556236901));
#39414=CARTESIAN_POINT('Ctrl Pts',(60.3437307199346,14.3437359546381,7.61366571077001));
#39415=CARTESIAN_POINT('Ctrl Pts',(60.3241830913251,14.4166886977762,7.54513815595856));
#39416=CARTESIAN_POINT('Ctrl Pts',(60.3038121512208,14.4927140812436,7.48057696383332));
#39417=CARTESIAN_POINT('Ctrl Pts',(60.2827016030933,14.5714997194312,7.42026729962752));
#39418=CARTESIAN_POINT('Ctrl Pts',(60.261564320174,14.6503851332198,7.35988125813867));
#39419=CARTESIAN_POINT('Ctrl Pts',(60.2396854082702,14.7320383440592,7.30375667536574));
#39420=CARTESIAN_POINT('Ctrl Pts',(60.217137186371,14.8161894538073,7.25220561167405));
#39421=CARTESIAN_POINT('Ctrl Pts',(60.1950163805995,14.8987454248511,7.20163173173175));
#39422=CARTESIAN_POINT('Ctrl Pts',(60.1722512295677,14.9837061251435,7.15545893497819));
#39423=CARTESIAN_POINT('Ctrl Pts',(60.1489011520715,15.0708498007199,7.11401788880129));
#39424=CARTESIAN_POINT('Ctrl Pts',(60.1416346893341,15.0979686088474,7.1011215796608));
#39425=CARTESIAN_POINT('Ctrl Pts',(60.1343115246348,15.1252990315773,7.088683816123));
#39426=CARTESIAN_POINT('Ctrl Pts',(60.1269333077644,15.1528349118068,7.0767154567206));
#39427=CARTESIAN_POINT('Ctrl Pts',(60.115868753157,15.1941283917649,7.05876741202421));
#39428=CARTESIAN_POINT('Ctrl Pts',(60.1046804027641,15.2358838838842,7.04187489341861));
#39429=CARTESIAN_POINT('Ctrl Pts',(60.0933772939441,15.2780676602837,7.02603075613024));
#39430=CARTESIAN_POINT('Ctrl Pts',(67.4086397233445,15.458048217099,10.0018117506529));
#39431=CARTESIAN_POINT('Ctrl Pts',(67.3922281881599,15.4516726940089,10.2792252787835));
#39432=CARTESIAN_POINT('Ctrl Pts',(67.364342691712,15.488118577317,10.5560719127008));
#39433=CARTESIAN_POINT('Ctrl Pts',(67.3243238737158,15.5698466331085,10.8168646145657));
#39434=CARTESIAN_POINT('Ctrl Pts',(67.2047485806183,15.8140481541644,11.5961071140833));
#39435=CARTESIAN_POINT('Ctrl Pts',(66.9768469397625,16.4625291088528,12.2320200381455));
#39436=CARTESIAN_POINT('Ctrl Pts',(66.7200527868787,17.2188383863881,12.4398697983789));
#39437=CARTESIAN_POINT('Ctrl Pts',(66.4632586339949,17.9751476639235,12.6477195586123));
#39438=CARTESIAN_POINT('Ctrl Pts',(66.177571969083,18.8392852643059,12.4275061550171));
#39439=CARTESIAN_POINT('Ctrl Pts',(65.9682965015873,19.4182523936639,11.8778290289181));
#39440=CARTESIAN_POINT('Ctrl Pts',(65.7590210340916,19.9972195230219,11.328151902819));
#39441=CARTESIAN_POINT('Ctrl Pts',(65.6261567640121,20.2910161813555,10.4490110542162));
#39442=CARTESIAN_POINT('Ctrl Pts',(65.6065790035572,20.162021829958,9.63407278056602));
#39443=CARTESIAN_POINT('Ctrl Pts',(65.5870012431022,20.0330274785606,8.81913450691581));
#39444=CARTESIAN_POINT('Ctrl Pts',(65.6807099922719,19.4812421174321,8.0683988082182));
#39445=CARTESIAN_POINT('Ctrl Pts',(65.8231242605019,18.747685284561,7.71802880880715));
#39446=CARTESIAN_POINT('Ctrl Pts',(65.965538528732,18.0141284516898,7.36765880939609));
#39447=CARTESIAN_POINT('Ctrl Pts',(66.1566583160225,17.0988001470759,7.41765450927157));
#39448=CARTESIAN_POINT('Ctrl Pts',(66.288284454746,16.4055051616424,7.84562973884659));
#39449=CARTESIAN_POINT('Ctrl Pts',(66.4199105934694,15.7122101762088,8.2736049684216));
#39450=CARTESIAN_POINT('Ctrl Pts',(66.4920430836257,15.2409485099556,9.07955972769615));
#39451=CARTESIAN_POINT('Ctrl Pts',(66.4497626823333,15.1966815676295,9.90260247183729));
#39452=CARTESIAN_POINT('Ctrl Pts',(66.4481055265245,15.194946550497,9.93486115488336));
#39453=CARTESIAN_POINT('Ctrl Pts',(66.4462726093384,15.1938674837542,9.96714608853559));
#39454=CARTESIAN_POINT('Ctrl Pts',(66.4442667934687,15.1934336836835,9.99943462192776));
#39455=CARTESIAN_POINT('Origin',(63.7511045350785,17.0820569767664,10.));
#39456=CARTESIAN_POINT('Origin',(59.8874012299222,16.0467807963563,10.));
#39457=CARTESIAN_POINT('Origin',(32.5,-56.2916512459885,7.));
#39458=CARTESIAN_POINT('Ctrl Pts',(33.0411029802559,-57.8673300091754,7.));
#39459=CARTESIAN_POINT('Ctrl Pts',(32.9847118979684,-57.8942994847502,7.));
#39460=CARTESIAN_POINT('Ctrl Pts',(32.926851576823,-57.9177556703938,7.));
#39461=CARTESIAN_POINT('Ctrl Pts',(32.8678400671121,-57.9378112590822,7.));
#39462=CARTESIAN_POINT('Ctrl Pts',(32.8304073365834,-57.9505331069156,7.));
#39463=CARTESIAN_POINT('Ctrl Pts',(32.7925106111617,-57.9618858706107,7.));
#39464=CARTESIAN_POINT('Ctrl Pts',(32.7542246213985,-57.9718900412709,7.));
#39465=CARTESIAN_POINT('Ctrl Pts',(32.7280436563274,-57.9787311558468,7.));
#39466=CARTESIAN_POINT('Ctrl Pts',(32.701680564454,-57.9849415097954,7.));
#39467=CARTESIAN_POINT('Ctrl Pts',(32.6751582392643,-57.9905258833636,7.));
#39468=CARTESIAN_POINT('Ctrl Pts',(32.6611164412593,-57.9934824358178,7.));
#39469=CARTESIAN_POINT('Ctrl Pts',(32.6470302109915,-57.9962633359852,7.));
#39470=CARTESIAN_POINT('Ctrl Pts',(32.6329169442101,-57.9988669117463,7.));
#39471=CARTESIAN_POINT('Ctrl Pts',(32.5680410961479,-58.010835025728,7.));
#39472=CARTESIAN_POINT('Ctrl Pts',(32.5025225397611,-58.0190759833501,7.));
#39473=CARTESIAN_POINT('Ctrl Pts',(32.4367003115489,-58.0236879112333,7.));
#39474=CARTESIAN_POINT('Ctrl Pts',(32.3892242862367,-58.0270143863598,7.));
#39475=CARTESIAN_POINT('Ctrl Pts',(32.3415895125008,-58.028451944497,7.));
#39476=CARTESIAN_POINT('Ctrl Pts',(32.2939162953792,-58.0280221779963,7.));
#39477=CARTESIAN_POINT('Ctrl Pts',(32.2808248417186,-58.0279041606153,7.));
#39478=CARTESIAN_POINT('Ctrl Pts',(32.2677304665503,-58.0276452537954,7.));
#39479=CARTESIAN_POINT('Ctrl Pts',(32.2546356186087,-58.0272457331356,7.));
#39480=CARTESIAN_POINT('Ctrl Pts',(32.2413147456947,-58.0268393165083,7.));
#39481=CARTESIAN_POINT('Ctrl Pts',(32.2280015696053,-58.0262876036841,7.));
#39482=CARTESIAN_POINT('Ctrl Pts',(32.2147036648802,-58.0255917126622,7.));
#39483=CARTESIAN_POINT('Ctrl Pts',(32.1469436447844,-58.0220457713574,7.));
#39484=CARTESIAN_POINT('Ctrl Pts',(32.079541568506,-58.014758960148,7.));
#39485=CARTESIAN_POINT('Ctrl Pts',(32.0128409971697,-58.0038315324587,7.));
#39486=CARTESIAN_POINT('Ctrl Pts',(31.9451753892729,-57.992746004666,7.));
#39487=CARTESIAN_POINT('Ctrl Pts',(31.8782306837704,-57.9779139314693,7.));
#39488=CARTESIAN_POINT('Ctrl Pts',(31.8123515210902,-57.9593890229558,7.));
#39489=CARTESIAN_POINT('Ctrl Pts',(31.7715359667913,-57.9479118824071,7.));
#39490=CARTESIAN_POINT('Ctrl Pts',(31.7311291966112,-57.9350162530871,7.));
#39491=CARTESIAN_POINT('Ctrl Pts',(31.6912132914401,-57.9207048672865,7.));
#39492=CARTESIAN_POINT('Ctrl Pts',(31.6585126282316,-57.9089804229803,7.));
#39493=CARTESIAN_POINT('Ctrl Pts',(31.6261413907848,-57.8963056503894,7.));
#39494=CARTESIAN_POINT('Ctrl Pts',(31.5941456454821,-57.8826781573685,7.));
#39495=CARTESIAN_POINT('Ctrl Pts',(31.5810720086376,-57.8771098890512,7.));
#39496=CARTESIAN_POINT('Ctrl Pts',(31.5680588096177,-57.871381337824,7.));
#39497=CARTESIAN_POINT('Ctrl Pts',(31.5551310605861,-57.8655025242476,7.));
#39498=CARTESIAN_POINT('Ctrl Pts',(31.490968379375,-57.8363249434884,7.));
#39499=CARTESIAN_POINT('Ctrl Pts',(31.4287956226581,-57.803402900412,7.));
#39500=CARTESIAN_POINT('Ctrl Pts',(31.3689686687732,-57.7668089348842,7.));
#39501=CARTESIAN_POINT('Ctrl Pts',(31.3623206919839,-57.7627426099644,7.));
#39502=CARTESIAN_POINT('Ctrl Pts',(31.3557016803175,-57.7586308923568,7.));
#39503=CARTESIAN_POINT('Ctrl Pts',(31.3491121238469,-57.7544738418221,7.));
#39504=CARTESIAN_POINT('Ctrl Pts',(31.2920857291914,-57.7184984912118,7.));
#39505=CARTESIAN_POINT('Ctrl Pts',(31.2372638568357,-57.6791321880063,7.));
#39506=CARTESIAN_POINT('Ctrl Pts',(31.1847406170453,-57.6367028360903,7.));
#39507=CARTESIAN_POINT('Ctrl Pts',(31.1282350066813,-57.591056443428,7.));
#39508=CARTESIAN_POINT('Ctrl Pts',(31.0743888197088,-57.5418647466871,7.));
#39509=CARTESIAN_POINT('Ctrl Pts',(31.0233480125428,-57.4894785917789,7.));
#39510=CARTESIAN_POINT('Ctrl Pts',(31.0140057592583,-57.4798900927929,7.));
#39511=CARTESIAN_POINT('Ctrl Pts',(31.0047575885043,-57.4701944343076,7.));
#39512=CARTESIAN_POINT('Ctrl Pts',(30.9956045330475,-57.4603935892201,7.));
#39513=CARTESIAN_POINT('Ctrl Pts',(30.9877334105821,-57.4519654034288,7.));
#39514=CARTESIAN_POINT('Ctrl Pts',(30.9799390127843,-57.4434662551244,7.));
#39515=CARTESIAN_POINT('Ctrl Pts',(30.972222708447,-57.4348989264989,7.));
#39516=CARTESIAN_POINT('Ctrl Pts',(30.9246610658009,-57.3820917529218,7.));
#39517=CARTESIAN_POINT('Ctrl Pts',(30.8800520830315,-57.326684922902,7.));
#39518=CARTESIAN_POINT('Ctrl Pts',(30.8384919344894,-57.2690469053851,7.));
#39519=CARTESIAN_POINT('Ctrl Pts',(30.7960555285534,-57.2101936434387,7.));
#39520=CARTESIAN_POINT('Ctrl Pts',(30.7567972003304,-57.1490134679121,7.));
#39521=CARTESIAN_POINT('Ctrl Pts',(30.7208469686892,-57.0858509476833,7.));
#39522=CARTESIAN_POINT('Ctrl Pts',(30.6846788710275,-57.0223056491995,7.));
#39523=CARTESIAN_POINT('Ctrl Pts',(30.6518584168246,-56.9567530680472,7.));
#39524=CARTESIAN_POINT('Ctrl Pts',(30.6225557950443,-56.8895077659752,7.));
#39525=CARTESIAN_POINT('Ctrl Pts',(30.61531398285,-56.8728888486576,7.));
#39526=CARTESIAN_POINT('Ctrl Pts',(30.6082872384635,-56.8561664060562,7.));
#39527=CARTESIAN_POINT('Ctrl Pts',(30.601478558356,-56.8393449408623,7.));
#39528=CARTESIAN_POINT('Ctrl Pts',(30.5961524552616,-56.8261863173984,7.));
#39529=CARTESIAN_POINT('Ctrl Pts',(30.5909593217401,-56.8129655378888,7.));
#39530=CARTESIAN_POINT('Ctrl Pts',(30.5859080296146,-56.7997050116615,7.));
#39531=CARTESIAN_POINT('Ctrl Pts',(30.5590883753464,-56.7292987235297,7.));
#39532=CARTESIAN_POINT('Ctrl Pts',(30.5362121102666,-56.6576494456512,7.));
#39533=CARTESIAN_POINT('Ctrl Pts',(30.5174063251175,-56.5851265992832,7.));
#39534=CARTESIAN_POINT('Ctrl Pts',(30.4985800832282,-56.512524863307,7.));
#39535=CARTESIAN_POINT('Ctrl Pts',(30.4838325489478,-56.4390467231888,7.));
#39536=CARTESIAN_POINT('Ctrl Pts',(30.4733321890522,-56.3650308463661,7.));
#39537=CARTESIAN_POINT('Ctrl Pts',(30.463070824065,-56.2926996182489,7.));
#39538=CARTESIAN_POINT('Ctrl Pts',(30.456865076811,-56.219853902728,7.));
#39539=CARTESIAN_POINT('Ctrl Pts',(30.4549187470152,-56.1467933164485,7.));
#39540=CARTESIAN_POINT('Ctrl Pts',(30.4545002099162,-56.1310824302986,7.));
#39541=CARTESIAN_POINT('Ctrl Pts',(30.4542788241661,-56.1153615760887,7.));
#39542=CARTESIAN_POINT('Ctrl Pts',(30.4542569357502,-56.0996336954518,7.));
#39543=CARTESIAN_POINT('Ctrl Pts',(30.4542384011808,-56.0863157149705,7.));
#39544=CARTESIAN_POINT('Ctrl Pts',(30.454362914285,-56.0729926961468,7.));
#39545=CARTESIAN_POINT('Ctrl Pts',(30.4546294175093,-56.0596661744469,7.));
#39546=CARTESIAN_POINT('Ctrl Pts',(30.8457462639859,-55.0728640868079,7.));
#39547=CARTESIAN_POINT('Ctrl Pts',(30.8954489009101,-55.0171697369459,7.));
#39548=CARTESIAN_POINT('Ctrl Pts',(30.9483278083151,-54.9645336576406,7.));
#39549=CARTESIAN_POINT('Ctrl Pts',(31.0040355064375,-54.9150549466841,7.));
#39550=CARTESIAN_POINT('Ctrl Pts',(31.0582842091666,-54.8668720927416,7.));
#39551=CARTESIAN_POINT('Ctrl Pts',(31.1152164855574,-54.8216833321804,7.));
#39552=CARTESIAN_POINT('Ctrl Pts',(31.1745316088326,-54.7796213191208,7.));
#39553=CARTESIAN_POINT('Ctrl Pts',(31.1877704598448,-54.7702332795547,7.));
#39554=CARTESIAN_POINT('Ctrl Pts',(31.2011298591295,-54.7609999648588,7.));
#39555=CARTESIAN_POINT('Ctrl Pts',(31.2146007862069,-54.751926999635,7.));
#39556=CARTESIAN_POINT('Ctrl Pts',(31.2764177227105,-54.710291935328,7.));
#39557=CARTESIAN_POINT('Ctrl Pts',(31.3404582876332,-54.6721113383667,7.));
#39558=CARTESIAN_POINT('Ctrl Pts',(31.4063841811862,-54.6375086613779,7.));
#39559=CARTESIAN_POINT('Ctrl Pts',(31.4526685058674,-54.6132153002982,7.));
#39560=CARTESIAN_POINT('Ctrl Pts',(31.4998826441907,-54.5906864700306,7.));
#39561=CARTESIAN_POINT('Ctrl Pts',(31.5479126485799,-54.5699799289933,7.));
#39562=CARTESIAN_POINT('Ctrl Pts',(31.5661734302878,-54.5621073995064,7.));
#39563=CARTESIAN_POINT('Ctrl Pts',(31.5845521531086,-54.5544984112208,7.));
#39564=CARTESIAN_POINT('Ctrl Pts',(31.6030425567498,-54.5471566321368,7.));
#39565=CARTESIAN_POINT('Ctrl Pts',(31.6206506674855,-54.5401651752915,7.));
#39566=CARTESIAN_POINT('Ctrl Pts',(31.6383657020183,-54.533414128645,7.));
#39567=CARTESIAN_POINT('Ctrl Pts',(31.6561506796624,-54.526917958604,7.));
#39568=CARTESIAN_POINT('Ctrl Pts',(31.7243409101195,-54.502010683428,7.));
#39569=CARTESIAN_POINT('Ctrl Pts',(31.7936290797769,-54.4808156487355,7.));
#39570=CARTESIAN_POINT('Ctrl Pts',(31.8637026768779,-54.4634492156365,7.));
#39571=CARTESIAN_POINT('Ctrl Pts',(31.9322713952984,-54.4464557386294,7.));
#39572=CARTESIAN_POINT('Ctrl Pts',(32.0015931052551,-54.433128170902,7.));
#39573=CARTESIAN_POINT('Ctrl Pts',(32.0713763152269,-54.4236245382735,7.));
#39574=CARTESIAN_POINT('Ctrl Pts',(32.139629084154,-54.4143293332804,7.));
#39575=CARTESIAN_POINT('Ctrl Pts',(32.2083241022735,-54.4086921780743,7.));
#39576=CARTESIAN_POINT('Ctrl Pts',(32.277177509568,-54.4069083838669,7.));
#39577=CARTESIAN_POINT('Ctrl Pts',(32.2995513062292,-54.4063287429972,7.));
#39578=CARTESIAN_POINT('Ctrl Pts',(32.321941690546,-54.4061563640029,7.));
#39579=CARTESIAN_POINT('Ctrl Pts',(32.3443384586624,-54.406399061125,7.));
#39580=CARTESIAN_POINT('Ctrl Pts',(32.3569726508651,-54.4065359684712,7.));
#39581=CARTESIAN_POINT('Ctrl Pts',(32.3696101792394,-54.4068051101149,7.));
#39582=CARTESIAN_POINT('Ctrl Pts',(32.3822313254191,-54.4072071047832,7.));
#39583=CARTESIAN_POINT('Ctrl Pts',(32.4504997772513,-54.4093815153527,7.));
#39584=CARTESIAN_POINT('Ctrl Pts',(32.5184090639295,-54.4154389583228,7.));
#39585=CARTESIAN_POINT('Ctrl Pts',(32.5856896940916,-54.4255188703989,7.));
#39586=CARTESIAN_POINT('Ctrl Pts',(32.5954003979292,-54.4269737176655,7.));
#39587=CARTESIAN_POINT('Ctrl Pts',(32.6050979865285,-54.428512445765,7.));
#39588=CARTESIAN_POINT('Ctrl Pts',(32.6147816267371,-54.4301355621263,7.));
#39589=CARTESIAN_POINT('Ctrl Pts',(32.6832009663072,-54.4416036203246,7.));
#39590=CARTESIAN_POINT('Ctrl Pts',(32.7509260353084,-54.4572806254719,7.));
#39591=CARTESIAN_POINT('Ctrl Pts',(32.8176612516359,-54.4769468185459,7.));
#39592=CARTESIAN_POINT('Ctrl Pts',(32.8799198172925,-54.4952937879587,7.));
#39593=CARTESIAN_POINT('Ctrl Pts',(32.9413172465801,-54.5171136895536,7.));
#39594=CARTESIAN_POINT('Ctrl Pts',(33.0015881176757,-54.5422590913504,7.));
#39595=CARTESIAN_POINT('Ctrl Pts',(33.0148899910938,-54.5478087199798,7.));
#39596=CARTESIAN_POINT('Ctrl Pts',(33.0281368751359,-54.553520427398,7.));
#39597=CARTESIAN_POINT('Ctrl Pts',(33.0413257086146,-54.5593927822714,7.));
#39598=CARTESIAN_POINT('Ctrl Pts',(33.0516354979594,-54.563983236901,7.));
#39599=CARTESIAN_POINT('Ctrl Pts',(33.0619091366608,-54.5686716446485,7.));
#39600=CARTESIAN_POINT('Ctrl Pts',(33.0721334452454,-54.5734515734014,7.));
#39601=CARTESIAN_POINT('Ctrl Pts',(33.13407312627,-54.6024087649643,7.));
#39602=CARTESIAN_POINT('Ctrl Pts',(33.1943201438224,-54.6347718932536,7.));
#39603=CARTESIAN_POINT('Ctrl Pts',(33.2526025547429,-54.6703158299708,7.));
#39604=CARTESIAN_POINT('Ctrl Pts',(33.3106158338357,-54.7056956347569,7.));
#39605=CARTESIAN_POINT('Ctrl Pts',(33.36668338626,-54.7442277671426,7.));
#39606=CARTESIAN_POINT('Ctrl Pts',(33.420501371871,-54.7857268573679,7.));
#39607=CARTESIAN_POINT('Ctrl Pts',(33.4731665001685,-54.8263369784294,7.));
#39608=CARTESIAN_POINT('Ctrl Pts',(33.5236779674717,-54.8697891009245,7.));
#39609=CARTESIAN_POINT('Ctrl Pts',(33.5717071750085,-54.9159326392378,7.));
#39610=CARTESIAN_POINT('Ctrl Pts',(33.5818268624642,-54.9256550188018,7.));
#39611=CARTESIAN_POINT('Ctrl Pts',(33.5918361778029,-54.935496940484,7.));
#39612=CARTESIAN_POINT('Ctrl Pts',(33.6017317564147,-54.9454570805868,7.));
#39613=CARTESIAN_POINT('Ctrl Pts',(33.6111117333405,-54.9548982550757,7.));
#39614=CARTESIAN_POINT('Ctrl Pts',(33.6203906592327,-54.9644470263966,7.));
#39615=CARTESIAN_POINT('Ctrl Pts',(33.6295510505887,-54.9740864762536,7.));
#39616=CARTESIAN_POINT('Ctrl Pts',(33.6745642996402,-55.0214537709762,7.));
#39617=CARTESIAN_POINT('Ctrl Pts',(33.716801866203,-55.0710902388509,7.));
#39618=CARTESIAN_POINT('Ctrl Pts',(33.7559956009587,-55.1228219103356,7.));
#39619=CARTESIAN_POINT('Ctrl Pts',(33.794443925836,-55.1735697179659,7.));
#39620=CARTESIAN_POINT('Ctrl Pts',(33.8299635740397,-55.2263345331734,7.));
#39621=CARTESIAN_POINT('Ctrl Pts',(33.8622555275508,-55.2809712643406,7.));
#39622=CARTESIAN_POINT('Ctrl Pts',(33.8934985744639,-55.3338332862821,7.));
#39623=CARTESIAN_POINT('Ctrl Pts',(33.921720456862,-55.3884482094617,7.));
#39624=CARTESIAN_POINT('Ctrl Pts',(33.9466019284157,-55.4446928633988,7.));
#39625=CARTESIAN_POINT('Ctrl Pts',(33.9507443558517,-55.4540568351838,7.));
#39626=CARTESIAN_POINT('Ctrl Pts',(33.9547940777726,-55.4634659867188,7.));
#39627=CARTESIAN_POINT('Ctrl Pts',(33.9587494776695,-55.4729197548336,7.));
#39628=CARTESIAN_POINT('Ctrl Pts',(33.9629351903496,-55.4829239915992,7.));
#39629=CARTESIAN_POINT('Ctrl Pts',(33.9670152760995,-55.4929781929138,7.));
#39630=CARTESIAN_POINT('Ctrl Pts',(33.9709895856635,-55.5030806790321,7.));
#39631=CARTESIAN_POINT('Origin',(32.5,-56.2916512459885,-3.54592528053767));
#39632=CARTESIAN_POINT('Ctrl Pts',(33.5295805874755,-58.0719425970214,-1.79592528053768));
#39633=CARTESIAN_POINT('Ctrl Pts',(33.6151116017801,-58.0235064542129,-1.79058130531689));
#39634=CARTESIAN_POINT('Ctrl Pts',(34.2640553995263,-57.5898394701863,-1.74819136657341));
#39635=CARTESIAN_POINT('Ctrl Pts',(34.9180311095446,-56.062943931961,-1.66875546430726));
#39636=CARTESIAN_POINT('Ctrl Pts',(33.6191501107478,-54.1363165628765,-1.55761757373922));
#39637=CARTESIAN_POINT('Ctrl Pts',(31.2961996587745,-54.182342369509,-1.44647968317117));
#39638=CARTESIAN_POINT('Ctrl Pts',(30.0749499288325,-56.1591174155133,-1.33534179260313));
#39639=CARTESIAN_POINT('Ctrl Pts',(31.0734520820822,-58.2571645498346,-1.22420390203509));
#39640=CARTESIAN_POINT('Ctrl Pts',(32.7280434754779,-58.4718761792197,-1.14439839801327));
#39641=CARTESIAN_POINT('Ctrl Pts',(33.436201766478,-58.1266820552905,-1.10163885751414));
#39642=CARTESIAN_POINT('Ctrl Pts',(33.5268019957928,-58.0733321975144,-1.09592528053768));
#39643=CARTESIAN_POINT('Ctrl Pts',(33.5243188290626,-58.0704843676252,-1.85407471946232));
#39644=CARTESIAN_POINT('Ctrl Pts',(33.9297573522988,-57.832304408809,-1.82862455259619));
#39645=CARTESIAN_POINT('Ctrl Pts',(34.7395102025176,-56.9114816531044,-1.76612842220737));
#39646=CARTESIAN_POINT('Ctrl Pts',(34.4535014835806,-54.8495668967865,-1.66658632829587));
#39647=CARTESIAN_POINT('Ctrl Pts',(32.3487507516394,-53.8677941230741,-1.55544843772784));
#39648=CARTESIAN_POINT('Ctrl Pts',(30.3811218874152,-55.1044118987674,-1.44431054715979));
#39649=CARTESIAN_POINT('Ctrl Pts',(30.3535878576004,-57.4278205885651,-1.33317265659175));
#39650=CARTESIAN_POINT('Ctrl Pts',(32.0395408012641,-58.5450270011375,-1.2364273806926));
#39651=CARTESIAN_POINT('Ctrl Pts',(33.1630292684131,-58.2758908569843,-1.17672806831612));
#39652=CARTESIAN_POINT('Ctrl Pts',(33.5270487244507,-58.0682282925651,-1.15407471946232));
#39653=CARTESIAN_POINT('Ctrl Pts',(32.8002165734083,-54.6529242983091,-2.));
#39654=CARTESIAN_POINT('Ctrl Pts',(32.2553008763614,-54.5530951452,-1.96295403647732));
#39655=CARTESIAN_POINT('Ctrl Pts',(31.067360018651,-54.9418786009696,-1.88886210943196));
#39656=CARTESIAN_POINT('Ctrl Pts',(30.5876880485777,-56.7662967044641,-1.77772421886392));
#39657=CARTESIAN_POINT('Ctrl Pts',(31.862316082722,-58.1542462926904,-1.66658632829588));
#39658=CARTESIAN_POINT('Ctrl Pts',(33.7186881749666,-57.8383051703362,-1.55544843772784));
#39659=CARTESIAN_POINT('Ctrl Pts',(34.4605498617843,-56.1062143874073,-1.44431054715979));
#39660=CARTESIAN_POINT('Ctrl Pts',(33.4074116483785,-54.5440967590365,-1.33317265659175));
#39661=CARTESIAN_POINT('Ctrl Pts',(31.5239535863333,-54.5814146779316,-1.22203476602371));
#39662=CARTESIAN_POINT('Ctrl Pts',(30.5337591344129,-56.1841922550787,-1.11089687545567));
#39663=CARTESIAN_POINT('Ctrl Pts',(31.3433489080176,-57.8852977549106,-0.999758984887625));
#39664=CARTESIAN_POINT('Ctrl Pts',(33.2116035654679,-58.127735859695,-0.888621094319584));
#39665=CARTESIAN_POINT('Ctrl Pts',(34.4285349719857,-56.6895771946011,-0.777483203751541));
#39666=CARTESIAN_POINT('Ctrl Pts',(33.8802486292119,-54.8871962644418,-0.6663453131835));
#39667=CARTESIAN_POINT('Ctrl Pts',(32.068608990815,-54.3703269630488,-0.555207422615458));
#39668=CARTESIAN_POINT('Ctrl Pts',(30.6518244621987,-55.6120685434763,-0.444069532047416));
#39669=CARTESIAN_POINT('Ctrl Pts',(30.9266969543788,-57.4758393880095,-0.332931641479375));
#39670=CARTESIAN_POINT('Ctrl Pts',(32.6416310686724,-58.2557096429587,-0.221793750911333));
#39671=CARTESIAN_POINT('Ctrl Pts',(34.2269289097961,-57.2378548494304,-0.110655860343291));
#39672=CARTESIAN_POINT('Ctrl Pts',(34.2315490093866,-55.3539292291843,0.000482030224750882));
#39673=CARTESIAN_POINT('Ctrl Pts',(32.6512627267286,-54.3283111741666,0.111619920792793));
#39674=CARTESIAN_POINT('Ctrl Pts',(30.9325239231375,-55.0997605683743,0.222757811360835));
#39675=CARTESIAN_POINT('Ctrl Pts',(30.648513765023,-56.9621610088766,0.333895701928876));
#39676=CARTESIAN_POINT('Ctrl Pts',(32.0591899470587,-58.210836263271,0.445033592496918));
#39677=CARTESIAN_POINT('Ctrl Pts',(33.8733445736997,-57.7028597043182,0.556171483064959));
#39678=CARTESIAN_POINT('Ctrl Pts',(34.4304613352259,-55.9031880402636,0.667309373633002));
#39679=CARTESIAN_POINT('Ctrl Pts',(33.2206049447144,-54.4590811533792,0.778447264201043));
#39680=CARTESIAN_POINT('Ctrl Pts',(31.3511706755798,-54.6923464552708,0.889585154769084));
#39681=CARTESIAN_POINT('Ctrl Pts',(30.5332729159539,-56.3894735693295,1.00072304533713));
#39682=CARTESIAN_POINT('Ctrl Pts',(31.5155427604287,-57.9970628015172,1.11186093590517));
#39683=CARTESIAN_POINT('Ctrl Pts',(33.3988974808522,-58.0436694962152,1.22299882647321));
#39684=CARTESIAN_POINT('Ctrl Pts',(34.4594811428283,-56.4866340172583,1.33413671704125));
#39685=CARTESIAN_POINT('Ctrl Pts',(33.7265294927624,-54.7511285964952,1.44527460760929));
#39686=CARTESIAN_POINT('Ctrl Pts',(31.8709214881723,-54.4256810275324,1.55641249817733));
#39687=CARTESIAN_POINT('Ctrl Pts',(30.5911161796977,-55.8081771610621,1.66755038874538));
#39688=CARTESIAN_POINT('Ctrl Pts',(31.0585338801586,-57.633202607495,1.77868827931342));
#39689=CARTESIAN_POINT('Ctrl Pts',(32.845341867449,-58.2302908785133,1.88982616988146));
#39690=CARTESIAN_POINT('Ctrl Pts',(34.3160545270196,-57.0529203082132,2.0009640604495));
#39691=CARTESIAN_POINT('Ctrl Pts',(34.1245118825503,-55.1787515318803,2.11210195101754));
#39692=CARTESIAN_POINT('Ctrl Pts',(32.4460350887647,-54.323232485012,2.22323984158559));
#39693=CARTESIAN_POINT('Ctrl Pts',(30.8169529902366,-55.2694294534524,2.33437773215363));
#39694=CARTESIAN_POINT('Ctrl Pts',(30.7283829067961,-57.1512776213849,2.44551562272167));
#39695=CARTESIAN_POINT('Ctrl Pts',(32.2613940402694,-58.2463000190907,2.55665351328971));
#39696=CARTESIAN_POINT('Ctrl Pts',(34.0128039146598,-57.5522102275515,2.66779140385775));
#39697=CARTESIAN_POINT('Ctrl Pts',(34.3795272095987,-55.7043165044765,2.77892929442579));
#39698=CARTESIAN_POINT('Ctrl Pts',(33.0258979343036,-54.3940169311364,2.89006718499384));
#39699=CARTESIAN_POINT('Ctrl Pts',(31.1909083156521,-54.8206435668173,3.00120507556187));
#39700=CARTESIAN_POINT('Ctrl Pts',(30.5541451617937,-56.5937002136054,3.11234296612992));
#39701=CARTESIAN_POINT('Ctrl Pts',(31.6984450088402,-58.0902880148654,3.22348085669796));
#39702=CARTESIAN_POINT('Ctrl Pts',(33.5764172295469,-57.9405631836442,3.334618747266));
#39703=CARTESIAN_POINT('Ctrl Pts',(34.4691325526481,-56.2815705559534,3.44575663783404));
#39704=CARTESIAN_POINT('Ctrl Pts',(33.5594785188274,-54.6318048981748,3.55689452840209));
#39705=CARTESIAN_POINT('Ctrl Pts',(31.6800717814225,-54.5013154264873,3.66803241897013));
#39706=CARTESIAN_POINT('Ctrl Pts',(30.5511546410956,-56.0095406341798,3.77917030953817));
#39707=CARTESIAN_POINT('Ctrl Pts',(31.2060377591921,-57.77598488421,3.89030820010622));
#39708=CARTESIAN_POINT('Ctrl Pts',(33.0452991908126,-58.1838017216931,4.00144609067425));
#39709=CARTESIAN_POINT('Ctrl Pts',(34.3854420890035,-56.8597117703073,4.1125839812423));
#39710=CARTESIAN_POINT('Ctrl Pts',(33.9998184606928,-55.0156695787891,4.22372187181033));
#39711=CARTESIAN_POINT('Ctrl Pts',(32.2413939863492,-54.3395478778331,4.33485976237838));
#39712=CARTESIAN_POINT('Ctrl Pts',(30.7196745288183,-55.4502085281907,4.44599765294642));
#39713=CARTESIAN_POINT('Ctrl Pts',(30.8275071658684,-57.3310512405928,4.55713554351447));
#39714=CARTESIAN_POINT('Ctrl Pts',(32.4661914602743,-58.2605193506652,4.6682734340825));
#39715=CARTESIAN_POINT('Ctrl Pts',(34.135821096663,-57.3878601553885,4.77941132465055));
#39716=CARTESIAN_POINT('Ctrl Pts',(34.3081651275095,-55.5118285147887,4.89054921521859));
#39717=CARTESIAN_POINT('Ctrl Pts',(32.8254751197057,-54.349577461249,5.00168710578663));
#39718=CARTESIAN_POINT('Ctrl Pts',(31.0448740266844,-54.9649285726684,5.11282499635467));
#39719=CARTESIAN_POINT('Ctrl Pts',(30.5961662731525,-56.7946439827407,5.22396288692271));
#39720=CARTESIAN_POINT('Ctrl Pts',(31.8900590533422,-58.1639644570316,5.33510077749075));
#39721=CARTESIAN_POINT('Ctrl Pts',(33.7422378333798,-57.819535374986,5.4462386680588));
#39722=CARTESIAN_POINT('Ctrl Pts',(34.4573819695178,-56.076616703484,5.55737655862683));
#39723=CARTESIAN_POINT('Ctrl Pts',(33.3809127223489,-54.5305214257638,5.66851444919488));
#39724=CARTESIAN_POINT('Ctrl Pts',(31.4981330119909,-54.5964085667957,5.77965233976292));
#39725=CARTESIAN_POINT('Ctrl Pts',(30.5323756240669,-56.2139699170398,5.89079023033097));
#39726=CARTESIAN_POINT('Ctrl Pts',(31.3676029490312,-57.9026351433968,6.00192812089901));
#39727=CARTESIAN_POINT('Ctrl Pts',(33.2393344828578,-58.1167460012091,6.11306601146704));
#39728=CARTESIAN_POINT('Ctrl Pts',(34.4343281672319,-56.6603319824485,6.22420390203509));
#39729=CARTESIAN_POINT('Ctrl Pts',(33.8588424113751,-54.8664502505916,6.33534179260313));
#39730=CARTESIAN_POINT('Ctrl Pts',(32.0395269631849,-54.3770911652607,6.44647968317118));
#39731=CARTESIAN_POINT('Ctrl Pts',(30.6418187305185,-55.6401107988729,6.55761757373921));
#39732=CARTESIAN_POINT('Ctrl Pts',(30.9446640768632,-57.4995720858053,6.66875546430725));
#39733=CARTESIAN_POINT('Ctrl Pts',(32.6716452510335,-58.2532519029269,6.7798933548753));
#39734=CARTESIAN_POINT('Ctrl Pts',(34.2404831962862,-57.2117704392446,6.89103124544334));
#39735=CARTESIAN_POINT('Ctrl Pts',(34.2183071453089,-55.3274697977207,7.00216913601138));
#39736=CARTESIAN_POINT('Ctrl Pts',(32.6190914442238,-54.3269220694063,7.11330702657943));
#39737=CARTESIAN_POINT('Ctrl Pts',(31.4873233416682,-54.8574472987172,7.18739895362479));
#39738=CARTESIAN_POINT('Ctrl Pts',(31.1587240665777,-55.3034534568682,7.22444491714747));
#39739=CARTESIAN_POINT('Ctrl Pts',(32.8235677524625,-54.525462293325,-2.07481497238249));
#39740=CARTESIAN_POINT('Ctrl Pts',(32.2362679063105,-54.4178683176327,-2.03776900885981));
#39741=CARTESIAN_POINT('Ctrl Pts',(30.9559276871685,-54.8368917830923,-1.96367708181445));
#39742=CARTESIAN_POINT('Ctrl Pts',(30.4389462976543,-56.8032151562412,-1.85253919124641));
#39743=CARTESIAN_POINT('Ctrl Pts',(31.8127163182479,-58.2991210074574,-1.74140130067837));
#39744=CARTESIAN_POINT('Ctrl Pts',(33.8134790969391,-57.9586056331394,-1.63026341011032));
#39745=CARTESIAN_POINT('Ctrl Pts',(34.6130436110377,-56.0917909022585,-1.51912551954228));
#39746=CARTESIAN_POINT('Ctrl Pts',(33.477991135835,-54.4081700269832,-1.40798762897424));
#39747=CARTESIAN_POINT('Ctrl Pts',(31.4480356104804,-54.448390575124,-1.29684973840619));
#39748=CARTESIAN_POINT('Ctrl Pts',(30.3808227325527,-56.1758339752237,-1.18571184783816));
#39749=CARTESIAN_POINT('Ctrl Pts',(31.2533832993724,-58.0092533532185,-1.07457395727011));
#39750=CARTESIAN_POINT('Ctrl Pts',(33.2669528824098,-58.2705485634922,-0.963436066702072));
#39751=CARTESIAN_POINT('Ctrl Pts',(34.5785385674957,-56.7205283175549,-0.85229817613403));
#39752=CARTESIAN_POINT('Ctrl Pts',(33.9876059030427,-54.7779561935982,-0.741160285565989));
#39753=CARTESIAN_POINT('Ctrl Pts',(32.0350549182218,-54.2208842229542,-0.630022394997947));
#39754=CARTESIAN_POINT('Ctrl Pts',(30.5080713128749,-55.5592098448766,-0.518884504429905));
#39755=CARTESIAN_POINT('Ctrl Pts',(30.8043236932773,-57.56794685904,-0.407746613861863));
#39756=CARTESIAN_POINT('Ctrl Pts',(32.6526472907505,-58.4084762899819,-0.296608723293821));
#39757=CARTESIAN_POINT('Ctrl Pts',(34.3612513615134,-57.3114516183056,-0.185470832725779));
#39758=CARTESIAN_POINT('Ctrl Pts',(34.3662308175897,-55.2809921675532,-0.0743329421577379));
#39759=CARTESIAN_POINT('Ctrl Pts',(32.663028109885,-54.1756003992725,0.0368049484103038));
#39760=CARTESIAN_POINT('Ctrl Pts',(30.8106038901482,-55.0070539855567,0.147942838978346));
#39761=CARTESIAN_POINT('Ctrl Pts',(30.5045031059899,-57.0143140041392,0.259080729546387));
#39762=CARTESIAN_POINT('Ctrl Pts',(32.024903250764,-58.3601126089029,0.370218620114429));
#39763=CARTESIAN_POINT('Ctrl Pts',(33.9801648424124,-57.8126250680989,0.48135651068247));
#39764=CARTESIAN_POINT('Ctrl Pts',(34.5806147654118,-55.8729729399784,0.592494401250513));
#39765=CARTESIAN_POINT('Ctrl Pts',(33.2766543989476,-54.3165418129426,0.703632291818553));
#39766=CARTESIAN_POINT('Ctrl Pts',(31.261813452717,-54.5679507495102,0.814770182386596));
#39767=CARTESIAN_POINT('Ctrl Pts',(30.3802986954811,-56.3970822984609,0.925908072954637));
#39768=CARTESIAN_POINT('Ctrl Pts',(31.4389705811804,-58.1297116094828,1.03704596352268));
#39769=CARTESIAN_POINT('Ctrl Pts',(33.4688147268869,-58.1799434247417,1.14818385409072));
#39770=CARTESIAN_POINT('Ctrl Pts',(34.6118917659325,-56.5017999941152,1.25932174465876));
#39771=CARTESIAN_POINT('Ctrl Pts',(33.8219303211561,-54.6313050310709,1.3704596352268));
#39772=CARTESIAN_POINT('Ctrl Pts',(31.8219910617071,-54.2805437881517,1.48159752579485));
#39773=CARTESIAN_POINT('Ctrl Pts',(30.4426410726264,-55.7705720088982,1.59273541636289));
#39774=CARTESIAN_POINT('Ctrl Pts',(30.9464150418056,-57.7375499647951,1.70387330693093));
#39775=CARTESIAN_POINT('Ctrl Pts',(32.872202942073,-58.381080425761,1.81501119749897));
#39776=CARTESIAN_POINT('Ctrl Pts',(34.4573092683919,-57.1121326627429,1.92614908806701));
#39777=CARTESIAN_POINT('Ctrl Pts',(34.2508682239551,-55.0921889540774,2.03728697863506));
#39778=CARTESIAN_POINT('Ctrl Pts',(32.4418376379359,-54.1701266840256,2.1484248692031));
#39779=CARTESIAN_POINT('Ctrl Pts',(30.68604372152,-55.1899199052636,2.25956275977114));
#39780=CARTESIAN_POINT('Ctrl Pts',(30.5905845584601,-57.2181403171501,2.37070065033918));
#39781=CARTESIAN_POINT('Ctrl Pts',(32.2428350032855,-58.3983347751019,2.48183854090722));
#39782=CARTESIAN_POINT('Ctrl Pts',(34.1304714860531,-57.65025790744,2.59297643147526));
#39783=CARTESIAN_POINT('Ctrl Pts',(34.5257189268319,-55.6586329549041,2.70411432204331));
#39784=CARTESIAN_POINT('Ctrl Pts',(33.0668028606663,-54.2464168231134,2.81525221261135));
#39785=CARTESIAN_POINT('Ctrl Pts',(31.0890857081511,-54.7062269531163,2.92639010317939));
#39786=CARTESIAN_POINT('Ctrl Pts',(30.4027944078215,-56.6171939183195,3.03752799374743));
#39787=CARTESIAN_POINT('Ctrl Pts',(31.636099169942,-58.2301879836331,3.14866588431548));
#39788=CARTESIAN_POINT('Ctrl Pts',(33.660142159116,-58.0688173884789,3.25980377488351));
#39789=CARTESIAN_POINT('Ctrl Pts',(34.6222938731447,-56.2807864686682,3.37094166545156));
#39790=CARTESIAN_POINT('Ctrl Pts',(33.6418859366333,-54.5027002027541,3.4820795560196));
#39791=CARTESIAN_POINT('Ctrl Pts',(31.6162968524565,-54.3620611147965,3.59321744658764));
#39792=CARTESIAN_POINT('Ctrl Pts',(30.3995712810967,-55.9875977569607,3.70435533715568));
#39793=CARTESIAN_POINT('Ctrl Pts',(31.1053919366403,-57.8914380058304,3.81549322772373));
#39794=CARTESIAN_POINT('Ctrl Pts',(33.0877131684893,-58.3309752906067,3.92663111829176));
#39795=CARTESIAN_POINT('Ctrl Pts',(34.5320938721367,-56.9038961498249,4.03776900885981));
#39796=CARTESIAN_POINT('Ctrl Pts',(34.116476009031,-54.916422305255,4.14890689942785));
#39797=CARTESIAN_POINT('Ctrl Pts',(32.2212793229225,-54.1877111062503,4.26004478999589));
#39798=CARTESIAN_POINT('Ctrl Pts',(30.5811988331557,-55.3847601775417,4.37118268056393));
#39799=CARTESIAN_POINT('Ctrl Pts',(30.6974188126734,-57.4118969284484,4.48232057113197));
#39800=CARTESIAN_POINT('Ctrl Pts',(32.4635617944443,-58.4136601021044,4.59345846170002));
#39801=CARTESIAN_POINT('Ctrl Pts',(34.2630570813224,-57.4731245038337,4.70459635226806));
#39802=CARTESIAN_POINT('Ctrl Pts',(34.4488062226114,-55.4511730352461,4.8157342428361));
#39803=CARTESIAN_POINT('Ctrl Pts',(32.8507909365895,-54.1985208018218,4.92687213340414));
#39804=CARTESIAN_POINT('Ctrl Pts',(30.9316927097324,-54.8617346072315,5.03801002397219));
#39805=CARTESIAN_POINT('Ctrl Pts',(30.4480839679681,-56.833767317357,5.14914791454023));
#39806=CARTESIAN_POINT('Ctrl Pts',(31.8426171679855,-58.309595061432,5.26028580510826));
#39807=CARTESIAN_POINT('Ctrl Pts',(33.8388604739813,-57.9383759022264,5.37142369567631));
#39808=CARTESIAN_POINT('Ctrl Pts',(34.6096293165867,-56.0598910775539,5.48256158624434));
#39809=CARTESIAN_POINT('Ctrl Pts',(33.4494310938601,-54.3935387891867,5.5936994768124));
#39810=CARTESIAN_POINT('Ctrl Pts',(31.4202066831417,-54.4645507053438,5.70483736738043));
#39811=CARTESIAN_POINT('Ctrl Pts',(30.379331611233,-56.2079277768579,5.81597525794847));
#39812=CARTESIAN_POINT('Ctrl Pts',(31.2795238466775,-58.0279392630681,5.92711314851652));
#39813=CARTESIAN_POINT('Ctrl Pts',(33.2968407414035,-58.2587039015876,6.03825103908455));
#39814=CARTESIAN_POINT('Ctrl Pts',(34.5847823639129,-56.6890083802674,6.1493889296526));
#39815=CARTESIAN_POINT('Ctrl Pts',(33.9645346857693,-54.755596531712,6.26052682022064));
#39816=CARTESIAN_POINT('Ctrl Pts',(32.0037108581305,-54.2281745523389,6.37166471078869));
#39817=CARTESIAN_POINT('Ctrl Pts',(30.4972873242538,-55.5894332580934,6.48280260135673));
#39818=CARTESIAN_POINT('Ctrl Pts',(30.8236883185359,-57.5935255124717,6.59394049192477));
#39819=CARTESIAN_POINT('Ctrl Pts',(32.6849960096048,-58.4058273841964,6.70507838249281));
#39820=CARTESIAN_POINT('Ctrl Pts',(34.3758599154851,-57.2833383336781,6.81621627306086));
#39821=CARTESIAN_POINT('Ctrl Pts',(34.3519589865933,-55.2524746920757,6.92735416362889));
#39822=CARTESIAN_POINT('Ctrl Pts',(32.6283545092382,-54.1741032483986,7.03849205419694));
#39823=CARTESIAN_POINT('Ctrl Pts',(31.4085562246361,-54.7458933202255,7.1125839812423));
#39824=CARTESIAN_POINT('Ctrl Pts',(31.0543981323804,-55.2265903335148,7.14962994476498));
#39825=CARTESIAN_POINT('Ctrl Pts',(32.8469189315166,-54.3980002883409,-2.14962994476498));
#39826=CARTESIAN_POINT('Ctrl Pts',(32.2172349362596,-54.2826414900653,-2.1125839812423));
#39827=CARTESIAN_POINT('Ctrl Pts',(30.8444953556861,-54.7319049652148,-2.03849205419694));
#39828=CARTESIAN_POINT('Ctrl Pts',(30.2902045467308,-56.8401336080184,-1.92735416362889));
#39829=CARTESIAN_POINT('Ctrl Pts',(31.7631165537738,-58.4439957222243,-1.81621627306085));
#39830=CARTESIAN_POINT('Ctrl Pts',(33.9082700189114,-58.0789060959426,-1.70507838249281));
#39831=CARTESIAN_POINT('Ctrl Pts',(34.7655373602912,-56.0773674171097,-1.59394049192477));
#39832=CARTESIAN_POINT('Ctrl Pts',(33.5485706232913,-54.2722432949299,-1.48280260135673));
#39833=CARTESIAN_POINT('Ctrl Pts',(31.3721176346275,-54.3153664723165,-1.37166471078869));
#39834=CARTESIAN_POINT('Ctrl Pts',(30.2278863306926,-56.1674756953684,-1.26052682022065));
#39835=CARTESIAN_POINT('Ctrl Pts',(31.1634176907273,-58.1332089515266,-1.1493889296526));
#39836=CARTESIAN_POINT('Ctrl Pts',(33.3223021993517,-58.4133612672894,-1.03825103908456));
#39837=CARTESIAN_POINT('Ctrl Pts',(34.7285421630059,-56.7514794405087,-0.927113148516519));
#39838=CARTESIAN_POINT('Ctrl Pts',(34.0949631768734,-54.6687161227546,-0.815975257948478));
#39839=CARTESIAN_POINT('Ctrl Pts',(32.0015008456287,-54.0714414828596,-0.704837367380436));
#39840=CARTESIAN_POINT('Ctrl Pts',(30.3643181635511,-55.5063511462768,-0.593699476812395));
#39841=CARTESIAN_POINT('Ctrl Pts',(30.6819504321758,-57.6600543300705,-0.482561586244352));
#39842=CARTESIAN_POINT('Ctrl Pts',(32.6636635128286,-58.5612429370053,-0.371423695676311));
#39843=CARTESIAN_POINT('Ctrl Pts',(34.4955738132308,-57.3850483871807,-0.260285805108268));
#39844=CARTESIAN_POINT('Ctrl Pts',(34.5009126257928,-55.208055105922,-0.149147914540227));
#39845=CARTESIAN_POINT('Ctrl Pts',(32.6747934930414,-54.0228896243784,-0.038010023972185));
#39846=CARTESIAN_POINT('Ctrl Pts',(30.6886838571589,-54.9143474027391,0.0731278665958571));
#39847=CARTESIAN_POINT('Ctrl Pts',(30.3604924469568,-57.0664669994019,0.184265757163899));
#39848=CARTESIAN_POINT('Ctrl Pts',(31.9906165544693,-58.5093889545349,0.29540364773194));
#39849=CARTESIAN_POINT('Ctrl Pts',(34.086985111125,-57.9223904318795,0.406541538299982));
#39850=CARTESIAN_POINT('Ctrl Pts',(34.7307681955977,-55.8427578396932,0.517679428868024));
#39851=CARTESIAN_POINT('Ctrl Pts',(33.3327038531808,-54.1740024725061,0.628817319436065));
#39852=CARTESIAN_POINT('Ctrl Pts',(31.1724562298542,-54.4435550437495,0.739955210004107));
#39853=CARTESIAN_POINT('Ctrl Pts',(30.2273244750083,-56.4046910275923,0.851093100572148));
#39854=CARTESIAN_POINT('Ctrl Pts',(31.362398401932,-58.2623604174484,0.962230991140191));
#39855=CARTESIAN_POINT('Ctrl Pts',(33.5387319729216,-58.3162173532682,1.07336888170823));
#39856=CARTESIAN_POINT('Ctrl Pts',(34.7643023890366,-56.5169659709723,1.18450677227627));
#39857=CARTESIAN_POINT('Ctrl Pts',(33.9173311495497,-54.5114814656466,1.29564466284432));
#39858=CARTESIAN_POINT('Ctrl Pts',(31.7730606352419,-54.135406548771,1.40678255341236));
#39859=CARTESIAN_POINT('Ctrl Pts',(30.2941659655551,-55.7329668567343,1.5179204439804));
#39860=CARTESIAN_POINT('Ctrl Pts',(30.8342962034526,-57.8418973220951,1.62905833454844));
#39861=CARTESIAN_POINT('Ctrl Pts',(32.899064016697,-58.5318699730087,1.74019622511648));
#39862=CARTESIAN_POINT('Ctrl Pts',(34.5985640097642,-57.1713450172728,1.85133411568452));
#39863=CARTESIAN_POINT('Ctrl Pts',(34.37722456536,-55.0056263762742,1.96247200625257));
#39864=CARTESIAN_POINT('Ctrl Pts',(32.437640187107,-54.0170208830394,2.07360989682061));
#39865=CARTESIAN_POINT('Ctrl Pts',(30.5551344528034,-55.1104103570745,2.18474778738865));
#39866=CARTESIAN_POINT('Ctrl Pts',(30.4527862101241,-57.2850030129155,2.29588567795669));
#39867=CARTESIAN_POINT('Ctrl Pts',(32.2242759663018,-58.550369531113,2.40702356852473));
#39868=CARTESIAN_POINT('Ctrl Pts',(34.2481390574464,-57.7483055873284,2.51816145909278));
#39869=CARTESIAN_POINT('Ctrl Pts',(34.6719106440652,-55.6129494053317,2.62929934966082));
#39870=CARTESIAN_POINT('Ctrl Pts',(33.1077077870289,-54.0988167150904,2.74043724022886));
#39871=CARTESIAN_POINT('Ctrl Pts',(30.9872631006501,-54.5918103394153,2.8515751307969));
#39872=CARTESIAN_POINT('Ctrl Pts',(30.2514436538494,-56.6406876230335,2.96271302136494));
#39873=CARTESIAN_POINT('Ctrl Pts',(31.5737533310438,-58.3700879524008,3.07385091193298));
#39874=CARTESIAN_POINT('Ctrl Pts',(33.7438670886851,-58.1970715933135,3.18498880250103));
#39875=CARTESIAN_POINT('Ctrl Pts',(34.7754551936414,-56.2800023813831,3.29612669306906));
#39876=CARTESIAN_POINT('Ctrl Pts',(33.7242933544393,-54.3735955073335,3.40726458363711));
#39877=CARTESIAN_POINT('Ctrl Pts',(31.5525219234905,-54.2228068031056,3.51840247420514));
#39878=CARTESIAN_POINT('Ctrl Pts',(30.2479879210979,-55.9656548797418,3.6295403647732));
#39879=CARTESIAN_POINT('Ctrl Pts',(31.0047461140885,-58.0068911274507,3.74067825534123));
#39880=CARTESIAN_POINT('Ctrl Pts',(33.1301271461661,-58.4781488595202,3.85181614590928));
#39881=CARTESIAN_POINT('Ctrl Pts',(34.67874565527,-56.9480805293426,3.96295403647732));
#39882=CARTESIAN_POINT('Ctrl Pts',(34.2331335573692,-54.8171750317208,4.07409192704536));
#39883=CARTESIAN_POINT('Ctrl Pts',(32.2011646594958,-54.0358743346676,4.1852298176134));
#39884=CARTESIAN_POINT('Ctrl Pts',(30.442723137493,-55.3193118268927,4.29636770818144));
#39885=CARTESIAN_POINT('Ctrl Pts',(30.5673304594784,-57.492742616304,4.40750559874949));
#39886=CARTESIAN_POINT('Ctrl Pts',(32.4609321286143,-58.5668008535436,4.51864348931753));
#39887=CARTESIAN_POINT('Ctrl Pts',(34.3902930659818,-57.5583888522789,4.62978137988557));
#39888=CARTESIAN_POINT('Ctrl Pts',(34.5894473177133,-55.3905175557034,4.74091927045361));
#39889=CARTESIAN_POINT('Ctrl Pts',(32.8761067534734,-54.0474641423945,4.85205716102165));
#39890=CARTESIAN_POINT('Ctrl Pts',(30.8185113927803,-54.7585406417947,4.96319505158969));
#39891=CARTESIAN_POINT('Ctrl Pts',(30.3000016627836,-56.8728906519733,5.07433294215774));
#39892=CARTESIAN_POINT('Ctrl Pts',(31.7951752826287,-58.4552256658322,5.18547083272577));
#39893=CARTESIAN_POINT('Ctrl Pts',(33.9354831145828,-58.0572164294669,5.29660872329383));
#39894=CARTESIAN_POINT('Ctrl Pts',(34.7618766636556,-56.0431654516238,5.40774661386186));
#39895=CARTESIAN_POINT('Ctrl Pts',(33.5179494653713,-54.2565561526097,5.5188845044299));
#39896=CARTESIAN_POINT('Ctrl Pts',(31.3422803542925,-54.3326928438919,5.63002239499794));
#39897=CARTESIAN_POINT('Ctrl Pts',(30.226287598399,-56.2018856366762,5.74116028556598));
#39898=CARTESIAN_POINT('Ctrl Pts',(31.1914447443238,-58.1532433827394,5.85229817613403));
#39899=CARTESIAN_POINT('Ctrl Pts',(33.354346999949,-58.4006618019662,5.96343606670207));
#39900=CARTESIAN_POINT('Ctrl Pts',(34.7352365605938,-56.7176847780862,6.07457395727011));
#39901=CARTESIAN_POINT('Ctrl Pts',(34.0702269601635,-54.6447428128324,6.18571184783815));
#39902=CARTESIAN_POINT('Ctrl Pts',(31.9678947530762,-54.0792579394171,6.2968497384062));
#39903=CARTESIAN_POINT('Ctrl Pts',(30.3527559179891,-55.5387557173139,6.40798762897423));
#39904=CARTESIAN_POINT('Ctrl Pts',(30.7027125602088,-57.6874789391381,6.51912551954228));
#39905=CARTESIAN_POINT('Ctrl Pts',(32.6983467681761,-58.5584028654658,6.63026341011033));
#39906=CARTESIAN_POINT('Ctrl Pts',(34.5112366346842,-57.3549062281116,6.74140130067836));
#39907=CARTESIAN_POINT('Ctrl Pts',(34.4856108278775,-55.1774795864305,6.85253919124641));
#39908=CARTESIAN_POINT('Ctrl Pts',(32.6376175742527,-54.021284427391,6.96367708181444));
#39909=CARTESIAN_POINT('Ctrl Pts',(31.329789107604,-54.6343393417337,7.03776900885981));
#39910=CARTESIAN_POINT('Ctrl Pts',(30.9500721981832,-55.1497272101613,7.07481497238249));
#39911=CARTESIAN_POINT('Ctrl Pts',(32.8702701105707,-54.2705382833568,-2.22444491714747));
#39912=CARTESIAN_POINT('Ctrl Pts',(32.1982019662087,-54.147414662498,-2.18739895362479));
#39913=CARTESIAN_POINT('Ctrl Pts',(30.7330630242036,-54.6269181473375,-2.11330702657943));
#39914=CARTESIAN_POINT('Ctrl Pts',(30.1414627958074,-56.8770520597956,-2.00216913601138));
#39915=CARTESIAN_POINT('Ctrl Pts',(31.7135167892996,-58.5888704369913,-1.89103124544334));
#39916=CARTESIAN_POINT('Ctrl Pts',(34.0030609408839,-58.1992065587458,-1.7798933548753));
#39917=CARTESIAN_POINT('Ctrl Pts',(34.9180311095446,-56.062943931961,-1.66875546430726));
#39918=CARTESIAN_POINT('Ctrl Pts',(33.6191501107478,-54.1363165628765,-1.55761757373922));
#39919=CARTESIAN_POINT('Ctrl Pts',(31.2961996587745,-54.182342369509,-1.44647968317117));
#39920=CARTESIAN_POINT('Ctrl Pts',(30.0749499288325,-56.1591174155133,-1.33534179260313));
#39921=CARTESIAN_POINT('Ctrl Pts',(31.0734520820822,-58.2571645498346,-1.22420390203509));
#39922=CARTESIAN_POINT('Ctrl Pts',(33.3776515162936,-58.5561739710866,-1.11306601146705));
#39923=CARTESIAN_POINT('Ctrl Pts',(34.8785457585159,-56.7824305634625,-1.00192812089901));
#39924=CARTESIAN_POINT('Ctrl Pts',(34.2023204507043,-54.559476051911,-0.890790230330967));
#39925=CARTESIAN_POINT('Ctrl Pts',(31.9679467730355,-53.921998742765,-0.779652339762925));
#39926=CARTESIAN_POINT('Ctrl Pts',(30.2205650142273,-55.453492447677,-0.668514449194883));
#39927=CARTESIAN_POINT('Ctrl Pts',(30.5595771710743,-57.7521618011011,-0.557376558626841));
#39928=CARTESIAN_POINT('Ctrl Pts',(32.6746797349067,-58.7140095840285,-0.446238668058799));
#39929=CARTESIAN_POINT('Ctrl Pts',(34.6298962649481,-57.4586451560558,-0.335100777490757));
#39930=CARTESIAN_POINT('Ctrl Pts',(34.6355944339958,-55.1351180442909,-0.223962886922716));
#39931=CARTESIAN_POINT('Ctrl Pts',(32.6865588761979,-53.8701788494842,-0.112824996354674));
#39932=CARTESIAN_POINT('Ctrl Pts',(30.5667638241697,-54.8216408199215,-0.00168710578663165));
#39933=CARTESIAN_POINT('Ctrl Pts',(30.2164817879238,-57.1186199946645,0.109450784781409));
#39934=CARTESIAN_POINT('Ctrl Pts',(31.9563298581746,-58.6586653001669,0.220588675349451));
#39935=CARTESIAN_POINT('Ctrl Pts',(34.1938053798376,-58.0321557956601,0.331726565917493));
#39936=CARTESIAN_POINT('Ctrl Pts',(34.8809216257836,-55.8125427394079,0.442864456485535));
#39937=CARTESIAN_POINT('Ctrl Pts',(33.388753307414,-54.0314631320695,0.554002347053576));
#39938=CARTESIAN_POINT('Ctrl Pts',(31.0830990069914,-54.3191593379889,0.665140237621618));
#39939=CARTESIAN_POINT('Ctrl Pts',(30.0743502545355,-56.4122997567237,0.77627812818966));
#39940=CARTESIAN_POINT('Ctrl Pts',(31.2858262226837,-58.3950092254139,0.887416018757702));
#39941=CARTESIAN_POINT('Ctrl Pts',(33.6086492189562,-58.4524912817948,0.998553909325743));
#39942=CARTESIAN_POINT('Ctrl Pts',(34.9167130121408,-56.5321319478292,1.10969179989378));
#39943=CARTESIAN_POINT('Ctrl Pts',(34.0127319779433,-54.3916579002223,1.22082969046183));
#39944=CARTESIAN_POINT('Ctrl Pts',(31.7241302087767,-53.9902693093903,1.33196758102987));
#39945=CARTESIAN_POINT('Ctrl Pts',(30.1456908584837,-55.6953617045704,1.44310547159791));
#39946=CARTESIAN_POINT('Ctrl Pts',(30.7221773650996,-57.9462446793952,1.55424336216595));
#39947=CARTESIAN_POINT('Ctrl Pts',(32.925925091321,-58.6826595202564,1.66538125273399));
#39948=CARTESIAN_POINT('Ctrl Pts',(34.7398187511365,-57.2305573718025,1.77651914330204));
#39949=CARTESIAN_POINT('Ctrl Pts',(34.5035809067649,-54.9190637984713,1.88765703387008));
#39950=CARTESIAN_POINT('Ctrl Pts',(32.4334427362781,-53.863915082053,1.99879492443812));
#39951=CARTESIAN_POINT('Ctrl Pts',(30.4242251840868,-55.0309008088856,2.10993281500616));
#39952=CARTESIAN_POINT('Ctrl Pts',(30.3149878617883,-57.3518657086808,2.2210707055742));
#39953=CARTESIAN_POINT('Ctrl Pts',(32.2057169293179,-58.7024042871242,2.33220859614224));
#39954=CARTESIAN_POINT('Ctrl Pts',(34.3658066288398,-57.8463532672169,2.44334648671029));
#39955=CARTESIAN_POINT('Ctrl Pts',(34.8181023612983,-55.5672658557593,2.55448437727833));
#39956=CARTESIAN_POINT('Ctrl Pts',(33.1486127133916,-53.9512166070675,2.66562226784637));
#39957=CARTESIAN_POINT('Ctrl Pts',(30.8854404931491,-54.4773937257142,2.77676015841441));
#39958=CARTESIAN_POINT('Ctrl Pts',(30.1000928998772,-56.6641813277477,2.88789804898245));
#39959=CARTESIAN_POINT('Ctrl Pts',(31.5114074921456,-58.5099879211684,2.99903593955049));
#39960=CARTESIAN_POINT('Ctrl Pts',(33.8275920182542,-58.3253257981483,3.11017383011854));
#39961=CARTESIAN_POINT('Ctrl Pts',(34.9286165141379,-56.2792182940979,3.22131172068658));
#39962=CARTESIAN_POINT('Ctrl Pts',(33.8067007722452,-54.2444908119128,3.33244961125462));
#39963=CARTESIAN_POINT('Ctrl Pts',(31.4887469945245,-54.0835524914147,3.44358750182266));
#39964=CARTESIAN_POINT('Ctrl Pts',(30.0964045610991,-55.9437120025227,3.5547253923907));
#39965=CARTESIAN_POINT('Ctrl Pts',(30.9041002915367,-58.1223442490711,3.66586328295875));
#39966=CARTESIAN_POINT('Ctrl Pts',(33.1725411238428,-58.6253224284338,3.77700117352679));
#39967=CARTESIAN_POINT('Ctrl Pts',(34.8253974384033,-56.9922649088601,3.88813906409483));
#39968=CARTESIAN_POINT('Ctrl Pts',(34.3497911057074,-54.7179277581866,3.99927695466287));
#39969=CARTESIAN_POINT('Ctrl Pts',(32.181049996069,-53.8840375630849,4.11041484523092));
#39970=CARTESIAN_POINT('Ctrl Pts',(30.3042474418304,-55.2538634762437,4.22155273579895));
#39971=CARTESIAN_POINT('Ctrl Pts',(30.4372421062834,-57.5735883041596,4.332690626367));
#39972=CARTESIAN_POINT('Ctrl Pts',(32.4583024627843,-58.7199416049829,4.44382851693503));
#39973=CARTESIAN_POINT('Ctrl Pts',(34.5175290506412,-57.6436532007241,4.55496640750308));
#39974=CARTESIAN_POINT('Ctrl Pts',(34.7300884128151,-55.3298620761609,4.66610429807112));
#39975=CARTESIAN_POINT('Ctrl Pts',(32.9014225703573,-53.8964074829672,4.77724218863916));
#39976=CARTESIAN_POINT('Ctrl Pts',(30.7053300758282,-54.6553466763579,4.8883800792072));
#39977=CARTESIAN_POINT('Ctrl Pts',(30.1519193575992,-56.9120139865897,4.99951796977525));
#39978=CARTESIAN_POINT('Ctrl Pts',(31.7477333972719,-58.6008562702326,5.11065586034329));
#39979=CARTESIAN_POINT('Ctrl Pts',(34.0321057551844,-58.1760569567073,5.22179375091133));
#39980=CARTESIAN_POINT('Ctrl Pts',(34.9141240107243,-56.0264398256937,5.33293164147937));
#39981=CARTESIAN_POINT('Ctrl Pts',(33.5864678368826,-54.1195735160326,5.44406953204741));
#39982=CARTESIAN_POINT('Ctrl Pts',(31.2643540254432,-54.2008349824401,5.55520742261546));
#39983=CARTESIAN_POINT('Ctrl Pts',(30.0732435855651,-56.1958434964943,5.6663453131835));
#39984=CARTESIAN_POINT('Ctrl Pts',(31.10336564197,-58.2785475024108,5.77748320375154));
#39985=CARTESIAN_POINT('Ctrl Pts',(33.4118532584947,-58.5426197023447,5.88862109431958));
#39986=CARTESIAN_POINT('Ctrl Pts',(34.8856907572748,-56.7463611759051,5.99975898488763));
#39987=CARTESIAN_POINT('Ctrl Pts',(34.1759192345576,-54.5338890939528,6.11089687545566));
#39988=CARTESIAN_POINT('Ctrl Pts',(31.9320786480218,-53.9303413264954,6.22203476602372));
#39989=CARTESIAN_POINT('Ctrl Pts',(30.2082245117244,-55.4880781765343,6.33317265659174));
#39990=CARTESIAN_POINT('Ctrl Pts',(30.5817368018815,-57.7814323658044,6.44431054715979));
#39991=CARTESIAN_POINT('Ctrl Pts',(32.7116975267474,-58.7109783467354,6.55544843772783));
#39992=CARTESIAN_POINT('Ctrl Pts',(34.646613353883,-57.4264741225449,6.66658632829588));
#39993=CARTESIAN_POINT('Ctrl Pts',(34.6192626691618,-55.1024844807854,6.77772421886392));
#39994=CARTESIAN_POINT('Ctrl Pts',(32.6468806392671,-53.8684656063833,6.88886210943196));
#39995=CARTESIAN_POINT('Ctrl Pts',(31.2510219905719,-54.522785363242,6.96295403647732));
#39996=CARTESIAN_POINT('Ctrl Pts',(30.8457462639859,-55.0728640868079,7.));
#39997=CARTESIAN_POINT('Ctrl Pts',(32.8002165734083,-54.6529242983091,-2.));
#39998=CARTESIAN_POINT('Ctrl Pts',(32.7409294910778,-54.634811549331,-2.));
#39999=CARTESIAN_POINT('Ctrl Pts',(32.6807825146647,-54.6203475870769,-2.));
#40000=CARTESIAN_POINT('Ctrl Pts',(32.6200737029452,-54.6093586318095,-2.));
#40001=CARTESIAN_POINT('Ctrl Pts',(32.5553553259164,-54.5976439016079,-2.));
#40002=CARTESIAN_POINT('Ctrl Pts',(32.4899978846714,-54.5898778448639,-2.));
#40003=CARTESIAN_POINT('Ctrl Pts',(32.4243295074656,-54.5859022602815,-2.));
#40004=CARTESIAN_POINT('Ctrl Pts',(32.3668696774105,-54.5824236237718,-2.));
#40005=CARTESIAN_POINT('Ctrl Pts',(32.3091708471311,-54.5818478912346,-2.));
#40006=CARTESIAN_POINT('Ctrl Pts',(32.2514404192184,-54.5841026889815,-2.));
#40007=CARTESIAN_POINT('Ctrl Pts',(32.2224739676352,-54.5852340419287,-2.));
#40008=CARTESIAN_POINT('Ctrl Pts',(32.1934994333242,-54.5870784902626,-2.));
#40009=CARTESIAN_POINT('Ctrl Pts',(32.164542591354,-54.5896298423987,-2.));
#40010=CARTESIAN_POINT('Ctrl Pts',(32.1513153330264,-54.5907952800464,-2.));
#40011=CARTESIAN_POINT('Ctrl Pts',(32.1380900392148,-54.5921085587762,-2.));
#40012=CARTESIAN_POINT('Ctrl Pts',(32.1248906604594,-54.5935664859838,-2.));
#40013=CARTESIAN_POINT('Ctrl Pts',(32.0583157457256,-54.6009199668811,-2.));
#40014=CARTESIAN_POINT('Ctrl Pts',(31.9922802588125,-54.6119586521805,-2.));
#40015=CARTESIAN_POINT('Ctrl Pts',(31.9271057840968,-54.6265240331787,-2.));
#40016=CARTESIAN_POINT('Ctrl Pts',(31.8607754217499,-54.6413477353035,-2.));
#40017=CARTESIAN_POINT('Ctrl Pts',(31.7953358755732,-54.6598242742458,-2.));
#40018=CARTESIAN_POINT('Ctrl Pts',(31.7311141838614,-54.6818388621525,-2.));
#40019=CARTESIAN_POINT('Ctrl Pts',(31.6773947912155,-54.7002533613687,-2.));
#40020=CARTESIAN_POINT('Ctrl Pts',(31.624526967767,-54.7211443093805,-2.));
#40021=CARTESIAN_POINT('Ctrl Pts',(31.5727038894024,-54.7444721761566,-2.));
#40022=CARTESIAN_POINT('Ctrl Pts',(31.5488262835572,-54.7552205459113,-2.));
#40023=CARTESIAN_POINT('Ctrl Pts',(31.5251705391755,-54.7664866028724,-2.));
#40024=CARTESIAN_POINT('Ctrl Pts',(31.501756105982,-54.7782682438544,-2.));
#40025=CARTESIAN_POINT('Ctrl Pts',(31.4915364297278,-54.783410565925,-2.));
#40026=CARTESIAN_POINT('Ctrl Pts',(31.4813629900533,-54.7886510930647,-2.));
#40027=CARTESIAN_POINT('Ctrl Pts',(31.4712497594726,-54.7939828998507,-2.));
#40028=CARTESIAN_POINT('Ctrl Pts',(31.4091712444434,-54.8267113781603,-2.));
#40029=CARTESIAN_POINT('Ctrl Pts',(31.3492415725846,-54.8629343648032,-2.));
#40030=CARTESIAN_POINT('Ctrl Pts',(31.2918005106807,-54.9025187988006,-2.));
#40031=CARTESIAN_POINT('Ctrl Pts',(31.2404435140524,-54.93791051295,-2.));
#40032=CARTESIAN_POINT('Ctrl Pts',(31.1910752071398,-54.9759900914448,-2.));
#40033=CARTESIAN_POINT('Ctrl Pts',(31.1439444839342,-55.0166972030902,-2.));
#40034=CARTESIAN_POINT('Ctrl Pts',(31.0925988211616,-55.0610447854066,-2.));
#40035=CARTESIAN_POINT('Ctrl Pts',(31.043907590921,-55.1085103565108,-2.));
#40036=CARTESIAN_POINT('Ctrl Pts',(30.9979331337654,-55.1587747363377,-2.));
#40037=CARTESIAN_POINT('Ctrl Pts',(30.9801952413147,-55.1781677693093,-2.));
#40038=CARTESIAN_POINT('Ctrl Pts',(30.9628620787153,-55.1979778819377,-2.));
#40039=CARTESIAN_POINT('Ctrl Pts',(30.9459385065297,-55.218188320324,-2.));
#40040=CARTESIAN_POINT('Ctrl Pts',(30.9385143505167,-55.2270543827619,-2.));
#40041=CARTESIAN_POINT('Ctrl Pts',(30.9311694717035,-55.2359970996828,-2.));
#40042=CARTESIAN_POINT('Ctrl Pts',(30.923912574634,-55.2450044081391,-2.));
#40043=CARTESIAN_POINT('Ctrl Pts',(30.8800390053164,-55.2994605714461,-2.));
#40044=CARTESIAN_POINT('Ctrl Pts',(30.8392972474282,-55.3563704442589,-2.));
#40045=CARTESIAN_POINT('Ctrl Pts',(30.8017204449644,-55.4153538312338,-2.));
#40046=CARTESIAN_POINT('Ctrl Pts',(30.763273103291,-55.4757036822959,-2.));
#40047=CARTESIAN_POINT('Ctrl Pts',(30.7281385018843,-55.5382249057113,-2.));
#40048=CARTESIAN_POINT('Ctrl Pts',(30.6963834281664,-55.6025570259941,-2.));
#40049=CARTESIAN_POINT('Ctrl Pts',(30.6720872116783,-55.6517783609976,-2.));
#40050=CARTESIAN_POINT('Ctrl Pts',(30.6497699435205,-55.7020608595655,-2.));
#40051=CARTESIAN_POINT('Ctrl Pts',(30.629476572352,-55.7532569215707,-2.));
#40052=CARTESIAN_POINT('Ctrl Pts',(30.6168451594843,-55.7851234158567,-2.));
#40053=CARTESIAN_POINT('Ctrl Pts',(30.6049981367155,-55.8173440722639,-2.));
#40054=CARTESIAN_POINT('Ctrl Pts',(30.5939492528939,-55.8498849658379,-2.));
#40055=CARTESIAN_POINT('Ctrl Pts',(30.5877508307706,-55.868140402124,-2.));
#40056=CARTESIAN_POINT('Ctrl Pts',(30.581801893405,-55.8865028064696,-2.));
#40057=CARTESIAN_POINT('Ctrl Pts',(30.5761150803988,-55.9049328084338,-2.));
#40058=CARTESIAN_POINT('Ctrl Pts',(30.5540602837186,-55.9764086852896,-2.));
#40059=CARTESIAN_POINT('Ctrl Pts',(30.5359175198192,-56.0489705581569,-2.));
#40060=CARTESIAN_POINT('Ctrl Pts',(30.5217728584343,-56.1222396610388,-2.));
#40061=CARTESIAN_POINT('Ctrl Pts',(30.5111932477205,-56.1770418627137,-2.));
#40062=CARTESIAN_POINT('Ctrl Pts',(30.5028510892916,-56.2322406204203,-2.));
#40063=CARTESIAN_POINT('Ctrl Pts',(30.4967990447144,-56.2876867713494,-2.));
#40064=CARTESIAN_POINT('Ctrl Pts',(30.494911121078,-56.3049830912216,-2.));
#40065=CARTESIAN_POINT('Ctrl Pts',(30.4932461646271,-56.3223035268967,-2.));
#40066=CARTESIAN_POINT('Ctrl Pts',(30.4918060890607,-56.339643645384,-2.));
#40067=CARTESIAN_POINT('Ctrl Pts',(30.4904160490508,-56.3563812798787,-2.));
#40068=CARTESIAN_POINT('Ctrl Pts',(30.4892362965385,-56.3731287079821,-2.));
#40069=CARTESIAN_POINT('Ctrl Pts',(30.4882682431309,-56.3898758527173,-2.));
#40070=CARTESIAN_POINT('Ctrl Pts',(30.4839212193137,-56.465078559989,-2.));
#40071=CARTESIAN_POINT('Ctrl Pts',(30.4838360419498,-56.5403117892334,-2.));
#40072=CARTESIAN_POINT('Ctrl Pts',(30.4881238107187,-56.6152096419488,-2.));
#40073=CARTESIAN_POINT('Ctrl Pts',(30.4914053519372,-56.6725309211765,-2.));
#40074=CARTESIAN_POINT('Ctrl Pts',(30.4972490710536,-56.7296564032881,-2.));
#40075=CARTESIAN_POINT('Ctrl Pts',(30.5057249894128,-56.7864264638426,-2.));
#40076=CARTESIAN_POINT('Ctrl Pts',(30.5076920210892,-56.799601261268,-2.));
#40077=CARTESIAN_POINT('Ctrl Pts',(30.5098008972608,-56.8127569211082,-2.));
#40078=CARTESIAN_POINT('Ctrl Pts',(30.5120501580915,-56.8258920773861,-2.));
#40079=CARTESIAN_POINT('Ctrl Pts',(33.3325354057626,-57.7362457052863,-0.871480363390211));
#40080=CARTESIAN_POINT('Ctrl Pts',(33.2590763562245,-57.7795019958594,-0.877193940366669));
#40081=CARTESIAN_POINT('Ctrl Pts',(33.1823540930372,-57.8169005192734,-0.882907517343126));
#40082=CARTESIAN_POINT('Ctrl Pts',(33.1030496903124,-57.8476363980486,-0.888621094319584));
#40083=CARTESIAN_POINT('Ctrl Pts',(32.5888520129844,-58.0469231581002,-0.925667057842264));
#40084=CARTESIAN_POINT('Ctrl Pts',(31.966100460501,-57.9661104565054,-0.962713021364944));
#40085=CARTESIAN_POINT('Ctrl Pts',(31.5197930553252,-57.6421865224027,-0.999758984887625));
#40086=CARTESIAN_POINT('Ctrl Pts',(31.0734856501493,-57.3182625883,-1.03680494841031));
#40087=CARTESIAN_POINT('Ctrl Pts',(30.8036223922811,-56.7512274216894,-1.07385091193299));
#40088=CARTESIAN_POINT('Ctrl Pts',(30.8337231720004,-56.2005802421929,-1.11089687545567));
#40089=CARTESIAN_POINT('Ctrl Pts',(30.8638239517197,-55.6499330626964,-1.14794283897835));
#40090=CARTESIAN_POINT('Ctrl Pts',(31.1938887690265,-55.115673870314,-1.18498880250103));
#40091=CARTESIAN_POINT('Ctrl Pts',(31.6728308546874,-54.8423246209736,-1.22203476602371));
#40092=CARTESIAN_POINT('Ctrl Pts',(32.1517729403484,-54.5689753716333,-1.25908072954639));
#40093=CARTESIAN_POINT('Ctrl Pts',(32.7795922943635,-54.5565360653349,-1.29612669306907));
#40094=CARTESIAN_POINT('Ctrl Pts',(33.2690250069386,-54.8106693502475,-1.33317265659175));
#40095=CARTESIAN_POINT('Ctrl Pts',(33.7584577195138,-55.0648026351601,-1.37021862011443));
#40096=CARTESIAN_POINT('Ctrl Pts',(34.1095037906491,-55.5855085112837,-1.40726458363711));
#40097=CARTESIAN_POINT('Ctrl Pts',(34.1613832117471,-56.1345432465003,-1.44431054715979));
#40098=CARTESIAN_POINT('Ctrl Pts',(34.2132626328451,-56.6835779817169,-1.48135651068247));
#40099=CARTESIAN_POINT('Ctrl Pts',(33.9659754039058,-57.2609415760266,-1.51840247420515));
#40100=CARTESIAN_POINT('Ctrl Pts',(33.5329364407288,-57.6022802269071,-1.55544843772784));
#40101=CARTESIAN_POINT('Ctrl Pts',(33.470469460016,-57.6515192024594,-1.56079241294863));
#40102=CARTESIAN_POINT('Ctrl Pts',(33.4041372082081,-57.6958467816506,-1.56613638816942));
#40103=CARTESIAN_POINT('Ctrl Pts',(33.3347882996638,-57.7351190113229,-1.57148036339021));
#40104=CARTESIAN_POINT('Ctrl Pts',(31.0458737116219,-57.7433792852397,-2.));
#40105=CARTESIAN_POINT('Ctrl Pts',(31.5286078227264,-58.2269108712356,-1.96295403647732));
#40106=CARTESIAN_POINT('Ctrl Pts',(33.0063987810958,-58.6658791894418,-1.88886210943196));
#40107=CARTESIAN_POINT('Ctrl Pts',(34.7728277550873,-57.1516769644332,-1.77772421886392));
#40108=CARTESIAN_POINT('Ctrl Pts',(34.4535014835806,-54.8495668967865,-1.66658632829587));
#40109=CARTESIAN_POINT('Ctrl Pts',(32.3487507516394,-53.8677941230741,-1.55544843772784));
#40110=CARTESIAN_POINT('Ctrl Pts',(30.3811218874152,-55.1044118987674,-1.44431054715979));
#40111=CARTESIAN_POINT('Ctrl Pts',(30.3535878576004,-57.4278205885651,-1.33317265659175));
#40112=CARTESIAN_POINT('Ctrl Pts',(32.2903568834191,-58.7112317202033,-1.22203476602371));
#40113=CARTESIAN_POINT('Ctrl Pts',(34.4191815551847,-57.7799979545239,-1.11089687545567));
#40114=CARTESIAN_POINT('Ctrl Pts',(34.7912737376158,-55.4864512354733,-0.999758984887625));
#40115=CARTESIAN_POINT('Ctrl Pts',(33.0661792001092,-53.929919412126,-0.888621094319583));
#40116=CARTESIAN_POINT('Ctrl Pts',(30.822833264184,-54.5351044086332,-0.777483203751541));
#40117=CARTESIAN_POINT('Ctrl Pts',(30.1146276885619,-56.7480782089188,-0.6663453131835));
#40118=CARTESIAN_POINT('Ctrl Pts',(31.5897751037144,-58.543278448718,-0.555207422615457));
#40119=CARTESIAN_POINT('Ctrl Pts',(33.8980643703311,-58.2775391690228,-0.444069532047416));
#40120=CARTESIAN_POINT('Ctrl Pts',(34.926688116847,-56.1940939537869,-0.332931641479374));
#40121=CARTESIAN_POINT('Ctrl Pts',(33.7341373860101,-54.1999441339785,-0.221793750911332));
#40122=CARTESIAN_POINT('Ctrl Pts',(31.4119663698708,-54.1203575053852,-0.11065586034329));
#40123=CARTESIAN_POINT('Ctrl Pts',(30.0856850452223,-56.0281806868171,0.000482030224751475));
#40124=CARTESIAN_POINT('Ctrl Pts',(30.9692534931351,-58.1771614464075,0.111619920792793));
#40125=CARTESIAN_POINT('Ctrl Pts',(33.2539316216956,-58.6003133427487,0.222757811360835));
#40126=CARTESIAN_POINT('Ctrl Pts',(34.8485275651184,-56.9103206367347,0.333895701928877));
#40127=CARTESIAN_POINT('Ctrl Pts',(34.2934896049409,-54.6540528227808,0.445033592496919));
#40128=CARTESIAN_POINT('Ctrl Pts',(32.096850264347,-53.8966974164154,0.55617148306496));
#40129=CARTESIAN_POINT('Ctrl Pts',(30.2692184515671,-55.3314704112853,0.667309373633002));
#40130=CARTESIAN_POINT('Ctrl Pts',(30.4834462874739,-57.6451078131478,0.778447264201044));
#40131=CARTESIAN_POINT('Ctrl Pts',(32.5434486064222,-58.7199110699497,0.889585154769085));
#40132=CARTESIAN_POINT('Ctrl Pts',(34.563681922824,-57.5721005714895,1.00072304533713));
#40133=CARTESIAN_POINT('Ctrl Pts',(34.6950037716947,-55.2522802841409,1.11186093590517));
#40134=CARTESIAN_POINT('Ctrl Pts',(32.8172137752097,-53.883808025427,1.22299882647321));
#40135=CARTESIAN_POINT('Ctrl Pts',(30.6490744128704,-54.7192619732989,1.33413671704125));
#40136=CARTESIAN_POINT('Ctrl Pts',(30.1751082313325,-56.9939416545676,1.44527460760929));
#40137=CARTESIAN_POINT('Ctrl Pts',(31.8291418517329,-58.6258069603505,1.55641249817733));
#40138=CARTESIAN_POINT('Ctrl Pts',(34.0972195432855,-58.121193069651,1.66755038874538));
#40139=CARTESIAN_POINT('Ctrl Pts',(34.90334407317,-55.9419787993381,1.77868827931342));
#40140=CARTESIAN_POINT('Ctrl Pts',(33.5096605171051,-54.0828236849995,1.88982616988146));
#40141=CARTESIAN_POINT('Ctrl Pts',(31.1918232394055,-54.2454334870425,2.0009640604495));
#40142=CARTESIAN_POINT('Ctrl Pts',(30.0713749864112,-56.2809696095364,2.11210195101754));
#40143=CARTESIAN_POINT('Ctrl Pts',(31.1738747508358,-58.326282755013,2.22323984158559));
#40144=CARTESIAN_POINT('Ctrl Pts',(33.4901919951035,-58.5092746059889,2.33437773215363));
#40145=CARTESIAN_POINT('Ctrl Pts',(34.9001752767119,-56.6624506459969,2.44551562272167));
#40146=CARTESIAN_POINT('Ctrl Pts',(34.113250907707,-54.4762297900261,2.55665351328972));
#40147=CARTESIAN_POINT('Ctrl Pts',(31.8496996873681,-53.9516847809773,2.66779140385775));
#40148=CARTESIAN_POINT('Ctrl Pts',(30.1813757180883,-55.5689376143779,2.7789292944258));
#40149=CARTESIAN_POINT('Ctrl Pts',(30.63531484903,-57.8476984309217,2.89006718499383));
#40150=CARTESIAN_POINT('Ctrl Pts',(32.7960214456224,-58.7021916123209,3.00120507556188));
#40151=CARTESIAN_POINT('Ctrl Pts',(34.6857762559251,-57.350289859029,3.11234296612992));
#40152=CARTESIAN_POINT('Ctrl Pts',(34.5748652707907,-55.0294041774428,3.22348085669796));
#40153=CARTESIAN_POINT('Ctrl Pts',(32.5648065727292,-53.8638675525518,3.33461874726601));
#40154=CARTESIAN_POINT('Ctrl Pts',(30.4954296836915,-54.9205088752032,3.44575663783404));
#40155=CARTESIAN_POINT('Ctrl Pts',(30.2608587385459,-57.2321723596467,3.55689452840209));
#40156=CARTESIAN_POINT('Ctrl Pts',(32.0757991835954,-58.6829662025234,3.66803241897013));
#40157=CARTESIAN_POINT('Ctrl Pts',(34.2790154466699,-57.9449623463291,3.77917030953818));
#40158=CARTESIAN_POINT('Ctrl Pts',(34.8538786959893,-55.6936640901668,3.89030820010621));
#40159=CARTESIAN_POINT('Ctrl Pts',(33.2742100800909,-53.9897102593703,4.00144609067426));
#40160=CARTESIAN_POINT('Ctrl Pts',(30.9858981977034,-54.3927491193985,4.11258398124229));
#40161=CARTESIAN_POINT('Ctrl Pts',(30.0834608661246,-56.5338746309362,4.22372187181035));
#40162=CARTESIAN_POINT('Ctrl Pts',(31.3929092090316,-58.4532903311776,4.33485976237837));
#40163=CARTESIAN_POINT('Ctrl Pts',(33.71569030851,-58.394133262198,4.44599765294643));
#40164=CARTESIAN_POINT('Ctrl Pts',(34.9257362810773,-56.410550559801,4.55713554351446));
#40165=CARTESIAN_POINT('Ctrl Pts',(33.91547832718,-54.3181379674856,4.66827343408251));
#40166=CARTESIAN_POINT('Ctrl Pts',(31.609617005159,-54.0321044593028,4.77941132465054));
#40167=CARTESIAN_POINT('Ctrl Pts',(30.1187333412011,-55.8142597516569,4.89054921521859));
#40168=CARTESIAN_POINT('Ctrl Pts',(30.8074500449804,-58.0333768894161,5.00168710578662));
#40169=CARTESIAN_POINT('Ctrl Pts',(33.045376938239,-58.6582727998918,5.11282499635468));
#40170=CARTESIAN_POINT('Ctrl Pts',(34.7841140934679,-57.1169731495113,5.22396288692271));
#40171=CARTESIAN_POINT('Ctrl Pts',(34.4321757978777,-54.8202470274371,5.33510077749076));
#40172=CARTESIAN_POINT('Ctrl Pts',(32.3116949177892,-53.8703138209288,5.44623866805879));
#40173=CARTESIAN_POINT('Ctrl Pts',(30.3635721421369,-55.1366583239951,5.55737655862685));
#40174=CARTESIAN_POINT('Ctrl Pts',(30.370945362205,-57.4601807388668,5.66851444919488));
#40175=CARTESIAN_POINT('Ctrl Pts',(32.3270677340268,-58.7141352713797,5.77965233976293));
#40176=CARTESIAN_POINT('Ctrl Pts',(34.4414743886772,-57.7507618774265,5.89079023033096));
#40177=CARTESIAN_POINT('Ctrl Pts',(34.7788326566388,-55.451849617872,6.00192812089901));
#40178=CARTESIAN_POINT('Ctrl Pts',(33.0303393193103,-53.921614042038,6.11306601146705));
#40179=CARTESIAN_POINT('Ctrl Pts',(30.7964407564499,-54.5607069079647,6.22420390203509));
#40180=CARTESIAN_POINT('Ctrl Pts',(30.1217887402557,-56.7841397946826,6.33534179260313));
#40181=CARTESIAN_POINT('Ctrl Pts',(31.6240211855661,-58.5568181325984,6.44647968317118));
#40182=CARTESIAN_POINT('Ctrl Pts',(33.9278862659327,-58.2561121571832,6.55761757373921));
#40183=CARTESIAN_POINT('Ctrl Pts',(34.9251107981772,-56.157415110224,6.66875546430726));
#40184=CARTESIAN_POINT('Ctrl Pts',(33.7019669024841,-54.1813822458926,6.7798933548753));
#40185=CARTESIAN_POINT('Ctrl Pts',(31.3799180340502,-54.1373087230551,6.89103124544333));
#40186=CARTESIAN_POINT('Ctrl Pts',(30.0805564955408,-56.0643114795338,7.00216913601139));
#40187=CARTESIAN_POINT('Ctrl Pts',(31.0009129766989,-58.2011370798035,7.11330702657942));
#40188=CARTESIAN_POINT('Ctrl Pts',(32.5211546805143,-58.4569191413475,7.18739895362479));
#40189=CARTESIAN_POINT('Ctrl Pts',(33.1673657555108,-58.2350041503452,7.22444491714747));
#40190=CARTESIAN_POINT('Ctrl Pts',(31.1375785572409,-57.6518256858141,-2.07481497238249));
#40191=CARTESIAN_POINT('Ctrl Pts',(31.5898689183853,-58.1048632288923,-2.03776900885981));
#40192=CARTESIAN_POINT('Ctrl Pts',(32.974462612681,-58.516147898041,-1.96367708181445));
#40193=CARTESIAN_POINT('Ctrl Pts',(34.6294912924535,-57.0974392229326,-1.85253919124641));
#40194=CARTESIAN_POINT('Ctrl Pts',(34.3303034137843,-54.940512314437,-1.74140130067836));
#40195=CARTESIAN_POINT('Ctrl Pts',(32.3582893241016,-54.0206552913481,-1.63026341011032));
#40196=CARTESIAN_POINT('Ctrl Pts',(30.5147494765408,-55.1792854513053,-1.51912551954228));
#40197=CARTESIAN_POINT('Ctrl Pts',(30.4889518873457,-57.3561677789084,-1.40798762897424));
#40198=CARTESIAN_POINT('Ctrl Pts',(32.3035780800887,-58.5586402598713,-1.2968497384062));
#40199=CARTESIAN_POINT('Ctrl Pts',(34.2981478804346,-57.6861349893711,-1.18571184783816));
#40200=CARTESIAN_POINT('Ctrl Pts',(34.6467739743846,-55.5372313797063,-1.07457395727011));
#40201=CARTESIAN_POINT('Ctrl Pts',(33.0304729643073,-54.0788626331851,-0.963436066702072));
#40202=CARTESIAN_POINT('Ctrl Pts',(30.9286042125635,-54.6458814833823,-0.852298176134029));
#40203=CARTESIAN_POINT('Ctrl Pts',(30.2650618023749,-56.7192935259745,-0.741160285565989));
#40204=CARTESIAN_POINT('Ctrl Pts',(31.6471786691815,-58.4012790043313,-0.630022394997946));
#40205=CARTESIAN_POINT('Ctrl Pts',(33.8098950838865,-58.152298640154,-0.518884504429905));
#40206=CARTESIAN_POINT('Ctrl Pts',(34.7736484112179,-56.2002464293262,-0.407746613861864));
#40207=CARTESIAN_POINT('Ctrl Pts',(33.6563061966827,-54.3318581770161,-0.296608723293821));
#40208=CARTESIAN_POINT('Ctrl Pts',(31.4805834885329,-54.2572906994736,-0.185470832725779));
#40209=CARTESIAN_POINT('Ctrl Pts',(30.2379444342266,-56.044796524896,-0.0743329421577373));
#40210=CARTESIAN_POINT('Ctrl Pts',(31.0657904123944,-58.0582512642421,0.0368049484103042));
#40211=CARTESIAN_POINT('Ctrl Pts',(33.2063847314925,-58.4547169782088,0.147942838978346));
#40212=CARTESIAN_POINT('Ctrl Pts',(34.7004170746387,-56.8713040936593,0.259080729546388));
#40213=CARTESIAN_POINT('Ctrl Pts',(34.1803827251225,-54.7573283854238,0.370218620114429));
#40214=CARTESIAN_POINT('Ctrl Pts',(32.1222750053512,-54.0477357911158,0.481356510682471));
#40215=CARTESIAN_POINT('Ctrl Pts',(30.4099032594437,-55.3920244607626,0.592494401250513));
#40216=CARTESIAN_POINT('Ctrl Pts',(30.6106207621861,-57.5597517291987,0.703632291818554));
#40217=CARTESIAN_POINT('Ctrl Pts',(32.5407085089656,-58.5667722442102,0.814770182386597));
#40218=CARTESIAN_POINT('Ctrl Pts',(34.4335352954974,-57.4913487078745,0.925908072954637));
#40219=CARTESIAN_POINT('Ctrl Pts',(34.5565752984423,-55.3178284792041,1.03704596352268));
#40220=CARTESIAN_POINT('Ctrl Pts',(32.7972086074906,-54.0356592728607,1.14818385409072));
#40221=CARTESIAN_POINT('Ctrl Pts',(30.7658035075691,-54.8184251042163,1.25932174465876));
#40222=CARTESIAN_POINT('Ctrl Pts',(30.3217281242748,-56.9496515306538,1.37045963522681));
#40223=CARTESIAN_POINT('Ctrl Pts',(31.8714496921253,-58.4786028343079,1.48159752579484));
#40224=CARTESIAN_POINT('Ctrl Pts',(33.9964904850136,-58.0058125474547,1.59273541636289));
#40225=CARTESIAN_POINT('Ctrl Pts',(34.7517765656152,-55.9640309814584,1.70387330693093));
#40226=CARTESIAN_POINT('Ctrl Pts',(33.4459860188247,-54.2221239590531,1.81501119749897));
#40227=CARTESIAN_POINT('Ctrl Pts',(31.2743237407935,-54.3744787324154,1.92614908806701));
#40228=CARTESIAN_POINT('Ctrl Pts',(30.2245368429278,-56.2816432496664,2.03728697863506));
#40229=CARTESIAN_POINT('Ctrl Pts',(31.2575071782378,-58.1979681994494,2.1484248692031));
#40230=CARTESIAN_POINT('Ctrl Pts',(33.4277452841336,-58.3694196226251,2.25956275977114));
#40231=CARTESIAN_POINT('Ctrl Pts',(34.7488076101148,-56.6390660871692,2.37070065033918));
#40232=CARTESIAN_POINT('Ctrl Pts',(34.011510827345,-54.5907198076285,2.48183854090722));
#40233=CARTESIAN_POINT('Ctrl Pts',(31.8907110426077,-54.0992553634931,2.59297643147526));
#40234=CARTESIAN_POINT('Ctrl Pts',(30.3276003503782,-55.6145157340663,2.70411432204331));
#40235=CARTESIAN_POINT('Ctrl Pts',(30.7529116941352,-57.7495659179407,2.81525221261135));
#40236=CARTESIAN_POINT('Ctrl Pts',(32.7773527775791,-58.5501702687006,2.92639010317939));
#40237=CARTESIAN_POINT('Ctrl Pts',(34.5479297183105,-57.2835265446242,3.03752799374743));
#40238=CARTESIAN_POINT('Ctrl Pts',(34.4440133627694,-55.1090081110757,3.14866588431547));
#40239=CARTESIAN_POINT('Ctrl Pts',(32.5607195296748,-54.0169763509983,3.25980377488351));
#40240=CARTESIAN_POINT('Ctrl Pts',(30.6218484224618,-55.0069803188731,3.37094166545156));
#40241=CARTESIAN_POINT('Ctrl Pts',(30.4020707538584,-57.1728581554963,3.4820795560196));
#40242=CARTESIAN_POINT('Ctrl Pts',(32.1025515163817,-58.5321573142802,3.59321744658764));
#40243=CARTESIAN_POINT('Ctrl Pts',(34.1668213833381,-57.8406958596913,3.70435533715568));
#40244=CARTESIAN_POINT('Ctrl Pts',(34.705430735075,-55.7313763028164,3.81549322772372));
#40245=CARTESIAN_POINT('Ctrl Pts',(33.225384323732,-54.1348827553833,3.92663111829177));
#40246=CARTESIAN_POINT('Ctrl Pts',(31.0813854144196,-54.5125038668067,4.0377690088598));
#40247=CARTESIAN_POINT('Ctrl Pts',(30.2358605235516,-56.5185987513242,4.14890689942785));
#40248=CARTESIAN_POINT('Ctrl Pts',(31.4627281724074,-58.3169660103977,4.26004478999589));
#40249=CARTESIAN_POINT('Ctrl Pts',(33.6390224888347,-58.2615396970763,4.37118268056394));
#40250=CARTESIAN_POINT('Ctrl Pts',(34.772756603214,-56.4030521442201,4.48232057113197));
#40251=CARTESIAN_POINT('Ctrl Pts',(33.8262108251008,-54.4425980862378,4.59345846170002));
#40252=CARTESIAN_POINT('Ctrl Pts',(31.6657692360459,-54.1746033542736,4.70459635226805));
#40253=CARTESIAN_POINT('Ctrl Pts',(30.2689085309822,-55.8443665681263,4.81573424283611));
#40254=CARTESIAN_POINT('Ctrl Pts',(30.9141911400063,-57.923534517046,4.92687213340413));
#40255=CARTESIAN_POINT('Ctrl Pts',(33.0109826023927,-58.5090212073899,5.03801002397219));
#40256=CARTESIAN_POINT('Ctrl Pts',(34.6400658550227,-57.0649240129586,5.14914791454022));
#40257=CARTESIAN_POINT('Ctrl Pts',(34.3103226378947,-54.9130415101336,5.26028580510828));
#40258=CARTESIAN_POINT('Ctrl Pts',(32.3235704258736,-54.0230160838143,5.3714236956763));
#40259=CARTESIAN_POINT('Ctrl Pts',(30.498306510429,-55.2094982474935,5.48256158624436));
#40260=CARTESIAN_POINT('Ctrl Pts',(30.505214736491,-57.3864871280696,5.59369947681239));
#40261=CARTESIAN_POINT('Ctrl Pts',(32.3379737515305,-58.5613606978516,5.70483736738043));
#40262=CARTESIAN_POINT('Ctrl Pts',(34.3190348106915,-57.6587426929399,5.81597525794847));
#40263=CARTESIAN_POINT('Ctrl Pts',(34.6351174933556,-55.5048119219529,5.92711314851652));
#40264=CARTESIAN_POINT('Ctrl Pts',(32.9968933347409,-54.0710810433821,6.03825103908455));
#40265=CARTESIAN_POINT('Ctrl Pts',(30.9038761550678,-54.669869354557,6.1493889296526));
#40266=CARTESIAN_POINT('Ctrl Pts',(30.2717712405153,-56.7530808786254,6.26052682022064));
#40267=CARTESIAN_POINT('Ctrl Pts',(31.6792650131381,-58.4139648045911,6.37166471078869));
#40268=CARTESIAN_POINT('Ctrl Pts',(33.8378362540284,-58.1322229282863,6.48280260135672));
#40269=CARTESIAN_POINT('Ctrl Pts',(34.7721705665526,-56.1658807463968,6.59394049192477));
#40270=CARTESIAN_POINT('Ctrl Pts',(33.6261645529135,-54.3144668991412,6.70507838249281));
#40271=CARTESIAN_POINT('Ctrl Pts',(31.4505562891928,-54.2731728842735,6.81621627306085));
#40272=CARTESIAN_POINT('Ctrl Pts',(30.2331393178401,-56.0786487199456,6.9273541636289));
#40273=CARTESIAN_POINT('Ctrl Pts',(31.0954532825444,-58.080714868197,7.03849205419693));
#40274=CARTESIAN_POINT('Ctrl Pts',(32.5198205551868,-58.3203659687278,7.1125839812423));
#40275=CARTESIAN_POINT('Ctrl Pts',(33.1252781637591,-58.1124461032886,7.14962994476498));
#40276=CARTESIAN_POINT('Ctrl Pts',(31.2292834028599,-57.5602720863886,-2.14962994476498));
#40277=CARTESIAN_POINT('Ctrl Pts',(31.6511300140441,-57.982815586549,-2.1125839812423));
#40278=CARTESIAN_POINT('Ctrl Pts',(32.9425264442662,-58.3664166066402,-2.03849205419693));
#40279=CARTESIAN_POINT('Ctrl Pts',(34.4861548298198,-57.0432014814319,-1.9273541636289));
#40280=CARTESIAN_POINT('Ctrl Pts',(34.2071053439879,-55.0314577320876,-1.81621627306085));
#40281=CARTESIAN_POINT('Ctrl Pts',(32.3678278965638,-54.1735164596221,-1.70507838249281));
#40282=CARTESIAN_POINT('Ctrl Pts',(30.6483770656663,-55.2541590038433,-1.59394049192477));
#40283=CARTESIAN_POINT('Ctrl Pts',(30.6243159170911,-57.2845149692516,-1.48280260135673));
#40284=CARTESIAN_POINT('Ctrl Pts',(32.3167992767584,-58.4060487995394,-1.37166471078869));
#40285=CARTESIAN_POINT('Ctrl Pts',(34.1771142056845,-57.5922720242183,-1.26052682022064));
#40286=CARTESIAN_POINT('Ctrl Pts',(34.5022742111534,-55.5880115239392,-1.1493889296526));
#40287=CARTESIAN_POINT('Ctrl Pts',(32.9947667285052,-54.2278058542443,-1.03825103908456));
#40288=CARTESIAN_POINT('Ctrl Pts',(31.034375160943,-54.7566585581314,-0.927113148516519));
#40289=CARTESIAN_POINT('Ctrl Pts',(30.4154959161878,-56.6905088430302,-0.815975257948477));
#40290=CARTESIAN_POINT('Ctrl Pts',(31.7045822346487,-58.2592795599446,-0.704837367380435));
#40291=CARTESIAN_POINT('Ctrl Pts',(33.7217257974419,-58.0270581112851,-0.593699476812394));
#40292=CARTESIAN_POINT('Ctrl Pts',(34.6206087055887,-56.2063989048656,-0.482561586244352));
#40293=CARTESIAN_POINT('Ctrl Pts',(33.5784750073553,-54.4637722200536,-0.37142369567631));
#40294=CARTESIAN_POINT('Ctrl Pts',(31.549200607195,-54.394223893562,-0.260285805108268));
#40295=CARTESIAN_POINT('Ctrl Pts',(30.3902038232309,-56.061412362975,-0.149147914540226));
#40296=CARTESIAN_POINT('Ctrl Pts',(31.1623273316536,-57.9393410820767,-0.0380100239721848));
#40297=CARTESIAN_POINT('Ctrl Pts',(33.1588378412894,-58.3091206136688,0.0731278665958572));
#40298=CARTESIAN_POINT('Ctrl Pts',(34.5523065841589,-56.8322875505839,0.184265757163899));
#40299=CARTESIAN_POINT('Ctrl Pts',(34.067275845304,-54.8606039480667,0.295403647731941));
#40300=CARTESIAN_POINT('Ctrl Pts',(32.1476997463554,-54.1987741658161,0.406541538299982));
#40301=CARTESIAN_POINT('Ctrl Pts',(30.5505880673203,-55.45257851024,0.517679428868024));
#40302=CARTESIAN_POINT('Ctrl Pts',(30.7377952368983,-57.4743956452496,0.628817319436067));
#40303=CARTESIAN_POINT('Ctrl Pts',(32.537968411509,-58.4136334184707,0.739955210004107));
#40304=CARTESIAN_POINT('Ctrl Pts',(34.3033886681708,-57.4105968442596,0.85109310057215));
#40305=CARTESIAN_POINT('Ctrl Pts',(34.4181468251899,-55.3833766742673,0.96223099114019));
#40306=CARTESIAN_POINT('Ctrl Pts',(32.7772034397714,-54.1875105202945,1.07336888170823));
#40307=CARTESIAN_POINT('Ctrl Pts',(30.8825326022678,-54.9175882351338,1.18450677227627));
#40308=CARTESIAN_POINT('Ctrl Pts',(30.4683480172171,-56.9053614067402,1.29564466284432));
#40309=CARTESIAN_POINT('Ctrl Pts',(31.9137575325176,-58.3313987082653,1.40678255341236));
#40310=CARTESIAN_POINT('Ctrl Pts',(33.8957614267418,-57.8904320252583,1.5179204439804));
#40311=CARTESIAN_POINT('Ctrl Pts',(34.6002090580603,-55.9860831635788,1.62905833454844));
#40312=CARTESIAN_POINT('Ctrl Pts',(33.3823115205444,-54.3614242331065,1.74019622511649));
#40313=CARTESIAN_POINT('Ctrl Pts',(31.3568242421815,-54.5035239777884,1.85133411568452));
#40314=CARTESIAN_POINT('Ctrl Pts',(30.3776986994444,-56.2823168897962,1.96247200625257));
#40315=CARTESIAN_POINT('Ctrl Pts',(31.3411396056397,-58.0696536438858,2.07360989682061));
#40316=CARTESIAN_POINT('Ctrl Pts',(33.3652985731636,-58.2295646392613,2.18474778738865));
#40317=CARTESIAN_POINT('Ctrl Pts',(34.5974399435176,-56.6156815283417,2.29588567795669));
#40318=CARTESIAN_POINT('Ctrl Pts',(33.9097707469831,-54.7052098252309,2.40702356852473));
#40319=CARTESIAN_POINT('Ctrl Pts',(31.9317223978473,-54.246825946009,2.51816145909278));
#40320=CARTESIAN_POINT('Ctrl Pts',(30.4738249826682,-55.6600938537545,2.62929934966082));
#40321=CARTESIAN_POINT('Ctrl Pts',(30.8705085392404,-57.6514334049599,2.74043724022886));
#40322=CARTESIAN_POINT('Ctrl Pts',(32.7586841095359,-58.3981489250802,2.8515751307969));
#40323=CARTESIAN_POINT('Ctrl Pts',(34.4100831806958,-57.2167632302196,2.96271302136494));
#40324=CARTESIAN_POINT('Ctrl Pts',(34.3131614547482,-55.1886120447087,3.07385091193298));
#40325=CARTESIAN_POINT('Ctrl Pts',(32.5566324866203,-54.1700851494448,3.18498880250103));
#40326=CARTESIAN_POINT('Ctrl Pts',(30.7482671612322,-55.0934517625431,3.29612669306907));
#40327=CARTESIAN_POINT('Ctrl Pts',(30.5432827691709,-57.1135439513458,3.40726458363711));
#40328=CARTESIAN_POINT('Ctrl Pts',(32.1293038491678,-58.381348426037,3.51840247420515));
#40329=CARTESIAN_POINT('Ctrl Pts',(34.0546273200064,-57.7364293730534,3.6295403647732));
#40330=CARTESIAN_POINT('Ctrl Pts',(34.5569827741607,-55.769088515466,3.74067825534123));
#40331=CARTESIAN_POINT('Ctrl Pts',(33.1765585673731,-54.2800552513963,3.85181614590928));
#40332=CARTESIAN_POINT('Ctrl Pts',(31.1768726311357,-54.6322586142151,3.96295403647731));
#40333=CARTESIAN_POINT('Ctrl Pts',(30.3882601809785,-56.5033228717122,4.07409192704536));
#40334=CARTESIAN_POINT('Ctrl Pts',(31.5325471357831,-58.1806416896178,4.1852298176134));
#40335=CARTESIAN_POINT('Ctrl Pts',(33.5623546691594,-58.1289461319546,4.29636770818144));
#40336=CARTESIAN_POINT('Ctrl Pts',(34.6197769253507,-56.3955537286392,4.40750559874948));
#40337=CARTESIAN_POINT('Ctrl Pts',(33.7369433230217,-54.5670582049899,4.51864348931753));
#40338=CARTESIAN_POINT('Ctrl Pts',(31.7219214669328,-54.3171022492445,4.62978137988556));
#40339=CARTESIAN_POINT('Ctrl Pts',(30.4190837207633,-55.8744733845957,4.74091927045362));
#40340=CARTESIAN_POINT('Ctrl Pts',(31.0209322350323,-57.8136921446758,4.85205716102165));
#40341=CARTESIAN_POINT('Ctrl Pts',(32.9765882665465,-58.3597696148881,4.9631950515897));
#40342=CARTESIAN_POINT('Ctrl Pts',(34.4960176165775,-57.012874876406,5.07433294215773));
#40343=CARTESIAN_POINT('Ctrl Pts',(34.1884694779118,-55.0058359928302,5.18547083272578));
#40344=CARTESIAN_POINT('Ctrl Pts',(32.335445933958,-54.1757183466998,5.29660872329381));
#40345=CARTESIAN_POINT('Ctrl Pts',(30.633040878721,-55.2823381709919,5.40774661386187));
#40346=CARTESIAN_POINT('Ctrl Pts',(30.6394841107771,-57.3127935172724,5.5188845044299));
#40347=CARTESIAN_POINT('Ctrl Pts',(32.3488797690342,-58.4085861243234,5.63002239499795));
#40348=CARTESIAN_POINT('Ctrl Pts',(34.1965952327058,-57.5667235084533,5.74116028556598));
#40349=CARTESIAN_POINT('Ctrl Pts',(34.4914023300724,-55.5577742260338,5.85229817613403));
#40350=CARTESIAN_POINT('Ctrl Pts',(32.9634473501715,-54.2205480447262,5.96343606670206));
#40351=CARTESIAN_POINT('Ctrl Pts',(31.0113115536856,-54.7790318011494,6.07457395727011));
#40352=CARTESIAN_POINT('Ctrl Pts',(30.421753740775,-56.7220219625684,6.18571184783815));
#40353=CARTESIAN_POINT('Ctrl Pts',(31.7345088407102,-58.2711114765836,6.2968497384062));
#40354=CARTESIAN_POINT('Ctrl Pts',(33.747786242124,-58.0083336993896,6.40798762897423));
#40355=CARTESIAN_POINT('Ctrl Pts',(34.6192303349282,-56.1743463825696,6.51912551954228));
#40356=CARTESIAN_POINT('Ctrl Pts',(33.5503622033428,-54.4475515523897,6.63026341011032));
#40357=CARTESIAN_POINT('Ctrl Pts',(31.5211945443355,-54.4090370454918,6.74140130067836));
#40358=CARTESIAN_POINT('Ctrl Pts',(30.3857221401394,-56.0929859603577,6.85253919124641));
#40359=CARTESIAN_POINT('Ctrl Pts',(31.18999358839,-57.9602926565904,6.96367708181444));
#40360=CARTESIAN_POINT('Ctrl Pts',(32.5184864298593,-58.1838127961081,7.03776900885981));
#40361=CARTESIAN_POINT('Ctrl Pts',(33.0831905720075,-57.989888056232,7.07481497238249));
#40362=CARTESIAN_POINT('Ctrl Pts',(31.3209882484789,-57.468718486963,-2.22444491714747));
#40363=CARTESIAN_POINT('Ctrl Pts',(31.712391109703,-57.8607679442057,-2.18739895362479));
#40364=CARTESIAN_POINT('Ctrl Pts',(32.9105902758514,-58.2166853152393,-2.11330702657942));
#40365=CARTESIAN_POINT('Ctrl Pts',(34.342818367186,-56.9889637399312,-2.00216913601138));
#40366=CARTESIAN_POINT('Ctrl Pts',(34.0839072741917,-55.1224031497381,-1.89103124544334));
#40367=CARTESIAN_POINT('Ctrl Pts',(32.377366469026,-54.3263776278961,-1.7798933548753));
#40368=CARTESIAN_POINT('Ctrl Pts',(30.7820046547919,-55.3290325563813,-1.66875546430726));
#40369=CARTESIAN_POINT('Ctrl Pts',(30.7596799468364,-57.2128621595949,-1.55761757373921));
#40370=CARTESIAN_POINT('Ctrl Pts',(32.330020473428,-58.2534573392076,-1.44647968317118));
#40371=CARTESIAN_POINT('Ctrl Pts',(34.0560805309345,-57.4984090590655,-1.33534179260313));
#40372=CARTESIAN_POINT('Ctrl Pts',(34.3577744479221,-55.6387916681722,-1.22420390203509));
#40373=CARTESIAN_POINT('Ctrl Pts',(32.9590604927032,-54.3767490753035,-1.11306601146705));
#40374=CARTESIAN_POINT('Ctrl Pts',(31.1401461093225,-54.8674356328804,-1.00192812089901));
#40375=CARTESIAN_POINT('Ctrl Pts',(30.5659300300008,-56.6617241600859,-0.890790230330966));
#40376=CARTESIAN_POINT('Ctrl Pts',(31.7619858001159,-58.1172801155578,-0.779652339762924));
#40377=CARTESIAN_POINT('Ctrl Pts',(33.6335565109972,-57.9018175824163,-0.668514449194882));
#40378=CARTESIAN_POINT('Ctrl Pts',(34.4675689999596,-56.2125513804049,-0.557376558626841));
#40379=CARTESIAN_POINT('Ctrl Pts',(33.5006438180279,-54.595686263091,-0.446238668058798));
#40380=CARTESIAN_POINT('Ctrl Pts',(31.617817725857,-54.5311570876504,-0.335100777490757));
#40381=CARTESIAN_POINT('Ctrl Pts',(30.5424632122353,-56.0780282010539,-0.223962886922715));
#40382=CARTESIAN_POINT('Ctrl Pts',(31.2588642509128,-57.8204308999114,-0.112824996354674));
#40383=CARTESIAN_POINT('Ctrl Pts',(33.1112909510864,-58.1635242491288,-0.00168710578663179));
#40384=CARTESIAN_POINT('Ctrl Pts',(34.4041960936791,-56.7932710075085,0.10945078478141));
#40385=CARTESIAN_POINT('Ctrl Pts',(33.9541689654856,-54.9638795107098,0.220588675349452));
#40386=CARTESIAN_POINT('Ctrl Pts',(32.1731244873596,-54.3498125405165,0.331726565917493));
#40387=CARTESIAN_POINT('Ctrl Pts',(30.6912728751969,-55.5131325597174,0.442864456485535));
#40388=CARTESIAN_POINT('Ctrl Pts',(30.8649697116104,-57.3890395613005,0.554002347053577));
#40389=CARTESIAN_POINT('Ctrl Pts',(32.5352283140525,-58.2604945927311,0.665140237621618));
#40390=CARTESIAN_POINT('Ctrl Pts',(34.1732420408443,-57.3298449806446,0.776278128189661));
#40391=CARTESIAN_POINT('Ctrl Pts',(34.2797183519374,-55.4489248693306,0.887416018757702));
#40392=CARTESIAN_POINT('Ctrl Pts',(32.7571982720523,-54.3393617677281,0.998553909325745));
#40393=CARTESIAN_POINT('Ctrl Pts',(30.9992616969666,-55.0167513660514,1.10969179989379));
#40394=CARTESIAN_POINT('Ctrl Pts',(30.6149679101593,-56.8610712828264,1.22082969046183));
#40395=CARTESIAN_POINT('Ctrl Pts',(31.9560653729101,-58.1841945822227,1.33196758102987));
#40396=CARTESIAN_POINT('Ctrl Pts',(33.7950323684699,-57.775051503062,1.44310547159791));
#40397=CARTESIAN_POINT('Ctrl Pts',(34.4486415505055,-56.0081353456992,1.55424336216595));
#40398=CARTESIAN_POINT('Ctrl Pts',(33.318637022264,-54.5007245071601,1.665381252734));
#40399=CARTESIAN_POINT('Ctrl Pts',(31.4393247435695,-54.6325692231613,1.77651914330203));
#40400=CARTESIAN_POINT('Ctrl Pts',(30.5308605559611,-56.2829905299262,1.88765703387008));
#40401=CARTESIAN_POINT('Ctrl Pts',(31.4247720330417,-57.9413390883221,1.99879492443811));
#40402=CARTESIAN_POINT('Ctrl Pts',(33.3028518621937,-58.0897096558975,2.10993281500617));
#40403=CARTESIAN_POINT('Ctrl Pts',(34.4460722769204,-56.592296969514,2.2210707055742));
#40404=CARTESIAN_POINT('Ctrl Pts',(33.8080306666211,-54.8196998428333,2.33220859614224));
#40405=CARTESIAN_POINT('Ctrl Pts',(31.9727337530869,-54.3943965285248,2.44334648671029));
#40406=CARTESIAN_POINT('Ctrl Pts',(30.6200496149581,-55.7056719734428,2.55448437727833));
#40407=CARTESIAN_POINT('Ctrl Pts',(30.9881053843455,-57.5533008919789,2.66562226784637));
#40408=CARTESIAN_POINT('Ctrl Pts',(32.7400154414926,-58.2461275814599,2.77676015841441));
#40409=CARTESIAN_POINT('Ctrl Pts',(34.2722366430812,-57.1499999158147,2.88789804898245));
#40410=CARTESIAN_POINT('Ctrl Pts',(34.182309546727,-55.2682159783418,2.9990359395505));
#40411=CARTESIAN_POINT('Ctrl Pts',(32.5525454435658,-54.3231939478911,3.11017383011853));
#40412=CARTESIAN_POINT('Ctrl Pts',(30.8746859000024,-55.1799232062132,3.22131172068658));
#40413=CARTESIAN_POINT('Ctrl Pts',(30.6844947844835,-57.0542297471953,3.33244961125462));
#40414=CARTESIAN_POINT('Ctrl Pts',(32.156056181954,-58.2305395377939,3.44358750182266));
#40415=CARTESIAN_POINT('Ctrl Pts',(33.9424332566746,-57.6321628864156,3.55472539239071));
#40416=CARTESIAN_POINT('Ctrl Pts',(34.4085348132464,-55.8068007281157,3.66586328295874));
#40417=CARTESIAN_POINT('Ctrl Pts',(33.1277328110142,-54.4252277474093,3.77700117352679));
#40418=CARTESIAN_POINT('Ctrl Pts',(31.2723598478519,-54.7520133616234,3.88813906409483));
#40419=CARTESIAN_POINT('Ctrl Pts',(30.5406598384055,-56.4880469921002,3.99927695466287));
#40420=CARTESIAN_POINT('Ctrl Pts',(31.6023660991588,-58.044317368838,4.11041484523091));
#40421=CARTESIAN_POINT('Ctrl Pts',(33.4856868494842,-57.9963525668329,4.22155273579896));
#40422=CARTESIAN_POINT('Ctrl Pts',(34.4667972474874,-56.3880553130583,4.332690626367));
#40423=CARTESIAN_POINT('Ctrl Pts',(33.6476758209426,-54.6915183237421,4.44382851693504));
#40424=CARTESIAN_POINT('Ctrl Pts',(31.7780736978196,-54.4596011442154,4.55496640750308));
#40425=CARTESIAN_POINT('Ctrl Pts',(30.5692589105444,-55.904580201065,4.66610429807113));
#40426=CARTESIAN_POINT('Ctrl Pts',(31.1276733300582,-57.7038497723057,4.77724218863916));
#40427=CARTESIAN_POINT('Ctrl Pts',(32.9421939307002,-58.2105180223861,4.8883800792072));
#40428=CARTESIAN_POINT('Ctrl Pts',(34.3519693781324,-56.9608257398534,4.99951796977525));
#40429=CARTESIAN_POINT('Ctrl Pts',(34.0666163179288,-55.0986304755266,5.11065586034329));
#40430=CARTESIAN_POINT('Ctrl Pts',(32.3473214420424,-54.3284206095853,5.22179375091132));
#40431=CARTESIAN_POINT('Ctrl Pts',(30.7677752470131,-55.3551780944903,5.33293164147938));
#40432=CARTESIAN_POINT('Ctrl Pts',(30.7737534850632,-57.2390999064753,5.44406953204741));
#40433=CARTESIAN_POINT('Ctrl Pts',(32.3597857865378,-58.2558115507953,5.55520742261546));
#40434=CARTESIAN_POINT('Ctrl Pts',(34.0741556547201,-57.4747043239667,5.6663453131835));
#40435=CARTESIAN_POINT('Ctrl Pts',(34.3476871667892,-55.6107365301146,5.77748320375153));
#40436=CARTESIAN_POINT('Ctrl Pts',(32.9300013656021,-54.3700150460704,5.88862109431958));
#40437=CARTESIAN_POINT('Ctrl Pts',(31.1187469523034,-54.8881942477417,5.99975898488762));
#40438=CARTESIAN_POINT('Ctrl Pts',(30.5717362410347,-56.6909630465113,6.11089687545566));
#40439=CARTESIAN_POINT('Ctrl Pts',(31.7897526682823,-58.1282581485763,6.2220347660237));
#40440=CARTESIAN_POINT('Ctrl Pts',(33.6577362302197,-57.8844444704929,6.33317265659175));
#40441=CARTESIAN_POINT('Ctrl Pts',(34.4662901033037,-56.1828120187425,6.44431054715979));
#40442=CARTESIAN_POINT('Ctrl Pts',(33.4745598537722,-54.5806362056383,6.55544843772783));
#40443=CARTESIAN_POINT('Ctrl Pts',(31.5918327994781,-54.5449012067101,6.66658632829587));
#40444=CARTESIAN_POINT('Ctrl Pts',(30.5383049624387,-56.1073232007697,6.77772421886392));
#40445=CARTESIAN_POINT('Ctrl Pts',(31.2845338942354,-57.8398704449839,6.88886210943196));
#40446=CARTESIAN_POINT('Ctrl Pts',(32.5171523045318,-58.0472596234885,6.96295403647732));
#40447=CARTESIAN_POINT('Ctrl Pts',(33.0411029802559,-57.8673300091754,7.));
#40448=CARTESIAN_POINT('Ctrl Pts',(33.3327354544031,-57.732107437543,-1.3785196366098));
#40449=CARTESIAN_POINT('Ctrl Pts',(33.5202555818621,-57.6251326319318,-1.36412702194091));
#40450=CARTESIAN_POINT('Ctrl Pts',(33.6873867521344,-57.4836168424902,-1.34973440727202));
#40451=CARTESIAN_POINT('Ctrl Pts',(33.8186861741813,-57.3143142072736,-1.33534179260314));
#40452=CARTESIAN_POINT('Ctrl Pts',(34.1566451699303,-56.8785365954344,-1.29829582908045));
#40453=CARTESIAN_POINT('Ctrl Pts',(34.2572098089262,-56.2586641318033,-1.26124986555777));
#40454=CARTESIAN_POINT('Ctrl Pts',(34.0743731358877,-55.7383874678429,-1.22420390203509));
#40455=CARTESIAN_POINT('Ctrl Pts',(33.8915364628492,-55.2181108038826,-1.18715793851241));
#40456=CARTESIAN_POINT('Ctrl Pts',(33.4252984777762,-54.7974299395931,-1.15011197498973));
#40457=CARTESIAN_POINT('Ctrl Pts',(32.8890270880096,-54.6688706003778,-1.11306601146705));
#40458=CARTESIAN_POINT('Ctrl Pts',(32.352755698243,-54.5403112611625,-1.07602004794437));
#40459=CARTESIAN_POINT('Ctrl Pts',(31.7464509037828,-54.7038734470215,-1.03897408442169));
#40460=CARTESIAN_POINT('Ctrl Pts',(31.3475958266657,-55.0847026278185,-1.00192812089901));
#40461=CARTESIAN_POINT('Ctrl Pts',(30.9487407495486,-55.4655318086156,-0.96488215737633));
#40462=CARTESIAN_POINT('Ctrl Pts',(30.7573353897747,-56.0636279843508,-0.92783619385365));
#40463=CARTESIAN_POINT('Ctrl Pts',(30.8609753382403,-56.6052687314637,-0.890790230330969));
#40464=CARTESIAN_POINT('Ctrl Pts',(30.9646152867058,-57.1469094785766,-0.853744266808289));
#40465=CARTESIAN_POINT('Ctrl Pts',(31.3633005434108,-57.6320947970672,-0.816698303285608));
#40466=CARTESIAN_POINT('Ctrl Pts',(31.8745716235769,-57.8387770341222,-0.779652339762927));
#40467=CARTESIAN_POINT('Ctrl Pts',(32.3398155301954,-58.0268527049873,-0.745941438711884));
#40468=CARTESIAN_POINT('Ctrl Pts',(32.8982866368193,-57.9843126404343,-0.712230537660842));
#40469=CARTESIAN_POINT('Ctrl Pts',(33.3348489584778,-57.7359240281238,-0.678519636609799));
#40470=CARTESIAN_POINT('Ctrl Pts',(31.0458737116219,-57.7433792852397,-2.));
#40471=CARTESIAN_POINT('Ctrl Pts',(31.1022242475563,-57.7901329641036,-2.));
#40472=CARTESIAN_POINT('Ctrl Pts',(31.1610916221591,-57.8334666739877,-2.));
#40473=CARTESIAN_POINT('Ctrl Pts',(31.2221267441933,-57.8733637960044,-2.));
#40474=CARTESIAN_POINT('Ctrl Pts',(31.2848602944917,-57.9143711378001,-2.));
#40475=CARTESIAN_POINT('Ctrl Pts',(31.3498848969714,-57.9517482942034,-2.));
#40476=CARTESIAN_POINT('Ctrl Pts',(31.4168445551513,-57.9854278643729,-2.));
#40477=CARTESIAN_POINT('Ctrl Pts',(31.473423951905,-58.0138863394445,-2.));
#40478=CARTESIAN_POINT('Ctrl Pts',(31.5313856959209,-58.0397039720774,-2.));
#40479=CARTESIAN_POINT('Ctrl Pts',(31.5905192436884,-58.0628113946307,-2.));
#40480=CARTESIAN_POINT('Ctrl Pts',(31.6167907197732,-58.0730774131922,-2.));
#40481=CARTESIAN_POINT('Ctrl Pts',(31.6432934887176,-58.0828081409933,-2.));
#40482=CARTESIAN_POINT('Ctrl Pts',(31.6700089381818,-58.0919957886044,-2.));
#40483=CARTESIAN_POINT('Ctrl Pts',(31.6846879641888,-58.0970440180347,-2.));
#40484=CARTESIAN_POINT('Ctrl Pts',(31.6994311962746,-58.1019282705386,-2.));
#40485=CARTESIAN_POINT('Ctrl Pts',(31.7142355159248,-58.1066471169474,-2.));
#40486=CARTESIAN_POINT('Ctrl Pts',(31.7278877153664,-58.1109987274118,-2.));
#40487=CARTESIAN_POINT('Ctrl Pts',(31.7415938959754,-58.1152101596109,-2.));
#40488=CARTESIAN_POINT('Ctrl Pts',(31.7553302775603,-58.1192742594955,-2.));
#40489=CARTESIAN_POINT('Ctrl Pts',(31.8255274332676,-58.1400430660875,-2.));
#40490=CARTESIAN_POINT('Ctrl Pts',(31.8966328017476,-58.1570081793249,-2.));
#40491=CARTESIAN_POINT('Ctrl Pts',(31.9683123621892,-58.17010995281,-2.));
#40492=CARTESIAN_POINT('Ctrl Pts',(32.0394355875868,-58.1831100379521,-2.));
#40493=CARTESIAN_POINT('Ctrl Pts',(32.111125145623,-58.1923065191828,-2.));
#40494=CARTESIAN_POINT('Ctrl Pts',(32.1830533294046,-58.197590217694,-2.));
#40495=CARTESIAN_POINT('Ctrl Pts',(32.2428321680026,-58.2019814499467,-2.));
#40496=CARTESIAN_POINT('Ctrl Pts',(32.3027760709051,-58.203669194572,-2.));
#40497=CARTESIAN_POINT('Ctrl Pts',(32.3626887230984,-58.202563625202,-2.));
#40498=CARTESIAN_POINT('Ctrl Pts',(32.3876963771293,-58.2021021584617,-2.));
#40499=CARTESIAN_POINT('Ctrl Pts',(32.4126984595008,-58.2011537302573,-2.));
#40500=CARTESIAN_POINT('Ctrl Pts',(32.4376800452417,-58.1997105189462,-2.));
#40501=CARTESIAN_POINT('Ctrl Pts',(32.4492432419533,-58.1990425014528,-2.));
#40502=CARTESIAN_POINT('Ctrl Pts',(32.4608020410722,-58.1982684671836,-2.));
#40503=CARTESIAN_POINT('Ctrl Pts',(32.4723549281396,-58.1973875849089,-2.));
#40504=CARTESIAN_POINT('Ctrl Pts',(32.4844044306918,-58.1964688367937,-2.));
#40505=CARTESIAN_POINT('Ctrl Pts',(32.4964392274972,-58.1954344592285,-2.));
#40506=CARTESIAN_POINT('Ctrl Pts',(32.5084532356254,-58.1942844547156,-2.));
#40507=CARTESIAN_POINT('Ctrl Pts',(32.5768783070893,-58.1877346721503,-2.));
#40508=CARTESIAN_POINT('Ctrl Pts',(32.6446774036362,-58.1774344901189,-2.));
#40509=CARTESIAN_POINT('Ctrl Pts',(32.7115617527762,-58.1632926068254,-2.));
#40510=CARTESIAN_POINT('Ctrl Pts',(32.7721836417612,-58.150474844672,-2.));
#40511=CARTESIAN_POINT('Ctrl Pts',(32.832054420019,-58.1345005317109,-2.));
#40512=CARTESIAN_POINT('Ctrl Pts',(32.8909448795168,-58.115267443086,-2.));
#40513=CARTESIAN_POINT('Ctrl Pts',(32.9606152109761,-58.0925137462918,-2.));
#40514=CARTESIAN_POINT('Ctrl Pts',(33.0289150978522,-58.0651988064951,-2.));
#40515=CARTESIAN_POINT('Ctrl Pts',(33.0955156401826,-58.0335993051752,-2.));
#40516=CARTESIAN_POINT('Ctrl Pts',(33.1101787046012,-58.0266422218357,-2.));
#40517=CARTESIAN_POINT('Ctrl Pts',(33.1247592149198,-58.0194773027427,-2.));
#40518=CARTESIAN_POINT('Ctrl Pts',(33.1392533337009,-58.0121072627471,-2.));
#40519=CARTESIAN_POINT('Ctrl Pts',(33.1542086549699,-58.0045027082679,-2.));
#40520=CARTESIAN_POINT('Ctrl Pts',(33.1690773275608,-57.9966767059944,-2.));
#40521=CARTESIAN_POINT('Ctrl Pts',(33.1838253280879,-57.9886488037404,-2.));
#40522=CARTESIAN_POINT('Ctrl Pts',(33.244061954076,-57.9558596982169,-2.));
#40523=CARTESIAN_POINT('Ctrl Pts',(33.3023667325498,-57.9196691076173,-2.));
#40524=CARTESIAN_POINT('Ctrl Pts',(33.3585069616667,-57.8803506668589,-2.));
#40525=CARTESIAN_POINT('Ctrl Pts',(33.414635850494,-57.8410401683998,-2.));
#40526=CARTESIAN_POINT('Ctrl Pts',(33.4686017655928,-57.7986021545391,-2.));
#40527=CARTESIAN_POINT('Ctrl Pts',(33.5201343260522,-57.7532746488578,-2.));
#40528=CARTESIAN_POINT('Ctrl Pts',(33.5574338655248,-57.7204663608107,-2.));
#40529=CARTESIAN_POINT('Ctrl Pts',(33.5934578302879,-57.6861435081566,-2.));
#40530=CARTESIAN_POINT('Ctrl Pts',(33.6280882155819,-57.6503888642621,-2.));
#40531=CARTESIAN_POINT('Ctrl Pts',(33.6540651537304,-57.6235685974622,-2.));
#40532=CARTESIAN_POINT('Ctrl Pts',(33.6792576937978,-57.5959425522059,-2.));
#40533=CARTESIAN_POINT('Ctrl Pts',(33.7036104502874,-57.5675443623166,-2.));
#40534=CARTESIAN_POINT('Ctrl Pts',(33.7117026688617,-57.5581078798471,-2.));
#40535=CARTESIAN_POINT('Ctrl Pts',(33.7196957778872,-57.5485935241117,-2.));
#40536=CARTESIAN_POINT('Ctrl Pts',(33.7275879316751,-57.5390030774457,-2.));
#40537=CARTESIAN_POINT('Ctrl Pts',(33.7694510935145,-57.4881314862826,-2.));
#40538=CARTESIAN_POINT('Ctrl Pts',(33.80847982562,-57.4351175563013,-2.));
#40539=CARTESIAN_POINT('Ctrl Pts',(33.8444097934509,-57.380171662872,-2.));
#40540=CARTESIAN_POINT('Ctrl Pts',(33.8696919535248,-57.3415089265284,-2.));
#40541=CARTESIAN_POINT('Ctrl Pts',(33.8934389529984,-57.3018891510446,-2.));
#40542=CARTESIAN_POINT('Ctrl Pts',(33.9155436487628,-57.2613822920818,-2.));
#40543=CARTESIAN_POINT('Ctrl Pts',(33.9226388854396,-57.2483802695959,-2.));
#40544=CARTESIAN_POINT('Ctrl Pts',(33.9295657377069,-57.2352850255039,-2.));
#40545=CARTESIAN_POINT('Ctrl Pts',(33.9363174100524,-57.2221046384035,-2.));
#40546=CARTESIAN_POINT('Ctrl Pts',(33.965080442193,-57.1659544168891,-2.));
#40547=CARTESIAN_POINT('Ctrl Pts',(33.9906110255055,-57.1083731117427,-2.));
#40548=CARTESIAN_POINT('Ctrl Pts',(34.0126532831744,-57.0495480070032,-2.));
#40549=CARTESIAN_POINT('Ctrl Pts',(34.0329745304529,-56.9953158354375,-2.));
#40550=CARTESIAN_POINT('Ctrl Pts',(34.0503306992963,-56.9400259525623,-2.));
#40551=CARTESIAN_POINT('Ctrl Pts',(34.064482015077,-56.8838229928238,-2.));
#40552=CARTESIAN_POINT('Ctrl Pts',(34.0671303463503,-56.8733049563224,-2.));
#40553=CARTESIAN_POINT('Ctrl Pts',(34.0696663195691,-56.8627549469952,-2.));
#40554=CARTESIAN_POINT('Ctrl Pts',(34.0720901513885,-56.8521746541717,-2.));
#40555=CARTESIAN_POINT('Origin',(32.5,-56.2916512459885,3.));
#40556=CARTESIAN_POINT('Origin',(-32.5,-56.2916512459885,7.));
#40557=CARTESIAN_POINT('Ctrl Pts',(-33.5940263469955,-57.5480995545471,
7.));
#40558=CARTESIAN_POINT('Ctrl Pts',(-33.6455781063537,-57.5127482049916,
7.));
#40559=CARTESIAN_POINT('Ctrl Pts',(-33.6948218851486,-57.4743678095888,
7.));
#40560=CARTESIAN_POINT('Ctrl Pts',(-33.7416962543705,-57.4332901552822,
7.));
#40561=CARTESIAN_POINT('Ctrl Pts',(-33.7714300137986,-57.4072334187053,
7.));
#40562=CARTESIAN_POINT('Ctrl Pts',(-33.8002101105626,-57.3800903099151,
7.));
#40563=CARTESIAN_POINT('Ctrl Pts',(-33.8280169255491,-57.3519357930303,
7.));
#40564=CARTESIAN_POINT('Ctrl Pts',(-33.8470314135077,-57.3326835441645,
7.));
#40565=CARTESIAN_POINT('Ctrl Pts',(-33.865590736976,-57.3129582161004,7.));
#40566=CARTESIAN_POINT('Ctrl Pts',(-33.88368758978,-57.2927820234305,7.));
#40567=CARTESIAN_POINT('Ctrl Pts',(-33.8932692324261,-57.2820994439668,
7.));
#40568=CARTESIAN_POINT('Ctrl Pts',(-33.9027209649851,-57.2712905501713,
7.));
#40569=CARTESIAN_POINT('Ctrl Pts',(-33.9120326400169,-57.2603695730079,
7.));
#40570=CARTESIAN_POINT('Ctrl Pts',(-33.954835257131,-57.2101695389172,7.));
#40571=CARTESIAN_POINT('Ctrl Pts',(-33.9947314176855,-57.1575493212694,
7.));
#40572=CARTESIAN_POINT('Ctrl Pts',(-34.0316365850473,-57.1028515989214,
7.));
#40573=CARTESIAN_POINT('Ctrl Pts',(-34.0582554670344,-57.0633993400583,
7.));
#40574=CARTESIAN_POINT('Ctrl Pts',(-34.0833178684594,-57.0228651370504,
7.));
#40575=CARTESIAN_POINT('Ctrl Pts',(-34.1067823366534,-56.981363974441,7.));
#40576=CARTESIAN_POINT('Ctrl Pts',(-34.1132255641423,-56.9699679594307,
7.));
#40577=CARTESIAN_POINT('Ctrl Pts',(-34.1195482496941,-56.9584989762171,
7.));
#40578=CARTESIAN_POINT('Ctrl Pts',(-34.1257494077654,-56.9469592829674,
7.));
#40579=CARTESIAN_POINT('Ctrl Pts',(-34.1320583289994,-56.9352190539746,
7.));
#40580=CARTESIAN_POINT('Ctrl Pts',(-34.1382375551786,-56.9234128304559,
7.));
#40581=CARTESIAN_POINT('Ctrl Pts',(-34.1442842647394,-56.9115477362169,
7.));
#40582=CARTESIAN_POINT('Ctrl Pts',(-34.1750933788667,-56.851092865867,7.));
#40583=CARTESIAN_POINT('Ctrl Pts',(-34.2024838356472,-56.7890775491619,
7.));
#40584=CARTESIAN_POINT('Ctrl Pts',(-34.2263706778433,-56.7258494467084,
7.));
#40585=CARTESIAN_POINT('Ctrl Pts',(-34.2506031310785,-56.6617065171708,
7.));
#40586=CARTESIAN_POINT('Ctrl Pts',(-34.2712305305178,-56.5963146349483,
7.));
#40587=CARTESIAN_POINT('Ctrl Pts',(-34.2881270714822,-56.5299991241842,
7.));
#40588=CARTESIAN_POINT('Ctrl Pts',(-34.2985953641524,-56.4889131896894,
7.));
#40589=CARTESIAN_POINT('Ctrl Pts',(-34.3076308154854,-56.4474720283024,
7.));
#40590=CARTESIAN_POINT('Ctrl Pts',(-34.3151947514507,-56.4057480909205,
7.));
#40591=CARTESIAN_POINT('Ctrl Pts',(-34.3213914047069,-56.3715663139163,
7.));
#40592=CARTESIAN_POINT('Ctrl Pts',(-34.3266003410262,-56.3371946653748,
7.));
#40593=CARTESIAN_POINT('Ctrl Pts',(-34.3307964558649,-56.3026718438894,
7.));
#40594=CARTESIAN_POINT('Ctrl Pts',(-34.3325110301801,-56.2885654751929,
7.));
#40595=CARTESIAN_POINT('Ctrl Pts',(-34.334056573613,-56.274431305155,7.));
#40596=CARTESIAN_POINT('Ctrl Pts',(-34.3354292580426,-56.2602960059048,
7.));
#40597=CARTESIAN_POINT('Ctrl Pts',(-34.3422420688138,-56.1901406833092,
7.));
#40598=CARTESIAN_POINT('Ctrl Pts',(-34.344817121763,-56.1198364598138,7.));
#40599=CARTESIAN_POINT('Ctrl Pts',(-34.3430393002911,-56.0497278067116,
7.));
#40600=CARTESIAN_POINT('Ctrl Pts',(-34.3428417470506,-56.0419372654097,
7.));
#40601=CARTESIAN_POINT('Ctrl Pts',(-34.3425903992471,-56.0341491124172,
7.));
#40602=CARTESIAN_POINT('Ctrl Pts',(-34.3422850635953,-56.0263638020432,
7.));
#40603=CARTESIAN_POINT('Ctrl Pts',(-34.3396426913258,-55.9589897888101,
7.));
#40604=CARTESIAN_POINT('Ctrl Pts',(-34.3329614085342,-55.8918294784485,
7.));
#40605=CARTESIAN_POINT('Ctrl Pts',(-34.3224781325168,-55.8251283238202,
7.));
#40606=CARTESIAN_POINT('Ctrl Pts',(-34.311200007843,-55.7533698452166,7.));
#40607=CARTESIAN_POINT('Ctrl Pts',(-34.2955218532054,-55.682141849139,7.));
#40608=CARTESIAN_POINT('Ctrl Pts',(-34.275674530723,-55.6117461590084,7.));
#40609=CARTESIAN_POINT('Ctrl Pts',(-34.2720417381032,-55.5988611492648,
7.));
#40610=CARTESIAN_POINT('Ctrl Pts',(-34.2682690985559,-55.5860040383836,
7.));
#40611=CARTESIAN_POINT('Ctrl Pts',(-34.2643578043072,-55.5731767072662,
7.));
#40612=CARTESIAN_POINT('Ctrl Pts',(-34.260994380672,-55.5621461516716,7.));
#40613=CARTESIAN_POINT('Ctrl Pts',(-34.2575311418944,-55.5511465602876,
7.));
#40614=CARTESIAN_POINT('Ctrl Pts',(-34.2539698127282,-55.5401805087525,
7.));
#40615=CARTESIAN_POINT('Ctrl Pts',(-34.2320182882534,-55.4725873328828,
7.));
#40616=CARTESIAN_POINT('Ctrl Pts',(-34.2063390660098,-55.4062514121211,
7.));
#40617=CARTESIAN_POINT('Ctrl Pts',(-34.1772031614855,-55.3414402692491,
7.));
#40618=CARTESIAN_POINT('Ctrl Pts',(-34.1474529585405,-55.2752626548922,
7.));
#40619=CARTESIAN_POINT('Ctrl Pts',(-34.1140985516191,-55.2106738831258,
7.));
#40620=CARTESIAN_POINT('Ctrl Pts',(-34.0773733357091,-55.1479588367781,
7.));
#40621=CARTESIAN_POINT('Ctrl Pts',(-34.0404255621234,-55.0848637323531,
7.));
#40622=CARTESIAN_POINT('Ctrl Pts',(-34.0000656101091,-55.023664132488,7.));
#40623=CARTESIAN_POINT('Ctrl Pts',(-33.9564808025865,-54.9646647046815,
7.));
#40624=CARTESIAN_POINT('Ctrl Pts',(-33.9457092805123,-54.9500836229904,
7.));
#40625=CARTESIAN_POINT('Ctrl Pts',(-33.9347405679519,-54.9356370335807,
7.));
#40626=CARTESIAN_POINT('Ctrl Pts',(-33.9235770661179,-54.9213297828376,
7.));
#40627=CARTESIAN_POINT('Ctrl Pts',(-33.9148444639817,-54.9101379964017,
7.));
#40628=CARTESIAN_POINT('Ctrl Pts',(-33.9059915496783,-54.8990302862249,
7.));
#40629=CARTESIAN_POINT('Ctrl Pts',(-33.8970332940984,-54.8880255398733,
7.));
#40630=CARTESIAN_POINT('Ctrl Pts',(-33.8494695086148,-54.8295959282035,
7.));
#40631=CARTESIAN_POINT('Ctrl Pts',(-33.7988575668702,-54.7739598965231,
7.));
#40632=CARTESIAN_POINT('Ctrl Pts',(-33.7454538506294,-54.7214122178979,
7.));
#40633=CARTESIAN_POINT('Ctrl Pts',(-33.6919920462483,-54.6688073822592,
7.));
#40634=CARTESIAN_POINT('Ctrl Pts',(-33.635731898188,-54.6192966067788,7.));
#40635=CARTESIAN_POINT('Ctrl Pts',(-33.576882466568,-54.5731951202712,7.));
#40636=CARTESIAN_POINT('Ctrl Pts',(-33.5193724814535,-54.5281429297942,
7.));
#40637=CARTESIAN_POINT('Ctrl Pts',(-33.4593891253538,-54.4863457606538,
7.));
#40638=CARTESIAN_POINT('Ctrl Pts',(-33.3970899730292,-54.4481299156499,
7.));
#40639=CARTESIAN_POINT('Ctrl Pts',(-33.3836932591,-54.4399120390982,7.));
#40640=CARTESIAN_POINT('Ctrl Pts',(-33.3701893374023,-54.4318599153431,
7.));
#40641=CARTESIAN_POINT('Ctrl Pts',(-33.356579582449,-54.4239770468377,7.));
#40642=CARTESIAN_POINT('Ctrl Pts',(-33.3450551424613,-54.417302007843,7.));
#40643=CARTESIAN_POINT('Ctrl Pts',(-33.3334548151719,-54.4107483324245,
7.));
#40644=CARTESIAN_POINT('Ctrl Pts',(-33.3217804591138,-54.404315872452,7.));
#40645=CARTESIAN_POINT('Ctrl Pts',(-32.2716262263503,-54.2496319067047,
7.));
#40646=CARTESIAN_POINT('Ctrl Pts',(-32.1985421824115,-54.2648284787439,
7.));
#40647=CARTESIAN_POINT('Ctrl Pts',(-32.1265185433228,-54.2843049160509,
7.));
#40648=CARTESIAN_POINT('Ctrl Pts',(-32.0558148702163,-54.307809841484,7.));
#40649=CARTESIAN_POINT('Ctrl Pts',(-31.9869629438687,-54.3306991670822,
7.));
#40650=CARTESIAN_POINT('Ctrl Pts',(-31.9193621916132,-54.3574095812673,
7.));
#40651=CARTESIAN_POINT('Ctrl Pts',(-31.8532778586781,-54.3877469743477,
7.));
#40652=CARTESIAN_POINT('Ctrl Pts',(-31.8385281517267,-54.3945181353435,
7.));
#40653=CARTESIAN_POINT('Ctrl Pts',(-31.8238521663117,-54.4014710566228,
7.));
#40654=CARTESIAN_POINT('Ctrl Pts',(-31.8092592837343,-54.4086007385189,
7.));
#40655=CARTESIAN_POINT('Ctrl Pts',(-31.74229379234,-54.4413182396107,7.));
#40656=CARTESIAN_POINT('Ctrl Pts',(-31.6772081432285,-54.4776886923633,
7.));
#40657=CARTESIAN_POINT('Ctrl Pts',(-31.6142783994125,-54.5174808471838,
7.));
#40658=CARTESIAN_POINT('Ctrl Pts',(-31.5700975698183,-54.5454175636663,
7.));
#40659=CARTESIAN_POINT('Ctrl Pts',(-31.5269799619039,-54.5750417875592,
7.));
#40660=CARTESIAN_POINT('Ctrl Pts',(-31.4850325697142,-54.606283716683,7.));
#40661=CARTESIAN_POINT('Ctrl Pts',(-31.4690843649994,-54.6181617537992,
7.));
#40662=CARTESIAN_POINT('Ctrl Pts',(-31.4533054231774,-54.6302737016023,
7.));
#40663=CARTESIAN_POINT('Ctrl Pts',(-31.4377020509801,-54.6426159725235,
7.));
#40664=CARTESIAN_POINT('Ctrl Pts',(-31.422843222849,-54.6543693089207,7.));
#40665=CARTESIAN_POINT('Ctrl Pts',(-31.4081391340328,-54.6663354489501,
7.));
#40666=CARTESIAN_POINT('Ctrl Pts',(-31.3936208031221,-54.6784895996313,
7.));
#40667=CARTESIAN_POINT('Ctrl Pts',(-31.3379553553305,-54.7250904275332,
7.));
#40668=CARTESIAN_POINT('Ctrl Pts',(-31.2849558324703,-54.7744982188797,
7.));
#40669=CARTESIAN_POINT('Ctrl Pts',(-31.2348792620953,-54.8265005113965,
7.));
#40670=CARTESIAN_POINT('Ctrl Pts',(-31.1858781211836,-54.8773860182167,
7.));
#40671=CARTESIAN_POINT('Ctrl Pts',(-31.1396752549576,-54.9307565896498,
7.));
#40672=CARTESIAN_POINT('Ctrl Pts',(-31.096553263537,-54.9864387998288,7.));
#40673=CARTESIAN_POINT('Ctrl Pts',(-31.0543769959251,-55.0408998235516,
7.));
#40674=CARTESIAN_POINT('Ctrl Pts',(-31.0151475676859,-55.0975728716759,
7.));
#40675=CARTESIAN_POINT('Ctrl Pts',(-30.9791760532886,-55.1563097700977,
7.));
#40676=CARTESIAN_POINT('Ctrl Pts',(-30.9674871681193,-55.1753962298242,
7.));
#40677=CARTESIAN_POINT('Ctrl Pts',(-30.9561426884338,-55.1947006860194,
7.));
#40678=CARTESIAN_POINT('Ctrl Pts',(-30.9451544835008,-55.2142182090111,
7.));
#40679=CARTESIAN_POINT('Ctrl Pts',(-30.9389559540756,-55.2252281911972,
7.));
#40680=CARTESIAN_POINT('Ctrl Pts',(-30.9328702747781,-55.2363071797393,
7.));
#40681=CARTESIAN_POINT('Ctrl Pts',(-30.9269078406191,-55.2474384074061,
7.));
#40682=CARTESIAN_POINT('Ctrl Pts',(-30.8946567103501,-55.3076478225486,
7.));
#40683=CARTESIAN_POINT('Ctrl Pts',(-30.8659479672295,-55.3694877086145,
7.));
#40684=CARTESIAN_POINT('Ctrl Pts',(-30.8410371126545,-55.4327943978594,
7.));
#40685=CARTESIAN_POINT('Ctrl Pts',(-30.8374416946983,-55.4419315395249,
7.));
#40686=CARTESIAN_POINT('Ctrl Pts',(-30.8339254773263,-55.4510992635148,
7.));
#40687=CARTESIAN_POINT('Ctrl Pts',(-30.8304893165615,-55.4602971020131,
7.));
#40688=CARTESIAN_POINT('Ctrl Pts',(-30.8062112767693,-55.5252840174526,
7.));
#40689=CARTESIAN_POINT('Ctrl Pts',(-30.7859254272784,-55.5917741517056,
7.));
#40690=CARTESIAN_POINT('Ctrl Pts',(-30.7695892422356,-55.6594016433948,
7.));
#40691=CARTESIAN_POINT('Ctrl Pts',(-30.7543489013014,-55.722492629887,7.));
#40692=CARTESIAN_POINT('Ctrl Pts',(-30.7425467760704,-55.7865743173994,
7.));
#40693=CARTESIAN_POINT('Ctrl Pts',(-30.7341878976062,-55.8513431276971,
7.));
#40694=CARTESIAN_POINT('Ctrl Pts',(-30.7323430806796,-55.8656377005953,
7.));
#40695=CARTESIAN_POINT('Ctrl Pts',(-30.7306661227298,-55.8799656907132,
7.));
#40696=CARTESIAN_POINT('Ctrl Pts',(-30.7291573147787,-55.8943237313175,
7.));
#40697=CARTESIAN_POINT('Ctrl Pts',(-30.7279778703852,-55.9055474993793,
7.));
#40698=CARTESIAN_POINT('Ctrl Pts',(-30.7269013312117,-55.9167889366509,
7.));
#40699=CARTESIAN_POINT('Ctrl Pts',(-30.725928716623,-55.9280334133084,7.));
#40700=CARTESIAN_POINT('Ctrl Pts',(-30.7200365397427,-55.9961533512166,
7.));
#40701=CARTESIAN_POINT('Ctrl Pts',(-30.717940322368,-56.064510368579,7.));
#40702=CARTESIAN_POINT('Ctrl Pts',(-30.7195810692414,-56.1327563913084,
7.));
#40703=CARTESIAN_POINT('Ctrl Pts',(-30.7212142395892,-56.20068727235,7.));
#40704=CARTESIAN_POINT('Ctrl Pts',(-30.7265502690067,-56.2685092688714,
7.));
#40705=CARTESIAN_POINT('Ctrl Pts',(-30.7355805426345,-56.3358665624723,
7.));
#40706=CARTESIAN_POINT('Ctrl Pts',(-30.7444173748262,-56.4017809660634,
7.));
#40707=CARTESIAN_POINT('Ctrl Pts',(-30.7567922827294,-56.4672512454211,
7.));
#40708=CARTESIAN_POINT('Ctrl Pts',(-30.7727391547474,-56.5319175326533,
7.));
#40709=CARTESIAN_POINT('Ctrl Pts',(-30.7760991368497,-56.5455426227323,
7.));
#40710=CARTESIAN_POINT('Ctrl Pts',(-30.7796178313477,-56.559131898849,7.));
#40711=CARTESIAN_POINT('Ctrl Pts',(-30.7832957741898,-56.5726817853209,
7.));
#40712=CARTESIAN_POINT('Ctrl Pts',(-30.7867820846143,-56.5855256799889,
7.));
#40713=CARTESIAN_POINT('Ctrl Pts',(-30.7904121023242,-56.5983358602818,
7.));
#40714=CARTESIAN_POINT('Ctrl Pts',(-30.7941799173868,-56.6110887258481,
7.));
#40715=CARTESIAN_POINT('Ctrl Pts',(-30.81269457301,-56.6737549953548,7.));
#40716=CARTESIAN_POINT('Ctrl Pts',(-30.8345622313403,-56.7351520397333,
7.));
#40717=CARTESIAN_POINT('Ctrl Pts',(-30.8597663049837,-56.7949606498833,
7.));
#40718=CARTESIAN_POINT('Ctrl Pts',(-30.8844910319696,-56.8536317829029,
7.));
#40719=CARTESIAN_POINT('Ctrl Pts',(-30.9124268768218,-56.9107751110263,
7.));
#40720=CARTESIAN_POINT('Ctrl Pts',(-30.9435976955084,-56.9660591310642,
7.));
#40721=CARTESIAN_POINT('Ctrl Pts',(-30.9737560234748,-57.0195474152303,
7.));
#40722=CARTESIAN_POINT('Ctrl Pts',(-31.0069429902717,-57.0712957444527,
7.));
#40723=CARTESIAN_POINT('Ctrl Pts',(-31.0432115502758,-57.1209660579171,
7.));
#40724=CARTESIAN_POINT('Ctrl Pts',(-31.0492497804945,-57.1292355008643,
7.));
#40725=CARTESIAN_POINT('Ctrl Pts',(-31.0553734904689,-57.1374472482072,
7.));
#40726=CARTESIAN_POINT('Ctrl Pts',(-31.0615830007349,-57.1455996184163,
7.));
#40727=CARTESIAN_POINT('Ctrl Pts',(-31.0681540675972,-57.1542266707015,
7.));
#40728=CARTESIAN_POINT('Ctrl Pts',(-31.0748212184917,-57.1627872296296,
7.));
#40729=CARTESIAN_POINT('Ctrl Pts',(-31.0815830733445,-57.1712803260695,
7.));
#40730=CARTESIAN_POINT('Origin',(-32.5,-56.2916512459885,-3.54592528053767));
#40731=CARTESIAN_POINT('Ctrl Pts',(-33.5269872402601,-58.0734398505124,
-1.79592528053768));
#40732=CARTESIAN_POINT('Ctrl Pts',(-33.4422748054587,-58.1232938101479,
-1.79058130531689));
#40733=CARTESIAN_POINT('Ctrl Pts',(-32.7422362990183,-58.4684621317491,
-1.74819136657341));
#40734=CARTESIAN_POINT('Ctrl Pts',(-31.092918091713,-58.2713739433871,-1.66875546430726));
#40735=CARTESIAN_POINT('Ctrl Pts',(-30.0738503853478,-56.1831963302234,
-1.55761757373922));
#40736=CARTESIAN_POINT('Ctrl Pts',(-31.2751851021384,-54.1944751483927,
-1.44647968317117));
#40737=CARTESIAN_POINT('Ctrl Pts',(-33.5977473666623,-54.1252293793916,
-1.33534179260314));
#40738=CARTESIAN_POINT('Ctrl Pts',(-34.9154583912003,-56.0389811637256,
-1.22420390203509));
#40739=CARTESIAN_POINT('Ctrl Pts',(-34.2741084270659,-57.5792551456252,
-1.14439839801327));
#40740=CARTESIAN_POINT('Ctrl Pts',(-33.6210824061175,-58.0199411501776,
-1.10163885751414));
#40741=CARTESIAN_POINT('Ctrl Pts',(-33.5295799600393,-58.0717283210701,
-1.09592528053768));
#40742=CARTESIAN_POINT('Ctrl Pts',(-33.5283546803393,-58.0681541983481,
-1.85407471946233));
#40743=CARTESIAN_POINT('Ctrl Pts',(-33.1193657433931,-58.3001842134597,
-1.82862455259619));
#40744=CARTESIAN_POINT('Ctrl Pts',(-31.9170343357855,-58.5410390719136,
-1.76612842220737));
#40745=CARTESIAN_POINT('Ctrl Pts',(-30.2743670907292,-57.2623912321518,
-1.66658632829588));
#40746=CARTESIAN_POINT('Ctrl Pts',(-30.4765028746714,-54.9487367869862,
-1.55544843772783));
#40747=CARTESIAN_POINT('Ctrl Pts',(-32.5312595152503,-53.8630292597193,
-1.44431054715979));
#40748=CARTESIAN_POINT('Ctrl Pts',(-34.5571577499755,-55.0008883544571,
-1.33317265659175));
#40749=CARTESIAN_POINT('Ctrl Pts',(-34.6817103419943,-57.0195698185232,
-1.23642738069259));
#40750=CARTESIAN_POINT('Ctrl Pts',(-33.8868873402924,-57.8579713309385,
-1.17672806831612));
#40751=CARTESIAN_POINT('Ctrl Pts',(-33.5250365419916,-58.0693901510839,
-1.15407471946233));
#40752=CARTESIAN_POINT('Ctrl Pts',(-30.9307125467393,-55.7322829513575,
-2.));
#40753=CARTESIAN_POINT('Ctrl Pts',(-31.116715812632,-55.2104575382394,-1.96295403647732));
#40754=CARTESIAN_POINT('Ctrl Pts',(-32.0473824090187,-54.3760622611663,
-1.88886210943196));
#40755=CARTESIAN_POINT('Ctrl Pts',(-33.8672110770871,-54.8728632770319,
-1.77772421886392));
#40756=CARTESIAN_POINT('Ctrl Pts',(-34.4318965215284,-56.6706982888813,
-1.66658632829587));
#40757=CARTESIAN_POINT('Ctrl Pts',(-33.2300975250658,-58.1203931132112,
-1.55544843772783));
#40758=CARTESIAN_POINT('Ctrl Pts',(-31.359132031047,-57.8968187913668,-1.44431054715979));
#40759=CARTESIAN_POINT('Ctrl Pts',(-30.5328676198999,-56.2037155410781,
-1.33317265659175));
#40760=CARTESIAN_POINT('Ctrl Pts',(-31.5069148948352,-54.5912519864218,
-1.22203476602371));
#40761=CARTESIAN_POINT('Ctrl Pts',(-33.3900582128529,-54.5351072237228,
-1.11089687545567));
#40762=CARTESIAN_POINT('Ctrl Pts',(-34.4584638908576,-56.0867852734615,
-0.999758984887624));
#40763=CARTESIAN_POINT('Ctrl Pts',(-33.7342941276566,-57.8259603059919,
-0.888621094319583));
#40764=CARTESIAN_POINT('Ctrl Pts',(-31.8803464986039,-58.1607744839985,
-0.777483203751541));
#40765=CARTESIAN_POINT('Ctrl Pts',(-30.5935820077056,-56.7847541278006,
-0.6663453131835));
#40766=CARTESIAN_POINT('Ctrl Pts',(-31.0517798775847,-54.9573935418363,
-0.555207422615458));
#40767=CARTESIAN_POINT('Ctrl Pts',(-32.8355518820609,-54.3512929431319,
-0.444069532047416));
#40768=CARTESIAN_POINT('Ctrl Pts',(-34.3121885227868,-55.5212249175371,
-0.332931641479374));
#40769=CARTESIAN_POINT('Ctrl Pts',(-34.1301089195294,-57.3963365394661,
-0.221793750911332));
#40770=CARTESIAN_POINT('Ctrl Pts',(-32.4559719031607,-58.2603173390955,
-0.110655860343291));
#40771=CARTESIAN_POINT('Ctrl Pts',(-30.8221344198831,-57.3223556597407,
0.000482030224751014));
#40772=CARTESIAN_POINT('Ctrl Pts',(-30.724066271727,-55.4409785805667,0.111619920792793));
#40773=CARTESIAN_POINT('Ctrl Pts',(-32.2515304349823,-54.3382318197086,
0.222757811360835));
#40774=CARTESIAN_POINT('Ctrl Pts',(-34.0064215941321,-55.0234720228687,
0.333895701928876));
#40775=CARTESIAN_POINT('Ctrl Pts',(-34.3824679916267,-56.8694910461268,
0.445033592496918));
#40776=CARTESIAN_POINT('Ctrl Pts',(-33.0354700840103,-58.1866067496581,
0.55617148306496));
#40777=CARTESIAN_POINT('Ctrl Pts',(-31.1983503377325,-57.7692481891733,
0.667309373633001));
#40778=CARTESIAN_POINT('Ctrl Pts',(-30.5526452880963,-55.9994283901304,
0.778447264201044));
#40779=CARTESIAN_POINT('Ctrl Pts',(-31.6893760912439,-54.4970834847716,
0.889585154769084));
#40780=CARTESIAN_POINT('Ctrl Pts',(-33.5680801509383,-54.6373268031956,
1.00072304533713));
#40781=CARTESIAN_POINT('Ctrl Pts',(-34.4691583357458,-56.2917920453437,
1.11186093590517));
#40782=CARTESIAN_POINT('Ctrl Pts',(-33.5678435640106,-57.9461284122851,
1.22299882647321));
#40783=CARTESIAN_POINT('Ctrl Pts',(-31.6891194679972,-58.0861030658479,
1.33413671704125));
#40784=CARTESIAN_POINT('Ctrl Pts',(-30.5526035189214,-56.5835956182358,
1.44527460760929));
#40785=CARTESIAN_POINT('Ctrl Pts',(-31.1985616539627,-54.8138681758263,
1.55641249817734));
#40786=CARTESIAN_POINT('Ctrl Pts',(-33.0357410664429,-54.3967723367386,
1.66755038874538));
#40787=CARTESIAN_POINT('Ctrl Pts',(-34.3825506050928,-55.7140806526746,
1.77868827931342));
#40788=CARTESIAN_POINT('Ctrl Pts',(-34.0062402253245,-57.5600458827673,
1.88982616988146));
#40789=CARTESIAN_POINT('Ctrl Pts',(-32.2512510853912,-58.2450351172427,
2.0009640604495));
#40790=CARTESIAN_POINT('Ctrl Pts',(-30.7239446480037,-57.1420699414794,
2.11210195101754));
#40791=CARTESIAN_POINT('Ctrl Pts',(-30.8222818161361,-55.2607068893292,
2.22323984158559));
#40792=CARTESIAN_POINT('Ctrl Pts',(-32.4562534645774,-54.3229788985336,
2.33437773215363));
#40793=CARTESIAN_POINT('Ctrl Pts',(-34.1302668130106,-55.1871990336263,
2.44551562272167));
#40794=CARTESIAN_POINT('Ctrl Pts',(-34.3120784590119,-57.0623368040342,
2.55665351328971));
#40795=CARTESIAN_POINT('Ctrl Pts',(-32.8352741411123,-58.2320573429941,
2.66779140385776));
#40796=CARTESIAN_POINT('Ctrl Pts',(-31.0515895995852,-57.6257021756631,
2.77892929442579));
#40797=CARTESIAN_POINT('Ctrl Pts',(-30.593651523649,-55.7982750632342,2.89006718499384));
#40798=CARTESIAN_POINT('Ctrl Pts',(-31.8806158275789,-54.4224407661471,
3.00120507556188));
#40799=CARTESIAN_POINT('Ctrl Pts',(-33.7345094888202,-54.7575160195471,
3.11234296612992));
#40800=CARTESIAN_POINT('Ctrl Pts',(-34.4584426146545,-56.4968026439861,
3.22348085669796));
#40801=CARTESIAN_POINT('Ctrl Pts',(-33.3897910050459,-58.0483118672624,
3.334618747266));
#40802=CARTESIAN_POINT('Ctrl Pts',(-31.506703597602,-57.9919297020008,3.44575663783404));
#40803=CARTESIAN_POINT('Ctrl Pts',(-30.5327916520213,-56.3792633834812,
3.55689452840209));
#40804=CARTESIAN_POINT('Ctrl Pts',(-31.3594878170038,-54.6864046819268,
3.66803241897013));
#40805=CARTESIAN_POINT('Ctrl Pts',(-33.230107717374,-54.4628463651893,3.77917030953817));
#40806=CARTESIAN_POINT('Ctrl Pts',(-34.4324517440405,-55.9132138959114,
3.89030820010621));
#40807=CARTESIAN_POINT('Ctrl Pts',(-33.8660007739066,-57.7099694249181,
4.00144609067425));
#40808=CARTESIAN_POINT('Ctrl Pts',(-32.0492338038872,-58.2085222399532,
4.1125839812423));
#40809=CARTESIAN_POINT('Ctrl Pts',(-30.6450582452589,-56.9525412953674,
4.22372187181033));
#40810=CARTESIAN_POINT('Ctrl Pts',(-30.9387319111105,-55.0916401936805,
4.33485976237839));
#40811=CARTESIAN_POINT('Ctrl Pts',(-32.6614519649159,-54.3291228170264,
4.44599765294642));
#40812=CARTESIAN_POINT('Ctrl Pts',(-34.2363932038283,-55.3629299683766,
4.55713554351447));
#40813=CARTESIAN_POINT('Ctrl Pts',(-34.2219940520658,-57.2468062367663,
4.6682734340825));
#40814=CARTESIAN_POINT('Ctrl Pts',(-32.6314342140599,-58.2564183114437,
4.77941132465055));
#40815=CARTESIAN_POINT('Ctrl Pts',(-30.9205711526377,-57.4676568060689,
4.89054921521858));
#40816=CARTESIAN_POINT('Ctrl Pts',(-30.6553772206224,-55.602484080847,5.00168710578664));
#40817=CARTESIAN_POINT('Ctrl Pts',(-32.0785874510053,-54.3681138654151,
5.11282499635467));
#40818=CARTESIAN_POINT('Ctrl Pts',(-33.8875213407722,-54.8943792530067,
5.22396288692272));
#40819=CARTESIAN_POINT('Ctrl Pts',(-34.4264412632309,-56.6995834937722,
5.33510077749075));
#40820=CARTESIAN_POINT('Ctrl Pts',(-33.2020675476878,-58.1314028177064,
5.4462386680588));
#40821=CARTESIAN_POINT('Ctrl Pts',(-31.3350836476587,-57.8792764730931,
5.55737655862684));
#40822=CARTESIAN_POINT('Ctrl Pts',(-30.5343604901147,-56.173979132908,5.66851444919488));
#40823=CARTESIAN_POINT('Ctrl Pts',(-31.5328102757062,-54.5763876565427,
5.77965233976292));
#40824=CARTESIAN_POINT('Ctrl Pts',(-33.4165381765594,-54.5487979003782,
5.89079023033096));
#40825=CARTESIAN_POINT('Ctrl Pts',(-34.4613514910016,-56.1164585823091,
6.00192812089901));
#40826=CARTESIAN_POINT('Ctrl Pts',(-33.7109111712192,-57.8444810565579,
6.11306601146705));
#40827=CARTESIAN_POINT('Ctrl Pts',(-31.8521228057563,-58.1511689306775,
6.22420390203509));
#40828=CARTESIAN_POINT('Ctrl Pts',(-30.5863185401119,-56.7558427953566,
6.33534179260313));
#40829=CARTESIAN_POINT('Ctrl Pts',(-31.0721788644701,-54.9355898635397,
6.44647968317117));
#40830=CARTESIAN_POINT('Ctrl Pts',(-32.8648400497806,-54.3566488617232,
6.55761757373922));
#40831=CARTESIAN_POINT('Ctrl Pts',(-34.3237580856512,-55.5486512349919,
6.66875546430725));
#40832=CARTESIAN_POINT('Ctrl Pts',(-34.1129733567613,-57.4211007417246,
6.7798933548753));
#40833=CARTESIAN_POINT('Ctrl Pts',(-32.4266050042152,-58.2590134407085,
6.89103124544334));
#40834=CARTESIAN_POINT('Ctrl Pts',(-30.805840812616,-57.2976582429661,7.00216913601138));
#40835=CARTESIAN_POINT('Ctrl Pts',(-30.7389488982073,-55.4124226867889,
7.11330702657942));
#40836=CARTESIAN_POINT('Ctrl Pts',(-31.7642812766211,-54.697545560418,7.18739895362479));
#40837=CARTESIAN_POINT('Ctrl Pts',(-32.3148335773694,-54.6359733196,7.22444491714747));
#40838=CARTESIAN_POINT('Ctrl Pts',(-30.8086516228787,-55.6887746631347,
-2.07481497238249));
#40839=CARTESIAN_POINT('Ctrl Pts',(-31.009122429711,-55.1263610888822,-2.03776900885981));
#40840=CARTESIAN_POINT('Ctrl Pts',(-32.01217730928,-54.2270656189395,-1.96367708181445));
#40841=CARTESIAN_POINT('Ctrl Pts',(-33.97355427561,-54.7625083704828,-1.85253919124641));
#40842=CARTESIAN_POINT('Ctrl Pts',(-34.5821615821014,-56.7001809895466,
-1.74140130067836));
#40843=CARTESIAN_POINT('Ctrl Pts',(-33.2868853227587,-58.2626346900185,
-1.63026341011032));
#40844=CARTESIAN_POINT('Ctrl Pts',(-31.270394051269,-58.0216705087069,-1.51912551954228));
#40845=CARTESIAN_POINT('Ctrl Pts',(-30.3798618750492,-56.1968758041266,
-1.40798762897424));
#40846=CARTESIAN_POINT('Ctrl Pts',(-31.429671630603,-54.4589930404121,-1.2968497384062));
#40847=CARTESIAN_POINT('Ctrl Pts',(-33.4592879307893,-54.3984812756124,
-1.18571184783816));
#40848=CARTESIAN_POINT('Ctrl Pts',(-34.6107953909719,-56.0708505702162,
-1.07457395727011));
#40849=CARTESIAN_POINT('Ctrl Pts',(-33.83029889799,-57.9453005715134,-0.963436066702071));
#40850=CARTESIAN_POINT('Ctrl Pts',(-31.832149159935,-58.3061569687477,-0.852298176134031));
#40851=CARTESIAN_POINT('Ctrl Pts',(-30.4452986954798,-56.8231082184978,
-0.741160285565987));
#40852=CARTESIAN_POINT('Ctrl Pts',(-30.939135705398,-54.8536134933191,-0.630022394997947));
#40853=CARTESIAN_POINT('Ctrl Pts',(-32.8616514807306,-54.2003697157939,
-0.518884504429905));
#40854=CARTESIAN_POINT('Ctrl Pts',(-34.4531425620492,-55.4613003006531,
-0.407746613861863));
#40855=CARTESIAN_POINT('Ctrl Pts',(-34.2569006046968,-57.4822601904945,
-0.296608723293821));
#40856=CARTESIAN_POINT('Ctrl Pts',(-32.4525473488097,-58.41344237785,-0.185470832725779));
#40857=CARTESIAN_POINT('Ctrl Pts',(-30.6916281685284,-57.4025249956444,
-0.0743329421577378));
#40858=CARTESIAN_POINT('Ctrl Pts',(-30.5859321707133,-55.3748123143236,
0.0368049484103037));
#40859=CARTESIAN_POINT('Ctrl Pts',(-32.2322041958065,-54.186292683661,0.147942838978346));
#40860=CARTESIAN_POINT('Ctrl Pts',(-34.1235927415348,-54.9248316321148,
0.259080729546387));
#40861=CARTESIAN_POINT('Ctrl Pts',(-34.5288884461575,-56.9144360685966,
0.370218620114429));
#40862=CARTESIAN_POINT('Ctrl Pts',(-33.0771195428256,-58.3339984967673,
0.48135651068247));
#40863=CARTESIAN_POINT('Ctrl Pts',(-31.0971065789877,-57.8841773231594,
0.592494401250513));
#40864=CARTESIAN_POINT('Ctrl Pts',(-30.4011778722795,-55.97669897132,0.703632291818555));
#40865=CARTESIAN_POINT('Ctrl Pts',(-31.6263248618463,-54.3575000079462,
0.814770182386596));
#40866=CARTESIAN_POINT('Ctrl Pts',(-33.6511566132587,-54.5086516076903,
0.925908072954639));
#40867=CARTESIAN_POINT('Ctrl Pts',(-34.6223216616804,-56.2918029968741,
1.03704596352268));
#40868=CARTESIAN_POINT('Ctrl Pts',(-33.6509016243366,-58.0748154867945,
1.14818385409072));
#40869=CARTESIAN_POINT('Ctrl Pts',(-31.626048278158,-58.2256775246255,1.25932174465876));
#40870=CARTESIAN_POINT('Ctrl Pts',(-30.4011328542517,-56.6063033762813,
1.3704596352268));
#40871=CARTESIAN_POINT('Ctrl Pts',(-31.0973343316294,-54.6989245646767,
1.48159752579485));
#40872=CARTESIAN_POINT('Ctrl Pts',(-33.0774116025732,-54.2493865472287,
1.59273541636289));
#40873=CARTESIAN_POINT('Ctrl Pts',(-34.5289774853909,-55.669156569411,1.70387330693093));
#40874=CARTESIAN_POINT('Ctrl Pts',(-34.1233972656596,-57.6587030286353,
1.81501119749897));
#40875=CARTESIAN_POINT('Ctrl Pts',(-32.2319031180934,-58.3969714877809,
1.92614908806701));
#40876=CARTESIAN_POINT('Ctrl Pts',(-30.5858010869615,-57.2082164536586,
2.03728697863506));
#40877=CARTESIAN_POINT('Ctrl Pts',(-30.691787029426,-55.1805188903994,2.1484248692031));
#40878=CARTESIAN_POINT('Ctrl Pts',(-32.4528508103867,-54.1698533733089,
2.25956275977114));
#40879=CARTESIAN_POINT('Ctrl Pts',(-34.2570707793086,-55.1012935119064,
2.37070065033918));
#40880=CARTESIAN_POINT('Ctrl Pts',(-34.4530239373915,-57.1222815840843,
2.48183854090722));
#40881=CARTESIAN_POINT('Ctrl Pts',(-32.8613521367821,-58.3829842878142,
2.59297643147526));
#40882=CARTESIAN_POINT('Ctrl Pts',(-30.9389306273641,-57.7294661410314,
2.70411432204331));
#40883=CARTESIAN_POINT('Ctrl Pts',(-30.4453736184506,-55.7598997148858,
2.81525221261135));
#40884=CARTESIAN_POINT('Ctrl Pts',(-31.8324394376172,-54.2770514956311,
2.92639010317939));
#40885=CARTESIAN_POINT('Ctrl Pts',(-33.8305310101846,-54.6381892749935,
3.03752799374743));
#40886=CARTESIAN_POINT('Ctrl Pts',(-34.6107724598819,-56.5127595479419,
3.14866588431547));
#40887=CARTESIAN_POINT('Ctrl Pts',(-33.4589999392619,-58.1849468845733,
3.25980377488351));
#40888=CARTESIAN_POINT('Ctrl Pts',(-31.4294438984359,-58.1241792517757,
3.37094166545156));
#40889=CARTESIAN_POINT('Ctrl Pts',(-30.3797799983045,-56.386077952999,3.4820795560196));
#40890=CARTESIAN_POINT('Ctrl Pts',(-31.2707775106533,-54.5615468184256,
3.59321744658764));
#40891=CARTESIAN_POINT('Ctrl Pts',(-33.286896307836,-54.3205998871159,3.70435533715568));
#40892=CARTESIAN_POINT('Ctrl Pts',(-34.5827599904381,-55.8837786178316,
3.81549322772373));
#40893=CARTESIAN_POINT('Ctrl Pts',(-33.9722498337018,-57.8202877906762,
3.92663111829176));
#40894=CARTESIAN_POINT('Ctrl Pts',(-32.014172707701,-58.3576185982774,4.03776900885981));
#40895=CARTESIAN_POINT('Ctrl Pts',(-30.5007788120545,-57.0039460586119,
4.14890689942784));
#40896=CARTESIAN_POINT('Ctrl Pts',(-30.8172947423318,-54.9983019990856,
4.2600447899959));
#40897=CARTESIAN_POINT('Ctrl Pts',(-32.6740098783535,-54.1764751726168,
4.37118268056393));
#40898=CARTESIAN_POINT('Ctrl Pts',(-34.371451798864,-55.2906929942526,4.48232057113198));
#40899=CARTESIAN_POINT('Ctrl Pts',(-34.3559326650591,-57.3210992545064,
4.59345846170001));
#40900=CARTESIAN_POINT('Ctrl Pts',(-32.6416573134427,-58.4092400794901,
4.70459635226807));
#40901=CARTESIAN_POINT('Ctrl Pts',(-30.7977214198623,-57.5591278267734,
4.81573424283609));
#40902=CARTESIAN_POINT('Ctrl Pts',(-30.5119004088011,-55.5488798920819,
4.92687213340414));
#40903=CARTESIAN_POINT('Ctrl Pts',(-32.0458095141463,-54.2184989881245,
5.03801002397219));
#40904=CARTESIAN_POINT('Ctrl Pts',(-33.9954442941986,-54.7856978830043,
5.14914791454022));
#40905=CARTESIAN_POINT('Ctrl Pts',(-34.576282007745,-56.731312917807,5.26028580510827));
#40906=CARTESIAN_POINT('Ctrl Pts',(-33.2566751425585,-58.274500741577,5.37142369567631));
#40907=CARTESIAN_POINT('Ctrl Pts',(-31.2444751578683,-58.002763729403,5.48256158624435));
#40908=CARTESIAN_POINT('Ctrl Pts',(-30.38147086237,-56.1648264650488,5.59369947681239));
#40909=CARTESIAN_POINT('Ctrl Pts',(-31.4575811830053,-54.4429725464192,
5.70483736738043));
#40910=CARTESIAN_POINT('Ctrl Pts',(-33.4878275355304,-54.4132368283281,
5.81597525794848));
#40911=CARTESIAN_POINT('Ctrl Pts',(-34.6139075918674,-56.1028319020359,
5.92711314851651));
#40912=CARTESIAN_POINT('Ctrl Pts',(-33.8050971891886,-57.9652618866616,
6.03825103908456));
#40913=CARTESIAN_POINT('Ctrl Pts',(-31.8017301968603,-58.2958042848038,
6.1493889296526));
#40914=CARTESIAN_POINT('Ctrl Pts',(-30.4374702672965,-56.7919481304539,
6.26052682022065));
#40915=CARTESIAN_POINT('Ctrl Pts',(-30.9611213481761,-54.8301139006692,
6.37166471078868));
#40916=CARTESIAN_POINT('Ctrl Pts',(-32.893217714717,-54.2061422236913,6.48280260135673));
#40917=CARTESIAN_POINT('Ctrl Pts',(-34.4656120183837,-55.4908598675899,
6.59394049192477));
#40918=CARTESIAN_POINT('Ctrl Pts',(-34.2384322187942,-57.5089505799534,
6.70507838249281));
#40919=CARTESIAN_POINT('Ctrl Pts',(-32.4208962597951,-58.4120370607959,
6.81621627306085));
#40920=CARTESIAN_POINT('Ctrl Pts',(-30.6740672263624,-57.3759065863185,
6.92735416362889));
#40921=CARTESIAN_POINT('Ctrl Pts',(-30.6019723844374,-55.344035311361,7.03849205419694));
#40922=CARTESIAN_POINT('Ctrl Pts',(-31.70705625587,-54.5735542468395,7.1125839812423));
#40923=CARTESIAN_POINT('Ctrl Pts',(-32.3004311270297,-54.5071928486349,
7.14962994476498));
#40924=CARTESIAN_POINT('Ctrl Pts',(-30.6865906990182,-55.6452663749118,
-2.14962994476498));
#40925=CARTESIAN_POINT('Ctrl Pts',(-30.9015290467899,-55.042264639525,-2.1125839812423));
#40926=CARTESIAN_POINT('Ctrl Pts',(-31.9769722095413,-54.0780689767127,
-2.03849205419694));
#40927=CARTESIAN_POINT('Ctrl Pts',(-34.0798974741329,-54.6521534639338,
-1.92735416362889));
#40928=CARTESIAN_POINT('Ctrl Pts',(-34.7324266426746,-56.7296636902117,
-1.81621627306085));
#40929=CARTESIAN_POINT('Ctrl Pts',(-33.3436731204516,-58.4048762668258,
-1.70507838249281));
#40930=CARTESIAN_POINT('Ctrl Pts',(-31.181656071491,-58.146522226047,-1.59394049192477));
#40931=CARTESIAN_POINT('Ctrl Pts',(-30.2268561301985,-56.190036067175,-1.48280260135673));
#40932=CARTESIAN_POINT('Ctrl Pts',(-31.3524283663707,-54.3267340944024,
-1.37166471078868));
#40933=CARTESIAN_POINT('Ctrl Pts',(-33.5285176487258,-54.2618553275021,
-1.26052682022064));
#40934=CARTESIAN_POINT('Ctrl Pts',(-34.7631268910861,-56.0549158669708,
-1.1493889296526));
#40935=CARTESIAN_POINT('Ctrl Pts',(-33.9263036683235,-58.0646408370349,
-1.03825103908456));
#40936=CARTESIAN_POINT('Ctrl Pts',(-31.7839518212659,-58.4515394534968,
-0.92711314851652));
#40937=CARTESIAN_POINT('Ctrl Pts',(-30.2970153832539,-56.861462309195,-0.815975257948476));
#40938=CARTESIAN_POINT('Ctrl Pts',(-30.8264915332113,-54.7498334448018,
-0.704837367380436));
#40939=CARTESIAN_POINT('Ctrl Pts',(-32.8877510794003,-54.0494464884559,
-0.593699476812393));
#40940=CARTESIAN_POINT('Ctrl Pts',(-34.5940966013115,-55.4013756837693,
-0.482561586244352));
#40941=CARTESIAN_POINT('Ctrl Pts',(-34.3836922898643,-57.5681838415228,
-0.37142369567631));
#40942=CARTESIAN_POINT('Ctrl Pts',(-32.4491227944587,-58.5665674166046,
-0.260285805108268));
#40943=CARTESIAN_POINT('Ctrl Pts',(-30.5611219171738,-57.482694331548,-0.149147914540227));
#40944=CARTESIAN_POINT('Ctrl Pts',(-30.4477980696998,-55.3086460480806,
-0.0380100239721851));
#40945=CARTESIAN_POINT('Ctrl Pts',(-32.2128779566306,-54.0343535476132,
0.0731278665958571));
#40946=CARTESIAN_POINT('Ctrl Pts',(-34.2407638889375,-54.826191241361,0.184265757163899));
#40947=CARTESIAN_POINT('Ctrl Pts',(-34.6753089006883,-56.9593810910663,
0.29540364773194));
#40948=CARTESIAN_POINT('Ctrl Pts',(-33.1187690016409,-58.4813902438765,
0.406541538299982));
#40949=CARTESIAN_POINT('Ctrl Pts',(-30.9958628202429,-57.9991064571456,
0.517679428868024));
#40950=CARTESIAN_POINT('Ctrl Pts',(-30.2497104564626,-55.9539695525095,
0.628817319436065));
#40951=CARTESIAN_POINT('Ctrl Pts',(-31.5632736324488,-54.2179165311209,
0.739955210004108));
#40952=CARTESIAN_POINT('Ctrl Pts',(-33.734233075579,-54.379976412185,0.851093100572149));
#40953=CARTESIAN_POINT('Ctrl Pts',(-34.775484987615,-56.2918139484046,0.962230991140192));
#40954=CARTESIAN_POINT('Ctrl Pts',(-33.7339596846625,-58.2035025613039,
1.07336888170823));
#40955=CARTESIAN_POINT('Ctrl Pts',(-31.5629770883189,-58.365251983403,1.18450677227627));
#40956=CARTESIAN_POINT('Ctrl Pts',(-30.2496621895819,-56.6290111343268,
1.29564466284432));
#40957=CARTESIAN_POINT('Ctrl Pts',(-30.9961070092961,-54.583980953527,1.40678255341236));
#40958=CARTESIAN_POINT('Ctrl Pts',(-33.1190821387036,-54.1020007577187,
1.5179204439804));
#40959=CARTESIAN_POINT('Ctrl Pts',(-34.675404365689,-55.6242324861476,1.62905833454844));
#40960=CARTESIAN_POINT('Ctrl Pts',(-34.2405543059947,-57.7573601745032,
1.74019622511648));
#40961=CARTESIAN_POINT('Ctrl Pts',(-32.2125551507957,-58.5489078583191,
1.85133411568453));
#40962=CARTESIAN_POINT('Ctrl Pts',(-30.4476575259194,-57.274362965838,1.96247200625257));
#40963=CARTESIAN_POINT('Ctrl Pts',(-30.5612922427159,-55.1003308914696,
2.07360989682061));
#40964=CARTESIAN_POINT('Ctrl Pts',(-32.4494481561959,-54.0167278480842,
2.18474778738865));
#40965=CARTESIAN_POINT('Ctrl Pts',(-34.3838747456067,-55.0153879901866,
2.29588567795669));
#40966=CARTESIAN_POINT('Ctrl Pts',(-34.593969415771,-57.1822263641342,2.40702356852473));
#40967=CARTESIAN_POINT('Ctrl Pts',(-32.8874301324518,-58.5339112326344,
2.51816145909277));
#40968=CARTESIAN_POINT('Ctrl Pts',(-30.826271655143,-57.8332301063997,2.62929934966082));
#40969=CARTESIAN_POINT('Ctrl Pts',(-30.2970957132522,-55.7215243665374,
2.74043724022885));
#40970=CARTESIAN_POINT('Ctrl Pts',(-31.7842630476555,-54.1316622251152,
2.85157513079691));
#40971=CARTESIAN_POINT('Ctrl Pts',(-33.9265525315489,-54.51886253044,2.96271302136494));
#40972=CARTESIAN_POINT('Ctrl Pts',(-34.7631023051095,-56.5287164518977,
3.07385091193299));
#40973=CARTESIAN_POINT('Ctrl Pts',(-33.5282088734779,-58.3215819018844,
3.18498880250102));
#40974=CARTESIAN_POINT('Ctrl Pts',(-31.3521841992698,-58.2564288015505,
3.29612669306907));
#40975=CARTESIAN_POINT('Ctrl Pts',(-30.2267683445876,-56.3928925225169,
3.40726458363711));
#40976=CARTESIAN_POINT('Ctrl Pts',(-31.1820672043028,-54.4366889549245,
3.51840247420515));
#40977=CARTESIAN_POINT('Ctrl Pts',(-33.343684898298,-54.1783534090425,3.6295403647732));
#40978=CARTESIAN_POINT('Ctrl Pts',(-34.7330682368358,-55.854343339752,3.74067825534123));
#40979=CARTESIAN_POINT('Ctrl Pts',(-34.0784988934969,-57.9306061564343,
3.85181614590928));
#40980=CARTESIAN_POINT('Ctrl Pts',(-31.9791116115147,-58.5067149566014,
3.96295403647732));
#40981=CARTESIAN_POINT('Ctrl Pts',(-30.3564993788501,-57.0553508218565,
4.07409192704536));
#40982=CARTESIAN_POINT('Ctrl Pts',(-30.6958575735532,-54.9049638044908,
4.1852298176134));
#40983=CARTESIAN_POINT('Ctrl Pts',(-32.686567791791,-54.0238275282073,4.29636770818144));
#40984=CARTESIAN_POINT('Ctrl Pts',(-34.5065103938996,-55.2184560201286,
4.40750559874949));
#40985=CARTESIAN_POINT('Ctrl Pts',(-34.4898712780524,-57.3953922722465,
4.51864348931752));
#40986=CARTESIAN_POINT('Ctrl Pts',(-32.6518804128256,-58.5620618475364,
4.62978137988557));
#40987=CARTESIAN_POINT('Ctrl Pts',(-30.6748716870867,-57.650598847478,4.7409192704536));
#40988=CARTESIAN_POINT('Ctrl Pts',(-30.3684235969797,-55.4952757033166,
4.85205716102166));
#40989=CARTESIAN_POINT('Ctrl Pts',(-32.0130315772872,-54.0688841108341,
4.96319505158969));
#40990=CARTESIAN_POINT('Ctrl Pts',(-34.103367247625,-54.6770165130019,5.07433294215774));
#40991=CARTESIAN_POINT('Ctrl Pts',(-34.7261227522589,-56.7630423418419,
5.18547083272578));
#40992=CARTESIAN_POINT('Ctrl Pts',(-33.3112827374291,-58.4175986654476,
5.29660872329382));
#40993=CARTESIAN_POINT('Ctrl Pts',(-31.1538666680779,-58.126250985713,5.40774661386187));
#40994=CARTESIAN_POINT('Ctrl Pts',(-30.2285812346253,-56.1556737971897,
5.5188845044299));
#40995=CARTESIAN_POINT('Ctrl Pts',(-31.3823520903043,-54.3095574362958,
5.63002239499795));
#40996=CARTESIAN_POINT('Ctrl Pts',(-33.5591168945015,-54.2776757562781,
5.74116028556598));
#40997=CARTESIAN_POINT('Ctrl Pts',(-34.7664636927331,-56.0892052217628,
5.85229817613404));
#40998=CARTESIAN_POINT('Ctrl Pts',(-33.8992832071581,-58.0860427167654,
5.96343606670206));
#40999=CARTESIAN_POINT('Ctrl Pts',(-31.7513375879643,-58.4404396389301,
6.07457395727012));
#41000=CARTESIAN_POINT('Ctrl Pts',(-30.288621994481,-56.8280534655513,6.18571184783815));
#41001=CARTESIAN_POINT('Ctrl Pts',(-30.8500638318821,-54.7246379377986,
6.29684973840619));
#41002=CARTESIAN_POINT('Ctrl Pts',(-32.9215953796534,-54.0556355856595,
6.40798762897424));
#41003=CARTESIAN_POINT('Ctrl Pts',(-34.6074659511161,-55.4330685001879,
6.51912551954228));
#41004=CARTESIAN_POINT('Ctrl Pts',(-34.3638910808272,-57.5968004181822,
6.63026341011032));
#41005=CARTESIAN_POINT('Ctrl Pts',(-32.4151875153751,-58.5650606808834,
6.74140130067836));
#41006=CARTESIAN_POINT('Ctrl Pts',(-30.5422936401088,-57.4541549296709,
6.85253919124641));
#41007=CARTESIAN_POINT('Ctrl Pts',(-30.4649958706675,-55.275647935933,6.96367708181445));
#41008=CARTESIAN_POINT('Ctrl Pts',(-31.649831235119,-54.4495629332609,7.03776900885981));
#41009=CARTESIAN_POINT('Ctrl Pts',(-32.28602867669,-54.3784123776698,7.07481497238249));
#41010=CARTESIAN_POINT('Ctrl Pts',(-30.5645297751576,-55.601758086689,-2.22444491714747));
#41011=CARTESIAN_POINT('Ctrl Pts',(-30.7939356638689,-54.9581681901677,
-2.18739895362479));
#41012=CARTESIAN_POINT('Ctrl Pts',(-31.9417671098026,-53.9290723344859,
-2.11330702657942));
#41013=CARTESIAN_POINT('Ctrl Pts',(-34.1862406726558,-54.5417985573849,
-2.00216913601139));
#41014=CARTESIAN_POINT('Ctrl Pts',(-34.8826917032476,-56.7591463908769,
-1.89103124544334));
#41015=CARTESIAN_POINT('Ctrl Pts',(-33.4004609181446,-58.5471178436331,
-1.7798933548753));
#41016=CARTESIAN_POINT('Ctrl Pts',(-31.092918091713,-58.2713739433871,-1.66875546430726));
#41017=CARTESIAN_POINT('Ctrl Pts',(-30.0738503853478,-56.1831963302234,
-1.55761757373922));
#41018=CARTESIAN_POINT('Ctrl Pts',(-31.2751851021384,-54.1944751483927,
-1.44647968317117));
#41019=CARTESIAN_POINT('Ctrl Pts',(-33.5977473666623,-54.1252293793916,
-1.33534179260314));
#41020=CARTESIAN_POINT('Ctrl Pts',(-34.9154583912003,-56.0389811637256,
-1.22420390203509));
#41021=CARTESIAN_POINT('Ctrl Pts',(-34.0223084386569,-58.1839811025563,
-1.11306601146705));
#41022=CARTESIAN_POINT('Ctrl Pts',(-31.7357544825969,-58.596921938246,-1.00192812089901));
#41023=CARTESIAN_POINT('Ctrl Pts',(-30.1487320710282,-56.8998163998922,
-0.890790230330965));
#41024=CARTESIAN_POINT('Ctrl Pts',(-30.7138473610247,-54.6460533962845,
-0.779652339762925));
#41025=CARTESIAN_POINT('Ctrl Pts',(-32.91385067807,-53.8985232611178,-0.668514449194883));
#41026=CARTESIAN_POINT('Ctrl Pts',(-34.7350506405739,-55.3414510668855,
-0.557376558626841));
#41027=CARTESIAN_POINT('Ctrl Pts',(-34.5104839750318,-57.654107492551,-0.446238668058799));
#41028=CARTESIAN_POINT('Ctrl Pts',(-32.4456982401077,-58.7196924553593,
-0.335100777490757));
#41029=CARTESIAN_POINT('Ctrl Pts',(-30.4306156658192,-57.5628636674515,
-0.223962886922716));
#41030=CARTESIAN_POINT('Ctrl Pts',(-30.3096639686861,-55.2424797818376,
-0.112824996354674));
#41031=CARTESIAN_POINT('Ctrl Pts',(-32.1935517174549,-53.8824144115655,
-0.00168710578663172));
#41032=CARTESIAN_POINT('Ctrl Pts',(-34.3579350363402,-54.7275508506072,
0.10945078478141));
#41033=CARTESIAN_POINT('Ctrl Pts',(-34.8217293552191,-57.004326113536,0.220588675349451));
#41034=CARTESIAN_POINT('Ctrl Pts',(-33.1604184604562,-58.6287819909857,
0.331726565917493));
#41035=CARTESIAN_POINT('Ctrl Pts',(-30.8946190614981,-58.1140355911318,
0.442864456485535));
#41036=CARTESIAN_POINT('Ctrl Pts',(-30.0982430406458,-55.931240133699,0.554002347053576));
#41037=CARTESIAN_POINT('Ctrl Pts',(-31.5002224030512,-54.0783330542954,
0.665140237621618));
#41038=CARTESIAN_POINT('Ctrl Pts',(-33.8173095378994,-54.2513012166797,
0.776278128189661));
#41039=CARTESIAN_POINT('Ctrl Pts',(-34.9286483135496,-56.291824899935,0.887416018757701));
#41040=CARTESIAN_POINT('Ctrl Pts',(-33.8170177449885,-58.3321896358132,
0.998553909325746));
#41041=CARTESIAN_POINT('Ctrl Pts',(-31.4999058984797,-58.5048264421807,
1.10969179989378));
#41042=CARTESIAN_POINT('Ctrl Pts',(-30.0981915249122,-56.6517188923722,
1.22082969046183));
#41043=CARTESIAN_POINT('Ctrl Pts',(-30.8948796869627,-54.4690373423775,
1.33196758102987));
#41044=CARTESIAN_POINT('Ctrl Pts',(-33.1607526748339,-53.9546149682087,
1.44310547159791));
#41045=CARTESIAN_POINT('Ctrl Pts',(-34.8218312459871,-55.5793084028841,
1.55424336216595));
#41046=CARTESIAN_POINT('Ctrl Pts',(-34.3577113463298,-57.8560173203711,
1.665381252734));
#41047=CARTESIAN_POINT('Ctrl Pts',(-32.193207183498,-58.7008442288573,1.77651914330204));
#41048=CARTESIAN_POINT('Ctrl Pts',(-30.3095139648772,-57.3405094780172,
1.88765703387008));
#41049=CARTESIAN_POINT('Ctrl Pts',(-30.4307974560059,-55.0201428925398,
1.99879492443812));
#41050=CARTESIAN_POINT('Ctrl Pts',(-32.4460455020051,-53.8636023228594,
2.10993281500616));
#41051=CARTESIAN_POINT('Ctrl Pts',(-34.5106787119048,-54.9294824684668,
2.2210707055742));
#41052=CARTESIAN_POINT('Ctrl Pts',(-34.7349148941505,-57.2421711441843,
2.33220859614225));
#41053=CARTESIAN_POINT('Ctrl Pts',(-32.9135081281216,-58.6848381774545,
2.44334648671029));
#41054=CARTESIAN_POINT('Ctrl Pts',(-30.7136126829218,-57.9369940717681,
2.55448437727833));
#41055=CARTESIAN_POINT('Ctrl Pts',(-30.1488178080539,-55.6831490181888,
2.66562226784637));
#41056=CARTESIAN_POINT('Ctrl Pts',(-31.7360866576937,-53.9862729545993,
2.77676015841441));
#41057=CARTESIAN_POINT('Ctrl Pts',(-34.0225740529132,-54.3995357858862,
2.88789804898245));
#41058=CARTESIAN_POINT('Ctrl Pts',(-34.9154321503369,-56.5446733558537,
2.9990359395505));
#41059=CARTESIAN_POINT('Ctrl Pts',(-33.5974178076939,-58.4582169191953,
3.11017383011854));
#41060=CARTESIAN_POINT('Ctrl Pts',(-31.2749245001037,-58.3886783513254,
3.22131172068658));
#41061=CARTESIAN_POINT('Ctrl Pts',(-30.0737566908708,-56.3997070920348,
3.33244961125462));
#41062=CARTESIAN_POINT('Ctrl Pts',(-31.0933568979523,-54.3118310914232,
3.44358750182266));
#41063=CARTESIAN_POINT('Ctrl Pts',(-33.4004734887601,-54.0361069309691,
3.5547253923907));
#41064=CARTESIAN_POINT('Ctrl Pts',(-34.8833764832336,-55.8249080616723,
3.66586328295875));
#41065=CARTESIAN_POINT('Ctrl Pts',(-34.184747953292,-58.0409245221923,3.77700117352678));
#41066=CARTESIAN_POINT('Ctrl Pts',(-31.9440505153285,-58.6558113149255,
3.88813906409484));
#41067=CARTESIAN_POINT('Ctrl Pts',(-30.2122199456457,-57.106755585101,3.99927695466286));
#41068=CARTESIAN_POINT('Ctrl Pts',(-30.5744204047746,-54.811625609896,4.11041484523092));
#41069=CARTESIAN_POINT('Ctrl Pts',(-32.6991257052286,-53.8711798837978,
4.22155273579895));
#41070=CARTESIAN_POINT('Ctrl Pts',(-34.6415689889353,-55.1462190460047,
4.332690626367));
#41071=CARTESIAN_POINT('Ctrl Pts',(-34.6238098910457,-57.4696852899865,
4.44382851693503));
#41072=CARTESIAN_POINT('Ctrl Pts',(-32.6621035122086,-58.7148836155829,
4.55496640750309));
#41073=CARTESIAN_POINT('Ctrl Pts',(-30.5520219543112,-57.7420698681824,
4.66610429807112));
#41074=CARTESIAN_POINT('Ctrl Pts',(-30.2249467851584,-55.4416715145514,
4.77724218863917));
#41075=CARTESIAN_POINT('Ctrl Pts',(-31.9802536404281,-53.9192692335435,
4.8883800792072));
#41076=CARTESIAN_POINT('Ctrl Pts',(-34.2112902010514,-54.5683351429997,
4.99951796977525));
#41077=CARTESIAN_POINT('Ctrl Pts',(-34.8759634967729,-56.7947717658766,
5.1106558603433));
#41078=CARTESIAN_POINT('Ctrl Pts',(-33.3658903322998,-58.5606965893182,
5.22179375091132));
#41079=CARTESIAN_POINT('Ctrl Pts',(-31.0632581782874,-58.2497382420229,
5.33293164147938));
#41080=CARTESIAN_POINT('Ctrl Pts',(-30.0756916068807,-56.1465211293305,
5.44406953204741));
#41081=CARTESIAN_POINT('Ctrl Pts',(-31.3071229976034,-54.1761423261723,
5.55520742261546));
#41082=CARTESIAN_POINT('Ctrl Pts',(-33.6304062534726,-54.1421146842281,
5.66634531318349));
#41083=CARTESIAN_POINT('Ctrl Pts',(-34.9190197935987,-56.0755785414895,
5.77748320375154));
#41084=CARTESIAN_POINT('Ctrl Pts',(-33.9934692251276,-58.2068235468692,
5.88862109431958));
#41085=CARTESIAN_POINT('Ctrl Pts',(-31.7009449790683,-58.5850749930563,
5.99975898488762));
#41086=CARTESIAN_POINT('Ctrl Pts',(-30.1397737216657,-56.8641588006487,
6.11089687545567));
#41087=CARTESIAN_POINT('Ctrl Pts',(-30.7390063155881,-54.6191619749281,
6.2220347660237));
#41088=CARTESIAN_POINT('Ctrl Pts',(-32.9499730445898,-53.9051289476276,
6.33317265659175));
#41089=CARTESIAN_POINT('Ctrl Pts',(-34.7493198838486,-55.3752771327861,
6.44431054715979));
#41090=CARTESIAN_POINT('Ctrl Pts',(-34.4893499428602,-57.684650256411,6.55544843772784));
#41091=CARTESIAN_POINT('Ctrl Pts',(-32.4094787709551,-58.7180843009709,
6.66658632829587));
#41092=CARTESIAN_POINT('Ctrl Pts',(-30.4105200538552,-57.5324032730232,
6.77772421886391));
#41093=CARTESIAN_POINT('Ctrl Pts',(-30.3280193568976,-55.2072605605051,
6.88886210943196));
#41094=CARTESIAN_POINT('Ctrl Pts',(-31.592606214368,-54.3255716196824,6.96295403647732));
#41095=CARTESIAN_POINT('Ctrl Pts',(-32.2716262263503,-54.2496319067047,
7.));
#41096=CARTESIAN_POINT('Ctrl Pts',(-30.9307125467393,-55.7322829513575,
-2.));
#41097=CARTESIAN_POINT('Ctrl Pts',(-30.9446699885302,-55.6718824515124,
-2.));
#41098=CARTESIAN_POINT('Ctrl Pts',(-30.9622173189428,-55.6125616548506,
-2.));
#41099=CARTESIAN_POINT('Ctrl Pts',(-30.9830550110868,-55.5544917980889,
-2.));
#41100=CARTESIAN_POINT('Ctrl Pts',(-31.0052689439603,-55.4925866748552,
-2.));
#41101=CARTESIAN_POINT('Ctrl Pts',(-31.0312220593616,-55.4321024422544,
-2.));
#41102=CARTESIAN_POINT('Ctrl Pts',(-31.0606132871179,-55.3732441671078,
-2.));
#41103=CARTESIAN_POINT('Ctrl Pts',(-31.0863306114047,-55.3217431763545,
-2.));
#41104=CARTESIAN_POINT('Ctrl Pts',(-31.1146814237679,-55.2714866571797,
-2.));
#41105=CARTESIAN_POINT('Ctrl Pts',(-31.1454993456463,-55.222618038693,-2.));
#41106=CARTESIAN_POINT('Ctrl Pts',(-31.1609623517179,-55.1980980289612,
-2.));
#41107=CARTESIAN_POINT('Ctrl Pts',(-31.1770469579248,-55.17392756714,-2.));
#41108=CARTESIAN_POINT('Ctrl Pts',(-31.1937349146793,-55.1501258793141,
-2.));
#41109=CARTESIAN_POINT('Ctrl Pts',(-31.2013578381332,-55.1392534611361,
-2.));
#41110=CARTESIAN_POINT('Ctrl Pts',(-31.2091078133261,-55.1284566647586,
-2.));
#41111=CARTESIAN_POINT('Ctrl Pts',(-31.2169701001334,-55.1177546356319,
-2.));
#41112=CARTESIAN_POINT('Ctrl Pts',(-31.2566258561146,-55.063775804033,-2.));
#41113=CARTESIAN_POINT('Ctrl Pts',(-31.2992033789008,-55.0121067330815,
-2.));
#41114=CARTESIAN_POINT('Ctrl Pts',(-31.3444046039572,-54.9629466687741,
-2.));
#41115=CARTESIAN_POINT('Ctrl Pts',(-31.3904074837192,-54.9129147387853,
-2.));
#41116=CARTESIAN_POINT('Ctrl Pts',(-31.4391284049847,-54.865480696815,-2.));
#41117=CARTESIAN_POINT('Ctrl Pts',(-31.4903044396693,-54.8208703724992,
-2.));
#41118=CARTESIAN_POINT('Ctrl Pts',(-31.5331115543923,-54.7835552643125,
-2.));
#41119=CARTESIAN_POINT('Ctrl Pts',(-31.577637552122,-54.7482158610154,-2.));
#41120=CARTESIAN_POINT('Ctrl Pts',(-31.6237516110813,-54.7149996928445,
-2.));
#41121=CARTESIAN_POINT('Ctrl Pts',(-31.6449987764397,-54.6996952621866,
-2.));
#41122=CARTESIAN_POINT('Ctrl Pts',(-31.6665833415013,-54.684841812944,-2.));
#41123=CARTESIAN_POINT('Ctrl Pts',(-31.6884937600032,-54.6704551374906,
-2.));
#41124=CARTESIAN_POINT('Ctrl Pts',(-31.6980569751773,-54.6641758017952,
-2.));
#41125=CARTESIAN_POINT('Ctrl Pts',(-31.7076821200989,-54.6579856106301,
-2.));
#41126=CARTESIAN_POINT('Ctrl Pts',(-31.7173562109458,-54.6518932018194,
-2.));
#41127=CARTESIAN_POINT('Ctrl Pts',(-31.7767391574745,-54.6144958698777,
-2.));
#41128=CARTESIAN_POINT('Ctrl Pts',(-31.838074016068,-54.5807067450326,-2.));
#41129=CARTESIAN_POINT('Ctrl Pts',(-31.9010756694416,-54.5507535435306,
-2.));
#41130=CARTESIAN_POINT('Ctrl Pts',(-31.9574042848586,-54.5239729389342,
-2.));
#41131=CARTESIAN_POINT('Ctrl Pts',(-32.015066314809,-54.5002585220973,-2.));
#41132=CARTESIAN_POINT('Ctrl Pts',(-32.073885064195,-54.4797956759538,-2.));
#41133=CARTESIAN_POINT('Ctrl Pts',(-32.1379640249069,-54.457502819887,-2.));
#41134=CARTESIAN_POINT('Ctrl Pts',(-32.2034160279195,-54.4390677641938,
-2.));
#41135=CARTESIAN_POINT('Ctrl Pts',(-32.2699334847344,-54.4243849072971,
-2.));
#41136=CARTESIAN_POINT('Ctrl Pts',(-32.2955972920838,-54.4187199581427,
-2.));
#41137=CARTESIAN_POINT('Ctrl Pts',(-32.3214199362499,-54.413614055249,-2.));
#41138=CARTESIAN_POINT('Ctrl Pts',(-32.3473844776344,-54.4090630310329,
-2.));
#41139=CARTESIAN_POINT('Ctrl Pts',(-32.3587747917672,-54.4070665545815,
-2.));
#41140=CARTESIAN_POINT('Ctrl Pts',(-32.3701918520604,-54.4051770614555,
-2.));
#41141=CARTESIAN_POINT('Ctrl Pts',(-32.3816208594173,-54.4033960585375,
-2.));
#41142=CARTESIAN_POINT('Ctrl Pts',(-32.4507180638674,-54.3926285160109,
-2.));
#41143=CARTESIAN_POINT('Ctrl Pts',(-32.5203743381977,-54.3858000563254,
-2.));
#41144=CARTESIAN_POINT('Ctrl Pts',(-32.590243851397,-54.3827492853075,-2.));
#41145=CARTESIAN_POINT('Ctrl Pts',(-32.6617320286106,-54.3796278372085,
-2.));
#41146=CARTESIAN_POINT('Ctrl Pts',(-32.7334442999928,-54.380460992488,-2.));
#41147=CARTESIAN_POINT('Ctrl Pts',(-32.8050350906898,-54.3851263529469,
-2.));
#41148=CARTESIAN_POINT('Ctrl Pts',(-32.8598101377312,-54.38869588104,-2.));
#41149=CARTESIAN_POINT('Ctrl Pts',(-32.9145147054614,-54.3945098111846,
-2.));
#41150=CARTESIAN_POINT('Ctrl Pts',(-32.9689984939196,-54.4025332699526,
-2.));
#41151=CARTESIAN_POINT('Ctrl Pts',(-33.002911398737,-54.4075273939151,-2.));
#41152=CARTESIAN_POINT('Ctrl Pts',(-33.0367388219446,-54.4133779008071,
-2.));
#41153=CARTESIAN_POINT('Ctrl Pts',(-33.0704445092145,-54.4200797349956,
-2.));
#41154=CARTESIAN_POINT('Ctrl Pts',(-33.0893533889089,-54.4238394618153,
-2.));
#41155=CARTESIAN_POINT('Ctrl Pts',(-33.1082301633052,-54.4278687326753,
-2.));
#41156=CARTESIAN_POINT('Ctrl Pts',(-33.1270344168137,-54.4321588085735,
-2.));
#41157=CARTESIAN_POINT('Ctrl Pts',(-33.1999617463234,-54.4487967345891,
-2.));
#41158=CARTESIAN_POINT('Ctrl Pts',(-33.2718735596469,-54.4693655783604,
-2.));
#41159=CARTESIAN_POINT('Ctrl Pts',(-33.3423988006913,-54.493750495395,-2.));
#41160=CARTESIAN_POINT('Ctrl Pts',(-33.3951487097682,-54.5119893860017,
-2.));
#41161=CARTESIAN_POINT('Ctrl Pts',(-33.4471233201863,-54.532364245129,-2.));
#41162=CARTESIAN_POINT('Ctrl Pts',(-33.4981671222724,-54.5548460975971,
-2.));
#41163=CARTESIAN_POINT('Ctrl Pts',(-33.5140901369522,-54.5618592677029,
-2.));
#41164=CARTESIAN_POINT('Ctrl Pts',(-33.5299225529266,-54.5690775909281,
-2.));
#41165=CARTESIAN_POINT('Ctrl Pts',(-33.5456595742609,-54.5765005080885,
-2.));
#41166=CARTESIAN_POINT('Ctrl Pts',(-33.5608498130208,-54.5836655161015,
-2.));
#41167=CARTESIAN_POINT('Ctrl Pts',(-33.5759433895169,-54.5910175352492,
-2.));
#41168=CARTESIAN_POINT('Ctrl Pts',(-33.5909308710173,-54.5985527495268,
-2.));
#41169=CARTESIAN_POINT('Ctrl Pts',(-33.658231843262,-54.6323894716568,-2.));
#41170=CARTESIAN_POINT('Ctrl Pts',(-33.7234283245604,-54.6699323219136,
-2.));
#41171=CARTESIAN_POINT('Ctrl Pts',(-33.7861478874234,-54.7110945661211,
-2.));
#41172=CARTESIAN_POINT('Ctrl Pts',(-33.8341488046827,-54.742597105173,-2.));
#41173=CARTESIAN_POINT('Ctrl Pts',(-33.8806990672183,-54.7762206567485,
-2.));
#41174=CARTESIAN_POINT('Ctrl Pts',(-33.9256254254142,-54.8119460488582,
-2.));
#41175=CARTESIAN_POINT('Ctrl Pts',(-33.9360516193134,-54.8202369471242,
-2.));
#41176=CARTESIAN_POINT('Ctrl Pts',(-33.9463903172992,-54.8286411175249,
-2.));
#41177=CARTESIAN_POINT('Ctrl Pts',(-33.9566410663199,-54.8371566128168,
-2.));
#41178=CARTESIAN_POINT('Ctrl Pts',(-33.3347877909359,-57.7349452754743,
-0.871480363390215));
#41179=CARTESIAN_POINT('Ctrl Pts',(-33.4089783616458,-57.692956018043,-0.877193940366672));
#41180=CARTESIAN_POINT('Ctrl Pts',(-33.4797275640263,-57.6452118511612,
-0.882907517343129));
#41181=CARTESIAN_POINT('Ctrl Pts',(-33.5459978166813,-57.5919001635712,
-0.888621094319586));
#41182=CARTESIAN_POINT('Ctrl Pts',(-33.9756840487236,-57.2462352951484,
-0.925667057842266));
#41183=CARTESIAN_POINT('Ctrl Pts',(-34.2170739697906,-56.6665102843049,
-0.962713021364947));
#41184=CARTESIAN_POINT('Ctrl Pts',(-34.1597013173233,-56.1180347705934,
-0.999758984887627));
#41185=CARTESIAN_POINT('Ctrl Pts',(-34.102328664856,-55.5695592568819,-1.03680494841031));
#41186=CARTESIAN_POINT('Ctrl Pts',(-33.7461934388544,-55.0523332403023,
-1.07385091193299));
#41187=CARTESIAN_POINT('Ctrl Pts',(-33.254268606184,-54.8030776924624,-1.11089687545567));
#41188=CARTESIAN_POINT('Ctrl Pts',(-32.7623437735136,-54.5538221446225,
-1.14794283897835));
#41189=CARTESIAN_POINT('Ctrl Pts',(-32.1346293341744,-54.5725370655222,
-1.18498880250103));
#41190=CARTESIAN_POINT('Ctrl Pts',(-31.6584309020156,-54.850638451748,-1.22203476602371));
#41191=CARTESIAN_POINT('Ctrl Pts',(-31.1822324698568,-55.1287398379739,
-1.25908072954639));
#41192=CARTESIAN_POINT('Ctrl Pts',(-30.8575500448784,-55.666227689526,-1.29612669306907));
#41193=CARTESIAN_POINT('Ctrl Pts',(-30.8329195675803,-56.2171554903502,
-1.33317265659175));
#41194=CARTESIAN_POINT('Ctrl Pts',(-30.8082890902823,-56.7680832911743,
-1.37021862011443));
#41195=CARTESIAN_POINT('Ctrl Pts',(-31.0837105606646,-57.3324510412706,
-1.40726458363711));
#41196=CARTESIAN_POINT('Ctrl Pts',(-31.5332488781923,-57.6518973032928,
-1.44431054715979));
#41197=CARTESIAN_POINT('Ctrl Pts',(-31.9827871957199,-57.971343565315,-1.48135651068247));
#41198=CARTESIAN_POINT('Ctrl Pts',(-32.6064423603928,-58.0458683392631,
-1.51840247420516));
#41199=CARTESIAN_POINT('Ctrl Pts',(-33.1185697754731,-57.8415149221822,
-1.55544843772784));
#41200=CARTESIAN_POINT('Ctrl Pts',(-33.1924454681488,-57.8120364178238,
-1.56079241294863));
#41201=CARTESIAN_POINT('Ctrl Pts',(-33.2640004019439,-57.7767547923516,
-1.56613638816942));
#41202=CARTESIAN_POINT('Ctrl Pts',(-33.3326856027611,-57.7363329907929,
-1.57148036339021));
#41203=CARTESIAN_POINT('Ctrl Pts',(-34.4842965055667,-55.7582049595679,
-2.));
#41204=CARTESIAN_POINT('Ctrl Pts',(-34.6616800870191,-56.4180307560557,
-1.96295403647732));
#41205=CARTESIAN_POINT('Ctrl Pts',(-34.3029408546812,-57.9173199920238,
-1.88886210943196));
#41206=CARTESIAN_POINT('Ctrl Pts',(-32.1083909227282,-58.6899905331757,
-1.77772421886392));
#41207=CARTESIAN_POINT('Ctrl Pts',(-30.2743670907292,-57.2623912321518,
-1.66658632829588));
#41208=CARTESIAN_POINT('Ctrl Pts',(-30.4765028746714,-54.9487367869862,
-1.55544843772783));
#41209=CARTESIAN_POINT('Ctrl Pts',(-32.5312595152503,-53.8630292597193,
-1.44431054715979));
#41210=CARTESIAN_POINT('Ctrl Pts',(-34.5571577499755,-55.0008883544571,
-1.33317265659175));
#41211=CARTESIAN_POINT('Ctrl Pts',(-34.7002397993375,-57.3198853035068,
-1.22203476602371));
#41212=CARTESIAN_POINT('Ctrl Pts',(-32.8293553152893,-58.697884688863,-1.11089687545567));
#41213=CARTESIAN_POINT('Ctrl Pts',(-30.6570393620673,-57.873352597378,-0.999758984887624));
#41214=CARTESIAN_POINT('Ctrl Pts',(-30.1715905180573,-55.6011108576298,
-0.888621094319583));
#41215=CARTESIAN_POINT('Ctrl Pts',(-31.817369145763,-53.960908709333,-0.77748320375154));
#41216=CARTESIAN_POINT('Ctrl Pts',(-34.087963584719,-54.4540716106361,-0.666345313183499));
#41217=CARTESIAN_POINT('Ctrl Pts',(-34.9050789303496,-56.6291869825843,
-0.555207422615457));
#41218=CARTESIAN_POINT('Ctrl Pts',(-33.5207972588595,-58.4953545827796,
-0.444069532047416));
#41219=CARTESIAN_POINT('Ctrl Pts',(-31.2021687803137,-58.3444462635109,
-0.332931641479373));
#41220=CARTESIAN_POINT('Ctrl Pts',(-30.0714596841225,-56.3145920190741,
-0.221793750911332));
#41221=CARTESIAN_POINT('Ctrl Pts',(-31.1636212068567,-54.2637395061114,
-0.11065586034329));
#41222=CARTESIAN_POINT('Ctrl Pts',(-33.4789853310955,-54.069057766837,0.000482030224751219));
#41223=CARTESIAN_POINT('Ctrl Pts',(-34.8982731111897,-55.908740964546,0.111619920792794));
#41224=CARTESIAN_POINT('Ctrl Pts',(-34.1223942983453,-58.0989063257425,
0.222757811360835));
#41225=CARTESIAN_POINT('Ctrl Pts',(-31.8615195930587,-58.6348705964901,
0.333895701928877));
#41226=CARTESIAN_POINT('Ctrl Pts',(-30.1850532410697,-57.0260596319961,
0.445033592496918));
#41227=CARTESIAN_POINT('Ctrl Pts',(-30.6274839128386,-54.7450363379152,
0.556171483064961));
#41228=CARTESIAN_POINT('Ctrl Pts',(-32.783849793945,-53.8796472115696,0.667309373633002));
#41229=CARTESIAN_POINT('Ctrl Pts',(-34.6804047400893,-55.2219927306232,
0.778447264201044));
#41230=CARTESIAN_POINT('Ctrl Pts',(-34.5812104999015,-57.5434088201914,
0.889585154769086));
#41231=CARTESIAN_POINT('Ctrl Pts',(-32.5770606867505,-58.7190770058698,
1.00072304533713));
#41232=CARTESIAN_POINT('Ctrl Pts',(-30.5023763530244,-57.6728948648119,
1.11186093590517));
#41233=CARTESIAN_POINT('Ctrl Pts',(-30.2561395980006,-55.3624447749947,
1.22299882647321));
#41234=CARTESIAN_POINT('Ctrl Pts',(-32.0637337160182,-53.9025079060376,
1.33413671704125));
#41235=CARTESIAN_POINT('Ctrl Pts',(-34.2706473113688,-54.629381030845,1.4452746076093));
#41236=CARTESIAN_POINT('Ctrl Pts',(-34.8568673421131,-56.8777489350102,
1.55641249817734));
#41237=CARTESIAN_POINT('Ctrl Pts',(-33.2858199659299,-58.5896549776086,
1.66755038874538));
#41238=CARTESIAN_POINT('Ctrl Pts',(-30.9955026631254,-58.198172143523,1.77868827931342));
#41239=CARTESIAN_POINT('Ctrl Pts',(-30.0822688349231,-56.0616291105052,
1.88982616988146));
#41240=CARTESIAN_POINT('Ctrl Pts',(-31.3820117610517,-54.1356279467243,
2.0009640604495));
#41241=CARTESIAN_POINT('Ctrl Pts',(-33.7050620011389,-54.1830593597269,
2.11210195101755));
#41242=CARTESIAN_POINT('Ctrl Pts',(-34.9251053252509,-56.1605088392832,
2.22323984158559));
#41243=CARTESIAN_POINT('Ctrl Pts',(-33.925422242596,-58.2579944509529,2.33437773215363));
#41244=CARTESIAN_POINT('Ctrl Pts',(-31.6210340159052,-58.55566382727,2.44551562272167));
#41245=CARTESIAN_POINT('Ctrl Pts',(-30.1211733226087,-56.7810568122912,
2.55665351328971));
#41246=CARTESIAN_POINT('Ctrl Pts',(-30.7986796648578,-54.5584913322389,
2.66779140385775));
#41247=CARTESIAN_POINT('Ctrl Pts',(-33.0334238041475,-53.9223067766118,
2.7789292944258));
#41248=CARTESIAN_POINT('Ctrl Pts',(-34.7799190860636,-55.4548100839991,
2.89006718499384));
#41249=CARTESIAN_POINT('Ctrl Pts',(-34.4395785724647,-57.7532835973795,
3.00120507556188));
#41250=CARTESIAN_POINT('Ctrl Pts',(-32.3239197951718,-58.7139084434935,
3.11234296612992));
#41251=CARTESIAN_POINT('Ctrl Pts',(-30.3694292262435,-57.4574138064661,
3.22348085669796));
#41252=CARTESIAN_POINT('Ctrl Pts',(-30.3650742488504,-55.1338834771873,
3.334618747266));
#41253=CARTESIAN_POINT('Ctrl Pts',(-32.3148410231895,-53.870071116671,3.44575663783405));
#41254=CARTESIAN_POINT('Ctrl Pts',(-34.4340859088485,-54.822758511107,3.55689452840208));
#41255=CARTESIAN_POINT('Ctrl Pts',(-34.7830400281131,-57.1199400841539,
3.66803241897013));
#41256=CARTESIAN_POINT('Ctrl Pts',(-33.0423017182097,-58.6589794901991,
3.77917030953817));
#41257=CARTESIAN_POINT('Ctrl Pts',(-30.8051884955116,-58.0311765069792,
3.89030820010621));
#41258=CARTESIAN_POINT('Ctrl Pts',(-30.1193554633367,-55.8111663248381,
4.00144609067426));
#41259=CARTESIAN_POINT('Ctrl Pts',(-31.6125533739246,-54.0309494400522,
4.11258398124229));
#41260=CARTESIAN_POINT('Ctrl Pts',(-33.9180412456697,-54.3199785564283,
4.22372187181034));
#41261=CARTESIAN_POINT('Ctrl Pts',(-34.9255798836094,-56.4137020456762,
4.33485976237838));
#41262=CARTESIAN_POINT('Ctrl Pts',(-33.71295774606,-58.3957110541618,4.44599765294642));
#41263=CARTESIAN_POINT('Ctrl Pts',(-31.3901016278141,-58.451850257884,4.55713554351447));
#41264=CARTESIAN_POINT('Ctrl Pts',(-30.0831480764379,-56.5307348090517,
4.6682734340825));
#41265=CARTESIAN_POINT('Ctrl Pts',(-30.9883665002518,-54.3907834608548,
4.77941132465055));
#41266=CARTESIAN_POINT('Ctrl Pts',(-33.2772002083032,-53.990717959075,4.89054921521859));
#41267=CARTESIAN_POINT('Ctrl Pts',(-34.8546537539781,-55.6967227784588,
5.00168710578663));
#41268=CARTESIAN_POINT('Ctrl Pts',(-34.2768660104017,-57.9472723924375,
5.11282499635467));
#41269=CARTESIAN_POINT('Ctrl Pts',(-32.0726926657226,-58.6824131526073,
5.22396288692272));
#41270=CARTESIAN_POINT('Ctrl Pts',(-30.2596385516872,-57.2292625110704,
5.33510077749076));
#41271=CARTESIAN_POINT('Ctrl Pts',(-30.4972127153845,-54.9179054771162,
5.44623866805879));
#41272=CARTESIAN_POINT('Ctrl Pts',(-32.5679607208419,-53.8639538597436,
5.55737655862685));
#41273=CARTESIAN_POINT('Ctrl Pts',(-34.5765036531329,-55.0321005249753,
5.66851444919488));
#41274=CARTESIAN_POINT('Ctrl Pts',(-34.6843989531681,-57.3531295774156,
5.77965233976293));
#41275=CARTESIAN_POINT('Ctrl Pts',(-32.7928896947834,-58.7025728310562,
5.89079023033096));
#41276=CARTESIAN_POINT('Ctrl Pts',(-30.6332940299706,-57.8452774805725,
6.00192812089901));
#41277=CARTESIAN_POINT('Ctrl Pts',(-30.1823177935136,-55.5659199366928,
6.11306601146705));
#41278=CARTESIAN_POINT('Ctrl Pts',(-31.8527378172474,-53.9508533596396,
6.22420390203509));
#41279=CARTESIAN_POINT('Ctrl Pts',(-34.1156133119216,-54.4783040835128,
6.33534179260312));
#41280=CARTESIAN_POINT('Ctrl Pts',(-34.8996815919165,-56.6656147589772,
6.44647968317118));
#41281=CARTESIAN_POINT('Ctrl Pts',(-33.4873299906743,-58.510467673716,6.55761757373921));
#41282=CARTESIAN_POINT('Ctrl Pts',(-31.1711925871668,-58.3247407101007,
6.66875546430726));
#41283=CARTESIAN_POINT('Ctrl Pts',(-30.0714699489351,-56.2774508415845,
6.7798933548753));
#41284=CARTESIAN_POINT('Ctrl Pts',(-31.1943253650081,-54.2444600690086,
6.89103124544334));
#41285=CARTESIAN_POINT('Ctrl Pts',(-33.5128402220712,-54.0826823257856,
7.00216913601138));
#41286=CARTESIAN_POINT('Ctrl Pts',(-34.903205848792,-55.9481454299591,7.11330702657942));
#41287=CARTESIAN_POINT('Ctrl Pts',(-34.3645996631225,-57.3926056844023,
7.18739895362479));
#41288=CARTESIAN_POINT('Ctrl Pts',(-33.8493101059357,-57.841283396055,7.22444491714747));
#41289=CARTESIAN_POINT('Ctrl Pts',(-34.3591563398468,-55.7918468858113,
-2.07481497238249));
#41290=CARTESIAN_POINT('Ctrl Pts',(-34.5253531804484,-56.4100605999883,
-2.03776900885981));
#41291=CARTESIAN_POINT('Ctrl Pts',(-34.189237929385,-57.8147967775173,-1.96367708181445));
#41292=CARTESIAN_POINT('Ctrl Pts',(-32.1330878491652,-58.5387386537266,
-1.85253919124641));
#41293=CARTESIAN_POINT('Ctrl Pts',(-30.4147271983626,-57.2011712670918,
-1.74140130067836));
#41294=CARTESIAN_POINT('Ctrl Pts',(-30.6041152374846,-55.033428030193,-1.63026341011032));
#41295=CARTESIAN_POINT('Ctrl Pts',(-32.5292881259404,-54.0161909253172,
-1.51912551954228));
#41296=CARTESIAN_POINT('Ctrl Pts',(-34.4274225712752,-55.0822906457469,
-1.40798762897424));
#41297=CARTESIAN_POINT('Ctrl Pts',(-34.561481114665,-57.2550394601585,-1.2968497384062));
#41298=CARTESIAN_POINT('Ctrl Pts',(-32.8085844382453,-58.5461349624701,
-1.18571184783815));
#41299=CARTESIAN_POINT('Ctrl Pts',(-30.7732661452114,-57.7736021978399,
-1.07457395727011));
#41300=CARTESIAN_POINT('Ctrl Pts',(-30.3184322564854,-55.6446599635185,
-0.96343606670207));
#41301=CARTESIAN_POINT('Ctrl Pts',(-31.860419434863,-54.1078975824522,-0.85229817613403));
#41302=CARTESIAN_POINT('Ctrl Pts',(-33.9878182558372,-54.5699590394787,
-0.741160285565987));
#41303=CARTESIAN_POINT('Ctrl Pts',(-34.7534020135839,-56.6079002051822,
-0.630022394997947));
#41304=CARTESIAN_POINT('Ctrl Pts',(-33.4564204191172,-58.3563774692333,
-0.518884504429904));
#41305=CARTESIAN_POINT('Ctrl Pts',(-31.2840168375231,-58.2149862216467,
-0.407746613861863));
#41306=CARTESIAN_POINT('Ctrl Pts',(-30.2246161991564,-56.3131452533626,
-0.29660872329382));
#41307=CARTESIAN_POINT('Ctrl Pts',(-31.2479002766274,-54.3916302777182,
-0.185470832725779));
#41308=CARTESIAN_POINT('Ctrl Pts',(-33.4172453712524,-54.209226192034,-0.0743329421577374));
#41309=CARTESIAN_POINT('Ctrl Pts',(-34.7470254051468,-55.9328892992031,
0.0368049484103048));
#41310=CARTESIAN_POINT('Ctrl Pts',(-34.0200775877185,-57.9849313227407,
0.147942838978346));
#41311=CARTESIAN_POINT('Ctrl Pts',(-31.9017855229282,-58.4870948699203,
0.259080729546388));
#41312=CARTESIAN_POINT('Ctrl Pts',(-30.3310459494339,-56.9797439796361,
0.370218620114429));
#41313=CARTESIAN_POINT('Ctrl Pts',(-30.7455746179339,-54.8425740019479,
0.481356510682472));
#41314=CARTESIAN_POINT('Ctrl Pts',(-32.7659487342222,-54.0317608617915,
0.592494401250513));
#41315=CARTESIAN_POINT('Ctrl Pts',(-34.5428969584923,-55.2894510179814,
0.703632291818555));
#41316=CARTESIAN_POINT('Ctrl Pts',(-34.4499584283865,-57.4644664091971,
0.814770182386597));
#41317=CARTESIAN_POINT('Ctrl Pts',(-32.5722008348668,-58.5659907805945,
0.92590807295464));
#41318=CARTESIAN_POINT('Ctrl Pts',(-30.6283569983197,-57.5857863833555,
1.03704596352268));
#41319=CARTESIAN_POINT('Ctrl Pts',(-30.3976492271164,-55.4210454183169,
1.14818385409072));
#41320=CARTESIAN_POINT('Ctrl Pts',(-32.0912469605976,-54.0531798407264,
1.25932174465876));
#41321=CARTESIAN_POINT('Ctrl Pts',(-34.1589809866262,-54.7342125263452,
1.37045963522681));
#41322=CARTESIAN_POINT('Ctrl Pts',(-34.7082309014681,-56.8407865346196,
1.48159752579485));
#41323=CARTESIAN_POINT('Ctrl Pts',(-33.2362620291564,-58.4447307855874,
1.59273541636289));
#41324=CARTESIAN_POINT('Ctrl Pts',(-31.0903841717777,-58.0779369163799,
1.70387330693093));
#41325=CARTESIAN_POINT('Ctrl Pts',(-30.2347436681021,-56.0761355152048,
1.81501119749897));
#41326=CARTESIAN_POINT('Ctrl Pts',(-31.4525179747665,-54.2715981065311,
1.92614908806701));
#41327=CARTESIAN_POINT('Ctrl Pts',(-33.6290644583814,-54.3160382453633,
2.03728697863506));
#41328=CARTESIAN_POINT('Ctrl Pts',(-34.772165438778,-56.1687793686431,2.1484248692031));
#41329=CARTESIAN_POINT('Ctrl Pts',(-33.8355276249524,-58.133986514719,2.25956275977114));
#41330=CARTESIAN_POINT('Ctrl Pts',(-31.6764662300946,-58.4128832958229,
2.37070065033918));
#41331=CARTESIAN_POINT('Ctrl Pts',(-30.2711946343393,-56.7501923253057,
2.48183854090722));
#41332=CARTESIAN_POINT('Ctrl Pts',(-30.9059738661454,-54.66779350468,2.59297643147526));
#41333=CARTESIAN_POINT('Ctrl Pts',(-32.9997832957543,-54.0717300904733,
2.70411432204331));
#41334=CARTESIAN_POINT('Ctrl Pts',(-34.6361354068315,-55.5075856855278,
2.81525221261135));
#41335=CARTESIAN_POINT('Ctrl Pts',(-34.3172585546124,-57.6611053799802,
2.92639010317939));
#41336=CARTESIAN_POINT('Ctrl Pts',(-32.3350243382431,-58.5611481749239,
3.03752799374743));
#41337=CARTESIAN_POINT('Ctrl Pts',(-30.503794216031,-57.3838946929672,3.14866588431548));
#41338=CARTESIAN_POINT('Ctrl Pts',(-30.4997138863991,-55.206898397108,3.25980377488351));
#41339=CARTESIAN_POINT('Ctrl Pts',(-32.3265181213336,-54.0227886857625,
3.37094166545156));
#41340=CARTESIAN_POINT('Ctrl Pts',(-34.3121122872295,-54.9153946064446,
3.48207955601959));
#41341=CARTESIAN_POINT('Ctrl Pts',(-34.6390595258738,-57.0677038371105,
3.59321744658764));
#41342=CARTESIAN_POINT('Ctrl Pts',(-33.0081013218997,-58.5096833300925,
3.70435533715568));
#41343=CARTESIAN_POINT('Ctrl Pts',(-30.9120722157322,-57.9214729022893,
3.81549322772372));
#41344=CARTESIAN_POINT('Ctrl Pts',(-30.2694914188265,-55.8414682290595,
3.92663111829176));
#41345=CARTESIAN_POINT('Ctrl Pts',(-31.6685204219656,-54.173521176607,4.03776900885981));
#41346=CARTESIAN_POINT('Ctrl Pts',(-33.8286121124817,-54.4443225979688,
4.14890689942785));
#41347=CARTESIAN_POINT('Ctrl Pts',(-34.7726100689923,-56.406004880834,4.26004478999589));
#41348=CARTESIAN_POINT('Ctrl Pts',(-33.6364622561333,-58.2630179851871,
4.37118268056393));
#41349=CARTESIAN_POINT('Ctrl Pts',(-31.460097652016,-58.3156167556941,4.48232057113198));
#41350=CARTESIAN_POINT('Ctrl Pts',(-30.2355674600263,-56.5156569431084,
4.59345846170002));
#41351=CARTESIAN_POINT('Ctrl Pts',(-31.0836980528375,-54.5106621730211,
4.70459635226806));
#41352=CARTESIAN_POINT('Ctrl Pts',(-33.2281858787453,-54.1358269042488,
4.8157342428361));
#41353=CARTESIAN_POINT('Ctrl Pts',(-34.7061569138339,-55.7342420941505,
4.92687213340414));
#41354=CARTESIAN_POINT('Ctrl Pts',(-34.1648075018169,-57.842860222152,5.03801002397218));
#41355=CARTESIAN_POINT('Ctrl Pts',(-32.0996409118516,-58.5316391425983,
5.14914791454023));
#41356=CARTESIAN_POINT('Ctrl Pts',(-30.4009275183955,-57.1701318172633,
5.26028580510827));
#41357=CARTESIAN_POINT('Ctrl Pts',(-30.6235190068059,-55.0045411047512,
5.37142369567631));
#41358=CARTESIAN_POINT('Ctrl Pts',(-32.5636747606314,-54.017057215205,5.48256158624435));
#41359=CARTESIAN_POINT('Ctrl Pts',(-34.445548420111,-55.1115344127627,5.59369947681239));
#41360=CARTESIAN_POINT('Ctrl Pts',(-34.5466392755034,-57.2861871754458,
5.70483736738044));
#41361=CARTESIAN_POINT('Ctrl Pts',(-32.7744185314064,-58.550527445779,5.81597525794847));
#41362=CARTESIAN_POINT('Ctrl Pts',(-30.7510183185456,-57.7472976454435,
5.92711314851652));
#41363=CARTESIAN_POINT('Ctrl Pts',(-30.3284830135764,-55.6116883669947,
6.03825103908455));
#41364=CARTESIAN_POINT('Ctrl Pts',(-31.8935575720505,-54.0984763759544,
6.1493889296526));
#41365=CARTESIAN_POINT('Ctrl Pts',(-34.0137242459347,-54.5926632852668,
6.26052682022064));
#41366=CARTESIAN_POINT('Ctrl Pts',(-34.748345059677,-56.6420306545566,6.37166471078869));
#41367=CARTESIAN_POINT('Ctrl Pts',(-33.4250637727444,-58.3705374492314,
6.48280260135672));
#41368=CARTESIAN_POINT('Ctrl Pts',(-31.2549941659053,-58.1965234039931,
6.59394049192477));
#41369=CARTESIAN_POINT('Ctrl Pts',(-30.2246258166159,-56.2783463937137,
6.70507838249281));
#41370=CARTESIAN_POINT('Ctrl Pts',(-31.2766680692063,-54.3735667032384,
6.81621627306085));
#41371=CARTESIAN_POINT('Ctrl Pts',(-33.4489651948854,-54.221991514694,6.9273541636289));
#41372=CARTESIAN_POINT('Ctrl Pts',(-34.7516470583929,-55.9698087119449,
7.03849205419693));
#41373=CARTESIAN_POINT('Ctrl Pts',(-34.2470082093303,-57.3231737116671,
7.1125839812423));
#41374=CARTESIAN_POINT('Ctrl Pts',(-33.7642155196223,-57.7435554488857,
7.14962994476498));
#41375=CARTESIAN_POINT('Ctrl Pts',(-34.2340161741268,-55.8254888120548,
-2.14962994476498));
#41376=CARTESIAN_POINT('Ctrl Pts',(-34.3890262738776,-56.4020904439209,
-2.1125839812423));
#41377=CARTESIAN_POINT('Ctrl Pts',(-34.0755350040887,-57.7122735630108,
-2.03849205419694));
#41378=CARTESIAN_POINT('Ctrl Pts',(-32.1577847756022,-58.3874867742776,
-1.92735416362889));
#41379=CARTESIAN_POINT('Ctrl Pts',(-30.555087305996,-57.1399513020318,-1.81621627306086));
#41380=CARTESIAN_POINT('Ctrl Pts',(-30.7317276002978,-55.1181192733998,
-1.70507838249281));
#41381=CARTESIAN_POINT('Ctrl Pts',(-32.5273167366305,-54.1693525909151,
-1.59394049192477));
#41382=CARTESIAN_POINT('Ctrl Pts',(-34.297687392575,-55.1636929370367,-1.48280260135673));
#41383=CARTESIAN_POINT('Ctrl Pts',(-34.4227224299925,-57.1901936168101,
-1.37166471078869));
#41384=CARTESIAN_POINT('Ctrl Pts',(-32.7878135612013,-58.3943852360772,
-1.26052682022064));
#41385=CARTESIAN_POINT('Ctrl Pts',(-30.8894929283555,-57.6738517983019,
-1.1493889296526));
#41386=CARTESIAN_POINT('Ctrl Pts',(-30.4652739949134,-55.6882090694072,
-1.03825103908456));
#41387=CARTESIAN_POINT('Ctrl Pts',(-31.9034697239631,-54.2548864555713,
-0.927113148516517));
#41388=CARTESIAN_POINT('Ctrl Pts',(-33.8876729269555,-54.6858464683214,
-0.815975257948478));
#41389=CARTESIAN_POINT('Ctrl Pts',(-34.6017250968181,-56.5866134277799,
-0.704837367380434));
#41390=CARTESIAN_POINT('Ctrl Pts',(-33.3920435793749,-58.217400355687,-0.593699476812393));
#41391=CARTESIAN_POINT('Ctrl Pts',(-31.3658648947325,-58.0855261797824,
-0.482561586244351));
#41392=CARTESIAN_POINT('Ctrl Pts',(-30.3777727141903,-56.3116984876511,
-0.371423695676309));
#41393=CARTESIAN_POINT('Ctrl Pts',(-31.3321793463982,-54.519521049325,-0.260285805108268));
#41394=CARTESIAN_POINT('Ctrl Pts',(-33.3555054114092,-54.3493946172309,
-0.149147914540226));
#41395=CARTESIAN_POINT('Ctrl Pts',(-34.5957776991039,-55.9570376338604,
-0.0380100239721841));
#41396=CARTESIAN_POINT('Ctrl Pts',(-33.9177608770916,-57.8709563197388,
0.0731278665958575));
#41397=CARTESIAN_POINT('Ctrl Pts',(-31.9420514527978,-58.3393191433505,
0.184265757163899));
#41398=CARTESIAN_POINT('Ctrl Pts',(-30.4770386577982,-56.933428327276,0.295403647731941));
#41399=CARTESIAN_POINT('Ctrl Pts',(-30.8636653230293,-54.9401116659806,
0.406541538299983));
#41400=CARTESIAN_POINT('Ctrl Pts',(-32.7480476744994,-54.1838745120134,
0.517679428868024));
#41401=CARTESIAN_POINT('Ctrl Pts',(-34.4053891768952,-55.3569093053397,
0.628817319436066));
#41402=CARTESIAN_POINT('Ctrl Pts',(-34.3187063568714,-57.3855239982029,
0.739955210004108));
#41403=CARTESIAN_POINT('Ctrl Pts',(-32.5673409829831,-58.412904555319,0.85109310057215));
#41404=CARTESIAN_POINT('Ctrl Pts',(-30.7543376436151,-57.4986779018991,
0.962230991140191));
#41405=CARTESIAN_POINT('Ctrl Pts',(-30.5391588562322,-55.4796460616391,
1.07336888170823));
#41406=CARTESIAN_POINT('Ctrl Pts',(-32.1187602051768,-54.2038517754153,
1.18450677227628));
#41407=CARTESIAN_POINT('Ctrl Pts',(-34.0473146618836,-54.8390440218455,
1.29564466284432));
#41408=CARTESIAN_POINT('Ctrl Pts',(-34.559594460823,-56.8038241342291,1.40678255341236));
#41409=CARTESIAN_POINT('Ctrl Pts',(-33.1867040923831,-58.299806593566,1.5179204439804));
#41410=CARTESIAN_POINT('Ctrl Pts',(-31.18526568043,-57.9577016892369,1.62905833454844));
#41411=CARTESIAN_POINT('Ctrl Pts',(-30.3872185012811,-56.0906419199043,
1.74019622511648));
#41412=CARTESIAN_POINT('Ctrl Pts',(-31.5230241884812,-54.4075682663379,
1.85133411568453));
#41413=CARTESIAN_POINT('Ctrl Pts',(-33.5530669156239,-54.4490171309997,
1.96247200625257));
#41414=CARTESIAN_POINT('Ctrl Pts',(-34.6192255523049,-56.1770498980029,
2.07360989682061));
#41415=CARTESIAN_POINT('Ctrl Pts',(-33.7456330073089,-58.0099785784851,
2.18474778738865));
#41416=CARTESIAN_POINT('Ctrl Pts',(-31.731898444284,-58.2701027643757,2.29588567795669));
#41417=CARTESIAN_POINT('Ctrl Pts',(-30.42121594607,-56.7193278383203,2.40702356852474));
#41418=CARTESIAN_POINT('Ctrl Pts',(-31.0132680674328,-54.7770956771211,
2.51816145909277));
#41419=CARTESIAN_POINT('Ctrl Pts',(-32.9661427873613,-54.2211534043347,
2.62929934966082));
#41420=CARTESIAN_POINT('Ctrl Pts',(-34.4923517275992,-55.5603612870565,
2.74043724022886));
#41421=CARTESIAN_POINT('Ctrl Pts',(-34.1949385367603,-57.568927162581,2.8515751307969));
#41422=CARTESIAN_POINT('Ctrl Pts',(-32.3461288813143,-58.4083879063543,
2.96271302136494));
#41423=CARTESIAN_POINT('Ctrl Pts',(-30.6381592058186,-57.3103755794683,
3.07385091193299));
#41424=CARTESIAN_POINT('Ctrl Pts',(-30.6343535239478,-55.2799133170287,
3.18498880250102));
#41425=CARTESIAN_POINT('Ctrl Pts',(-32.3381952194778,-54.175506254854,3.29612669306907));
#41426=CARTESIAN_POINT('Ctrl Pts',(-34.1901386656105,-55.0080307017823,
3.4072645836371));
#41427=CARTESIAN_POINT('Ctrl Pts',(-34.4950790236344,-57.0154675900672,
3.51840247420515));
#41428=CARTESIAN_POINT('Ctrl Pts',(-32.9739009255896,-58.360387169986,3.62954036477319));
#41429=CARTESIAN_POINT('Ctrl Pts',(-31.0189559359529,-57.8117692975993,
3.74067825534124));
#41430=CARTESIAN_POINT('Ctrl Pts',(-30.4196273743162,-55.871770133281,3.85181614590928));
#41431=CARTESIAN_POINT('Ctrl Pts',(-31.7244874700066,-54.3160929131617,
3.96295403647732));
#41432=CARTESIAN_POINT('Ctrl Pts',(-33.7391829792937,-54.5686666395095,
4.07409192704536));
#41433=CARTESIAN_POINT('Ctrl Pts',(-34.6196402543753,-56.3983077159918,
4.1852298176134));
#41434=CARTESIAN_POINT('Ctrl Pts',(-33.5599667662066,-58.1303249162125,
4.29636770818144));
#41435=CARTESIAN_POINT('Ctrl Pts',(-31.5300936762181,-58.1793832535041,
4.40750559874949));
#41436=CARTESIAN_POINT('Ctrl Pts',(-30.3879868436147,-56.5005790771652,
4.51864348931753));
#41437=CARTESIAN_POINT('Ctrl Pts',(-31.1790296054234,-54.6305408851872,
4.62978137988557));
#41438=CARTESIAN_POINT('Ctrl Pts',(-33.1791715491872,-54.2809358494227,
4.74091927045361));
#41439=CARTESIAN_POINT('Ctrl Pts',(-34.5576600736897,-55.7717614098421,
4.85205716102165));
#41440=CARTESIAN_POINT('Ctrl Pts',(-34.0527489932321,-57.7384480518666,
4.96319505158969));
#41441=CARTESIAN_POINT('Ctrl Pts',(-32.1265891579805,-58.3808651325893,
5.07433294215774));
#41442=CARTESIAN_POINT('Ctrl Pts',(-30.5422164851038,-57.1110011234561,
5.18547083272577));
#41443=CARTESIAN_POINT('Ctrl Pts',(-30.7498252982273,-55.0911767323862,
5.29660872329383));
#41444=CARTESIAN_POINT('Ctrl Pts',(-32.559388800421,-54.1701605706663,5.40774661386186));
#41445=CARTESIAN_POINT('Ctrl Pts',(-34.314593187089,-55.1909683005502,5.51888450442991));
#41446=CARTESIAN_POINT('Ctrl Pts',(-34.4088795978388,-57.2192447734761,
5.63002239499795));
#41447=CARTESIAN_POINT('Ctrl Pts',(-32.7559473680293,-58.3984820605017,
5.74116028556599));
#41448=CARTESIAN_POINT('Ctrl Pts',(-30.8687426071208,-57.6493178103144,
5.85229817613403));
#41449=CARTESIAN_POINT('Ctrl Pts',(-30.474648233639,-55.6574567972966,5.96343606670207));
#41450=CARTESIAN_POINT('Ctrl Pts',(-31.9343773268536,-54.2460993922691,
6.07457395727011));
#41451=CARTESIAN_POINT('Ctrl Pts',(-33.9118351799479,-54.7070224870209,
6.18571184783815));
#41452=CARTESIAN_POINT('Ctrl Pts',(-34.5970085274374,-56.618446550136,6.29684973840619));
#41453=CARTESIAN_POINT('Ctrl Pts',(-33.3627975548144,-58.2306072247468,
6.40798762897424));
#41454=CARTESIAN_POINT('Ctrl Pts',(-31.3387957446438,-58.0683060978855,
6.51912551954228));
#41455=CARTESIAN_POINT('Ctrl Pts',(-30.3777816842967,-56.2792419458429,
6.63026341011032));
#41456=CARTESIAN_POINT('Ctrl Pts',(-31.3590107734043,-54.5026733374681,
6.74140130067836));
#41457=CARTESIAN_POINT('Ctrl Pts',(-33.3850901676996,-54.3613007036025,
6.8525391912464));
#41458=CARTESIAN_POINT('Ctrl Pts',(-34.6000882679937,-55.9914719939308,
6.96367708181445));
#41459=CARTESIAN_POINT('Ctrl Pts',(-34.129416755538,-57.2537417389318,7.03776900885981));
#41460=CARTESIAN_POINT('Ctrl Pts',(-33.6791209333089,-57.6458275017164,
7.07481497238249));
#41461=CARTESIAN_POINT('Ctrl Pts',(-34.1088760084069,-55.8591307382982,
-2.22444491714747));
#41462=CARTESIAN_POINT('Ctrl Pts',(-34.2526993673069,-56.3941202878534,
-2.18739895362479));
#41463=CARTESIAN_POINT('Ctrl Pts',(-33.9618320787925,-57.6097503485045,
-2.11330702657943));
#41464=CARTESIAN_POINT('Ctrl Pts',(-32.1824817020393,-58.2362348948284,
-2.00216913601138));
#41465=CARTESIAN_POINT('Ctrl Pts',(-30.6954474136293,-57.0787313369718,
-1.89103124544334));
#41466=CARTESIAN_POINT('Ctrl Pts',(-30.8593399631111,-55.2028105166065,
-1.7798933548753));
#41467=CARTESIAN_POINT('Ctrl Pts',(-32.5253453473206,-54.3225142565131,
-1.66875546430726));
#41468=CARTESIAN_POINT('Ctrl Pts',(-34.1679522138747,-55.2450952283264,
-1.55761757373922));
#41469=CARTESIAN_POINT('Ctrl Pts',(-34.28396374532,-57.1253477734617,-1.44647968317117));
#41470=CARTESIAN_POINT('Ctrl Pts',(-32.7670426841572,-58.2426355096843,
-1.33534179260313));
#41471=CARTESIAN_POINT('Ctrl Pts',(-31.0057197114997,-57.5741013987637,
-1.22420390203509));
#41472=CARTESIAN_POINT('Ctrl Pts',(-30.6121157333415,-55.7317581752959,
-1.11306601146705));
#41473=CARTESIAN_POINT('Ctrl Pts',(-31.946520013063,-54.4018753286905,-1.00192812089901));
#41474=CARTESIAN_POINT('Ctrl Pts',(-33.7875275980737,-54.8017338971639,
-0.890790230330965));
#41475=CARTESIAN_POINT('Ctrl Pts',(-34.4500481800523,-56.5653266503777,
-0.779652339762924));
#41476=CARTESIAN_POINT('Ctrl Pts',(-33.3276667396325,-58.0784232421408,
-0.668514449194882));
#41477=CARTESIAN_POINT('Ctrl Pts',(-31.4477129519419,-57.9560661379181,
-0.557376558626841));
#41478=CARTESIAN_POINT('Ctrl Pts',(-30.5309292292241,-56.3102517219397,
-0.446238668058798));
#41479=CARTESIAN_POINT('Ctrl Pts',(-31.416458416169,-54.6474118209318,-0.335100777490757));
#41480=CARTESIAN_POINT('Ctrl Pts',(-33.293765451566,-54.4895630424278,-0.223962886922715));
#41481=CARTESIAN_POINT('Ctrl Pts',(-34.444529993061,-55.9811859685177,-0.112824996354673));
#41482=CARTESIAN_POINT('Ctrl Pts',(-33.8154441664647,-57.7569813167368,
-0.00168710578663119));
#41483=CARTESIAN_POINT('Ctrl Pts',(-31.9823173826674,-58.1915434167808,
0.10945078478141));
#41484=CARTESIAN_POINT('Ctrl Pts',(-30.6230313661624,-56.887112674916,0.220588675349452));
#41485=CARTESIAN_POINT('Ctrl Pts',(-30.9817560281246,-55.0376493300133,
0.331726565917494));
#41486=CARTESIAN_POINT('Ctrl Pts',(-32.7301466147767,-54.3359881622352,
0.442864456485535));
#41487=CARTESIAN_POINT('Ctrl Pts',(-34.2678813952981,-55.424367592698,0.554002347053577));
#41488=CARTESIAN_POINT('Ctrl Pts',(-34.1874542853563,-57.3065815872086,
0.66514023762162));
#41489=CARTESIAN_POINT('Ctrl Pts',(-32.5624811310993,-58.2598183300436,
0.776278128189661));
#41490=CARTESIAN_POINT('Ctrl Pts',(-30.8803182889104,-57.4115694204427,
0.887416018757703));
#41491=CARTESIAN_POINT('Ctrl Pts',(-30.6806684853481,-55.5382467049613,
0.998553909325745));
#41492=CARTESIAN_POINT('Ctrl Pts',(-32.1462734497562,-54.3545237101042,
1.10969179989379));
#41493=CARTESIAN_POINT('Ctrl Pts',(-33.935648337141,-54.9438755173456,1.22082969046183));
#41494=CARTESIAN_POINT('Ctrl Pts',(-34.4109580201779,-56.7668617338386,
1.33196758102987));
#41495=CARTESIAN_POINT('Ctrl Pts',(-33.1371461556097,-58.1548824015447,
1.44310547159791));
#41496=CARTESIAN_POINT('Ctrl Pts',(-31.2801471890823,-57.8374664620939,
1.55424336216595));
#41497=CARTESIAN_POINT('Ctrl Pts',(-30.5396933344601,-56.1051483246038,
1.66538125273399));
#41498=CARTESIAN_POINT('Ctrl Pts',(-31.593530402196,-54.5435384261447,1.77651914330204));
#41499=CARTESIAN_POINT('Ctrl Pts',(-33.4770693728664,-54.5819960166361,
1.88765703387008));
#41500=CARTESIAN_POINT('Ctrl Pts',(-34.4662856658319,-56.1853204273629,
1.99879492443812));
#41501=CARTESIAN_POINT('Ctrl Pts',(-33.6557383896654,-57.8859706422512,
2.10993281500616));
#41502=CARTESIAN_POINT('Ctrl Pts',(-31.7873306584733,-58.1273222329285,
2.2210707055742));
#41503=CARTESIAN_POINT('Ctrl Pts',(-30.5712372578007,-56.6884633513348,
2.33220859614225));
#41504=CARTESIAN_POINT('Ctrl Pts',(-31.1205622687204,-54.8863978495622,
2.44334648671028));
#41505=CARTESIAN_POINT('Ctrl Pts',(-32.9325022789682,-54.3705767181961,
2.55448437727833));
#41506=CARTESIAN_POINT('Ctrl Pts',(-34.3485680483669,-55.6131368885852,
2.66562226784637));
#41507=CARTESIAN_POINT('Ctrl Pts',(-34.072618518908,-57.4767489451818,2.77676015841441));
#41508=CARTESIAN_POINT('Ctrl Pts',(-32.3572334243856,-58.2556276377847,
2.88789804898246));
#41509=CARTESIAN_POINT('Ctrl Pts',(-30.7725241956062,-57.2368564659694,
2.99903593955049));
#41510=CARTESIAN_POINT('Ctrl Pts',(-30.7689931614965,-55.3529282369495,
3.11017383011854));
#41511=CARTESIAN_POINT('Ctrl Pts',(-32.3498723176219,-54.3282238239455,
3.22131172068658));
#41512=CARTESIAN_POINT('Ctrl Pts',(-34.0681650439915,-55.1006667971199,
3.33244961125462));
#41513=CARTESIAN_POINT('Ctrl Pts',(-34.351098521395,-56.9632313430239,3.44358750182266));
#41514=CARTESIAN_POINT('Ctrl Pts',(-32.9397005292796,-58.2110910098794,
3.5547253923907));
#41515=CARTESIAN_POINT('Ctrl Pts',(-31.1258396561734,-57.7020656929093,
3.66586328295875));
#41516=CARTESIAN_POINT('Ctrl Pts',(-30.569763329806,-55.9020720375025,3.77700117352679));
#41517=CARTESIAN_POINT('Ctrl Pts',(-31.7804545180476,-54.4586646497165,
3.88813906409483));
#41518=CARTESIAN_POINT('Ctrl Pts',(-33.6497538461057,-54.69301068105,3.99927695466287));
#41519=CARTESIAN_POINT('Ctrl Pts',(-34.4666704397583,-56.3906105511496,
4.11041484523092));
#41520=CARTESIAN_POINT('Ctrl Pts',(-33.4834712762798,-57.9976318472376,
4.22155273579895));
#41521=CARTESIAN_POINT('Ctrl Pts',(-31.6000897004201,-58.0431497513143,
4.332690626367));
#41522=CARTESIAN_POINT('Ctrl Pts',(-30.540406227203,-56.4855012112218,4.44382851693504));
#41523=CARTESIAN_POINT('Ctrl Pts',(-31.2743611580092,-54.7504195973536,
4.55496640750308));
#41524=CARTESIAN_POINT('Ctrl Pts',(-33.1301572196292,-54.4260447945964,
4.66610429807112));
#41525=CARTESIAN_POINT('Ctrl Pts',(-34.4091632335455,-55.8092807255337,
4.77724218863916));
#41526=CARTESIAN_POINT('Ctrl Pts',(-33.9406904846474,-57.6340358815812,
4.88838007920721));
#41527=CARTESIAN_POINT('Ctrl Pts',(-32.1535374041094,-58.2300911225802,
4.99951796977525));
#41528=CARTESIAN_POINT('Ctrl Pts',(-30.6835054518121,-57.051870429649,5.11065586034329));
#41529=CARTESIAN_POINT('Ctrl Pts',(-30.8761315896487,-55.1778123600212,
5.22179375091132));
#41530=CARTESIAN_POINT('Ctrl Pts',(-32.5551028402105,-54.3232639261277,
5.33293164147938));
#41531=CARTESIAN_POINT('Ctrl Pts',(-34.1836379540671,-55.2704021883376,
5.44406953204741));
#41532=CARTESIAN_POINT('Ctrl Pts',(-34.2711199201742,-57.1523023715063,
5.55520742261546));
#41533=CARTESIAN_POINT('Ctrl Pts',(-32.7374762046522,-58.2464366752245,
5.6663453131835));
#41534=CARTESIAN_POINT('Ctrl Pts',(-30.9864668956958,-57.5513379751853,
5.77748320375154));
#41535=CARTESIAN_POINT('Ctrl Pts',(-30.6208134537018,-55.7032252275985,
5.88862109431958));
#41536=CARTESIAN_POINT('Ctrl Pts',(-31.9751970816568,-54.3937224085839,
5.99975898488763));
#41537=CARTESIAN_POINT('Ctrl Pts',(-33.809946113961,-54.8213816887749,6.11089687545566));
#41538=CARTESIAN_POINT('Ctrl Pts',(-34.4456719951979,-56.5948624457155,
6.22203476602371));
#41539=CARTESIAN_POINT('Ctrl Pts',(-33.3005313368845,-58.0906770002622,
6.33317265659175));
#41540=CARTESIAN_POINT('Ctrl Pts',(-31.4225973233824,-57.940088791778,6.44431054715979));
#41541=CARTESIAN_POINT('Ctrl Pts',(-30.5309375519776,-56.2801374979719,
6.55544843772783));
#41542=CARTESIAN_POINT('Ctrl Pts',(-31.4413534776024,-54.631779971698,6.66658632829587));
#41543=CARTESIAN_POINT('Ctrl Pts',(-33.3212151405137,-54.5006098925109,
6.77772421886392));
#41544=CARTESIAN_POINT('Ctrl Pts',(-34.4485294775946,-56.0131352759167,
6.88886210943196));
#41545=CARTESIAN_POINT('Ctrl Pts',(-34.0118253017458,-57.1843097661965,
6.96295403647732));
#41546=CARTESIAN_POINT('Ctrl Pts',(-33.5940263469955,-57.5480995545471,
7.));
#41547=CARTESIAN_POINT('Ctrl Pts',(-33.3311039683456,-57.7330494773494,
-1.37851963660979));
#41548=CARTESIAN_POINT('Ctrl Pts',(-33.1447009981387,-57.8419592717116,
-1.3641270219409));
#41549=CARTESIAN_POINT('Ctrl Pts',(-32.9385791362006,-57.9159412173671,
-1.34973440727202));
#41550=CARTESIAN_POINT('Ctrl Pts',(-32.7263090322414,-57.9449985351604,
-1.33534179260313));
#41551=CARTESIAN_POINT('Ctrl Pts',(-32.1799350266047,-58.0197908060441,
-1.29829582908045));
#41552=CARTESIAN_POINT('Ctrl Pts',(-31.5928273690522,-57.7969461024039,
-1.26124986555777));
#41553=CARTESIAN_POINT('Ctrl Pts',(-31.2336728772496,-57.3784665466725,
-1.22420390203509));
#41554=CARTESIAN_POINT('Ctrl Pts',(-30.874518385447,-56.9599869909411,-1.18715793851241));
#41555=CARTESIAN_POINT('Ctrl Pts',(-30.7433170593942,-56.3458725831185,
-1.15011197498972));
#41556=CARTESIAN_POINT('Ctrl Pts',(-30.9001171096548,-55.8171682381063,
-1.11306601146704));
#41557=CARTESIAN_POINT('Ctrl Pts',(-31.0569171599153,-55.2884638930941,
-1.07602004794436));
#41558=CARTESIAN_POINT('Ctrl Pts',(-31.5017185864892,-54.8451696108923,
-1.03897408442168));
#41559=CARTESIAN_POINT('Ctrl Pts',(-32.0309538972779,-54.690165564537,-1.001928120899));
#41560=CARTESIAN_POINT('Ctrl Pts',(-32.5601892080666,-54.5351615181817,
-0.964882157376321));
#41561=CARTESIAN_POINT('Ctrl Pts',(-33.1738584030701,-54.6684477076728,
-0.92783619385364));
#41562=CARTESIAN_POINT('Ctrl Pts',(-33.5911130975683,-55.029022927954,-0.89079023033096));
#41563=CARTESIAN_POINT('Ctrl Pts',(-34.0083677920666,-55.3895981482352,
-0.85374426680828));
#41564=CARTESIAN_POINT('Ctrl Pts',(-34.2292079860594,-55.9774623993065,
-0.816698303285599));
#41565=CARTESIAN_POINT('Ctrl Pts',(-34.1525645096526,-56.5235772901359,
-0.779652339762918));
#41566=CARTESIAN_POINT('Ctrl Pts',(-34.0828208613931,-57.0205281937339,
-0.745941438711876));
#41567=CARTESIAN_POINT('Ctrl Pts',(-33.7667445152314,-57.4829083508763,
-0.712230537660833));
#41568=CARTESIAN_POINT('Ctrl Pts',(-33.333352483612,-57.7367881187288,-0.678519636609791));
#41569=CARTESIAN_POINT('Ctrl Pts',(-34.4842965055667,-55.7582049595679,
-2.));
#41570=CARTESIAN_POINT('Ctrl Pts',(-34.4966111053925,-55.8303827605032,
-2.));
#41571=CARTESIAN_POINT('Ctrl Pts',(-34.5047055015069,-55.9030302259436,
-2.));
#41572=CARTESIAN_POINT('Ctrl Pts',(-34.5087398487957,-55.9758367243127,
-2.));
#41573=CARTESIAN_POINT('Ctrl Pts',(-34.5128864619035,-56.0506692458712,
-2.));
#41574=CARTESIAN_POINT('Ctrl Pts',(-34.5127437096053,-56.1256707869288,
-2.));
#41575=CARTESIAN_POINT('Ctrl Pts',(-34.5084312212538,-56.2004993443971,
-2.));
#41576=CARTESIAN_POINT('Ctrl Pts',(-34.5047872656981,-56.2637277905937,
-2.));
#41577=CARTESIAN_POINT('Ctrl Pts',(-34.4981650958835,-56.3268329649123,
-2.));
#41578=CARTESIAN_POINT('Ctrl Pts',(-34.4886099106142,-56.3895978470298,
-2.));
#41579=CARTESIAN_POINT('Ctrl Pts',(-34.4843647905612,-56.4174826501178,
-2.));
#41580=CARTESIAN_POINT('Ctrl Pts',(-34.4795404472607,-56.4453001134184,
-2.));
#41581=CARTESIAN_POINT('Ctrl Pts',(-34.4741394411489,-56.4730302233706,
-2.));
#41582=CARTESIAN_POINT('Ctrl Pts',(-34.4711718179615,-56.4882667396012,
-2.));
#41583=CARTESIAN_POINT('Ctrl Pts',(-34.4680300836906,-56.5034768715492,
-2.));
#41584=CARTESIAN_POINT('Ctrl Pts',(-34.4647145599135,-56.5186572039182,
-2.));
#41585=CARTESIAN_POINT('Ctrl Pts',(-34.4616570554945,-56.5326561785661,
-2.));
#41586=CARTESIAN_POINT('Ctrl Pts',(-34.4584511621501,-56.5466318131544,
-2.));
#41587=CARTESIAN_POINT('Ctrl Pts',(-34.455102574428,-56.5605599363278,-2.));
#41588=CARTESIAN_POINT('Ctrl Pts',(-34.4379902743587,-56.6317368750642,
-2.));
#41589=CARTESIAN_POINT('Ctrl Pts',(-34.4171297712858,-56.7017985031099,
-2.));
#41590=CARTESIAN_POINT('Ctrl Pts',(-34.3926364221818,-56.7704257260604,
-2.));
#41591=CARTESIAN_POINT('Ctrl Pts',(-34.3683331729296,-56.8385203136065,
-2.));
#41592=CARTESIAN_POINT('Ctrl Pts',(-34.3404527390919,-56.9052035572272,
-2.));
#41593=CARTESIAN_POINT('Ctrl Pts',(-34.3090644243598,-56.9701370641959,
-2.));
#41594=CARTESIAN_POINT('Ctrl Pts',(-34.2829778948812,-57.0241026835084,
-2.));
#41595=CARTESIAN_POINT('Ctrl Pts',(-34.2544675459326,-57.0768595084288,
-2.));
#41596=CARTESIAN_POINT('Ctrl Pts',(-34.2235537441983,-57.1281926115905,
-2.));
#41597=CARTESIAN_POINT('Ctrl Pts',(-34.2106502677957,-57.1496191411066,
-2.));
#41598=CARTESIAN_POINT('Ctrl Pts',(-34.1973278568808,-57.1707973646492,
-2.));
#41599=CARTESIAN_POINT('Ctrl Pts',(-34.1835872002804,-57.1917104459739,
-2.));
#41600=CARTESIAN_POINT('Ctrl Pts',(-34.1772270825361,-57.201390453523,-2.));
#41601=CARTESIAN_POINT('Ctrl Pts',(-34.1707773506251,-57.2110136443072,
-2.));
#41602=CARTESIAN_POINT('Ctrl Pts',(-34.1642380419192,-57.2205782911529,
-2.));
#41603=CARTESIAN_POINT('Ctrl Pts',(-34.157417623102,-57.2305541005635,-2.));
#41604=CARTESIAN_POINT('Ctrl Pts',(-34.1505044191199,-57.2404593595929,
-2.));
#41605=CARTESIAN_POINT('Ctrl Pts',(-34.1435014736481,-57.2502888014669,
-2.));
#41606=CARTESIAN_POINT('Ctrl Pts',(-34.1036166314025,-57.306271778928,-2.));
#41607=CARTESIAN_POINT('Ctrl Pts',(-34.060796839317,-57.3598374440704,-2.));
#41608=CARTESIAN_POINT('Ctrl Pts',(-34.0151074156417,-57.4106900609363,
-2.));
#41609=CARTESIAN_POINT('Ctrl Pts',(-33.9736959571746,-57.4567812755301,
-2.));
#41610=CARTESIAN_POINT('Ctrl Pts',(-33.9299264067076,-57.5006437323222,
-2.));
#41611=CARTESIAN_POINT('Ctrl Pts',(-33.8838248402233,-57.5420278185054,
-2.));
#41612=CARTESIAN_POINT('Ctrl Pts',(-33.8292843968241,-57.5909872483519,
-2.));
#41613=CARTESIAN_POINT('Ctrl Pts',(-33.7714790326439,-57.6364792135475,
-2.));
#41614=CARTESIAN_POINT('Ctrl Pts',(-33.7108128089775,-57.6783572197639,
-2.));
#41615=CARTESIAN_POINT('Ctrl Pts',(-33.6974562676305,-57.6875772649185,
-2.));
#41616=CARTESIAN_POINT('Ctrl Pts',(-33.6839610126009,-57.6966218980591,
-2.));
#41617=CARTESIAN_POINT('Ctrl Pts',(-33.6703313137196,-57.7054891532988,
-2.));
#41618=CARTESIAN_POINT('Ctrl Pts',(-33.6562679227736,-57.7146385613776,
-2.));
#41619=CARTESIAN_POINT('Ctrl Pts',(-33.6420560771609,-57.7236022055286,
-2.));
#41620=CARTESIAN_POINT('Ctrl Pts',(-33.6277297174331,-57.7323603945599,
-2.));
#41621=CARTESIAN_POINT('Ctrl Pts',(-33.569215230036,-57.7681322829829,-2.));
#41622=CARTESIAN_POINT('Ctrl Pts',(-33.5087208994633,-57.8005303979709,
-2.));
#41623=CARTESIAN_POINT('Ctrl Pts',(-33.4466000497741,-57.8294900318504,
-2.));
#41624=CARTESIAN_POINT('Ctrl Pts',(-33.3844917460994,-57.8584438170014,
-2.));
#41625=CARTESIAN_POINT('Ctrl Pts',(-33.3207564252812,-57.8839606526953,
-2.));
#41626=CARTESIAN_POINT('Ctrl Pts',(-33.2557354106634,-57.9059253945374,
-2.));
#41627=CARTESIAN_POINT('Ctrl Pts',(-33.208672827818,-57.921823600505,-2.));
#41628=CARTESIAN_POINT('Ctrl Pts',(-33.1609363812249,-57.9358598412448,
-2.));
#41629=CARTESIAN_POINT('Ctrl Pts',(-33.1126567567386,-57.9479733084138,
-2.));
#41630=CARTESIAN_POINT('Ctrl Pts',(-33.0764412555869,-57.9570598597049,
-2.));
#41631=CARTESIAN_POINT('Ctrl Pts',(-33.0399201288692,-57.9650642116716,
-2.));
#41632=CARTESIAN_POINT('Ctrl Pts',(-33.0031501969155,-57.971955216011,-2.));
#41633=CARTESIAN_POINT('Ctrl Pts',(-32.9909318988865,-57.9742450310926,
-2.));
#41634=CARTESIAN_POINT('Ctrl Pts',(-32.9786957156912,-57.9764100788847,
-2.));
#41635=CARTESIAN_POINT('Ctrl Pts',(-32.9664441134404,-57.978449652198,-2.));
#41636=CARTESIAN_POINT('Ctrl Pts',(-32.9014564692778,-57.9892684056978,
-2.));
#41637=CARTESIAN_POINT('Ctrl Pts',(-32.8360307197657,-57.9965613002934,
-2.));
#41638=CARTESIAN_POINT('Ctrl Pts',(-32.7704812212859,-58.0002046036746,
-2.));
#41639=CARTESIAN_POINT('Ctrl Pts',(-32.7243572374865,-58.0027682185004,
-2.));
#41640=CARTESIAN_POINT('Ctrl Pts',(-32.6781720129221,-58.0035238244839,
-2.));
#41641=CARTESIAN_POINT('Ctrl Pts',(-32.6320397021299,-58.0024136109099,
-2.));
#41642=CARTESIAN_POINT('Ctrl Pts',(-32.617232011996,-58.0020572511633,-2.));
#41643=CARTESIAN_POINT('Ctrl Pts',(-32.602427781608,-58.0015084555319,-2.));
#41644=CARTESIAN_POINT('Ctrl Pts',(-32.5876374051278,-58.0007653782452,
-2.));
#41645=CARTESIAN_POINT('Ctrl Pts',(-32.5246283833583,-57.9975997676203,
-2.));
#41646=CARTESIAN_POINT('Ctrl Pts',(-32.4619962285786,-57.9909192311159,
-2.));
#41647=CARTESIAN_POINT('Ctrl Pts',(-32.400031070834,-57.9805958152526,-2.));
#41648=CARTESIAN_POINT('Ctrl Pts',(-32.3429040942487,-57.9710784419776,
-2.));
#41649=CARTESIAN_POINT('Ctrl Pts',(-32.286343647263,-57.9584643876265,-2.));
#41650=CARTESIAN_POINT('Ctrl Pts',(-32.2305948723589,-57.942618319326,-2.));
#41651=CARTESIAN_POINT('Ctrl Pts',(-32.2201618224275,-57.9396528223787,
-2.));
#41652=CARTESIAN_POINT('Ctrl Pts',(-32.2097572620708,-57.9365740341467,
-2.));
#41653=CARTESIAN_POINT('Ctrl Pts',(-32.1993825459687,-57.9333829869217,
-2.));
#41654=CARTESIAN_POINT('Origin',(-32.5,-56.2916512459885,3.));
#41655=CARTESIAN_POINT('Origin',(-65.,8.89946740503873E-15,7.));
#41656=CARTESIAN_POINT('Ctrl Pts',(-66.6351293272515,0.319230454628283,
7.));
#41657=CARTESIAN_POINT('Ctrl Pts',(-66.6302897730465,0.381554702501259,
7.));
#41658=CARTESIAN_POINT('Ctrl Pts',(-66.6216732730338,0.443394711745685,
7.));
#41659=CARTESIAN_POINT('Ctrl Pts',(-66.6095363361235,0.504531338378675,
7.));
#41660=CARTESIAN_POINT('Ctrl Pts',(-66.6018369189666,0.543315126700851,
7.));
#41661=CARTESIAN_POINT('Ctrl Pts',(-66.5927196857307,0.581816142993964,
7.));
#41662=CARTESIAN_POINT('Ctrl Pts',(-66.5822397317333,0.619979888911372,
7.));
#41663=CARTESIAN_POINT('Ctrl Pts',(-66.5750556337901,0.646141462580533,
7.));
#41664=CARTESIAN_POINT('Ctrl Pts',(-66.5672309975512,0.672144565072526,
7.));
#41665=CARTESIAN_POINT('Ctrl Pts',(-66.5587815171007,0.697971622792422,
7.));
#41666=CARTESIAN_POINT('Ctrl Pts',(-66.5543304403759,0.711576981862657,
7.));
#41667=CARTESIAN_POINT('Ctrl Pts',(-66.5497059363263,0.725133119483741,
7.));
#41668=CARTESIAN_POINT('Ctrl Pts',(-66.5449151802375,0.738624322294838,
7.));
#41669=CARTESIAN_POINT('Ctrl Pts',(-66.5228385613039,0.800794079613728,
7.));
#41670=CARTESIAN_POINT('Ctrl Pts',(-66.4972129904487,0.861656595066855,
7.));
#41671=CARTESIAN_POINT('Ctrl Pts',(-66.4682928028772,0.92096726482602,7.));
#41672=CARTESIAN_POINT('Ctrl Pts',(-66.4474370013299,0.963739171303899,
7.));
#41673=CARTESIAN_POINT('Ctrl Pts',(-66.4248666019437,1.00570421605069,7.));
#41674=CARTESIAN_POINT('Ctrl Pts',(-66.4006603556943,1.04676903427261,7.));
#41675=CARTESIAN_POINT('Ctrl Pts',(-66.3939846935385,1.05809399767726,7.));
#41676=CARTESIAN_POINT('Ctrl Pts',(-66.3871845384137,1.06935047516562,7.));
#41677=CARTESIAN_POINT('Ctrl Pts',(-66.3802613700562,1.08053645880643,7.));
#41678=CARTESIAN_POINT('Ctrl Pts',(-66.3732910155434,1.09179868262147,7.));
#41679=CARTESIAN_POINT('Ctrl Pts',(-66.3662003390708,1.10298231941115,7.));
#41680=CARTESIAN_POINT('Ctrl Pts',(-66.3589938160321,1.11408178978621,7.));
#41681=CARTESIAN_POINT('Ctrl Pts',(-66.3220437714873,1.17099216425959,7.));
#41682=CARTESIAN_POINT('Ctrl Pts',(-66.282032873356,1.22572189959788,7.));
#41683=CARTESIAN_POINT('Ctrl Pts',(-66.2392195751637,1.27802354476839,7.));
#41684=CARTESIAN_POINT('Ctrl Pts',(-66.1957886597093,1.3310796844594,7.));
#41685=CARTESIAN_POINT('Ctrl Pts',(-66.1494735383167,1.38163817192085,7.));
#41686=CARTESIAN_POINT('Ctrl Pts',(-66.1004928622018,1.42942737710376,7.));
#41687=CARTESIAN_POINT('Ctrl Pts',(-66.0701495067946,1.45903262048774,7.));
#41688=CARTESIAN_POINT('Ctrl Pts',(-66.0387821881987,1.48757476215782,7.));
#41689=CARTESIAN_POINT('Ctrl Pts',(-66.0064342584863,1.5149840981904,7.));
#41690=CARTESIAN_POINT('Ctrl Pts',(-65.9799267072476,1.53744471269536,7.));
#41691=CARTESIAN_POINT('Ctrl Pts',(-65.9527605445103,1.55914459484554,7.));
#41692=CARTESIAN_POINT('Ctrl Pts',(-65.9249567185444,1.58004263011316,7.));
#41693=CARTESIAN_POINT('Ctrl Pts',(-65.9136073279895,1.58857310949302,7.));
#41694=CARTESIAN_POINT('Ctrl Pts',(-65.9021495270296,1.59697131003777,7.));
#41695=CARTESIAN_POINT('Ctrl Pts',(-65.8906044505102,1.60522061990068,7.));
#41696=CARTESIAN_POINT('Ctrl Pts',(-65.8332561981007,1.64619769817525,7.));
#41697=CARTESIAN_POINT('Ctrl Pts',(-65.7736595595608,1.68357914695984,7.));
#41698=CARTESIAN_POINT('Ctrl Pts',(-65.7120551180979,1.71709301893351,7.));
#41699=CARTESIAN_POINT('Ctrl Pts',(-65.705214574854,1.72081439169597,7.));
#41700=CARTESIAN_POINT('Ctrl Pts',(-65.6983492298774,1.72448805151161,7.));
#41701=CARTESIAN_POINT('Ctrl Pts',(-65.6914593790744,1.72811360467695,7.));
#41702=CARTESIAN_POINT('Ctrl Pts',(-65.6317930119903,1.75951103144772,7.));
#41703=CARTESIAN_POINT('Ctrl Pts',(-65.5702916682012,1.78730397727325,7.));
#41704=CARTESIAN_POINT('Ctrl Pts',(-65.5072864773022,1.81157490046172,7.));
#41705=CARTESIAN_POINT('Ctrl Pts',(-65.4395015551833,1.8376870765318,7.));
#41706=CARTESIAN_POINT('Ctrl Pts',(-65.3699753257167,1.85972336261184,7.));
#41707=CARTESIAN_POINT('Ctrl Pts',(-65.2990847711306,1.87773280074162,7.));
#41708=CARTESIAN_POINT('Ctrl Pts',(-65.2861211425289,1.88102615439927,7.));
#41709=CARTESIAN_POINT('Ctrl Pts',(-65.273111817844,1.88418469347464,7.));
#41710=CARTESIAN_POINT('Ctrl Pts',(-65.2600590169346,1.88720850991533,7.));
#41711=CARTESIAN_POINT('Ctrl Pts',(-65.2488130849145,1.88981374647487,7.));
#41712=CARTESIAN_POINT('Ctrl Pts',(-65.2375439537466,1.89231686461784,7.));
#41713=CARTESIAN_POINT('Ctrl Pts',(-65.2262547951615,1.89471805492211,7.));
#41714=CARTESIAN_POINT('Ctrl Pts',(-65.1567411013575,1.90950353307062,7.));
#41715=CARTESIAN_POINT('Ctrl Pts',(-65.0864519774285,1.92043226303262,7.));
#41716=CARTESIAN_POINT('Ctrl Pts',(-65.0157547334709,1.92760520158801,7.));
#41717=CARTESIAN_POINT('Ctrl Pts',(-64.943565800346,1.93492948684578,7.));
#41718=CARTESIAN_POINT('Ctrl Pts',(-64.8709504429878,1.93833807717024,7.));
#41719=CARTESIAN_POINT('Ctrl Pts',(-64.7982722132928,1.93789067648522,7.));
#41720=CARTESIAN_POINT('Ctrl Pts',(-64.7251526999809,1.93744055929771,7.));
#41721=CARTESIAN_POINT('Ctrl Pts',(-64.6519684871743,1.93308764503056,7.));
#41722=CARTESIAN_POINT('Ctrl Pts',(-64.5790772350549,1.92484184820749,7.));
#41723=CARTESIAN_POINT('Ctrl Pts',(-64.5610671587083,1.92280446476293,7.));
#41724=CARTESIAN_POINT('Ctrl Pts',(-64.5430749514564,1.9205291753851,7.));
#41725=CARTESIAN_POINT('Ctrl Pts',(-64.5251060094349,1.91801563698977,7.));
#41726=CARTESIAN_POINT('Ctrl Pts',(-64.5110402166547,1.91604808040399,7.));
#41727=CARTESIAN_POINT('Ctrl Pts',(-64.4969870784137,1.9139341585107,7.));
#41728=CARTESIAN_POINT('Ctrl Pts',(-64.4829704723558,1.9116773971743,7.));
#41729=CARTESIAN_POINT('Ctrl Pts',(-64.408583493524,1.89970062782901,7.));
#41730=CARTESIAN_POINT('Ctrl Pts',(-64.3350918229631,1.88368734539382,6.99999999999999));
#41731=CARTESIAN_POINT('Ctrl Pts',(-64.262879083689,1.86371221647072,7.));
#41732=CARTESIAN_POINT('Ctrl Pts',(-64.1905873442587,1.8437152349172,7.));
#41733=CARTESIAN_POINT('Ctrl Pts',(-64.1195762102382,1.81974781464992,6.99999999999999));
#41734=CARTESIAN_POINT('Ctrl Pts',(-64.0502233635423,1.79183341393623,7.));
#41735=CARTESIAN_POINT('Ctrl Pts',(-63.9824494700609,1.76455453915751,7.));
#41736=CARTESIAN_POINT('Ctrl Pts',(-63.916258181573,1.73350624794761,7.));
#41737=CARTESIAN_POINT('Ctrl Pts',(-63.8520110121349,1.69866187350007,7.));
#41738=CARTESIAN_POINT('Ctrl Pts',(-63.8381915579471,1.6911669092769,7.));
#41739=CARTESIAN_POINT('Ctrl Pts',(-63.8244621191575,1.68349613170073,7.));
#41740=CARTESIAN_POINT('Ctrl Pts',(-63.8108264207747,1.67564897964535,7.));
#41741=CARTESIAN_POINT('Ctrl Pts',(-63.7992831576295,1.66900599455043,7.));
#41742=CARTESIAN_POINT('Ctrl Pts',(-63.7878070738684,1.66223660984748,7.));
#41743=CARTESIAN_POINT('Ctrl Pts',(-63.7763989699203,1.65534250909263,7.));
#41744=CARTESIAN_POINT('Ctrl Pts',(-63.1173724903363,0.823232180103149,
7.));
#41745=CARTESIAN_POINT('Ctrl Pts',(-63.0939903977405,0.752339169258933,
7.));
#41746=CARTESIAN_POINT('Ctrl Pts',(-63.0748445296608,0.680224887836885,
7.));
#41747=CARTESIAN_POINT('Ctrl Pts',(-63.0598471165381,0.607239755688797,
7.));
#41748=CARTESIAN_POINT('Ctrl Pts',(-63.045242974325,0.536168482221851,7.));
#41749=CARTESIAN_POINT('Ctrl Pts',(-63.0345730321077,0.4642705233706,7.));
#41750=CARTESIAN_POINT('Ctrl Pts',(-63.0278019508403,0.391872562027519,
7.));
#41751=CARTESIAN_POINT('Ctrl Pts',(-63.0262906434537,0.375713315160443,
7.));
#41752=CARTESIAN_POINT('Ctrl Pts',(-63.0249735943537,0.359527040989821,
7.));
#41753=CARTESIAN_POINT('Ctrl Pts',(-63.0238511666264,0.34332437073834,7.));
#41754=CARTESIAN_POINT('Ctrl Pts',(-63.0187005423181,0.268973153977023,
7.));
#41755=CARTESIAN_POINT('Ctrl Pts',(-63.0176530289114,0.194423667889717,
7.));
#41756=CARTESIAN_POINT('Ctrl Pts',(-63.0206465481662,0.120030528064432,
7.));
#41757=CARTESIAN_POINT('Ctrl Pts',(-63.0227481861611,0.0678018848184103,
7.));
#41758=CARTESIAN_POINT('Ctrl Pts',(-63.0268427413746,0.0156503275540584,
7.));
#41759=CARTESIAN_POINT('Ctrl Pts',(-63.0329233152999,-0.036296614856767,
7.));
#41760=CARTESIAN_POINT('Ctrl Pts',(-63.0352354057117,-0.056049031149148,
7.));
#41761=CARTESIAN_POINT('Ctrl Pts',(-63.0378347617044,-0.0757718050677318,
7.));
#41762=CARTESIAN_POINT('Ctrl Pts',(-63.0407214327969,-0.0954576801195959,
7.));
#41763=CARTESIAN_POINT('Ctrl Pts',(-63.0434693778843,-0.114197502533115,
7.));
#41764=CARTESIAN_POINT('Ctrl Pts',(-63.0464788571282,-0.1329097260904,7.));
#41765=CARTESIAN_POINT('Ctrl Pts',(-63.0497439151797,-0.151555113564703,
7.));
#41766=CARTESIAN_POINT('Ctrl Pts',(-63.0622655750455,-0.223061101005544,
7.));
#41767=CARTESIAN_POINT('Ctrl Pts',(-63.0785510722461,-0.293661819118036,
6.99999999999999));
#41768=CARTESIAN_POINT('Ctrl Pts',(-63.0985450713842,-0.363028531313167,
7.));
#41769=CARTESIAN_POINT('Ctrl Pts',(-63.118109525179,-0.430904988957711,
7.));
#41770=CARTESIAN_POINT('Ctrl Pts',(-63.1412253035865,-0.497600711633542,
7.));
#41771=CARTESIAN_POINT('Ctrl Pts',(-63.1678836571873,-0.562784339590762,
7.));
#41772=CARTESIAN_POINT('Ctrl Pts',(-63.1939574718371,-0.626538683126413,
7.));
#41773=CARTESIAN_POINT('Ctrl Pts',(-63.2234205963263,-0.688847181210932,
7.));
#41774=CARTESIAN_POINT('Ctrl Pts',(-63.2563003837665,-0.749366435838956,
7.));
#41775=CARTESIAN_POINT('Ctrl Pts',(-63.2669864355877,-0.7690354161301,7.));
#41776=CARTESIAN_POINT('Ctrl Pts',(-63.2780336415132,-0.788515094659207,
7.));
#41777=CARTESIAN_POINT('Ctrl Pts',(-63.2894436727967,-0.80779272412078,
7.));
#41778=CARTESIAN_POINT('Ctrl Pts',(-63.2958782979571,-0.818664238535167,
7.));
#41779=CARTESIAN_POINT('Ctrl Pts',(-63.3024290949197,-0.829472548274647,
7.));
#41780=CARTESIAN_POINT('Ctrl Pts',(-63.3090867443711,-0.840200273664074,
7.));
#41781=CARTESIAN_POINT('Ctrl Pts',(-63.3451024516394,-0.898233761323215,
7.));
#41782=CARTESIAN_POINT('Ctrl Pts',(-63.3843017903685,-0.954015012532752,
7.));
#41783=CARTESIAN_POINT('Ctrl Pts',(-63.426670904758,-1.00724100895717,7.));
#41784=CARTESIAN_POINT('Ctrl Pts',(-63.4327868741032,-1.01492416606788,
7.));
#41785=CARTESIAN_POINT('Ctrl Pts',(-63.4389689569132,-1.02255401966981,
6.99999999999999));
#41786=CARTESIAN_POINT('Ctrl Pts',(-63.4452171764819,-1.03012959441513,
6.99999999999999));
#41787=CARTESIAN_POINT('Ctrl Pts',(-63.489358667261,-1.08364838630305,7.));
#41788=CARTESIAN_POINT('Ctrl Pts',(-63.5367987510362,-1.13446181351563,
7.));
#41789=CARTESIAN_POINT('Ctrl Pts',(-63.5871991852739,-1.18242370278709,
7.));
#41790=CARTESIAN_POINT('Ctrl Pts',(-63.6342187269495,-1.2271682786137,7.));
#41791=CARTESIAN_POINT('Ctrl Pts',(-63.6838158179714,-1.26943087719056,
7.));
#41792=CARTESIAN_POINT('Ctrl Pts',(-63.7357299598937,-1.30905529562496,
7.));
#41793=CARTESIAN_POINT('Ctrl Pts',(-63.7471862226625,-1.31779949774095,
7.));
#41794=CARTESIAN_POINT('Ctrl Pts',(-63.7587553477597,-1.326415076375,6.99999999999999));
#41795=CARTESIAN_POINT('Ctrl Pts',(-63.7704345647747,-1.33490009616143,
6.99999999999999));
#41796=CARTESIAN_POINT('Ctrl Pts',(-63.7795655910355,-1.34153384039215,
6.99999999999999));
#41797=CARTESIAN_POINT('Ctrl Pts',(-63.7887633889776,-1.3480873027534,7.));
#41798=CARTESIAN_POINT('Ctrl Pts',(-63.7980157939557,-1.35455228245181,
7.));
#41799=CARTESIAN_POINT('Ctrl Pts',(-63.8540658571293,-1.39371642640913,
7.));
#41800=CARTESIAN_POINT('Ctrl Pts',(-63.912219564704,-1.42971188598758,7.));
#41801=CARTESIAN_POINT('Ctrl Pts',(-63.9721458438494,-1.46241564585894,
7.));
#41802=CARTESIAN_POINT('Ctrl Pts',(-64.0317950323718,-1.49496818817889,
7.));
#41803=CARTESIAN_POINT('Ctrl Pts',(-64.0932015440209,-1.52425966112384,
7.));
#41804=CARTESIAN_POINT('Ctrl Pts',(-64.1560527983748,-1.55011955109708,
7.));
#41805=CARTESIAN_POINT('Ctrl Pts',(-64.2175568101543,-1.57542512365694,
7.));
#41806=CARTESIAN_POINT('Ctrl Pts',(-64.2804452599811,-1.59744473905974,
7.));
#41807=CARTESIAN_POINT('Ctrl Pts',(-64.344423329557,-1.61596906267658,7.));
#41808=CARTESIAN_POINT('Ctrl Pts',(-64.3578992522694,-1.6198709052144,7.));
#41809=CARTESIAN_POINT('Ctrl Pts',(-64.3714234817642,-1.62361749283973,
7.));
#41810=CARTESIAN_POINT('Ctrl Pts',(-64.3849931909711,-1.62720657518054,
7.));
#41811=CARTESIAN_POINT('Ctrl Pts',(-64.3978648608679,-1.63061103156344,
7.));
#41812=CARTESIAN_POINT('Ctrl Pts',(-64.4107792257301,-1.63387407363082,
6.99999999999999));
#41813=CARTESIAN_POINT('Ctrl Pts',(-64.4237128649824,-1.63698901055556,
6.99999999999999));
#41814=CARTESIAN_POINT('Ctrl Pts',(-64.487243192052,-1.65228965082931,6.99999999999999));
#41815=CARTESIAN_POINT('Ctrl Pts',(-64.5513507147979,-1.6640519139839,6.99999999999999));
#41816=CARTESIAN_POINT('Ctrl Pts',(-64.6157505860683,-1.67213050417994,
7.));
#41817=CARTESIAN_POINT('Ctrl Pts',(-64.6789248748248,-1.68005535216058,
7.));
#41818=CARTESIAN_POINT('Ctrl Pts',(-64.7423813719211,-1.68443544217815,
7.));
#41819=CARTESIAN_POINT('Ctrl Pts',(-64.8058448176641,-1.68508431664668,
7.));
#41820=CARTESIAN_POINT('Ctrl Pts',(-64.8672458810559,-1.68571210453165,
7.));
#41821=CARTESIAN_POINT('Ctrl Pts',(-64.9286541093687,-1.68284715374126,
7.));
#41822=CARTESIAN_POINT('Ctrl Pts',(-64.9898031298831,-1.67627454330083,
7.));
#41823=CARTESIAN_POINT('Ctrl Pts',(-64.9999907154541,-1.67517952933783,
7.));
#41824=CARTESIAN_POINT('Ctrl Pts',(-65.0101710541419,-1.67398149896703,
7.));
#41825=CARTESIAN_POINT('Ctrl Pts',(-65.0203428468639,-1.6726793313447,7.));
#41826=CARTESIAN_POINT('Ctrl Pts',(-65.0310998269282,-1.6713022494933,7.));
#41827=CARTESIAN_POINT('Ctrl Pts',(-65.0418472497685,-1.66980870242006,
7.));
#41828=CARTESIAN_POINT('Ctrl Pts',(-65.0525835864496,-1.66819940096573,
7.));
#41829=CARTESIAN_POINT('Origin',(-65.,8.88178419700125E-15,-3.54592528053767));
#41830=CARTESIAN_POINT('Ctrl Pts',(-67.0565599569794,-0.00149374744777858,
-1.79592528053768));
#41831=CARTESIAN_POINT('Ctrl Pts',(-67.0573792182402,-0.099782513364621,
-1.79058130531689));
#41832=CARTESIAN_POINT('Ctrl Pts',(-67.0062893847297,-0.878608585113931,
-1.74819136657341));
#41833=CARTESIAN_POINT('Ctrl Pts',(-66.0109392265833,-2.20843178543787,
-1.66875546430726));
#41834=CARTESIAN_POINT('Ctrl Pts',(-63.6930089313552,-2.04686416993215,
-1.55761757373922));
#41835=CARTESIAN_POINT('Ctrl Pts',(-62.5713939614548,-0.0121365548742068,
-1.44647968317118));
#41836=CARTESIAN_POINT('Ctrl Pts',(-63.67270376601,2.03388137208554,-1.33534179260313));
#41837=CARTESIAN_POINT('Ctrl Pts',(-65.9889058463299,2.21817250383823,-1.22420390203509));
#41838=CARTESIAN_POINT('Ctrl Pts',(-67.0021432190354,0.892617277286203,
-1.14439839801327));
#41839=CARTESIAN_POINT('Ctrl Pts',(-67.057275270459,0.106740644746507,-1.10163885751414));
#41840=CARTESIAN_POINT('Ctrl Pts',(-67.0563730581704,0.00160407492546514,
-1.09592528053768));
#41841=CARTESIAN_POINT('Ctrl Pts',(-67.052679279082,0.0023836951352375,
-1.85407471946232));
#41842=CARTESIAN_POINT('Ctrl Pts',(-67.0491241057456,-0.467845902355823,
-1.82862455259619));
#41843=CARTESIAN_POINT('Ctrl Pts',(-66.6565276815742,-1.62960580042266,
-1.76612842220737));
#41844=CARTESIAN_POINT('Ctrl Pts',(-64.7278715623352,-2.41277602144419,
-1.66658632829587));
#41845=CARTESIAN_POINT('Ctrl Pts',(-62.8252644286755,-1.08095990301172,
-1.55544843772783));
#41846=CARTESIAN_POINT('Ctrl Pts',(-62.9123886677794,1.24138962897178,-1.44431054715979));
#41847=CARTESIAN_POINT('Ctrl Pts',(-64.9107473342681,2.42691462884513,-1.33317265659175));
#41848=CARTESIAN_POINT('Ctrl Pts',(-66.7212428925551,1.52545313603056,-1.23642738069259));
#41849=CARTESIAN_POINT('Ctrl Pts',(-67.0499074437772,0.4179188137684,-1.17672806831612));
#41850=CARTESIAN_POINT('Ctrl Pts',(-67.0520762837074,-0.0011613687935888,
-1.15407471946233));
#41851=CARTESIAN_POINT('Ctrl Pts',(-63.7309291201476,-1.0793586530485,-2.));
#41852=CARTESIAN_POINT('Ctrl Pts',(-63.3720166889934,-0.657362393039501,
-1.96295403647732));
#41853=CARTESIAN_POINT('Ctrl Pts',(-63.1146663550338,0.565736448038662,
-1.88886210943196));
#41854=CARTESIAN_POINT('Ctrl Pts',(-64.4549392280646,1.89346495741706,-1.77772421886392));
#41855=CARTESIAN_POINT('Ctrl Pts',(-66.2941885938804,1.48351678997985,-1.66658632829587));
#41856=CARTESIAN_POINT('Ctrl Pts',(-66.9487863029052,-0.282071400691224,
-1.55544843772784));
#41857=CARTESIAN_POINT('Ctrl Pts',(-65.8196738053231,-1.79060584233581,
-1.44431054715979));
#41858=CARTESIAN_POINT('Ctrl Pts',(-63.9402861076227,-1.65960613559165,
-1.33317265659175));
#41859=CARTESIAN_POINT('Ctrl Pts',(-63.0308759410067,-0.0098403700792925,
-1.22203476602371));
#41860=CARTESIAN_POINT('Ctrl Pts',(-63.9238225935869,1.64907962812727,-1.11089687545567));
#41861=CARTESIAN_POINT('Ctrl Pts',(-65.8018090473224,1.79850365805791,-0.999758984887623));
#41862=CARTESIAN_POINT('Ctrl Pts',(-66.9458893611786,0.301774776475135,
-0.888621094319584));
#41863=CARTESIAN_POINT('Ctrl Pts',(-66.3088756966202,-1.47119119673886,
-0.777483203751541));
#41864=CARTESIAN_POINT('Ctrl Pts',(-64.4738329478959,-1.89754943555686,
-0.666345313183499));
#41865=CARTESIAN_POINT('Ctrl Pts',(-63.1203970290852,-0.587064100833463,
-0.555207422615458));
#41866=CARTESIAN_POINT('Ctrl Pts',(-63.4873829445486,1.26077017125902,-0.444069532047416));
#41867=CARTESIAN_POINT('Ctrl Pts',(-65.2388844462753,1.95460593523977,-0.332931641479374));
#41868=CARTESIAN_POINT('Ctrl Pts',(-66.7717322843115,0.859369365311616,
-0.221793750911332));
#41869=CARTESIAN_POINT('Ctrl Pts',(-66.6828934802986,-1.02245805795663,
-0.11065586034329));
#41870=CARTESIAN_POINT('Ctrl Pts',(-65.0536831830854,-1.96841785926,0.000482030224751804));
#41871=CARTESIAN_POINT('Ctrl Pts',(-63.3753360623109,-1.11266255483749,
0.111619920792793));
#41872=CARTESIAN_POINT('Ctrl Pts',(-63.1840622672629,0.761525447206216,
0.222757811360836));
#41873=CARTESIAN_POINT('Ctrl Pts',(-64.654936873825,1.93868054946277,0.333895701928877));
#41874=CARTESIAN_POINT('Ctrl Pts',(-66.4416516727014,1.34133936965716,0.445033592496918));
#41875=CARTESIAN_POINT('Ctrl Pts',(-66.9088063462926,-0.483744952595402,
0.55617148306496));
#41876=CARTESIAN_POINT('Ctrl Pts',(-65.6288089236944,-1.86605203086769,
0.667309373633002));
#41877=CARTESIAN_POINT('Ctrl Pts',(-63.7732555621069,-1.54034052425233,
0.778447264201044));
#41878=CARTESIAN_POINT('Ctrl Pts',(-63.0405552967276,0.195262133588727,
0.889585154769085));
#41879=CARTESIAN_POINT('Ctrl Pts',(-64.1013569898796,1.75213914576361,1.00072304533713));
#41880=CARTESIAN_POINT('Ctrl Pts',(-65.9846968214939,1.70526332739896,1.11186093590517));
#41881=CARTESIAN_POINT('Ctrl Pts',(-66.9667324851762,0.0975406463696029,
1.22299882647321));
#41882=CARTESIAN_POINT('Ctrl Pts',(-66.148595600912,-1.59946209441982,1.33413671704125));
#41883=CARTESIAN_POINT('Ctrl Pts',(-64.2791361371736,-1.83245904107736,
1.4452746076093));
#41884=CARTESIAN_POINT('Ctrl Pts',(-63.0694915422322,-0.388185445925422,
1.55641249817734));
#41885=CARTESIAN_POINT('Ctrl Pts',(-63.6268632321408,1.41139869019815,1.66755038874538));
#41886=CARTESIAN_POINT('Ctrl Pts',(-65.441082578101,1.91911359883674,1.77868827931342));
#41887=CARTESIAN_POINT('Ctrl Pts',(-66.8515740381086,0.670242066229977,
1.88982616988146));
#41888=CARTESIAN_POINT('Ctrl Pts',(-66.5672987827578,-1.19210963065827,
2.0009640604495));
#41889=CARTESIAN_POINT('Ctrl Pts',(-64.8484571771716,-1.96330986316269,
2.11210195101754));
#41890=CARTESIAN_POINT('Ctrl Pts',(-63.2683244359328,-0.937470312465873,
2.22323984158559));
#41891=CARTESIAN_POINT('Ctrl Pts',(-63.2732139770213,0.946446446867298,
2.33437773215363));
#41892=CARTESIAN_POINT('Ctrl Pts',(-64.8586503480276,1.96407003995017,2.44551562272167));
#41893=CARTESIAN_POINT('Ctrl Pts',(-66.5734656584984,1.18395805139743,2.55665351328971));
#41894=CARTESIAN_POINT('Ctrl Pts',(-66.8480700074313,-0.679844168596873,
2.66779140385775));
#41895=CARTESIAN_POINT('Ctrl Pts',(-65.4311149200231,-1.92137731111721,
2.7789292944258));
#41896=CARTESIAN_POINT('Ctrl Pts',(-63.6195554571419,-1.40425201087121,
2.89006718499384));
#41897=CARTESIAN_POINT('Ctrl Pts',(-63.0715325396448,0.398201080226113,
3.00120507556188));
#41898=CARTESIAN_POINT('Ctrl Pts',(-64.2886577589191,1.83617620668519,3.11234296612993));
#41899=CARTESIAN_POINT('Ctrl Pts',(-66.1568825986246,1.59347842751064,3.22348085669796));
#41900=CARTESIAN_POINT('Ctrl Pts',(-66.9661996758679,-0.107748227638456,
3.33461874726601));
#41901=CARTESIAN_POINT('Ctrl Pts',(-65.9758318915686,-1.71035170808284,
3.44575663783405));
#41902=CARTESIAN_POINT('Ctrl Pts',(-64.0922741102298,-1.74745087340982,
3.55689452840209));
#41903=CARTESIAN_POINT('Ctrl Pts',(-63.0395681301102,-0.185088436867097,
3.66803241897013));
#41904=CARTESIAN_POINT('Ctrl Pts',(-63.7812676733088,1.5466875449918,3.77917030953817));
#41905=CARTESIAN_POINT('Ctrl Pts',(-65.6384867364954,1.86276287627796,3.89030820010621));
#41906=CARTESIAN_POINT('Ctrl Pts',(-66.9112916488297,0.473830221762723,
4.00144609067426));
#41907=CARTESIAN_POINT('Ctrl Pts',(-66.4346696394808,-1.34880460837871,
4.11258398124229));
#41908=CARTESIAN_POINT('Ctrl Pts',(-64.6448782388305,-1.93686328389462,
4.22372187181034));
#41909=CARTESIAN_POINT('Ctrl Pts',(-63.1801338135814,-0.752089030319253,
4.33485976237838));
#41910=CARTESIAN_POINT('Ctrl Pts',(-63.3811335473526,1.12108084233402,4.44599765294643));
#41911=CARTESIAN_POINT('Ctrl Pts',(-65.0639001046135,1.96811270537377,4.55713554351446));
#41912=CARTESIAN_POINT('Ctrl Pts',(-66.6881781710758,1.01370869065611,4.66827343408251));
#41913=CARTESIAN_POINT('Ctrl Pts',(-66.767247613038,-0.868554387592529,
4.77941132465054));
#41914=CARTESIAN_POINT('Ctrl Pts',(-65.2287352713999,-1.95581977940925,
4.8905492152186));
#41915=CARTESIAN_POINT('Ctrl Pts',(-63.4808589446451,-1.25290115725712,
5.00168710578663));
#41916=CARTESIAN_POINT('Ctrl Pts',(-63.1234696485087,0.596812123952627,
5.11282499635468));
#41917=CARTESIAN_POINT('Ctrl Pts',(-64.483689875393,1.90025645848878,5.22396288692272));
#41918=CARTESIAN_POINT('Ctrl Pts',(-66.3164945930014,1.46437458763455,5.33510077749075));
#41919=CARTESIAN_POINT('Ctrl Pts',(-66.9442969223188,-0.311866110966441,
5.44623866805881));
#41920=CARTESIAN_POINT('Ctrl Pts',(-65.7924621445391,-1.80265190489435,
5.55737655862683));
#41921=CARTESIAN_POINT('Ctrl Pts',(-63.9152779448642,-1.64345059076356,
5.66851444919488));
#41922=CARTESIAN_POINT('Ctrl Pts',(-63.0309518163246,0.0200209171529774,
5.77965233976292));
#41923=CARTESIAN_POINT('Ctrl Pts',(-63.9489184664916,1.6651646276029,5.89079023033097));
#41924=CARTESIAN_POINT('Ctrl Pts',(-65.8289506914941,1.78616905068825,6.001928120899));
#41925=CARTESIAN_POINT('Ctrl Pts',(-66.9502374569467,0.272263260809152,
6.11306601146705));
#41926=CARTESIAN_POINT('Ctrl Pts',(-66.2864448139981,-1.49082960024053,
6.22420390203509));
#41927=CARTESIAN_POINT('Ctrl Pts',(-64.4451643957601,-1.88938584790037,
6.33534179260314));
#41928=CARTESIAN_POINT('Ctrl Pts',(-63.1117120727514,-0.558493595662741,
6.44647968317117));
#41929=CARTESIAN_POINT('Ctrl Pts',(-63.5066690059847,1.28345183053528,6.55761757373921));
#41930=CARTESIAN_POINT('Ctrl Pts',(-65.2684140085621,1.95091987271334,6.66875546430726));
#41931=CARTESIAN_POINT('Ctrl Pts',(-66.7846240008828,0.832135508767313,
6.77989335487529));
#41932=CARTESIAN_POINT('Ctrl Pts',(-66.6670561422041,-1.04722013035561,
6.89103124544334));
#41933=CARTESIAN_POINT('Ctrl Pts',(-65.0241955006465,-1.97020693527805,
7.00216913601138));
#41934=CARTESIAN_POINT('Ctrl Pts',(-63.3579443006206,-1.08544634211746,
7.11330702657943));
#41935=CARTESIAN_POINT('Ctrl Pts',(-63.2516046182892,0.1599017382992,7.18739895362479));
#41936=CARTESIAN_POINT('Ctrl Pts',(-63.4735576439471,0.667480137268208,
7.22444491714747));
#41937=CARTESIAN_POINT('Ctrl Pts',(-63.6322193753412,-1.16331236980973,
-2.07481497238249));
#41938=CARTESIAN_POINT('Ctrl Pts',(-63.2453903360215,-0.708492771249607,
-2.03776900885981));
#41939=CARTESIAN_POINT('Ctrl Pts',(-62.9680230067985,0.609740058317781,
-1.96367708181445));
#41940=CARTESIAN_POINT('Ctrl Pts',(-64.4125437948732,2.04074076818054,-1.85253919124641));
#41941=CARTESIAN_POINT('Ctrl Pts',(-66.3948520224261,1.59890637623529,-1.74140130067836));
#41942=CARTESIAN_POINT('Ctrl Pts',(-67.1003650694627,-0.304011228025904,
-1.63026341011032));
#41943=CARTESIAN_POINT('Ctrl Pts',(-65.8834289457431,-1.92988115670316,
-1.51912551954228));
#41944=CARTESIAN_POINT('Ctrl Pts',(-63.8578603822002,-1.78869214703848,
-1.40798762897424));
#41945=CARTESIAN_POINT('Ctrl Pts',(-62.8777152811561,-0.010605765010931,
-1.2968497384062));
#41946=CARTESIAN_POINT('Ctrl Pts',(-63.8401163177279,1.77734687611336,-1.18571184783815));
#41947=CARTESIAN_POINT('Ctrl Pts',(-65.8641746469915,1.93839327331802,-1.07457395727011));
#41948=CARTESIAN_POINT('Ctrl Pts',(-67.0972428003859,0.325247154297205,
-0.963436066702072));
#41949=CARTESIAN_POINT('Ctrl Pts',(-66.4106815043556,-1.58562208464047,
-0.852298176134029));
#41950=CARTESIAN_POINT('Ctrl Pts',(-64.4329070892513,-2.04514294157382,
-0.741160285565989));
#41951=CARTESIAN_POINT('Ctrl Pts',(-62.9741994190526,-0.632726599672803,
-0.630022394997946));
#41952=CARTESIAN_POINT('Ctrl Pts',(-63.3697299072724,1.358834277717,-0.518884504429905));
#41953=CARTESIAN_POINT('Ctrl Pts',(-65.2574651442524,2.10663735927427,-0.407746613861863));
#41954=CARTESIAN_POINT('Ctrl Pts',(-66.9095395923399,0.926212070546691,
-0.296608723293821));
#41955=CARTESIAN_POINT('Ctrl Pts',(-66.8137908073226,-1.10198598313283,
-0.185470832725779));
#41956=CARTESIAN_POINT('Ctrl Pts',(-65.0578587207854,-2.12152359010981,
-0.0743329421577371));
#41957=CARTESIAN_POINT('Ctrl Pts',(-63.2489678938882,-1.19920668612862,
0.036804948410304));
#41958=CARTESIAN_POINT('Ctrl Pts',(-63.0428166102798,0.820757743645075,
0.147942838978346));
#41959=CARTESIAN_POINT('Ctrl Pts',(-64.6280974800075,2.08947327927542,0.259080729546388));
#41960=CARTESIAN_POINT('Ctrl Pts',(-66.5537849435622,1.44567023799534,0.370218620114429));
#41961=CARTESIAN_POINT('Ctrl Pts',(-67.0572754273494,-0.521371173147915,
0.481356510682472));
#41962=CARTESIAN_POINT('Ctrl Pts',(-65.6777183812947,-2.01119563370879,
0.592494401250513));
#41963=CARTESIAN_POINT('Ctrl Pts',(-63.6778380150419,-1.66014992377275,
0.703632291818555));
#41964=CARTESIAN_POINT('Ctrl Pts',(-62.8881475079326,0.210449839557635,
0.814770182386596));
#41965=CARTESIAN_POINT('Ctrl Pts',(-64.0314595368616,1.88842247767949,0.925908072954638));
#41966=CARTESIAN_POINT('Ctrl Pts',(-66.0612876356907,1.83790060601568,1.03704596352268));
#41967=CARTESIAN_POINT('Ctrl Pts',(-67.1197071257548,0.105127466352834,
1.14818385409072));
#41968=CARTESIAN_POINT('Ctrl Pts',(-66.2379346445003,-1.72387003543737,
1.25932174465876));
#41969=CARTESIAN_POINT('Ctrl Pts',(-64.2230665440017,-1.97498974380221,
1.37045963522681));
#41970=CARTESIAN_POINT('Ctrl Pts',(-62.9193344468026,-0.418378941744453,
1.48159752579485));
#41971=CARTESIAN_POINT('Ctrl Pts',(-63.5200591267976,1.52117885042515,1.59273541636289));
#41972=CARTESIAN_POINT('Ctrl Pts',(-65.4753904717057,2.06838438946255,1.70387330693093));
#41973=CARTESIAN_POINT('Ctrl Pts',(-66.995591526567,0.722374239748765,1.81501119749897));
#41974=CARTESIAN_POINT('Ctrl Pts',(-66.6892050256144,-1.28483324388724,
1.92614908806702));
#41975=CARTESIAN_POINT('Ctrl Pts',(-64.8366700078289,-2.11601828839368,
2.03728697863506));
#41976=CARTESIAN_POINT('Ctrl Pts',(-63.1336327841659,-1.01038779625361,
2.1484248692031));
#41977=CARTESIAN_POINT('Ctrl Pts',(-63.1389026391995,1.02006210437423,2.25956275977114));
#41978=CARTESIAN_POINT('Ctrl Pts',(-64.8476560148535,2.11683759257734,2.37070065033918));
#41979=CARTESIAN_POINT('Ctrl Pts',(-66.6958515678104,1.27604762572331,2.48183854090722));
#41980=CARTESIAN_POINT('Ctrl Pts',(-66.9918149484855,-0.732723204319568,
2.59297643147526));
#41981=CARTESIAN_POINT('Ctrl Pts',(-65.4646475180941,-2.07082417580245,
2.70411432204331));
#41982=CARTESIAN_POINT('Ctrl Pts',(-63.5121829449299,-1.51347629442987,
2.81525221261135));
#41983=CARTESIAN_POINT('Ctrl Pts',(-62.9215341952643,0.429173603222892,
2.92639010317939));
#41984=CARTESIAN_POINT('Ctrl Pts',(-64.2333287680788,1.97899603468616,3.03752799374743));
#41985=CARTESIAN_POINT('Ctrl Pts',(-66.2468662141138,1.71742095225949,3.14866588431547));
#41986=CARTESIAN_POINT('Ctrl Pts',(-67.1191328739459,-0.116129004648151,
3.25980377488352));
#41987=CARTESIAN_POINT('Ctrl Pts',(-66.051733181654,-1.8433847666097,3.37094166545155));
#41988=CARTESIAN_POINT('Ctrl Pts',(-64.0216701807284,-1.88336954628658,
3.4820795560196));
#41989=CARTESIAN_POINT('Ctrl Pts',(-62.8870835583976,-0.199484821387324,
3.59321744658764));
#41990=CARTESIAN_POINT('Ctrl Pts',(-63.686473317166,1.66699062284606,3.70435533715568));
#41991=CARTESIAN_POINT('Ctrl Pts',(-65.6881489451415,2.00765064501607,3.81549322772372));
#41992=CARTESIAN_POINT('Ctrl Pts',(-67.0599540394824,0.510685263521478,
3.92663111829177));
#41993=CARTESIAN_POINT('Ctrl Pts',(-66.5462598400307,-1.45371613128932,
4.03776900885981));
#41994=CARTESIAN_POINT('Ctrl Pts',(-64.6172564731933,-2.08751466476978,
4.14890689942785));
#41995=CARTESIAN_POINT('Ctrl Pts',(-63.0385825971008,-0.81058735175515,
4.26004478999589));
#41996=CARTESIAN_POINT('Ctrl Pts',(-63.2552163137658,1.20827975739151,4.37118268056393));
#41997=CARTESIAN_POINT('Ctrl Pts',(-65.0688703258357,2.12119470101483,4.48232057113198));
#41998=CARTESIAN_POINT('Ctrl Pts',(-66.8194865472274,1.09255608031048,4.59345846170002));
#41999=CARTESIAN_POINT('Ctrl Pts',(-66.9047060983459,-0.936111514078443,
4.70459635226806));
#42000=CARTESIAN_POINT('Ctrl Pts',(-65.2465265552648,-2.1079456175936,4.8157342428361));
#42001=CARTESIAN_POINT('Ctrl Pts',(-63.3626984633988,-1.35035320305218,
4.92687213340414));
#42002=CARTESIAN_POINT('Ctrl Pts',(-62.9775110302329,0.643232834874313,
5.03801002397219));
#42003=CARTESIAN_POINT('Ctrl Pts',(-64.4435306995345,2.04806051976079,5.14914791454023));
#42004=CARTESIAN_POINT('Ctrl Pts',(-66.4188930069729,1.57827527209693,5.26028580510827));
#42005=CARTESIAN_POINT('Ctrl Pts',(-67.0955264998601,-0.336123404011301,
5.37142369567631));
#42006=CARTESIAN_POINT('Ctrl Pts',(-65.8541007317118,-1.94286417540809,
5.48256158624435));
#42007=CARTESIAN_POINT('Ctrl Pts',(-63.8309070567223,-1.77128000596151,
5.5936994768124));
#42008=CARTESIAN_POINT('Ctrl Pts',(-62.8777970581406,0.0215781663613025,
5.70483736738043));
#42009=CARTESIAN_POINT('Ctrl Pts',(-63.867164175545,1.79468298474188,5.81597525794848));
#42010=CARTESIAN_POINT('Ctrl Pts',(-65.8934273984406,1.92509926646557,5.92711314851651));
#42011=CARTESIAN_POINT('Ctrl Pts',(-67.1019290958798,0.293440200112785,
6.03825103908457));
#42012=CARTESIAN_POINT('Ctrl Pts',(-66.3865059227299,-1.60678798501314,
6.14938892965259));
#42013=CARTESIAN_POINT('Ctrl Pts',(-64.4020086652382,-2.03634438098786,
6.26052682022066));
#42014=CARTESIAN_POINT('Ctrl Pts',(-62.9648389371536,-0.601933848826785,
6.37166471078868));
#42015=CARTESIAN_POINT('Ctrl Pts',(-63.3905160600216,1.38328014168386,6.48280260135673));
#42016=CARTESIAN_POINT('Ctrl Pts',(-65.2892915487438,2.10266459070399,6.59394049192477));
#42017=CARTESIAN_POINT('Ctrl Pts',(-66.9234340409675,0.896859934344202,
6.70507838249281));
#42018=CARTESIAN_POINT('Ctrl Pts',(-66.796721623453,-1.12867407706945,6.81621627306086));
#42019=CARTESIAN_POINT('Ctrl Pts',(-65.026077453603,-2.12345182245078,6.92735416362889));
#42020=CARTESIAN_POINT('Ctrl Pts',(-63.2302233816263,-1.16987356610669,
7.03849205419693));
#42021=CARTESIAN_POINT('Ctrl Pts',(-63.1156124805061,0.172339073385996,
7.1125839812423));
#42022=CARTESIAN_POINT('Ctrl Pts',(-63.3548292594101,0.719397484879855,
7.14962994476498));
#42023=CARTESIAN_POINT('Ctrl Pts',(-63.5335096305347,-1.24726608657095,
-2.14962994476498));
#42024=CARTESIAN_POINT('Ctrl Pts',(-63.1187639830495,-0.759623149459712,
-2.1125839812423));
#42025=CARTESIAN_POINT('Ctrl Pts',(-62.8213796585631,0.653743668596897,
-2.03849205419694));
#42026=CARTESIAN_POINT('Ctrl Pts',(-64.370148361682,2.18801657894402,-1.9273541636289));
#42027=CARTESIAN_POINT('Ctrl Pts',(-66.4955154509718,1.71429596249072,-1.81621627306085));
#42028=CARTESIAN_POINT('Ctrl Pts',(-67.2519438360201,-0.325951055360581,
-1.70507838249281));
#42029=CARTESIAN_POINT('Ctrl Pts',(-65.9471840861633,-2.06915647107052,
-1.59394049192477));
#42030=CARTESIAN_POINT('Ctrl Pts',(-63.7754346567777,-1.91777815848532,
-1.48280260135673));
#42031=CARTESIAN_POINT('Ctrl Pts',(-62.7245546213054,-0.0113711599425682,
-1.37166471078869));
#42032=CARTESIAN_POINT('Ctrl Pts',(-63.756410041869,1.90561412409945,-1.26052682022064));
#42033=CARTESIAN_POINT('Ctrl Pts',(-65.9265402466607,2.07828288857813,-1.1493889296526));
#42034=CARTESIAN_POINT('Ctrl Pts',(-67.2485962395932,0.348719532119274,
-1.03825103908456));
#42035=CARTESIAN_POINT('Ctrl Pts',(-66.5124873120909,-1.70005297254208,
-0.927113148516519));
#42036=CARTESIAN_POINT('Ctrl Pts',(-64.3919812306068,-2.19273644759077,
-0.815975257948477));
#42037=CARTESIAN_POINT('Ctrl Pts',(-62.8280018090199,-0.67838909851214,
-0.704837367380436));
#42038=CARTESIAN_POINT('Ctrl Pts',(-63.2520768699961,1.45689838417497,-0.593699476812394));
#42039=CARTESIAN_POINT('Ctrl Pts',(-65.2760458422295,2.25866878330877,-0.482561586244352));
#42040=CARTESIAN_POINT('Ctrl Pts',(-67.0473469003682,0.993054775781761,
-0.37142369567631));
#42041=CARTESIAN_POINT('Ctrl Pts',(-66.9446881343466,-1.18151390830903,
-0.260285805108268));
#42042=CARTESIAN_POINT('Ctrl Pts',(-65.0620342584853,-2.27462932095962,
-0.149147914540226));
#42043=CARTESIAN_POINT('Ctrl Pts',(-63.1225997254656,-1.28575081741975,
-0.0380100239721848));
#42044=CARTESIAN_POINT('Ctrl Pts',(-62.9015709532967,0.879990040083932,
0.0731278665958575));
#42045=CARTESIAN_POINT('Ctrl Pts',(-64.6012580861897,2.24026600908808,0.184265757163899));
#42046=CARTESIAN_POINT('Ctrl Pts',(-66.6659182144232,1.55000110633352,0.295403647731941));
#42047=CARTESIAN_POINT('Ctrl Pts',(-67.2057445084059,-0.55899739370043,
0.406541538299982));
#42048=CARTESIAN_POINT('Ctrl Pts',(-65.7266278388951,-2.15633923654989,
0.517679428868024));
#42049=CARTESIAN_POINT('Ctrl Pts',(-63.5824204679769,-1.77995932329318,
0.628817319436066));
#42050=CARTESIAN_POINT('Ctrl Pts',(-62.7357397191377,0.225637545526547,
0.739955210004107));
#42051=CARTESIAN_POINT('Ctrl Pts',(-63.9615620838435,2.02470580959538,0.85109310057215));
#42052=CARTESIAN_POINT('Ctrl Pts',(-66.1378784498875,1.97053788463239,0.96223099114019));
#42053=CARTESIAN_POINT('Ctrl Pts',(-67.2726817663336,0.11271428633606,1.07336888170823));
#42054=CARTESIAN_POINT('Ctrl Pts',(-66.3272736880886,-1.84827797645492,
1.18450677227627));
#42055=CARTESIAN_POINT('Ctrl Pts',(-64.1669969508297,-2.11752044652707,
1.29564466284432));
#42056=CARTESIAN_POINT('Ctrl Pts',(-62.7691773513729,-0.44857243756348,
1.40678255341236));
#42057=CARTESIAN_POINT('Ctrl Pts',(-63.4132550214545,1.63095901065214,1.5179204439804));
#42058=CARTESIAN_POINT('Ctrl Pts',(-65.5096983653104,2.21765518008836,1.62905833454844));
#42059=CARTESIAN_POINT('Ctrl Pts',(-67.1396090150254,0.774506413267552,
1.74019622511649));
#42060=CARTESIAN_POINT('Ctrl Pts',(-66.8111112684709,-1.37755685711622,
1.85133411568452));
#42061=CARTESIAN_POINT('Ctrl Pts',(-64.8248828384863,-2.26872671362467,
1.96247200625257));
#42062=CARTESIAN_POINT('Ctrl Pts',(-62.9989411323989,-1.08330528004135,
2.07360989682061));
#42063=CARTESIAN_POINT('Ctrl Pts',(-63.0045913013778,1.09367776188117,2.18474778738865));
#42064=CARTESIAN_POINT('Ctrl Pts',(-64.8366616816794,2.26960514520452,2.29588567795669));
#42065=CARTESIAN_POINT('Ctrl Pts',(-66.8182374771223,1.36813720004919,2.40702356852474));
#42066=CARTESIAN_POINT('Ctrl Pts',(-67.1355598895398,-0.785602240042267,
2.51816145909277));
#42067=CARTESIAN_POINT('Ctrl Pts',(-65.4981801161651,-2.22027104048769,
2.62929934966082));
#42068=CARTESIAN_POINT('Ctrl Pts',(-63.4048104327177,-1.62270057798853,
2.74043724022886));
#42069=CARTESIAN_POINT('Ctrl Pts',(-62.771535850884,0.460146126219668,2.8515751307969));
#42070=CARTESIAN_POINT('Ctrl Pts',(-64.1779997772384,2.12181586268714,2.96271302136494));
#42071=CARTESIAN_POINT('Ctrl Pts',(-66.3368498296032,1.84136347700834,3.07385091193299));
#42072=CARTESIAN_POINT('Ctrl Pts',(-67.2720660720238,-0.124509781657844,
3.18498880250102));
#42073=CARTESIAN_POINT('Ctrl Pts',(-66.1276344717396,-1.97641782513655,
3.29612669306907));
#42074=CARTESIAN_POINT('Ctrl Pts',(-63.9510662512269,-2.01928821916335,
3.40726458363711));
#42075=CARTESIAN_POINT('Ctrl Pts',(-62.734598986685,-0.213881205907549,
3.51840247420515));
#42076=CARTESIAN_POINT('Ctrl Pts',(-63.5916789610234,1.78729370070031,3.62954036477319));
#42077=CARTESIAN_POINT('Ctrl Pts',(-65.7378111537875,2.15253841375417,3.74067825534123));
#42078=CARTESIAN_POINT('Ctrl Pts',(-67.2086164301352,0.547540305280233,
3.85181614590928));
#42079=CARTESIAN_POINT('Ctrl Pts',(-66.6578500405806,-1.55862765419993,
3.96295403647732));
#42080=CARTESIAN_POINT('Ctrl Pts',(-64.589634707556,-2.23816604564494,4.07409192704536));
#42081=CARTESIAN_POINT('Ctrl Pts',(-62.8970313806202,-0.869085673191047,
4.1852298176134));
#42082=CARTESIAN_POINT('Ctrl Pts',(-63.1292990801791,1.29547867244901,4.29636770818144));
#42083=CARTESIAN_POINT('Ctrl Pts',(-65.0738405470579,2.2742766966559,4.40750559874948));
#42084=CARTESIAN_POINT('Ctrl Pts',(-66.9507949233791,1.17140346996485,4.51864348931753));
#42085=CARTESIAN_POINT('Ctrl Pts',(-67.0421645836536,-1.00366864056436,
4.62978137988557));
#42086=CARTESIAN_POINT('Ctrl Pts',(-65.2643178391297,-2.26007145577794,
4.74091927045361));
#42087=CARTESIAN_POINT('Ctrl Pts',(-63.2445379821525,-1.44780524884724,
4.85205716102165));
#42088=CARTESIAN_POINT('Ctrl Pts',(-62.8315524119571,0.689653545795996,
4.96319505158969));
#42089=CARTESIAN_POINT('Ctrl Pts',(-64.4033715236759,2.1958645810328,5.07433294215774));
#42090=CARTESIAN_POINT('Ctrl Pts',(-66.5212914209443,1.6921759565593,5.18547083272578));
#42091=CARTESIAN_POINT('Ctrl Pts',(-67.2467560774014,-0.360380697056161,
5.29660872329382));
#42092=CARTESIAN_POINT('Ctrl Pts',(-65.9157393188846,-2.08307644592183,
5.40774661386186));
#42093=CARTESIAN_POINT('Ctrl Pts',(-63.7465361685802,-1.89910942115946,
5.5188845044299));
#42094=CARTESIAN_POINT('Ctrl Pts',(-62.7246422999565,0.0231354155696304,
5.63002239499795));
#42095=CARTESIAN_POINT('Ctrl Pts',(-63.7854098845984,1.92420134188086,5.74116028556599));
#42096=CARTESIAN_POINT('Ctrl Pts',(-65.957904105387,2.0640294822429,5.85229817613403));
#42097=CARTESIAN_POINT('Ctrl Pts',(-67.2536207348131,0.314617139416418,
5.96343606670207));
#42098=CARTESIAN_POINT('Ctrl Pts',(-66.4865670314617,-1.72274636978575,
6.07457395727011));
#42099=CARTESIAN_POINT('Ctrl Pts',(-64.3588529347165,-2.18330291407535,
6.18571184783816));
#42100=CARTESIAN_POINT('Ctrl Pts',(-62.8179658015557,-0.645374101990828,
6.29684973840619));
#42101=CARTESIAN_POINT('Ctrl Pts',(-63.2743631140587,1.48310845283244,6.40798762897424));
#42102=CARTESIAN_POINT('Ctrl Pts',(-65.3101690889255,2.25440930869465,6.51912551954228));
#42103=CARTESIAN_POINT('Ctrl Pts',(-67.0622440810523,0.96158435992109,6.63026341011032));
#42104=CARTESIAN_POINT('Ctrl Pts',(-66.9263871047018,-1.21012802378328,
6.74140130067837));
#42105=CARTESIAN_POINT('Ctrl Pts',(-65.0279594065595,-2.27669670962352,
6.8525391912464));
#42106=CARTESIAN_POINT('Ctrl Pts',(-63.1025024626319,-1.25430079009592,
6.96367708181444));
#42107=CARTESIAN_POINT('Ctrl Pts',(-62.979620342723,0.184776408472793,7.03776900885981));
#42108=CARTESIAN_POINT('Ctrl Pts',(-63.2361008748732,0.771314832491502,
7.07481497238249));
#42109=CARTESIAN_POINT('Ctrl Pts',(-63.4347998857283,-1.33121980333218,
-2.22444491714747));
#42110=CARTESIAN_POINT('Ctrl Pts',(-62.9921376300776,-0.810753527669818,
-2.18739895362479));
#42111=CARTESIAN_POINT('Ctrl Pts',(-62.6747363103277,0.697747278876015,
-2.11330702657943));
#42112=CARTESIAN_POINT('Ctrl Pts',(-64.3277529284907,2.3352923897075,-2.00216913601138));
#42113=CARTESIAN_POINT('Ctrl Pts',(-66.5961788795174,1.82968554874616,-1.89103124544334));
#42114=CARTESIAN_POINT('Ctrl Pts',(-67.4035226025776,-0.347890882695259,
-1.7798933548753));
#42115=CARTESIAN_POINT('Ctrl Pts',(-66.0109392265833,-2.20843178543787,
-1.66875546430726));
#42116=CARTESIAN_POINT('Ctrl Pts',(-63.6930089313552,-2.04686416993215,
-1.55761757373922));
#42117=CARTESIAN_POINT('Ctrl Pts',(-62.5713939614548,-0.0121365548742068,
-1.44647968317118));
#42118=CARTESIAN_POINT('Ctrl Pts',(-63.67270376601,2.03388137208554,-1.33534179260313));
#42119=CARTESIAN_POINT('Ctrl Pts',(-65.9889058463299,2.21817250383823,-1.22420390203509));
#42120=CARTESIAN_POINT('Ctrl Pts',(-67.3999496788005,0.372191909941345,
-1.11306601146705));
#42121=CARTESIAN_POINT('Ctrl Pts',(-66.6142931198262,-1.81448386044369,
-1.00192812089901));
#42122=CARTESIAN_POINT('Ctrl Pts',(-64.3510553719621,-2.34032995360773,
-0.890790230330967));
#42123=CARTESIAN_POINT('Ctrl Pts',(-62.6818041989874,-0.724051597351479,
-0.779652339762924));
#42124=CARTESIAN_POINT('Ctrl Pts',(-63.1344238327198,1.55496249063294,-0.668514449194883));
#42125=CARTESIAN_POINT('Ctrl Pts',(-65.2946265402067,2.41070020734328,-0.55737655862684));
#42126=CARTESIAN_POINT('Ctrl Pts',(-67.1851542083967,1.05989748101683,-0.446238668058799));
#42127=CARTESIAN_POINT('Ctrl Pts',(-67.0755854613707,-1.26104183348523,
-0.335100777490757));
#42128=CARTESIAN_POINT('Ctrl Pts',(-65.0662097961853,-2.42773505180942,
-0.223962886922715));
#42129=CARTESIAN_POINT('Ctrl Pts',(-62.9962315570428,-1.37229494871089,
-0.112824996354674));
#42130=CARTESIAN_POINT('Ctrl Pts',(-62.7603252963136,0.939222336522791,
-0.00168710578663132));
#42131=CARTESIAN_POINT('Ctrl Pts',(-64.5744186923722,2.39105873890073,0.10945078478141));
#42132=CARTESIAN_POINT('Ctrl Pts',(-66.778051485284,1.6543319746717,0.220588675349452));
#42133=CARTESIAN_POINT('Ctrl Pts',(-67.3542135894627,-0.596623614252945,
0.331726565917493));
#42134=CARTESIAN_POINT('Ctrl Pts',(-65.7755372964953,-2.30148283939099,
0.442864456485536));
#42135=CARTESIAN_POINT('Ctrl Pts',(-63.4870029209119,-1.89976872281361,
0.554002347053577));
#42136=CARTESIAN_POINT('Ctrl Pts',(-62.5833319303427,0.240825251495458,
0.665140237621619));
#42137=CARTESIAN_POINT('Ctrl Pts',(-63.8916646308255,2.16098914151126,0.77627812818966));
#42138=CARTESIAN_POINT('Ctrl Pts',(-66.2144692640843,2.10317516324911,0.887416018757702));
#42139=CARTESIAN_POINT('Ctrl Pts',(-67.4256564069122,0.12030110631929,0.998553909325744));
#42140=CARTESIAN_POINT('Ctrl Pts',(-66.416612731677,-1.97268591747247,1.10969179989378));
#42141=CARTESIAN_POINT('Ctrl Pts',(-64.1109273576576,-2.26005114925192,
1.22082969046183));
#42142=CARTESIAN_POINT('Ctrl Pts',(-62.6190202559434,-0.47876593338251,
1.33196758102987));
#42143=CARTESIAN_POINT('Ctrl Pts',(-63.3064509161112,1.74073917087914,1.44310547159791));
#42144=CARTESIAN_POINT('Ctrl Pts',(-65.5440062589152,2.36692597071417,1.55424336216595));
#42145=CARTESIAN_POINT('Ctrl Pts',(-67.2836265034836,0.82663858678634,1.665381252734));
#42146=CARTESIAN_POINT('Ctrl Pts',(-66.9330175113275,-1.47028047034519,
1.77651914330204));
#42147=CARTESIAN_POINT('Ctrl Pts',(-64.8130956691436,-2.42143513885566,
1.88765703387008));
#42148=CARTESIAN_POINT('Ctrl Pts',(-62.864249480632,-1.15622276382909,1.99879492443812));
#42149=CARTESIAN_POINT('Ctrl Pts',(-62.8702799635561,1.1672934193881,2.10993281500616));
#42150=CARTESIAN_POINT('Ctrl Pts',(-64.8256673485052,2.42237269783169,2.2210707055742));
#42151=CARTESIAN_POINT('Ctrl Pts',(-66.9406233864343,1.46022677437507,2.33220859614225));
#42152=CARTESIAN_POINT('Ctrl Pts',(-67.279304830594,-0.838481275764962,
2.44334648671029));
#42153=CARTESIAN_POINT('Ctrl Pts',(-65.5317127142361,-2.36971790517293,
2.55448437727833));
#42154=CARTESIAN_POINT('Ctrl Pts',(-63.2974379205056,-1.73192486154719,
2.66562226784637));
#42155=CARTESIAN_POINT('Ctrl Pts',(-62.6215375065036,0.491118649216447,
2.77676015841441));
#42156=CARTESIAN_POINT('Ctrl Pts',(-64.122670786398,2.26463569068811,2.88789804898245));
#42157=CARTESIAN_POINT('Ctrl Pts',(-66.4268334450924,1.96530600175719,2.9990359395505));
#42158=CARTESIAN_POINT('Ctrl Pts',(-67.4249992701018,-0.132890558667537,
3.11017383011854));
#42159=CARTESIAN_POINT('Ctrl Pts',(-66.2035357618251,-2.1094508836634,3.22131172068658));
#42160=CARTESIAN_POINT('Ctrl Pts',(-63.8804623217255,-2.15520689204011,
3.33244961125462));
#42161=CARTESIAN_POINT('Ctrl Pts',(-62.5821144149725,-0.228277590427775,
3.44358750182266));
#42162=CARTESIAN_POINT('Ctrl Pts',(-63.4968846048806,1.90759677855457,3.55472539239071));
#42163=CARTESIAN_POINT('Ctrl Pts',(-65.7874733624335,2.29742618249228,3.66586328295874));
#42164=CARTESIAN_POINT('Ctrl Pts',(-67.3572788207879,0.584395347038986,
3.77700117352679));
#42165=CARTESIAN_POINT('Ctrl Pts',(-66.7694402411304,-1.66353917711054,
3.88813906409483));
#42166=CARTESIAN_POINT('Ctrl Pts',(-64.5620129419189,-2.3888174265201,3.99927695466288));
#42167=CARTESIAN_POINT('Ctrl Pts',(-62.7554801641395,-0.927583994626942,
4.11041484523091));
#42168=CARTESIAN_POINT('Ctrl Pts',(-63.0033818465923,1.3826775875065,4.22155273579896));
#42169=CARTESIAN_POINT('Ctrl Pts',(-65.0788107682801,2.42735869229697,4.33269062636699));
#42170=CARTESIAN_POINT('Ctrl Pts',(-67.0821032995307,1.25025085961923,4.44382851693504));
#42171=CARTESIAN_POINT('Ctrl Pts',(-67.1796230689615,-1.07122576705027,
4.55496640750307));
#42172=CARTESIAN_POINT('Ctrl Pts',(-65.2821091229946,-2.41219729396228,
4.66610429807113));
#42173=CARTESIAN_POINT('Ctrl Pts',(-63.1263775009061,-1.5452572946423,4.77724218863916));
#42174=CARTESIAN_POINT('Ctrl Pts',(-62.6855937936814,0.736074256717683,
4.88838007920721));
#42175=CARTESIAN_POINT('Ctrl Pts',(-64.3632123478174,2.34366864230481,4.99951796977525));
#42176=CARTESIAN_POINT('Ctrl Pts',(-66.6236898349158,1.80607664102167,5.11065586034329));
#42177=CARTESIAN_POINT('Ctrl Pts',(-67.3979856549427,-0.384637990101019,
5.22179375091133));
#42178=CARTESIAN_POINT('Ctrl Pts',(-65.9773779060574,-2.22328871643558,
5.33293164147938));
#42179=CARTESIAN_POINT('Ctrl Pts',(-63.6621652804381,-2.0269388363574,5.44406953204741));
#42180=CARTESIAN_POINT('Ctrl Pts',(-62.5714875417724,0.0246926647779575,
5.55520742261546));
#42181=CARTESIAN_POINT('Ctrl Pts',(-63.7036555936518,2.05371969901984,5.66634531318349));
#42182=CARTESIAN_POINT('Ctrl Pts',(-66.0223808123334,2.20295969802022,5.77748320375154));
#42183=CARTESIAN_POINT('Ctrl Pts',(-67.4053123737463,0.335794078720048,
5.88862109431958));
#42184=CARTESIAN_POINT('Ctrl Pts',(-66.5866281401934,-1.83870475455836,
5.99975898488763));
#42185=CARTESIAN_POINT('Ctrl Pts',(-64.3156972041947,-2.33026144716284,
6.11089687545566));
#42186=CARTESIAN_POINT('Ctrl Pts',(-62.6710926659578,-0.688814355154873,
6.22203476602371));
#42187=CARTESIAN_POINT('Ctrl Pts',(-63.1582101680956,1.58293676398102,6.33317265659174));
#42188=CARTESIAN_POINT('Ctrl Pts',(-65.3310466291073,2.40615402668531,6.4443105471598));
#42189=CARTESIAN_POINT('Ctrl Pts',(-67.2010541211369,1.02630878549798,6.55544843772783));
#42190=CARTESIAN_POINT('Ctrl Pts',(-67.0560525859507,-1.29158197049712,
6.66658632829588));
#42191=CARTESIAN_POINT('Ctrl Pts',(-65.029841359516,-2.42994159679626,6.77772421886392));
#42192=CARTESIAN_POINT('Ctrl Pts',(-62.9747815436376,-1.33872801408515,
6.88886210943195));
#42193=CARTESIAN_POINT('Ctrl Pts',(-62.8436282049399,0.19721374355959,6.96295403647732));
#42194=CARTESIAN_POINT('Ctrl Pts',(-63.1173724903363,0.823232180103149,
7.));
#42195=CARTESIAN_POINT('Ctrl Pts',(-63.7309291201476,-1.0793586530485,-2.));
#42196=CARTESIAN_POINT('Ctrl Pts',(-63.6855968419863,-1.03706844878282,
-2.));
#42197=CARTESIAN_POINT('Ctrl Pts',(-63.6429944057487,-0.992209355217755,
-2.));
#42198=CARTESIAN_POINT('Ctrl Pts',(-63.6031204505543,-0.945126337779186,
-2.));
#42199=CARTESIAN_POINT('Ctrl Pts',(-63.5606157477688,-0.89493694340586,
-2.));
#42200=CARTESIAN_POINT('Ctrl Pts',(-63.5212107097549,-0.84222025720975,
-2.));
#42201=CARTESIAN_POINT('Ctrl Pts',(-63.4849325153247,-0.787339414503396,
-2.));
#42202=CARTESIAN_POINT('Ctrl Pts',(-63.4531890951982,-0.739318677135336,
-2.));
#42203=CARTESIAN_POINT('Ctrl Pts',(-63.423839907855,-0.689639781933985,
-2.));
#42204=CARTESIAN_POINT('Ctrl Pts',(-63.396926053755,-0.638518448146663,
-2.));
#42205=CARTESIAN_POINT('Ctrl Pts',(-63.383420898641,-0.61286617479071,-2.));
#42206=CARTESIAN_POINT('Ctrl Pts',(-63.3705293094229,-0.586850346515661,
-2.));
#42207=CARTESIAN_POINT('Ctrl Pts',(-63.3582588228031,-0.560496376493833,
-2.));
#42208=CARTESIAN_POINT('Ctrl Pts',(-63.352655640319,-0.548462126525787,
-2.));
#42209=CARTESIAN_POINT('Ctrl Pts',(-63.3471814025998,-0.536355708766487,
-2.));
#42210=CARTESIAN_POINT('Ctrl Pts',(-63.3418453144502,-0.524199442886152,
-2.));
#42211=CARTESIAN_POINT('Ctrl Pts',(-63.3149230085341,-0.462867114849718,
-2.));
#42212=CARTESIAN_POINT('Ctrl Pts',(-63.2914620509818,-0.400159371493074,
-2.));
#42213=CARTESIAN_POINT('Ctrl Pts',(-63.2714860817235,-0.33643388798648,
-2.));
#42214=CARTESIAN_POINT('Ctrl Pts',(-63.2511562856272,-0.271579658934033,
-2.));
#42215=CARTESIAN_POINT('Ctrl Pts',(-63.234435470142,-0.205670475316589,
-2.));
#42216=CARTESIAN_POINT('Ctrl Pts',(-63.2213878692165,-0.139046848337481,
-2.));
#42217=CARTESIAN_POINT('Ctrl Pts',(-63.2104743799197,-0.0833204167814306,
-2.));
#42218=CARTESIAN_POINT('Ctrl Pts',(-63.2021313216452,-0.0270932010480611,
-2.));
#42219=CARTESIAN_POINT('Ctrl Pts',(-63.196421114974,0.0294478216546492,
-2.));
#42220=CARTESIAN_POINT('Ctrl Pts',(-63.1937898541988,0.0555019005692096,
-2.));
#42221=CARTESIAN_POINT('Ctrl Pts',(-63.1917179786548,0.0816227252779034,
-2.));
#42222=CARTESIAN_POINT('Ctrl Pts',(-63.190213400761,0.10779240289025,-2.));
#42223=CARTESIAN_POINT('Ctrl Pts',(-63.1895569069957,0.119211040809892,
-2.));
#42224=CARTESIAN_POINT('Ctrl Pts',(-63.1890085369661,0.13063873197943,-2.));
#42225=CARTESIAN_POINT('Ctrl Pts',(-63.1885692788766,0.142059931628667,
-2.));
#42226=CARTESIAN_POINT('Ctrl Pts',(-63.185872337845,0.212183402760181,-2.));
#42227=CARTESIAN_POINT('Ctrl Pts',(-63.1872764272328,0.282193469675666,
-2.));
#42228=CARTESIAN_POINT('Ctrl Pts',(-63.1928363192171,0.351729486410014,
-2.));
#42229=CARTESIAN_POINT('Ctrl Pts',(-63.1978071231096,0.413897942851084,
-2.));
#42230=CARTESIAN_POINT('Ctrl Pts',(-63.2061000911937,0.475688445045345,
-2.));
#42231=CARTESIAN_POINT('Ctrl Pts',(-63.2177875010733,0.536855401025581,
-2.));
#42232=CARTESIAN_POINT('Ctrl Pts',(-63.2305203455448,0.603493719122557,
-2.));
#42233=CARTESIAN_POINT('Ctrl Pts',(-63.2472809681188,0.669392782961828,
-2.));
#42234=CARTESIAN_POINT('Ctrl Pts',(-63.2678240437403,0.734338936172986,
-2.));
#42235=CARTESIAN_POINT('Ctrl Pts',(-63.2757504472631,0.759397959811583,
-2.));
#42236=CARTESIAN_POINT('Ctrl Pts',(-63.2842405167728,0.784315071866599,
-2.));
#42237=CARTESIAN_POINT('Ctrl Pts',(-63.2932821667435,0.809077679605451,
-2.));
#42238=CARTESIAN_POINT('Ctrl Pts',(-63.2972485928261,0.81994063642485,-2.));
#42239=CARTESIAN_POINT('Ctrl Pts',(-63.3013210590997,0.830773275850983,
-2.));
#42240=CARTESIAN_POINT('Ctrl Pts',(-63.3054934693646,0.841562024914705,
-2.));
#42241=CARTESIAN_POINT('Ctrl Pts',(-63.3307175500364,0.906784824076589,
-2.));
#42242=CARTESIAN_POINT('Ctrl Pts',(-63.3596326694542,0.970522726119043,
-2.));
#42243=CARTESIAN_POINT('Ctrl Pts',(-63.3919260622227,1.03255684529061,-2.));
#42244=CARTESIAN_POINT('Ctrl Pts',(-63.4249680867552,1.09602905157818,-2.));
#42245=CARTESIAN_POINT('Ctrl Pts',(-63.4615471340117,1.157718383915,-2.));
#42246=CARTESIAN_POINT('Ctrl Pts',(-63.5013843211633,1.2173866717758,-2.));
#42247=CARTESIAN_POINT('Ctrl Pts',(-63.5318674685087,1.26304444384141,-2.));
#42248=CARTESIAN_POINT('Ctrl Pts',(-63.5642595400752,1.30751888441973,-2.));
#42249=CARTESIAN_POINT('Ctrl Pts',(-63.598455110112,1.35069719141984,-2.));
#42250=CARTESIAN_POINT('Ctrl Pts',(-63.6197386626115,1.37757165974682,-2.));
#42251=CARTESIAN_POINT('Ctrl Pts',(-63.6417211957385,1.40394389610583,-2.));
#42252=CARTESIAN_POINT('Ctrl Pts',(-63.6643801907862,1.42978501722721,-2.));
#42253=CARTESIAN_POINT('Ctrl Pts',(-63.6770896559072,1.44427934174985,-2.));
#42254=CARTESIAN_POINT('Ctrl Pts',(-63.6900164428917,1.45861113921278,-2.));
#42255=CARTESIAN_POINT('Ctrl Pts',(-63.7031327805923,1.47274978412593,-2.));
#42256=CARTESIAN_POINT('Ctrl Pts',(-63.7540080482568,1.52759034715398,-2.));
#42257=CARTESIAN_POINT('Ctrl Pts',(-63.8077798406737,1.57958602565017,-2.));
#42258=CARTESIAN_POINT('Ctrl Pts',(-63.8641630605125,1.62847278876025,-2.));
#42259=CARTESIAN_POINT('Ctrl Pts',(-63.9063355382102,1.66503820543689,-2.));
#42260=CARTESIAN_POINT('Ctrl Pts',(-63.9499701263561,1.69986415252965,-2.));
#42261=CARTESIAN_POINT('Ctrl Pts',(-63.9949639294371,1.73283039559633,-2.));
#42262=CARTESIAN_POINT('Ctrl Pts',(-64.0089991299055,1.74311376349253,-2.));
#42263=CARTESIAN_POINT('Ctrl Pts',(-64.0231666800404,1.75321609759807,-2.));
#42264=CARTESIAN_POINT('Ctrl Pts',(-64.0374636964878,1.76313352311854,-2.));
#42265=CARTESIAN_POINT('Ctrl Pts',(-64.051264901766,1.77270701881548,-2.));
#42266=CARTESIAN_POINT('Ctrl Pts',(-64.0651797317384,1.78210327688949,-2.));
#42267=CARTESIAN_POINT('Ctrl Pts',(-64.0792001599332,1.79131603215157,-2.));
#42268=CARTESIAN_POINT('Ctrl Pts',(-64.1421565047628,1.83268434052647,-2.));
#42269=CARTESIAN_POINT('Ctrl Pts',(-64.207269965244,1.87037681374959,-2.));
#42270=CARTESIAN_POINT('Ctrl Pts',(-64.2742791023089,1.90411417795052,-2.));
#42271=CARTESIAN_POINT('Ctrl Pts',(-64.3255634212839,1.92993450369772,-2.));
#42272=CARTESIAN_POINT('Ctrl Pts',(-64.3779590786546,1.95343777834416,-2.));
#42273=CARTESIAN_POINT('Ctrl Pts',(-64.4313627927198,1.97448349564832,-2.));
#42274=CARTESIAN_POINT('Ctrl Pts',(-64.4437562344803,1.97936759175068,-2.));
#42275=CARTESIAN_POINT('Ctrl Pts',(-64.4562040109557,1.98411926473273,-2.));
#42276=CARTESIAN_POINT('Ctrl Pts',(-64.4687042096542,1.98873909628093,-2.));
#42277=CARTESIAN_POINT('Ctrl Pts',(-66.6673159824367,0.00130059074132209,
-0.871480363390211));
#42278=CARTESIAN_POINT('Ctrl Pts',(-66.6680474999804,0.0865457667101201,
-0.877193940366669));
#42279=CARTESIAN_POINT('Ctrl Pts',(-66.6620744628598,0.171688078253671,
-0.882907517343126));
#42280=CARTESIAN_POINT('Ctrl Pts',(-66.6490403647761,0.255735261203265,
-0.888621094319584));
#42281=CARTESIAN_POINT('Ctrl Pts',(-66.5645292565598,0.800684403669395,
-0.925667057842264));
#42282=CARTESIAN_POINT('Ctrl Pts',(-66.1831691519411,1.29959403086365,-0.962713021364943));
#42283=CARTESIAN_POINT('Ctrl Pts',(-65.6794913573425,1.52414483947234,-0.999758984887624));
#42284=CARTESIAN_POINT('Ctrl Pts',(-65.1758135627439,1.74869564808103,-1.0368049484103));
#42285=CARTESIAN_POINT('Ctrl Pts',(-64.5498180781654,1.69888763810415,-1.07385091193299));
#42286=CARTESIAN_POINT('Ctrl Pts',(-64.0879958937795,1.39749696674795,-1.11089687545567));
#42287=CARTESIAN_POINT('Ctrl Pts',(-63.6261737093935,1.09610629539175,-1.14794283897835));
#42288=CARTESIAN_POINT('Ctrl Pts',(-63.3285248252001,0.543132962656229,
-1.18498880250103));
#42289=CARTESIAN_POINT('Ctrl Pts',(-63.3312687442061,-0.00831466463025846,
-1.22203476602371));
#42290=CARTESIAN_POINT('Ctrl Pts',(-63.3340126632121,-0.559762291916746,
-1.25908072954639));
#42291=CARTESIAN_POINT('Ctrl Pts',(-63.6371493854174,-1.1096842137542,-1.29612669306907));
#42292=CARTESIAN_POINT('Ctrl Pts',(-64.1019490294701,-1.40647845913029,
-1.33317265659175));
#42293=CARTESIAN_POINT('Ctrl Pts',(-64.5667486735228,-1.70327270450637,
-1.37021862011443));
#42294=CARTESIAN_POINT('Ctrl Pts',(-65.193211239423,-1.74693927342109,-1.40726458363711));
#42295=CARTESIAN_POINT('Ctrl Pts',(-65.6946279386367,-1.51735015093768,
-1.44431054715979));
#42296=CARTESIAN_POINT('Ctrl Pts',(-66.1960446378505,-1.28776102845428,
-1.48135651068247));
#42297=CARTESIAN_POINT('Ctrl Pts',(-66.5724154703778,-0.784916214572752,
-1.51840247420515));
#42298=CARTESIAN_POINT('Ctrl Pts',(-66.6515012684707,-0.23922910918681,
-1.55544843772783));
#42299=CARTESIAN_POINT('Ctrl Pts',(-66.6629095976148,-0.160512345140353,
-1.56079241294863));
#42300=CARTESIAN_POINT('Ctrl Pts',(-66.6681317812815,-0.0809040843243736,
-1.56613638816942));
#42301=CARTESIAN_POINT('Ctrl Pts',(-66.6674675207825,-0.00121113675535883,
-1.57148036339021));
#42302=CARTESIAN_POINT('Ctrl Pts',(-65.5301702171886,1.98517432567173,-2.));
#42303=CARTESIAN_POINT('Ctrl Pts',(-66.1902879097456,1.80888011517989,-1.96295403647732));
#42304=CARTESIAN_POINT('Ctrl Pts',(-67.3093622463653,0.748693059830641,
-1.88886210943196));
#42305=CARTESIAN_POINT('Ctrl Pts',(-66.8811995093437,-1.538373214553,-1.77772421886392));
#42306=CARTESIAN_POINT('Ctrl Pts',(-64.7278715623352,-2.41277602144419,
-1.66658632829587));
#42307=CARTESIAN_POINT('Ctrl Pts',(-62.8252644286755,-1.08095990301172,
-1.55544843772783));
#42308=CARTESIAN_POINT('Ctrl Pts',(-62.9123886677794,1.24138962897178,-1.44431054715979));
#42309=CARTESIAN_POINT('Ctrl Pts',(-64.9107473342681,2.42691462884513,-1.33317265659175));
#42310=CARTESIAN_POINT('Ctrl Pts',(-66.9905869477348,1.39134438721223,-1.22203476602371));
#42311=CARTESIAN_POINT('Ctrl Pts',(-67.24852778644,-0.917884815202466,-1.11089687545567));
#42312=CARTESIAN_POINT('Ctrl Pts',(-65.4483108550045,-2.38688976599862,
-0.999758984887625));
#42313=CARTESIAN_POINT('Ctrl Pts',(-63.2377776981899,-1.67118490708905,
-0.888621094319582));
#42314=CARTESIAN_POINT('Ctrl Pts',(-62.6402125087857,0.574193448178942,
-0.777483203751542));
#42315=CARTESIAN_POINT('Ctrl Pts',(-64.2025947176117,2.29399639382146,-0.666345313183498));
#42316=CARTESIAN_POINT('Ctrl Pts',(-66.4948474007694,1.91408331059476,-0.555207422615458));
#42317=CARTESIAN_POINT('Ctrl Pts',(-67.4188511430454,-0.217814411897149,
-0.444069532047416));
#42318=CARTESIAN_POINT('Ctrl Pts',(-66.1288520704621,-2.15034287637184,
-0.332931641479373));
#42319=CARTESIAN_POINT('Ctrl Pts',(-63.8056023683761,-2.11463875683277,
-0.221793750911332));
#42320=CARTESIAN_POINT('Ctrl Pts',(-62.5755981242121,-0.143381478345974,
-0.110655860343291));
#42321=CARTESIAN_POINT('Ctrl Pts',(-63.5646765331008,1.95911432942999,0.00048203022475183));
#42322=CARTESIAN_POINT('Ctrl Pts',(-65.8675227272721,2.26841065672896,0.111619920792793));
#42323=CARTESIAN_POINT('Ctrl Pts',(-67.3763155620569,0.501404942245523,
0.222757811360835));
#42324=CARTESIAN_POINT('Ctrl Pts',(-66.7100397977853,-1.7245423808174,0.333895701928876));
#42325=CARTESIAN_POINT('Ctrl Pts',(-64.4785452214709,-2.37199651591817,
0.445033592496919));
#42326=CARTESIAN_POINT('Ctrl Pts',(-62.7243441135659,-0.848335334231208,
0.55617148306496));
#42327=CARTESIAN_POINT('Ctrl Pts',(-63.0530766482751,1.45181679686654,0.667309373633002));
#42328=CARTESIAN_POINT('Ctrl Pts',(-65.1638502053818,2.42310455048397,0.778447264201043));
#42329=CARTESIAN_POINT('Ctrl Pts',(-67.1246498118468,1.17649722845177,0.889585154769086));
#42330=CARTESIAN_POINT('Ctrl Pts',(-67.1407333500909,-1.14697134880472,
1.00072304533713));
#42331=CARTESIAN_POINT('Ctrl Pts',(-65.1973793755662,-2.42060404314487,
1.11186093590517));
#42332=CARTESIAN_POINT('Ctrl Pts',(-63.0733618200821,-1.47863040518406,
1.22299882647321));
#42333=CARTESIAN_POINT('Ctrl Pts',(-62.7128180402749,0.816750411403611,
1.33413671704125));
#42334=CARTESIAN_POINT('Ctrl Pts',(-64.4457578465939,2.36455031387797,1.4452746076093));
#42335=CARTESIAN_POINT('Ctrl Pts',(-66.686001781468,1.74805049822323,1.55641249817733));
#42336=CARTESIAN_POINT('Ctrl Pts',(-67.3830291651992,-0.468459762690014,
1.66755038874538));
#42337=CARTESIAN_POINT('Ctrl Pts',(-65.898842928637,-2.25618349012117,1.77868827931342));
#42338=CARTESIAN_POINT('Ctrl Pts',(-63.5919355659201,-1.97879688218178,
1.88982616988146));
#42339=CARTESIAN_POINT('Ctrl Pts',(-62.5738455482538,0.109804953100741,
2.0009640604495));
#42340=CARTESIAN_POINT('Ctrl Pts',(-63.7764422147334,2.0979010695377,2.11210195101754));
#42341=CARTESIAN_POINT('Ctrl Pts',(-66.0989751981566,2.16576454521031,2.22323984158559));
#42342=CARTESIAN_POINT('Ctrl Pts',(-67.4156037194807,0.25127917121157,2.33437773215363));
#42343=CARTESIAN_POINT('Ctrl Pts',(-66.5212027615546,-1.89320487789678,
2.44551562272167));
#42344=CARTESIAN_POINT('Ctrl Pts',(-64.234427664365,-2.30481703186257,2.55665351328971));
#42345=CARTESIAN_POINT('Ctrl Pts',(-62.6483896081628,-0.606804018161647,
2.66779140385776));
#42346=CARTESIAN_POINT('Ctrl Pts',(-63.214807212685,1.64662359498827,2.77892929442579));
#42347=CARTESIAN_POINT('Ctrl Pts',(-65.4152320208998,2.39287795766376,2.89006718499384));
#42348=CARTESIAN_POINT('Ctrl Pts',(-67.2355902513335,0.948903988607916,
3.00120507556188));
#42349=CARTESIAN_POINT('Ctrl Pts',(-67.009687371404,-1.36361256252397,3.11234296612992));
#42350=CARTESIAN_POINT('Ctrl Pts',(-64.9442948490232,-2.42799907075925,
3.22348085669796));
#42351=CARTESIAN_POINT('Ctrl Pts',(-62.9298898830714,-1.27001049414664,
3.334618747266));
#42352=CARTESIAN_POINT('Ctrl Pts',(-62.8102801837888,1.05043309065765,3.44575663783405));
#42353=CARTESIAN_POINT('Ctrl Pts',(-64.6949458653977,2.40940335486023,3.55689452840209));
#42354=CARTESIAN_POINT('Ctrl Pts',(-66.8588310559542,1.56301940386929,3.66803241897013));
#42355=CARTESIAN_POINT('Ctrl Pts',(-67.3213071004237,-0.71401393333385,
3.77917030953817));
#42356=CARTESIAN_POINT('Ctrl Pts',(-65.6590644304509,-2.3375022198779,3.89030820010621));
#42357=CARTESIAN_POINT('Ctrl Pts',(-63.39357261301,-1.82144821550898,4.00144609067426));
#42358=CARTESIAN_POINT('Ctrl Pts',(-62.5984620009619,0.361797997181342,
4.1125839812423));
#42359=CARTESIAN_POINT('Ctrl Pts',(-64.0015063548152,2.21388639990767,4.22372187181034));
#42360=CARTESIAN_POINT('Ctrl Pts',(-66.3184832656195,2.03957947376812,4.33485976237838));
#42361=CARTESIAN_POINT('Ctrl Pts',(-67.4286374911296,-0.00157767540964147,
4.44599765294642));
#42362=CARTESIAN_POINT('Ctrl Pts',(-66.315832277707,-2.04129075981347,4.55713554351446));
#42363=CARTESIAN_POINT('Ctrl Pts',(-63.9986308592856,-2.21258726309084,
4.66827343408251));
#42364=CARTESIAN_POINT('Ctrl Pts',(-62.5979939690176,-0.358677549762027,
4.77941132465054));
#42365=CARTESIAN_POINT('Ctrl Pts',(-63.3959404447163,1.82353378810158,4.89054921521859));
#42366=CARTESIAN_POINT('Ctrl Pts',(-65.6621008123707,2.33664397819608,5.00168710578663));
#42367=CARTESIAN_POINT('Ctrl Pts',(-67.3222328179755,0.710997418429197,
5.11282499635467));
#42368=CARTESIAN_POINT('Ctrl Pts',(-66.8567987494513,-1.56543310762404,
5.22396288692272));
#42369=CARTESIAN_POINT('Ctrl Pts',(-64.6918158067504,-2.40900502421389,
5.33510077749075));
#42370=CARTESIAN_POINT('Ctrl Pts',(-62.80891719594,-1.04758718972751,5.4462386680588));
#42371=CARTESIAN_POINT('Ctrl Pts',(-62.9315418303621,1.27269881881277,5.55737655862684));
#42372=CARTESIAN_POINT('Ctrl Pts',(-64.947449081762,2.42806968006159,5.66851444919488));
#42373=CARTESIAN_POINT('Ctrl Pts',(-67.0114579748176,1.36099981154568,5.77965233976293));
#42374=CARTESIAN_POINT('Ctrl Pts',(-67.234354225073,-0.951806616989204,
5.89079023033096));
#42375=CARTESIAN_POINT('Ctrl Pts',(-65.4121253417219,-2.39341760299656,
6.00192812089901));
#42376=CARTESIAN_POINT('Ctrl Pts',(-63.2126643336617,-1.64429852840487,
6.11306601146705));
#42377=CARTESIAN_POINT('Ctrl Pts',(-62.649189925264,0.60985028512182,6.22420390203509));
#42378=CARTESIAN_POINT('Ctrl Pts',(-64.2374031554986,2.30582648807955,6.33534179260313));
#42379=CARTESIAN_POINT('Ctrl Pts',(-66.5236998933487,1.89119386508315,6.44647968317117));
#42380=CARTESIAN_POINT('Ctrl Pts',(-67.4151988715152,-0.254352246057023,
6.55761757373922));
#42381=CARTESIAN_POINT('Ctrl Pts',(-66.0963109962835,-2.16731896239628,
6.66875546430726));
#42382=CARTESIAN_POINT('Ctrl Pts',(-63.7734206371606,-2.09605634078855,
6.77989335487529));
#42383=CARTESIAN_POINT('Ctrl Pts',(-62.5742917867301,-0.107152602938497,
6.89103124544335));
#42384=CARTESIAN_POINT('Ctrl Pts',(-63.5933356141608,1.98161526205799,7.00216913601138));
#42385=CARTESIAN_POINT('Ctrl Pts',(-65.9042541560964,2.25300237548896,7.11330702657943));
#42386=CARTESIAN_POINT('Ctrl Pts',(-66.8857543436368,1.06431345694512,7.18739895362479));
#42387=CARTESIAN_POINT('Ctrl Pts',(-67.0166758614465,0.393720754290193,
7.22444491714747));
#42388=CARTESIAN_POINT('Ctrl Pts',(-65.4967348970877,1.85997880000277,-2.07481497238249));
#42389=CARTESIAN_POINT('Ctrl Pts',(-66.1152220988337,1.69480262890399,-2.03776900885981));
#42390=CARTESIAN_POINT('Ctrl Pts',(-67.1637217267118,0.701476540869023,
-1.96367708181445));
#42391=CARTESIAN_POINT('Ctrl Pts',(-66.7625611820115,-1.44135531502629,
-1.8525391912464));
#42392=CARTESIAN_POINT('Ctrl Pts',(-64.7450334117317,-2.26061368566345,
-1.74140130067836));
#42393=CARTESIAN_POINT('Ctrl Pts',(-62.962414682697,-1.01278889075624,-1.63026341011032));
#42394=CARTESIAN_POINT('Ctrl Pts',(-63.0440444094189,1.16310107509049,-1.51912551954228));
#42395=CARTESIAN_POINT('Ctrl Pts',(-64.9163760764189,2.27386063817903,-1.40798762897424));
#42396=CARTESIAN_POINT('Ctrl Pts',(-66.8650500736736,1.30359889821864,-1.2968497384062));
#42397=CARTESIAN_POINT('Ctrl Pts',(-67.1067238075329,-0.859998174993202,
-1.18571184783815));
#42398=CARTESIAN_POINT('Ctrl Pts',(-65.4200380164786,-2.23635995352639,
-1.07457395727011));
#42399=CARTESIAN_POINT('Ctrl Pts',(-63.3489126975537,-1.56579120426537,
-0.963436066702071));
#42400=CARTESIAN_POINT('Ctrl Pts',(-62.7890331093795,0.537981791776368,
-0.85229817613403));
#42401=CARTESIAN_POINT('Ctrl Pts',(-64.2528832853252,2.14932492558151,-0.741160285565987));
#42402=CARTESIAN_POINT('Ctrl Pts',(-66.4005744678012,1.79337115794137,-0.630022394997947));
#42403=CARTESIAN_POINT('Ctrl Pts',(-67.2663056781698,-0.204077890402237,
-0.518884504429904));
#42404=CARTESIAN_POINT('Ctrl Pts',(-66.0576607264394,-2.01473095388499,
-0.407746613861862));
#42405=CARTESIAN_POINT('Ctrl Pts',(-63.8809273599474,-1.98127852376001,
-0.296608723293821));
#42406=CARTESIAN_POINT('Ctrl Pts',(-62.7284936474651,-0.134339088808397,
-0.185470832725779));
#42407=CARTESIAN_POINT('Ctrl Pts',(-63.6551955739828,1.8355622840772,-0.0743329421577371));
#42408=CARTESIAN_POINT('Ctrl Pts',(-65.8128121849957,2.12535275953086,0.0368049484103043));
#42409=CARTESIAN_POINT('Ctrl Pts',(-67.2264526144558,0.469783711552746,
0.147942838978346));
#42410=CARTESIAN_POINT('Ctrl Pts',(-66.6021957013601,-1.61578367529074,
0.259080729546388));
#42411=CARTESIAN_POINT('Ctrl Pts',(-64.5114309002076,-2.22240595006454,
0.37021862011443));
#42412=CARTESIAN_POINT('Ctrl Pts',(-62.8678589330251,-0.794834849795569,
0.481356510682471));
#42413=CARTESIAN_POINT('Ctrl Pts',(-63.1758598665065,1.36025759991932,0.592494401250513));
#42414=CARTESIAN_POINT('Ctrl Pts',(-65.153516950348,2.27029084338244,0.703632291818555));
#42415=CARTESIAN_POINT('Ctrl Pts',(-66.9906582290337,1.10230113037648,0.814770182386596));
#42416=CARTESIAN_POINT('Ctrl Pts',(-67.0057274548323,-1.07463730786741,
0.925908072954638));
#42417=CARTESIAN_POINT('Ctrl Pts',(-65.1849315948547,-2.26794803117706,
1.03704596352268));
#42418=CARTESIAN_POINT('Ctrl Pts',(-63.1948657487746,-1.38538020118271,
1.14818385409072));
#42419=CARTESIAN_POINT('Ctrl Pts',(-62.8570597544889,0.765241838189812,
1.25932174465876));
#42420=CARTESIAN_POINT('Ctrl Pts',(-64.480711269498,2.21542934465705,1.37045963522681));
#42421=CARTESIAN_POINT('Ctrl Pts',(-66.5796736486789,1.63780924727067,1.48159752579485));
#42422=CARTESIAN_POINT('Ctrl Pts',(-67.232742822502,-0.438916228156898,
1.59273541636289));
#42423=CARTESIAN_POINT('Ctrl Pts',(-65.8421571698655,-2.11389670230682,
1.70387330693093));
#42424=CARTESIAN_POINT('Ctrl Pts',(-63.680735508938,-1.85400355161469,1.81501119749897));
#42425=CARTESIAN_POINT('Ctrl Pts',(-62.7268515981571,0.102880075699936,
1.92614908806701));
#42426=CARTESIAN_POINT('Ctrl Pts',(-63.8536061988389,1.96559640298739,2.03728697863505));
#42427=CARTESIAN_POINT('Ctrl Pts',(-66.0296680467136,2.02918005124097,2.1484248692031));
#42428=CARTESIAN_POINT('Ctrl Pts',(-67.2632630542012,0.235432186126848,
2.25956275977114));
#42429=CARTESIAN_POINT('Ctrl Pts',(-66.42526772103,-1.7738094289318,2.37070065033918));
#42430=CARTESIAN_POINT('Ctrl Pts',(-64.2827086791644,-2.15946315732203,
2.48183854090722));
#42431=CARTESIAN_POINT('Ctrl Pts',(-62.7966945178967,-0.568535767837546,
2.59297643147526));
#42432=CARTESIAN_POINT('Ctrl Pts',(-63.3273908515816,1.5427788575828,2.7041143220433));
#42433=CARTESIAN_POINT('Ctrl Pts',(-65.3890453074919,2.24197049835536,2.81525221261135));
#42434=CARTESIAN_POINT('Ctrl Pts',(-67.0946021813807,0.889061116308559,
2.92639010317939));
#42435=CARTESIAN_POINT('Ctrl Pts',(-66.8829459242478,-1.27761598813436,
3.03752799374744));
#42436=CARTESIAN_POINT('Ctrl Pts',(-64.9478079085913,-2.27487668948696,
3.14866588431547));
#42437=CARTESIAN_POINT('Ctrl Pts',(-63.0604419061002,-1.18991695809611,
3.25980377488352));
#42438=CARTESIAN_POINT('Ctrl Pts',(-62.9483754230397,0.984187259616866,
3.37094166545155));
#42439=CARTESIAN_POINT('Ctrl Pts',(-64.7141841822776,2.25745371715866,3.4820795560196));
#42440=CARTESIAN_POINT('Ctrl Pts',(-66.7416034008459,1.46444718612111,3.59321744658764));
#42441=CARTESIAN_POINT('Ctrl Pts',(-67.1749132754993,-0.668984462338426,
3.70435533715568));
#42442=CARTESIAN_POINT('Ctrl Pts',(-65.6175003638835,-2.19008704561055,
3.81549322772372));
#42443=CARTESIAN_POINT('Ctrl Pts',(-63.4948823662959,-1.70657811877716,
3.92663111829177));
#42444=CARTESIAN_POINT('Ctrl Pts',(-62.7499156079905,0.338981114121075,
4.0377690088598));
#42445=CARTESIAN_POINT('Ctrl Pts',(-64.0644766114669,2.0742670888862,4.14890689942785));
#42446=CARTESIAN_POINT('Ctrl Pts',(-66.2353327818609,1.91095287354468,4.26004478999589));
#42447=CARTESIAN_POINT('Ctrl Pts',(-67.2754748477136,-0.00147817890714668,
4.37118268056393));
#42448=CARTESIAN_POINT('Ctrl Pts',(-66.2328489791779,-1.91255623689868,
4.48232057113198));
#42449=CARTESIAN_POINT('Ctrl Pts',(-64.061782459797,-2.0730498824644,4.59345846170001));
#42450=CARTESIAN_POINT('Ctrl Pts',(-62.7494770926002,-0.336057458514918,
4.70459635226806));
#42451=CARTESIAN_POINT('Ctrl Pts',(-63.4971008700911,1.70853216420176,4.8157342428361));
#42452=CARTESIAN_POINT('Ctrl Pts',(-65.6203452556023,2.1892829291595,4.92687213340414));
#42453=CARTESIAN_POINT('Ctrl Pts',(-67.1757806124374,0.666158184716363,
5.03801002397219));
#42454=CARTESIAN_POINT('Ctrl Pts',(-66.7396992622713,-1.46670866903235,
5.14914791454022));
#42455=CARTESIAN_POINT('Ctrl Pts',(-64.7112515215779,-2.25708050733623,
5.26028580510827));
#42456=CARTESIAN_POINT('Ctrl Pts',(-62.9470983923676,-0.98152083615545,
5.3714236956763));
#42457=CARTESIAN_POINT('Ctrl Pts',(-63.0619896729133,1.19243574288083,5.48256158624435));
#42458=CARTESIAN_POINT('Ctrl Pts',(-64.9507632188372,2.27494284579563,5.59369947681239));
#42459=CARTESIAN_POINT('Ctrl Pts',(-66.8846048641049,1.27516801096355,5.70483736738043));
#42460=CARTESIAN_POINT('Ctrl Pts',(-67.093444105432,-0.89178068968993,5.81597525794848));
#42461=CARTESIAN_POINT('Ctrl Pts',(-65.3861345518295,-2.24247611081747,
5.92711314851652));
#42462=CARTESIAN_POINT('Ctrl Pts',(-63.3253831137711,-1.54060042191707,
6.03825103908456));
#42463=CARTESIAN_POINT('Ctrl Pts',(-62.7974443627954,0.571389921194157,
6.1493889296526));
#42464=CARTESIAN_POINT('Ctrl Pts',(-64.2854965201901,2.16040895192496,6.26052682022064));
#42465=CARTESIAN_POINT('Ctrl Pts',(-66.4276073705699,1.77192524115468,6.37166471078869));
#42466=CARTESIAN_POINT('Ctrl Pts',(-67.2628837380762,-0.238311456722607,
6.48280260135673));
#42467=CARTESIAN_POINT('Ctrl Pts',(-66.0271718634116,-2.03063643871026,
6.59394049192477));
#42468=CARTESIAN_POINT('Ctrl Pts',(-63.8507751778273,-1.96386801252777,
6.70507838249281));
#42469=CARTESIAN_POINT('Ctrl Pts',(-62.7272696944899,-0.100394996677825,
6.81621627306085));
#42470=CARTESIAN_POINT('Ctrl Pts',(-63.6820472627791,1.85664418964447,6.92735416362889));
#42471=CARTESIAN_POINT('Ctrl Pts',(-65.8472271368835,2.11091620548104,7.03849205419694));
#42472=CARTESIAN_POINT('Ctrl Pts',(-66.7668287645171,0.997192257060716,
7.1125839812423));
#42473=CARTESIAN_POINT('Ctrl Pts',(-66.8894936833815,0.36889065440289,7.14962994476498));
#42474=CARTESIAN_POINT('Ctrl Pts',(-65.4632995769868,1.73478327433381,-2.14962994476498));
#42475=CARTESIAN_POINT('Ctrl Pts',(-66.0401562879218,1.5807251426281,-2.1125839812423));
#42476=CARTESIAN_POINT('Ctrl Pts',(-67.0180812070583,0.654260021907404,
-2.03849205419694));
#42477=CARTESIAN_POINT('Ctrl Pts',(-66.6439228546792,-1.34433741549959,
-1.92735416362889));
#42478=CARTESIAN_POINT('Ctrl Pts',(-64.7621952611282,-2.1084513498827,-1.81621627306085));
#42479=CARTESIAN_POINT('Ctrl Pts',(-63.0995649367186,-0.944617878500769,
-1.70507838249281));
#42480=CARTESIAN_POINT('Ctrl Pts',(-63.1757001510583,1.08481252120919,-1.59394049192477));
#42481=CARTESIAN_POINT('Ctrl Pts',(-64.9220048185698,2.12080664751292,-1.48280260135673));
#42482=CARTESIAN_POINT('Ctrl Pts',(-66.7395131996123,1.21585340922505,-1.37166471078869));
#42483=CARTESIAN_POINT('Ctrl Pts',(-66.9649198286257,-0.802111534783937,
-1.26052682022064));
#42484=CARTESIAN_POINT('Ctrl Pts',(-65.3917651779528,-2.08583014105415,
-1.1493889296526));
#42485=CARTESIAN_POINT('Ctrl Pts',(-63.4600476969176,-1.46039750144169,
-1.03825103908456));
#42486=CARTESIAN_POINT('Ctrl Pts',(-62.9378537099731,0.501770135373796,
-0.927113148516519));
#42487=CARTESIAN_POINT('Ctrl Pts',(-64.3031718530388,2.00465345734157,-0.815975257948477));
#42488=CARTESIAN_POINT('Ctrl Pts',(-66.306301534833,1.67265900528797,-0.704837367380435));
#42489=CARTESIAN_POINT('Ctrl Pts',(-67.1137602132943,-0.190341368907323,
-0.593699476812392));
#42490=CARTESIAN_POINT('Ctrl Pts',(-65.9864693824166,-1.87911903139814,
-0.482561586244352));
#42491=CARTESIAN_POINT('Ctrl Pts',(-63.9562523515188,-1.84791829068725,
-0.371423695676309));
#42492=CARTESIAN_POINT('Ctrl Pts',(-62.8813891707182,-0.125296699270823,
-0.260285805108269));
#42493=CARTESIAN_POINT('Ctrl Pts',(-63.7457146148648,1.71201023872442,-0.149147914540226));
#42494=CARTESIAN_POINT('Ctrl Pts',(-65.7581016427195,1.98229486233276,-0.0380100239721847));
#42495=CARTESIAN_POINT('Ctrl Pts',(-67.0765896668548,0.438162480859971,
0.0731278665958568));
#42496=CARTESIAN_POINT('Ctrl Pts',(-66.4943516049349,-1.50702496976407,
0.184265757163899));
#42497=CARTESIAN_POINT('Ctrl Pts',(-64.5443165789444,-2.07281538421092,
0.295403647731941));
#42498=CARTESIAN_POINT('Ctrl Pts',(-63.0113737524843,-0.741334365359929,
0.406541538299983));
#42499=CARTESIAN_POINT('Ctrl Pts',(-63.298643084738,1.26869840297211,0.517679428868024));
#42500=CARTESIAN_POINT('Ctrl Pts',(-65.1431836953141,2.1174771362809,0.628817319436066));
#42501=CARTESIAN_POINT('Ctrl Pts',(-66.8566666462206,1.02810503230119,0.739955210004107));
#42502=CARTESIAN_POINT('Ctrl Pts',(-66.8707215595737,-1.0023032669301,0.851093100572149));
#42503=CARTESIAN_POINT('Ctrl Pts',(-65.1724838141431,-2.11529201920925,
0.96223099114019));
#42504=CARTESIAN_POINT('Ctrl Pts',(-63.3163696774672,-1.29212999718137,
1.07336888170823));
#42505=CARTESIAN_POINT('Ctrl Pts',(-63.0013014687027,0.713733264976017,
1.18450677227627));
#42506=CARTESIAN_POINT('Ctrl Pts',(-64.5156646924022,2.06630837543613,1.29564466284432));
#42507=CARTESIAN_POINT('Ctrl Pts',(-66.4733455158896,1.52756799631812,1.40678255341236));
#42508=CARTESIAN_POINT('Ctrl Pts',(-67.0824564798048,-0.409372693623786,
1.5179204439804));
#42509=CARTESIAN_POINT('Ctrl Pts',(-65.7854714110939,-1.97160991449247,
1.62905833454844));
#42510=CARTESIAN_POINT('Ctrl Pts',(-63.7695354519561,-1.7292102210476,1.74019622511648));
#42511=CARTESIAN_POINT('Ctrl Pts',(-62.8798576480604,0.0959551982991319,
1.85133411568453));
#42512=CARTESIAN_POINT('Ctrl Pts',(-63.9307701829444,1.83329173643707,1.96247200625256));
#42513=CARTESIAN_POINT('Ctrl Pts',(-65.9603608952703,1.89259555727163,2.07360989682061));
#42514=CARTESIAN_POINT('Ctrl Pts',(-67.110922388922,0.219585201042126,2.18474778738865));
#42515=CARTESIAN_POINT('Ctrl Pts',(-66.3293326805052,-1.65441397996682,
2.29588567795669));
#42516=CARTESIAN_POINT('Ctrl Pts',(-64.330989693964,-2.01410928278148,2.40702356852474));
#42517=CARTESIAN_POINT('Ctrl Pts',(-62.9449994276305,-0.530267517513444,
2.51816145909277));
#42518=CARTESIAN_POINT('Ctrl Pts',(-63.4399744904782,1.43893412017733,2.62929934966082));
#42519=CARTESIAN_POINT('Ctrl Pts',(-65.362858594084,2.09106303904696,2.74043724022886));
#42520=CARTESIAN_POINT('Ctrl Pts',(-66.953614111428,0.829218244009199,2.8515751307969));
#42521=CARTESIAN_POINT('Ctrl Pts',(-66.7562044770915,-1.19161941374474,
2.96271302136494));
#42522=CARTESIAN_POINT('Ctrl Pts',(-64.9513209681592,-2.12175430821468,
3.07385091193298));
#42523=CARTESIAN_POINT('Ctrl Pts',(-63.1909939291292,-1.10982342204557,
3.18498880250103));
#42524=CARTESIAN_POINT('Ctrl Pts',(-63.0864706622905,0.917941428576082,
3.29612669306907));
#42525=CARTESIAN_POINT('Ctrl Pts',(-64.7334224991575,2.10550407945709,3.40726458363711));
#42526=CARTESIAN_POINT('Ctrl Pts',(-66.6243757457373,1.36587496837294,3.51840247420515));
#42527=CARTESIAN_POINT('Ctrl Pts',(-67.0285194505751,-0.623954991343003,
3.6295403647732));
#42528=CARTESIAN_POINT('Ctrl Pts',(-65.5759362973161,-2.04267187134319,
3.74067825534123));
#42529=CARTESIAN_POINT('Ctrl Pts',(-63.5961921195818,-1.59170802204534,
3.85181614590928));
#42530=CARTESIAN_POINT('Ctrl Pts',(-62.9013692150191,0.316164231060809,
3.96295403647732));
#42531=CARTESIAN_POINT('Ctrl Pts',(-64.1274468681188,1.93464777786473,4.07409192704536));
#42532=CARTESIAN_POINT('Ctrl Pts',(-66.1521822981021,1.78232627332124,4.1852298176134));
#42533=CARTESIAN_POINT('Ctrl Pts',(-67.1223122042977,-0.00137868240465238,
4.29636770818144));
#42534=CARTESIAN_POINT('Ctrl Pts',(-66.1498656806486,-1.78382171398389,
4.40750559874949));
#42535=CARTESIAN_POINT('Ctrl Pts',(-64.1249340603086,-1.93351250183795,
4.51864348931752));
#42536=CARTESIAN_POINT('Ctrl Pts',(-62.9009602161829,-0.313437367267809,
4.62978137988557));
#42537=CARTESIAN_POINT('Ctrl Pts',(-63.5982612954659,1.59353054030193,4.74091927045361));
#42538=CARTESIAN_POINT('Ctrl Pts',(-65.578589698834,2.04192188012293,4.85205716102165));
#42539=CARTESIAN_POINT('Ctrl Pts',(-67.0293284068994,0.621318951003525,
4.96319505158969));
#42540=CARTESIAN_POINT('Ctrl Pts',(-66.6225997750913,-1.36798423044065,
5.07433294215773));
#42541=CARTESIAN_POINT('Ctrl Pts',(-64.7306872364055,-2.10515599045856,
5.18547083272578));
#42542=CARTESIAN_POINT('Ctrl Pts',(-63.0852795887951,-0.915454482583389,
5.29660872329381));
#42543=CARTESIAN_POINT('Ctrl Pts',(-63.1924375154646,1.11217266694889,5.40774661386187));
#42544=CARTESIAN_POINT('Ctrl Pts',(-64.9540773559123,2.12181601152967,5.5188845044299));
#42545=CARTESIAN_POINT('Ctrl Pts',(-66.7577517533922,1.18933621038143,5.63002239499795));
#42546=CARTESIAN_POINT('Ctrl Pts',(-66.9525339857911,-0.831754762390655,
5.74116028556598));
#42547=CARTESIAN_POINT('Ctrl Pts',(-65.360143761937,-2.09153461863839,5.85229817613403));
#42548=CARTESIAN_POINT('Ctrl Pts',(-63.4381018938804,-1.43690231542927,
5.96343606670207));
#42549=CARTESIAN_POINT('Ctrl Pts',(-62.945698800327,0.532929557266492,6.0745739572701));
#42550=CARTESIAN_POINT('Ctrl Pts',(-64.3335898848817,2.01499141577037,6.18571184783816));
#42551=CARTESIAN_POINT('Ctrl Pts',(-66.3315148477911,1.65265661722621,6.29684973840619));
#42552=CARTESIAN_POINT('Ctrl Pts',(-67.1105686046371,-0.222270667388193,
6.40798762897424));
#42553=CARTESIAN_POINT('Ctrl Pts',(-65.9580327305397,-1.89395391502424,
6.51912551954227));
#42554=CARTESIAN_POINT('Ctrl Pts',(-63.9281297184939,-1.83167968426698,
6.63026341011033));
#42555=CARTESIAN_POINT('Ctrl Pts',(-62.8802476022497,-0.0936373904171547,
6.74140130067836));
#42556=CARTESIAN_POINT('Ctrl Pts',(-63.7707589113974,1.73167311723095,6.85253919124641));
#42557=CARTESIAN_POINT('Ctrl Pts',(-65.7902001176707,1.96883003547312,6.96367708181445));
#42558=CARTESIAN_POINT('Ctrl Pts',(-66.6479031853974,0.930071057176316,
7.03776900885981));
#42559=CARTESIAN_POINT('Ctrl Pts',(-66.7623115053165,0.344060554515587,
7.07481497238249));
#42560=CARTESIAN_POINT('Ctrl Pts',(-65.4298642568859,1.60958774866485,-2.22444491714747));
#42561=CARTESIAN_POINT('Ctrl Pts',(-65.9650904770099,1.46664765635221,-2.18739895362479));
#42562=CARTESIAN_POINT('Ctrl Pts',(-66.8724406874047,0.607043502945785,
-2.11330702657942));
#42563=CARTESIAN_POINT('Ctrl Pts',(-66.5252845273472,-1.24731951597289,
-2.00216913601139));
#42564=CARTESIAN_POINT('Ctrl Pts',(-64.7793571105247,-1.95628901410196,
-1.89103124544334));
#42565=CARTESIAN_POINT('Ctrl Pts',(-63.2367151907402,-0.876446866245294,
-1.7798933548753));
#42566=CARTESIAN_POINT('Ctrl Pts',(-63.3073558926977,1.00652396732789,-1.66875546430726));
#42567=CARTESIAN_POINT('Ctrl Pts',(-64.9276335607206,1.96775265684681,-1.55761757373922));
#42568=CARTESIAN_POINT('Ctrl Pts',(-66.6139763255511,1.12810792023145,-1.44647968317117));
#42569=CARTESIAN_POINT('Ctrl Pts',(-66.8231158497185,-0.744224894574671,
-1.33534179260313));
#42570=CARTESIAN_POINT('Ctrl Pts',(-65.363492339427,-1.93530032858192,-1.22420390203509));
#42571=CARTESIAN_POINT('Ctrl Pts',(-63.5711826962814,-1.35500379861801,
-1.11306601146705));
#42572=CARTESIAN_POINT('Ctrl Pts',(-63.0866743105668,0.465558478971223,
-1.00192812089901));
#42573=CARTESIAN_POINT('Ctrl Pts',(-64.3534604207524,1.85998198910162,-0.890790230330965));
#42574=CARTESIAN_POINT('Ctrl Pts',(-66.2120286018649,1.55194685263457,-0.779652339762925));
#42575=CARTESIAN_POINT('Ctrl Pts',(-66.9612147484188,-0.176604847412408,
-0.668514449194881));
#42576=CARTESIAN_POINT('Ctrl Pts',(-65.915278038394,-1.74350710891129,-0.55737655862684));
#42577=CARTESIAN_POINT('Ctrl Pts',(-64.0315773430901,-1.7145580576145,-0.446238668058799));
#42578=CARTESIAN_POINT('Ctrl Pts',(-63.0342846939712,-0.116254309733247,
-0.335100777490757));
#42579=CARTESIAN_POINT('Ctrl Pts',(-63.8362336557469,1.58845819337163,-0.223962886922715));
#42580=CARTESIAN_POINT('Ctrl Pts',(-65.703391100443,1.83923696513466,-0.112824996354674));
#42581=CARTESIAN_POINT('Ctrl Pts',(-66.9267267192538,0.406541250167196,
-0.00168710578663183));
#42582=CARTESIAN_POINT('Ctrl Pts',(-66.3865075085097,-1.3982662642374,0.10945078478141));
#42583=CARTESIAN_POINT('Ctrl Pts',(-64.5772022576811,-1.9232248183573,0.220588675349452));
#42584=CARTESIAN_POINT('Ctrl Pts',(-63.1548885719436,-0.687833880924293,
0.331726565917493));
#42585=CARTESIAN_POINT('Ctrl Pts',(-63.4214263029693,1.17713920602489,0.442864456485535));
#42586=CARTESIAN_POINT('Ctrl Pts',(-65.1328504402804,1.96466342917937,0.554002347053577));
#42587=CARTESIAN_POINT('Ctrl Pts',(-66.7226750634076,0.953908934225895,
0.665140237621619));
#42588=CARTESIAN_POINT('Ctrl Pts',(-66.7357156643151,-0.929969225992781,
0.77627812818966));
#42589=CARTESIAN_POINT('Ctrl Pts',(-65.1600360334315,-1.96263600724144,
0.887416018757702));
#42590=CARTESIAN_POINT('Ctrl Pts',(-63.4378736061597,-1.19887979318002,
0.998553909325744));
#42591=CARTESIAN_POINT('Ctrl Pts',(-63.1455431829167,0.662224691762218,
1.10969179989378));
#42592=CARTESIAN_POINT('Ctrl Pts',(-64.5506181153062,1.91718740621521,1.22082969046183));
#42593=CARTESIAN_POINT('Ctrl Pts',(-66.3670173831005,1.41732674536556,1.33196758102987));
#42594=CARTESIAN_POINT('Ctrl Pts',(-66.9321701371076,-0.379829159090671,
1.44310547159791));
#42595=CARTESIAN_POINT('Ctrl Pts',(-65.7287856523224,-1.82932312667812,
1.55424336216595));
#42596=CARTESIAN_POINT('Ctrl Pts',(-63.858335394974,-1.60441689048052,1.66538125273399));
#42597=CARTESIAN_POINT('Ctrl Pts',(-63.0328636979636,0.0890303208983267,
1.77651914330204));
#42598=CARTESIAN_POINT('Ctrl Pts',(-64.00793416705,1.70098706988676,1.88765703387008));
#42599=CARTESIAN_POINT('Ctrl Pts',(-65.8910537438272,1.75601106330229,1.99879492443812));
#42600=CARTESIAN_POINT('Ctrl Pts',(-66.9585817236427,0.203738215957406,
2.10993281500616));
#42601=CARTESIAN_POINT('Ctrl Pts',(-66.2333976399805,-1.53501853100184,
2.2210707055742));
#42602=CARTESIAN_POINT('Ctrl Pts',(-64.3792707087636,-1.86875540824093,
2.33220859614224));
#42603=CARTESIAN_POINT('Ctrl Pts',(-63.0933043373643,-0.491999267189342,
2.44334648671029));
#42604=CARTESIAN_POINT('Ctrl Pts',(-63.5525581293749,1.33508938277185,2.55448437727833));
#42605=CARTESIAN_POINT('Ctrl Pts',(-65.336671880676,1.94015557973857,2.66562226784637));
#42606=CARTESIAN_POINT('Ctrl Pts',(-66.8126260414754,0.76937537170984,2.77676015841441));
#42607=CARTESIAN_POINT('Ctrl Pts',(-66.6294630299351,-1.10562283935512,
2.88789804898245));
#42608=CARTESIAN_POINT('Ctrl Pts',(-64.9548340277273,-1.9686319269424,2.9990359395505));
#42609=CARTESIAN_POINT('Ctrl Pts',(-63.3215459521581,-1.02972988599504,
3.11017383011853));
#42610=CARTESIAN_POINT('Ctrl Pts',(-63.2245659015414,0.851695597535297,
3.22131172068658));
#42611=CARTESIAN_POINT('Ctrl Pts',(-64.7526608160373,1.95355444175552,3.33244961125462));
#42612=CARTESIAN_POINT('Ctrl Pts',(-66.507148090629,1.26730275062476,3.44358750182267));
#42613=CARTESIAN_POINT('Ctrl Pts',(-66.8821256256507,-0.578925520347578,
3.5547253923907));
#42614=CARTESIAN_POINT('Ctrl Pts',(-65.5343722307488,-1.89525669707584,
3.66586328295875));
#42615=CARTESIAN_POINT('Ctrl Pts',(-63.6975018728677,-1.47683792531352,
3.77700117352679));
#42616=CARTESIAN_POINT('Ctrl Pts',(-63.0528228220476,0.293347348000542,
3.88813906409483));
#42617=CARTESIAN_POINT('Ctrl Pts',(-64.1904171247705,1.79502846684326,3.99927695466287));
#42618=CARTESIAN_POINT('Ctrl Pts',(-66.0690318143434,1.65369967309779,4.11041484523092));
#42619=CARTESIAN_POINT('Ctrl Pts',(-66.9691495608818,-0.0012791859021568,
4.22155273579895));
#42620=CARTESIAN_POINT('Ctrl Pts',(-66.0668823821194,-1.65508719106911,
4.332690626367));
#42621=CARTESIAN_POINT('Ctrl Pts',(-64.18808566082,-1.7939751212115,4.44382851693504));
#42622=CARTESIAN_POINT('Ctrl Pts',(-63.0524433397656,-0.2908172760207,4.55496640750308));
#42623=CARTESIAN_POINT('Ctrl Pts',(-63.6994217208407,1.47852891640211,4.66610429807113));
#42624=CARTESIAN_POINT('Ctrl Pts',(-65.5368341420657,1.89456083108635,4.77724218863916));
#42625=CARTESIAN_POINT('Ctrl Pts',(-66.8828762013613,0.576479717290691,
4.88838007920721));
#42626=CARTESIAN_POINT('Ctrl Pts',(-66.5055002879113,-1.26925979184896,
4.99951796977524));
#42627=CARTESIAN_POINT('Ctrl Pts',(-64.7501229512331,-1.95323147358089,
5.11065586034329));
#42628=CARTESIAN_POINT('Ctrl Pts',(-63.2234607852226,-0.849388129011331,
5.22179375091133));
#42629=CARTESIAN_POINT('Ctrl Pts',(-63.3228853580159,1.03190959101695,5.33293164147937));
#42630=CARTESIAN_POINT('Ctrl Pts',(-64.9573914929873,1.96868917726371,5.44406953204741));
#42631=CARTESIAN_POINT('Ctrl Pts',(-66.6308986426797,1.1035044097993,5.55520742261545));
#42632=CARTESIAN_POINT('Ctrl Pts',(-66.81162386615,-0.77172883509138,5.6663453131835));
#42633=CARTESIAN_POINT('Ctrl Pts',(-65.3341529720446,-1.94059312645931,
5.77748320375154));
#42634=CARTESIAN_POINT('Ctrl Pts',(-63.5508206739898,-1.33320420894148,
5.88862109431958));
#42635=CARTESIAN_POINT('Ctrl Pts',(-63.0939532378585,0.494469193338827,
5.99975898488762));
#42636=CARTESIAN_POINT('Ctrl Pts',(-64.3816832495733,1.86957387961578,6.11089687545566));
#42637=CARTESIAN_POINT('Ctrl Pts',(-66.2354223250123,1.53338799329774,6.22203476602371));
#42638=CARTESIAN_POINT('Ctrl Pts',(-66.9582534711981,-0.206229878053776,
6.33317265659175));
#42639=CARTESIAN_POINT('Ctrl Pts',(-65.8888935976679,-1.75727139133822,
6.44431054715979));
#42640=CARTESIAN_POINT('Ctrl Pts',(-64.0054842591603,-1.6994913560062,6.55544843772783));
#42641=CARTESIAN_POINT('Ctrl Pts',(-63.0332255100097,-0.0868797841564816,
6.66658632829588));
#42642=CARTESIAN_POINT('Ctrl Pts',(-63.8594705600155,1.60670204481743,6.77772421886391));
#42643=CARTESIAN_POINT('Ctrl Pts',(-65.733173098458,1.8267438654652,6.88886210943197));
#42644=CARTESIAN_POINT('Ctrl Pts',(-66.5289776062776,0.862949857291917,
6.96295403647732));
#42645=CARTESIAN_POINT('Ctrl Pts',(-66.6351293272515,0.319230454628283,
7.));
#42646=CARTESIAN_POINT('Ctrl Pts',(-66.6638321395092,-0.000941642735140673,
-1.3785196366098));
#42647=CARTESIAN_POINT('Ctrl Pts',(-66.664949390616,-0.216825623511897,
-1.36412702194091));
#42648=CARTESIAN_POINT('Ctrl Pts',(-66.625958965974,-0.432322760104835,
-1.34973440727202));
#42649=CARTESIAN_POINT('Ctrl Pts',(-66.5449886773087,-0.630681997774858,
-1.33534179260313));
#42650=CARTESIAN_POINT('Ctrl Pts',(-66.3365746796213,-1.14125003924375,
-1.29829582908045));
#42651=CARTESIAN_POINT('Ctrl Pts',(-65.8500335095242,-1.53827518391284,
-1.26124986555777));
#42652=CARTESIAN_POINT('Ctrl Pts',(-65.308044650618,-1.64007166792006,-1.22420390203509));
#42653=CARTESIAN_POINT('Ctrl Pts',(-64.7660557917118,-1.74186815192728,
-1.18715793851241));
#42654=CARTESIAN_POINT('Ctrl Pts',(-64.1686192439966,-1.54843597527264,
-1.15011197498973));
#42655=CARTESIAN_POINT('Ctrl Pts',(-63.7891495725199,-1.14829284068045,
-1.11306601146705));
#42656=CARTESIAN_POINT('Ctrl Pts',(-63.4096799010432,-0.748149706088263,
-1.07602004794437));
#42657=CARTESIAN_POINT('Ctrl Pts',(-63.248177105805,-0.141295613558517,
-1.03897408442169));
#42658=CARTESIAN_POINT('Ctrl Pts',(-63.3785567265502,0.394535351061421,
-1.00192812089901));
#42659=CARTESIAN_POINT('Ctrl Pts',(-63.5089363472953,0.930366315681358,
-0.964882157376327));
#42660=CARTESIAN_POINT('Ctrl Pts',(-63.9311983840238,1.39517415239149,-0.927836193853646));
#42661=CARTESIAN_POINT('Ctrl Pts',(-64.4520907659069,1.57623888133538,-0.890790230330965));
#42662=CARTESIAN_POINT('Ctrl Pts',(-64.9729831477899,1.75730361027927,-0.853744266808285));
#42663=CARTESIAN_POINT('Ctrl Pts',(-65.5925058748274,1.65462523145692,-0.816698303285605));
#42664=CARTESIAN_POINT('Ctrl Pts',(-66.0271315961051,1.31519409203792,-0.779652339762925));
#42665=CARTESIAN_POINT('Ctrl Pts',(-66.422630141453,1.00632023733061,-0.745941438711882));
#42666=CARTESIAN_POINT('Ctrl Pts',(-66.6650238854461,0.501402189087542,
-0.712230537660838));
#42667=CARTESIAN_POINT('Ctrl Pts',(-66.6681941903091,-0.000864019930029195,
-0.678519636609795));
#42668=CARTESIAN_POINT('Ctrl Pts',(-65.5301702171886,1.98517432567173,-2.));
#42669=CARTESIAN_POINT('Ctrl Pts',(-65.5988381452818,1.9597491377265,-2.));
#42670=CARTESIAN_POINT('Ctrl Pts',(-65.6658026948317,1.93043476164841,-2.));
#42671=CARTESIAN_POINT('Ctrl Pts',(-65.7308748757751,1.89752507621341,-2.));
#42672=CARTESIAN_POINT('Ctrl Pts',(-65.7977553584739,1.86370085800765,-2.));
#42673=CARTESIAN_POINT('Ctrl Pts',(-65.8626376079658,1.8260780441936,-2.));
#42674=CARTESIAN_POINT('Ctrl Pts',(-65.9252852210993,1.78493106183313,-2.));
#42675=CARTESIAN_POINT('Ctrl Pts',(-65.9782205027365,1.75016314345881,-2.));
#42676=CARTESIAN_POINT('Ctrl Pts',(-66.0295599817195,1.71287801549812,-2.));
#42677=CARTESIAN_POINT('Ctrl Pts',(-66.0791382962128,1.67322322119406,-2.));
#42678=CARTESIAN_POINT('Ctrl Pts',(-66.101163220464,1.65560677235613,-2.));
#42679=CARTESIAN_POINT('Ctrl Pts',(-66.1228402691632,1.63752248214409,-2.));
#42680=CARTESIAN_POINT('Ctrl Pts',(-66.1441533920284,1.61898256263349,-2.));
#42681=CARTESIAN_POINT('Ctrl Pts',(-66.155865605901,1.60879430895232,-2.));
#42682=CARTESIAN_POINT('Ctrl Pts',(-66.1674679023596,1.59846845594816,-2.));
#42683=CARTESIAN_POINT('Ctrl Pts',(-66.1789574836616,1.58800698854217,-2.));
#42684=CARTESIAN_POINT('Ctrl Pts',(-66.189551288702,1.57836114129823,-2.));
#42685=CARTESIAN_POINT('Ctrl Pts',(-66.200050702827,1.56859848611553,-2.));
#42686=CARTESIAN_POINT('Ctrl Pts',(-66.2104376446146,1.55873603375639,-2.));
#42687=CARTESIAN_POINT('Ctrl Pts',(-66.2635229555616,1.50833126968935,-2.));
#42688=CARTESIAN_POINT('Ctrl Pts',(-66.313768296129,1.45523826476751,-2.));
#42689=CARTESIAN_POINT('Ctrl Pts',(-66.3609549723782,1.39971629736103,-2.));
#42690=CARTESIAN_POINT('Ctrl Pts',(-66.4077748713716,1.34462589658441,-2.));
#42691=CARTESIAN_POINT('Ctrl Pts',(-66.4515839789323,1.28714326375225,-2.));
#42692=CARTESIAN_POINT('Ctrl Pts',(-66.4921238713298,1.22749743717261,-2.));
#42693=CARTESIAN_POINT('Ctrl Pts',(-66.5258166843552,1.1779256311354,-2.));
#42694=CARTESIAN_POINT('Ctrl Pts',(-66.557250703582,1.12685898698918,-2.));
#42695=CARTESIAN_POINT('Ctrl Pts',(-66.5862499617227,1.07442250688702,-2.));
#42696=CARTESIAN_POINT('Ctrl Pts',(-66.5983545270548,1.05253502286566,-2.));
#42697=CARTESIAN_POINT('Ctrl Pts',(-66.6100345605411,1.03040883225302,-2.));
#42698=CARTESIAN_POINT('Ctrl Pts',(-66.6212758238105,1.00805294268584,-2.));
#42699=CARTESIAN_POINT('Ctrl Pts',(-66.626479288449,0.99770463235463,-2.));
#42700=CARTESIAN_POINT('Ctrl Pts',(-66.6315887267729,0.987307105195716,
-2.));
#42701=CARTESIAN_POINT('Ctrl Pts',(-66.6366026612658,0.976861256572228,
-2.));
#42702=CARTESIAN_POINT('Ctrl Pts',(-66.6418315208287,0.965967640880585,
-2.));
#42703=CARTESIAN_POINT('Ctrl Pts',(-66.6469528966416,0.95502894077258,-2.));
#42704=CARTESIAN_POINT('Ctrl Pts',(-66.6519637514146,0.944050420215775,
-2.));
#42705=CARTESIAN_POINT('Ctrl Pts',(-66.6805038460108,0.88152056664477,-2.));
#42706=CARTESIAN_POINT('Ctrl Pts',(-66.7054830227983,0.817657226303972,
-2.));
#42707=CARTESIAN_POINT('Ctrl Pts',(-66.7266778091886,0.752664675159687,
-2.));
#42708=CARTESIAN_POINT('Ctrl Pts',(-66.745888539861,0.693756112801375,-2.));
#42709=CARTESIAN_POINT('Ctrl Pts',(-66.761989915918,0.633919258266641,-2.));
#42710=CARTESIAN_POINT('Ctrl Pts',(-66.7747787781587,0.573301385906269,
-2.));
#42711=CARTESIAN_POINT('Ctrl Pts',(-66.7899084885612,0.501588137552653,
-2.));
#42712=CARTESIAN_POINT('Ctrl Pts',(-66.8004026737972,0.428780273118141,
-2.));
#42713=CARTESIAN_POINT('Ctrl Pts',(-66.8063365292405,0.355301138761098,
-2.));
#42714=CARTESIAN_POINT('Ctrl Pts',(-66.8076429326892,0.339123900294253,
-2.));
#42715=CARTESIAN_POINT('Ctrl Pts',(-66.8087280690516,0.322914206659548,
-2.));
#42716=CARTESIAN_POINT('Ctrl Pts',(-66.809592371063,0.306676740191003,-2.));
#42717=CARTESIAN_POINT('Ctrl Pts',(-66.8104842013183,0.289922106189788,
-2.));
#42718=CARTESIAN_POINT('Ctrl Pts',(-66.8111409153919,0.273131754426448,
-2.));
#42719=CARTESIAN_POINT('Ctrl Pts',(-66.8115624311287,0.256344928107124,
-2.));
#42720=CARTESIAN_POINT('Ctrl Pts',(-66.8132840454943,0.187781790785841,
-2.));
#42721=CARTESIAN_POINT('Ctrl Pts',(-66.8110938642221,0.119190445572534,
-2.));
#42722=CARTESIAN_POINT('Ctrl Pts',(-66.8051125395792,0.0509093848503468,
-2.));
#42723=CARTESIAN_POINT('Ctrl Pts',(-66.7991324434424,-0.0173576516048459,
-2.));
#42724=CARTESIAN_POINT('Ctrl Pts',(-66.7893623072956,-0.0853156030450349,
-2.));
#42725=CARTESIAN_POINT('Ctrl Pts',(-66.7758731021339,-0.152611158192487,
-2.));
#42726=CARTESIAN_POINT('Ctrl Pts',(-66.7661100688796,-0.201317418857648,
-2.));
#42727=CARTESIAN_POINT('Ctrl Pts',(-66.7543977966376,-0.249676426291085,
-2.));
#42728=CARTESIAN_POINT('Ctrl Pts',(-66.7407489756121,-0.297544567370963,
-2.));
#42729=CARTESIAN_POINT('Ctrl Pts',(-66.7305106871662,-0.33345153947013,
-2.));
#42730=CARTESIAN_POINT('Ctrl Pts',(-66.7191824845106,-0.369082153865889,
-2.));
#42731=CARTESIAN_POINT('Ctrl Pts',(-66.7067658073163,-0.404371614833105,
-2.));
#42732=CARTESIAN_POINT('Ctrl Pts',(-66.7026385143847,-0.416101801623694,
-2.));
#42733=CARTESIAN_POINT('Ctrl Pts',(-66.6983941579974,-0.427785083074775,
-2.));
#42734=CARTESIAN_POINT('Ctrl Pts',(-66.6940333669371,-0.439418945656692,
-2.));
#42735=CARTESIAN_POINT('Ctrl Pts',(-66.6709086373701,-0.501111863824717,
-2.));
#42736=CARTESIAN_POINT('Ctrl Pts',(-66.6445114917904,-0.561421289136837,
-2.));
#42737=CARTESIAN_POINT('Ctrl Pts',(-66.6148919773948,-0.620012996760754,
-2.));
#42738=CARTESIAN_POINT('Ctrl Pts',(-66.5940505455908,-0.661240380249061,
-2.));
#42739=CARTESIAN_POINT('Ctrl Pts',(-66.5716128408251,-0.701616780535153,
-2.));
#42740=CARTESIAN_POINT('Ctrl Pts',(-66.5475858839724,-0.741014396591259,
-2.));
#42741=CARTESIAN_POINT('Ctrl Pts',(-66.5398732602616,-0.753660983073549,
-2.));
#42742=CARTESIAN_POINT('Ctrl Pts',(-66.5319957124564,-0.766208337095444,
-2.));
#42743=CARTESIAN_POINT('Ctrl Pts',(-66.5239568318932,-0.778646543728548,
-2.));
#42744=CARTESIAN_POINT('Ctrl Pts',(-66.489711530036,-0.831632794408527,
-2.));
#42745=CARTESIAN_POINT('Ctrl Pts',(-66.4526108600326,-0.88253505652559,
-2.));
#42746=CARTESIAN_POINT('Ctrl Pts',(-66.4126890994474,-0.931037995737605,
-2.));
#42747=CARTESIAN_POINT('Ctrl Pts',(-66.3758798548211,-0.975759383982511,
-2.));
#42748=CARTESIAN_POINT('Ctrl Pts',(-66.3366716809453,-1.01844109086248,
-2.));
#42749=CARTESIAN_POINT('Ctrl Pts',(-66.295069969863,-1.05880296618531,-2.));
#42750=CARTESIAN_POINT('Ctrl Pts',(-66.2872852045854,-1.06635572585249,
-2.));
#42751=CARTESIAN_POINT('Ctrl Pts',(-66.279416574172,-1.07382715133633,-2.));
#42752=CARTESIAN_POINT('Ctrl Pts',(-66.2714656498818,-1.08121658606209,
-2.));
#42753=CARTESIAN_POINT('Origin',(-65.,8.88178419700125E-15,3.));
#42754=CARTESIAN_POINT('Origin',(-32.5,56.2916512459885,7.));
#42755=CARTESIAN_POINT('Ctrl Pts',(-33.041102980256,57.8673300091754,7.));
#42756=CARTESIAN_POINT('Ctrl Pts',(-32.9847118979873,57.8942994847411,7.));
#42757=CARTESIAN_POINT('Ctrl Pts',(-32.9268515768618,57.917755670378,7.));
#42758=CARTESIAN_POINT('Ctrl Pts',(-32.8678400671714,57.9378112590619,7.));
#42759=CARTESIAN_POINT('Ctrl Pts',(-32.8304073366668,57.9505331068888,7.));
#42760=CARTESIAN_POINT('Ctrl Pts',(-32.7925106112697,57.9618858705791,7.));
#42761=CARTESIAN_POINT('Ctrl Pts',(-32.7542246215315,57.9718900412361,7.));
#42762=CARTESIAN_POINT('Ctrl Pts',(-32.7280436567717,57.9787311557329,7.));
#42763=CARTESIAN_POINT('Ctrl Pts',(-32.7016805652138,57.9849415096174,7.));
#42764=CARTESIAN_POINT('Ctrl Pts',(-32.6751582403431,57.9905258831364,7.));
#42765=CARTESIAN_POINT('Ctrl Pts',(-32.661116442106,57.9934824356489,7.));
#42766=CARTESIAN_POINT('Ctrl Pts',(-32.647030211604,57.9962633358689,7.));
#42767=CARTESIAN_POINT('Ctrl Pts',(-32.6329169445875,57.9988669116766,7.));
#42768=CARTESIAN_POINT('Ctrl Pts',(-32.5680410965272,58.0108350256729,7.));
#42769=CARTESIAN_POINT('Ctrl Pts',(-32.5025225401415,58.0190759833092,7.));
#42770=CARTESIAN_POINT('Ctrl Pts',(-32.4367003119297,58.0236879112065,7.));
#42771=CARTESIAN_POINT('Ctrl Pts',(-32.3892242866025,58.0270143863442,7.));
#42772=CARTESIAN_POINT('Ctrl Pts',(-32.3415895128512,58.0284519444914,7.));
#42773=CARTESIAN_POINT('Ctrl Pts',(-32.2939162957138,58.0280221779993,7.));
#42774=CARTESIAN_POINT('Ctrl Pts',(-32.2808248420334,58.0279041606205,7.));
#42775=CARTESIAN_POINT('Ctrl Pts',(-32.2677304668452,58.0276452538024,7.));
#42776=CARTESIAN_POINT('Ctrl Pts',(-32.2546356188837,58.0272457331439,7.));
#42777=CARTESIAN_POINT('Ctrl Pts',(-32.2413147458909,58.0268393165162,7.));
#42778=CARTESIAN_POINT('Ctrl Pts',(-32.2280015697223,58.0262876036899,7.));
#42779=CARTESIAN_POINT('Ctrl Pts',(-32.2147036649184,58.0255917126641,7.));
#42780=CARTESIAN_POINT('Ctrl Pts',(-32.1469436448299,58.0220457713611,7.));
#42781=CARTESIAN_POINT('Ctrl Pts',(-32.0795415685586,58.0147589601543,7.));
#42782=CARTESIAN_POINT('Ctrl Pts',(-32.0128409972292,58.0038315324684,7.));
#42783=CARTESIAN_POINT('Ctrl Pts',(-31.9451753893333,57.992746004678,7.));
#42784=CARTESIAN_POINT('Ctrl Pts',(-31.8782306838316,57.9779139314839,7.));
#42785=CARTESIAN_POINT('Ctrl Pts',(-31.8123515211519,57.9593890229731,7.));
#42786=CARTESIAN_POINT('Ctrl Pts',(-31.7715359668474,57.9479118824244,7.));
#42787=CARTESIAN_POINT('Ctrl Pts',(-31.7311291966618,57.9350162531039,7.));
#42788=CARTESIAN_POINT('Ctrl Pts',(-31.6912132914853,57.9207048673026,7.));
#42789=CARTESIAN_POINT('Ctrl Pts',(-31.6585126282827,57.9089804229995,7.));
#42790=CARTESIAN_POINT('Ctrl Pts',(-31.6261413908417,57.8963056504121,7.));
#42791=CARTESIAN_POINT('Ctrl Pts',(-31.5941456455447,57.882678157395,7.));
#42792=CARTESIAN_POINT('Ctrl Pts',(-31.5810720086146,57.8771098890419,7.));
#42793=CARTESIAN_POINT('Ctrl Pts',(-31.5680588095099,57.8713813377768,7.));
#42794=CARTESIAN_POINT('Ctrl Pts',(-31.5551310603946,57.8655025241604,7.));
#42795=CARTESIAN_POINT('Ctrl Pts',(-31.4909683792072,57.8363249434027,7.));
#42796=CARTESIAN_POINT('Ctrl Pts',(-31.4287956225132,57.8034029003303,7.));
#42797=CARTESIAN_POINT('Ctrl Pts',(-31.3689686686499,57.7668089348087,7.));
#42798=CARTESIAN_POINT('Ctrl Pts',(-31.3623206919021,57.7627426099135,7.));
#42799=CARTESIAN_POINT('Ctrl Pts',(-31.3557016802768,57.758630892331,7.));
#42800=CARTESIAN_POINT('Ctrl Pts',(-31.349112123847,57.754473841822,7.));
#42801=CARTESIAN_POINT('Ctrl Pts',(-31.292085729188,57.7184984912095,7.));
#42802=CARTESIAN_POINT('Ctrl Pts',(-31.2372638568291,57.6791321880014,7.));
#42803=CARTESIAN_POINT('Ctrl Pts',(-31.1847406170358,57.6367028360825,7.));
#42804=CARTESIAN_POINT('Ctrl Pts',(-31.1282350066725,57.5910564434202,7.));
#42805=CARTESIAN_POINT('Ctrl Pts',(-31.0743888197007,57.5418647466793,7.));
#42806=CARTESIAN_POINT('Ctrl Pts',(-31.0233480125353,57.4894785917711,7.));
#42807=CARTESIAN_POINT('Ctrl Pts',(-31.0140057588989,57.4798900924238,7.));
#42808=CARTESIAN_POINT('Ctrl Pts',(-31.0047575878001,57.4701944335691,7.));
#42809=CARTESIAN_POINT('Ctrl Pts',(-30.9956045320055,57.4603935881043,7.));
#42810=CARTESIAN_POINT('Ctrl Pts',(-30.9877334098267,57.4519654026063,7.));
#42811=CARTESIAN_POINT('Ctrl Pts',(-30.9799390123112,57.4434662546016,7.));
#42812=CARTESIAN_POINT('Ctrl Pts',(-30.97222270825,57.4348989262801,7.));
#42813=CARTESIAN_POINT('Ctrl Pts',(-30.9246610656086,57.382091752692,7.));
#42814=CARTESIAN_POINT('Ctrl Pts',(-30.8800520828446,57.3266849226614,6.99999999999999));
#42815=CARTESIAN_POINT('Ctrl Pts',(-30.8384919343084,57.269046905134,7.));
#42816=CARTESIAN_POINT('Ctrl Pts',(-30.7960555283788,57.2101936431771,7.));
#42817=CARTESIAN_POINT('Ctrl Pts',(-30.7567972001627,57.1490134676405,7.));
#42818=CARTESIAN_POINT('Ctrl Pts',(-30.7208469685291,57.0858509474018,7.));
#42819=CARTESIAN_POINT('Ctrl Pts',(-30.6846788708758,57.0223056489095,7.));
#42820=CARTESIAN_POINT('Ctrl Pts',(-30.6518584166819,56.9567530677491,7.));
#42821=CARTESIAN_POINT('Ctrl Pts',(-30.6225557949111,56.8895077656693,7.));
#42822=CARTESIAN_POINT('Ctrl Pts',(-30.615313982694,56.8728888482922,7.));
#42823=CARTESIAN_POINT('Ctrl Pts',(-30.6082872382863,56.8561664056305,7.));
#42824=CARTESIAN_POINT('Ctrl Pts',(-30.6014785581591,56.8393449403756,7.));
#42825=CARTESIAN_POINT('Ctrl Pts',(-30.5961524551096,56.8261863170131,7.));
#42826=CARTESIAN_POINT('Ctrl Pts',(-30.5909593216311,56.8129655376061,7.));
#42827=CARTESIAN_POINT('Ctrl Pts',(-30.5859080295463,56.7997050114821,7.));
#42828=CARTESIAN_POINT('Ctrl Pts',(-30.5590883752802,56.7292987233359,7.));
#42829=CARTESIAN_POINT('Ctrl Pts',(-30.5362121102038,56.657649445443,7.));
#42830=CARTESIAN_POINT('Ctrl Pts',(-30.5174063250598,56.5851265990605,7.));
#42831=CARTESIAN_POINT('Ctrl Pts',(-30.4985800831807,56.5125248630894,7.));
#42832=CARTESIAN_POINT('Ctrl Pts',(-30.4838325489097,56.4390467229768,7.));
#42833=CARTESIAN_POINT('Ctrl Pts',(-30.473332189023,56.3650308461601,7.));
#42834=CARTESIAN_POINT('Ctrl Pts',(-30.4630708240431,56.2926996180384,7.));
#42835=CARTESIAN_POINT('Ctrl Pts',(-30.4568650767968,56.2198539025132,7.));
#42836=CARTESIAN_POINT('Ctrl Pts',(-30.4549187470094,56.1467933162297,7.));
#42837=CARTESIAN_POINT('Ctrl Pts',(-30.4545002099142,56.1310824301527,7.));
#42838=CARTESIAN_POINT('Ctrl Pts',(-30.454278824166,56.1153615760157,7.));
#42839=CARTESIAN_POINT('Ctrl Pts',(-30.4542569357503,56.0996336954517,7.));
#42840=CARTESIAN_POINT('Ctrl Pts',(-30.4542384011809,56.0863157149704,7.));
#42841=CARTESIAN_POINT('Ctrl Pts',(-30.4543629142851,56.0729926961468,7.));
#42842=CARTESIAN_POINT('Ctrl Pts',(-30.4546294175093,56.0596661744468,7.));
#42843=CARTESIAN_POINT('Ctrl Pts',(-30.845746263986,55.0728640868079,7.));
#42844=CARTESIAN_POINT('Ctrl Pts',(-30.8954489009033,55.0171697369536,7.));
#42845=CARTESIAN_POINT('Ctrl Pts',(-30.9483278083006,54.9645336576551,7.));
#42846=CARTESIAN_POINT('Ctrl Pts',(-31.0040355064145,54.9150549467046,7.));
#42847=CARTESIAN_POINT('Ctrl Pts',(-31.0582842091438,54.8668720927604,7.));
#42848=CARTESIAN_POINT('Ctrl Pts',(-31.1152164855349,54.8216833321975,7.));
#42849=CARTESIAN_POINT('Ctrl Pts',(-31.1745316088105,54.7796213191364,7.));
#42850=CARTESIAN_POINT('Ctrl Pts',(-31.1877704600013,54.7702332794435,7.));
#42851=CARTESIAN_POINT('Ctrl Pts',(-31.2011298594679,54.7609999646249,7.));
#42852=CARTESIAN_POINT('Ctrl Pts',(-31.2146007867298,54.7519269992828,7.));
#42853=CARTESIAN_POINT('Ctrl Pts',(-31.2764177232488,54.7102919349934,7.));
#42854=CARTESIAN_POINT('Ctrl Pts',(-31.3404582881863,54.6721113380502,7.));
#42855=CARTESIAN_POINT('Ctrl Pts',(-31.4063841817531,54.6375086610803,7.));
#42856=CARTESIAN_POINT('Ctrl Pts',(-31.4526685064183,54.6132153000274,7.));
#42857=CARTESIAN_POINT('Ctrl Pts',(-31.4998826447241,54.5906864697851,7.));
#42858=CARTESIAN_POINT('Ctrl Pts',(-31.5479126490946,54.5699799287714,7.));
#42859=CARTESIAN_POINT('Ctrl Pts',(-31.5661734309803,54.5621073992138,7.));
#42860=CARTESIAN_POINT('Ctrl Pts',(-31.5845521539812,54.5544984108625,7.));
#42861=CARTESIAN_POINT('Ctrl Pts',(-31.6030425578044,54.547156631718,7.));
#42862=CARTESIAN_POINT('Ctrl Pts',(-31.620650668295,54.5401651749813,7.));
#42863=CARTESIAN_POINT('Ctrl Pts',(-31.6383657025794,54.5334141284368,7.));
#42864=CARTESIAN_POINT('Ctrl Pts',(-31.6561506799727,54.5269179584906,7.));
#42865=CARTESIAN_POINT('Ctrl Pts',(-31.7243409104461,54.5020106833212,7.));
#42866=CARTESIAN_POINT('Ctrl Pts',(-31.7936290801199,54.4808156486368,6.99999999999999));
#42867=CARTESIAN_POINT('Ctrl Pts',(-31.8637026772369,54.4634492155475,7.));
#42868=CARTESIAN_POINT('Ctrl Pts',(-31.9322713956587,54.4464557385536,7.));
#42869=CARTESIAN_POINT('Ctrl Pts',(-32.0015931056162,54.4331281708393,7.));
#42870=CARTESIAN_POINT('Ctrl Pts',(-32.0713763155884,54.4236245382242,7.));
#42871=CARTESIAN_POINT('Ctrl Pts',(-32.1396290845225,54.4143293332434,7.));
#42872=CARTESIAN_POINT('Ctrl Pts',(-32.2083241026487,54.4086921780503,7.));
#42873=CARTESIAN_POINT('Ctrl Pts',(-32.2771775099492,54.406908383857,7.));
#42874=CARTESIAN_POINT('Ctrl Pts',(-32.2995513064291,54.4063287429966,7.));
#42875=CARTESIAN_POINT('Ctrl Pts',(-32.3219416905641,54.4061563640051,7.));
#42876=CARTESIAN_POINT('Ctrl Pts',(-32.3443384584988,54.4063990611232,7.));
#42877=CARTESIAN_POINT('Ctrl Pts',(-32.3569726506304,54.4065359684675,7.));
#42878=CARTESIAN_POINT('Ctrl Pts',(-32.3696101789338,54.4068051101078,7.));
#42879=CARTESIAN_POINT('Ctrl Pts',(-32.3822313250428,54.4072071047712,7.));
#42880=CARTESIAN_POINT('Ctrl Pts',(-32.4504997768709,54.4093815153262,7.));
#42881=CARTESIAN_POINT('Ctrl Pts',(-32.5184090635457,54.415438958281,7.));
#42882=CARTESIAN_POINT('Ctrl Pts',(-32.585689693705,54.425518870341,7.));
#42883=CARTESIAN_POINT('Ctrl Pts',(-32.5954003976719,54.4269737176246,7.));
#42884=CARTESIAN_POINT('Ctrl Pts',(-32.6050979864,54.4285124457434,7.));
#42885=CARTESIAN_POINT('Ctrl Pts',(-32.6147816267372,54.4301355621262,7.));
#42886=CARTESIAN_POINT('Ctrl Pts',(-32.6832009663017,54.4416036203236,7.));
#42887=CARTESIAN_POINT('Ctrl Pts',(-32.7509260352975,54.4572806254693,7.));
#42888=CARTESIAN_POINT('Ctrl Pts',(-32.8176612516198,54.4769468185411,7.));
#42889=CARTESIAN_POINT('Ctrl Pts',(-32.8799198172771,54.4952937879535,7.));
#42890=CARTESIAN_POINT('Ctrl Pts',(-32.9413172465657,54.5171136895481,7.));
#42891=CARTESIAN_POINT('Ctrl Pts',(-33.001588117662,54.5422590913447,7.));
#42892=CARTESIAN_POINT('Ctrl Pts',(-33.0148899910673,54.5478087199686,7.));
#42893=CARTESIAN_POINT('Ctrl Pts',(-33.0281368750967,54.553520427381,7.));
#42894=CARTESIAN_POINT('Ctrl Pts',(-33.0413257085627,54.5593927822482,7.));
#42895=CARTESIAN_POINT('Ctrl Pts',(-33.0516354979444,54.5639832368939,7.));
#42896=CARTESIAN_POINT('Ctrl Pts',(-33.0619091366824,54.5686716446581,7.));
#42897=CARTESIAN_POINT('Ctrl Pts',(-33.0721334453033,54.5734515734285,7.));
#42898=CARTESIAN_POINT('Ctrl Pts',(-33.1340731263268,54.6024087649934,7.));
#42899=CARTESIAN_POINT('Ctrl Pts',(-33.1943201438779,54.6347718932848,7.));
#42900=CARTESIAN_POINT('Ctrl Pts',(-33.2526025547971,54.6703158300039,7.));
#42901=CARTESIAN_POINT('Ctrl Pts',(-33.3106158338828,54.7056956347883,7.));
#42902=CARTESIAN_POINT('Ctrl Pts',(-33.3666833863001,54.7442277671715,7.));
#42903=CARTESIAN_POINT('Ctrl Pts',(-33.4205013719045,54.7857268573937,7.));
#42904=CARTESIAN_POINT('Ctrl Pts',(-33.4731665002094,54.8263369784627,7.));
#42905=CARTESIAN_POINT('Ctrl Pts',(-33.5236779675191,54.8697891009662,7.));
#42906=CARTESIAN_POINT('Ctrl Pts',(-33.5717071750615,54.9159326392887,7.));
#42907=CARTESIAN_POINT('Ctrl Pts',(-33.5818268625425,54.9256550188778,7.));
#42908=CARTESIAN_POINT('Ctrl Pts',(-33.5918361779058,54.9354969405856,7.));
#42909=CARTESIAN_POINT('Ctrl Pts',(-33.6017317565417,54.9454570807147,7.));
#42910=CARTESIAN_POINT('Ctrl Pts',(-33.6111117333518,54.9548982550889,7.));
#42911=CARTESIAN_POINT('Ctrl Pts',(-33.6203906591309,54.9644470262927,7.));
#42912=CARTESIAN_POINT('Ctrl Pts',(-33.6295510503765,54.9740864760303,7.));
#42913=CARTESIAN_POINT('Ctrl Pts',(-33.6745642994388,55.021453770748,7.));
#42914=CARTESIAN_POINT('Ctrl Pts',(-33.7168018660127,55.0710902386183,7.));
#42915=CARTESIAN_POINT('Ctrl Pts',(-33.7559956007795,55.1228219100991,7.));
#42916=CARTESIAN_POINT('Ctrl Pts',(-33.7944439256698,55.1735697177282,7.));
#42917=CARTESIAN_POINT('Ctrl Pts',(-33.8299635738862,55.226334532935,7.));
#42918=CARTESIAN_POINT('Ctrl Pts',(-33.8622555274099,55.2809712641021,7.));
#42919=CARTESIAN_POINT('Ctrl Pts',(-33.8934985743347,55.3338332860427,7.));
#42920=CARTESIAN_POINT('Ctrl Pts',(-33.9217204567444,55.3884482092219,7.));
#42921=CARTESIAN_POINT('Ctrl Pts',(-33.9466019283097,55.4446928631591,7.));
#42922=CARTESIAN_POINT('Ctrl Pts',(-33.9507443557826,55.4540568350232,7.));
#42923=CARTESIAN_POINT('Ctrl Pts',(-33.9547940777389,55.4634659866381,7.));
#42924=CARTESIAN_POINT('Ctrl Pts',(-33.9587494776696,55.4729197548336,7.));
#42925=CARTESIAN_POINT('Ctrl Pts',(-33.9629351903496,55.4829239915992,7.));
#42926=CARTESIAN_POINT('Ctrl Pts',(-33.9670152760995,55.4929781929138,7.));
#42927=CARTESIAN_POINT('Ctrl Pts',(-33.9709895856635,55.5030806790321,7.));
#42928=CARTESIAN_POINT('Origin',(-32.5,56.2916512459885,-3.54592528053767));
#42929=CARTESIAN_POINT('Ctrl Pts',(-33.5295805874755,58.0719425970214,-1.79592528053768));
#42930=CARTESIAN_POINT('Ctrl Pts',(-33.61511160178,58.0235064542128,-1.79058130531689));
#42931=CARTESIAN_POINT('Ctrl Pts',(-34.2640553995263,57.5898394701862,-1.74819136657341));
#42932=CARTESIAN_POINT('Ctrl Pts',(-34.9180311095446,56.062943931961,-1.66875546430726));
#42933=CARTESIAN_POINT('Ctrl Pts',(-33.6191501107478,54.1363165628764,-1.55761757373921));
#42934=CARTESIAN_POINT('Ctrl Pts',(-31.2961996587746,54.182342369509,-1.44647968317118));
#42935=CARTESIAN_POINT('Ctrl Pts',(-30.0749499288325,56.1591174155132,-1.33534179260313));
#42936=CARTESIAN_POINT('Ctrl Pts',(-31.0734520820823,58.2571645498346,-1.22420390203509));
#42937=CARTESIAN_POINT('Ctrl Pts',(-32.7280434754779,58.4718761792196,-1.14439839801327));
#42938=CARTESIAN_POINT('Ctrl Pts',(-33.436201766478,58.1266820552905,-1.10163885751414));
#42939=CARTESIAN_POINT('Ctrl Pts',(-33.5268019957928,58.0733321975144,-1.09592528053768));
#42940=CARTESIAN_POINT('Ctrl Pts',(-33.5243188290626,58.0704843676251,-1.85407471946232));
#42941=CARTESIAN_POINT('Ctrl Pts',(-33.9297573522988,57.832304408809,-1.82862455259619));
#42942=CARTESIAN_POINT('Ctrl Pts',(-34.7395102025176,56.9114816531043,-1.76612842220737));
#42943=CARTESIAN_POINT('Ctrl Pts',(-34.4535014835806,54.8495668967864,-1.66658632829587));
#42944=CARTESIAN_POINT('Ctrl Pts',(-32.3487507516394,53.8677941230741,-1.55544843772783));
#42945=CARTESIAN_POINT('Ctrl Pts',(-30.3811218874153,55.1044118987673,-1.44431054715979));
#42946=CARTESIAN_POINT('Ctrl Pts',(-30.3535878576005,57.4278205885651,-1.33317265659175));
#42947=CARTESIAN_POINT('Ctrl Pts',(-32.0395408012642,58.5450270011374,-1.23642738069259));
#42948=CARTESIAN_POINT('Ctrl Pts',(-33.1630292684131,58.2758908569842,-1.17672806831612));
#42949=CARTESIAN_POINT('Ctrl Pts',(-33.5270487244507,58.0682282925651,-1.15407471946232));
#42950=CARTESIAN_POINT('Ctrl Pts',(-32.8002165734084,54.652924298309,-2.));
#42951=CARTESIAN_POINT('Ctrl Pts',(-32.2553008763615,54.5530951452,-1.96295403647732));
#42952=CARTESIAN_POINT('Ctrl Pts',(-31.067360018651,54.9418786009695,-1.88886210943196));
#42953=CARTESIAN_POINT('Ctrl Pts',(-30.5876880485778,56.766296704464,-1.77772421886392));
#42954=CARTESIAN_POINT('Ctrl Pts',(-31.862316082722,58.1542462926903,-1.66658632829587));
#42955=CARTESIAN_POINT('Ctrl Pts',(-33.7186881749666,57.8383051703362,-1.55544843772783));
#42956=CARTESIAN_POINT('Ctrl Pts',(-34.4605498617843,56.1062143874073,-1.44431054715979));
#42957=CARTESIAN_POINT('Ctrl Pts',(-33.4074116483786,54.5440967590365,-1.33317265659175));
#42958=CARTESIAN_POINT('Ctrl Pts',(-31.5239535863334,54.5814146779316,-1.22203476602371));
#42959=CARTESIAN_POINT('Ctrl Pts',(-30.5337591344129,56.1841922550788,-1.11089687545567));
#42960=CARTESIAN_POINT('Ctrl Pts',(-31.3433489080176,57.8852977549105,-0.999758984887625));
#42961=CARTESIAN_POINT('Ctrl Pts',(-33.2116035654679,58.127735859695,-0.888621094319583));
#42962=CARTESIAN_POINT('Ctrl Pts',(-34.4285349719857,56.689577194601,-0.777483203751541));
#42963=CARTESIAN_POINT('Ctrl Pts',(-33.880248629212,54.8871962644417,-0.6663453131835));
#42964=CARTESIAN_POINT('Ctrl Pts',(-32.068608990815,54.3703269630488,-0.555207422615458));
#42965=CARTESIAN_POINT('Ctrl Pts',(-30.6518244621988,55.6120685434762,-0.444069532047416));
#42966=CARTESIAN_POINT('Ctrl Pts',(-30.9266969543788,57.4758393880094,-0.332931641479374));
#42967=CARTESIAN_POINT('Ctrl Pts',(-32.6416310686724,58.2557096429586,-0.221793750911333));
#42968=CARTESIAN_POINT('Ctrl Pts',(-34.2269289097961,57.2378548494304,-0.11065586034329));
#42969=CARTESIAN_POINT('Ctrl Pts',(-34.2315490093866,55.3539292291843,0.000482030224750697));
#42970=CARTESIAN_POINT('Ctrl Pts',(-32.6512627267286,54.3283111741666,0.111619920792793));
#42971=CARTESIAN_POINT('Ctrl Pts',(-30.9325239231375,55.0997605683742,0.222757811360834));
#42972=CARTESIAN_POINT('Ctrl Pts',(-30.648513765023,56.9621610088766,0.333895701928876));
#42973=CARTESIAN_POINT('Ctrl Pts',(-32.0591899470587,58.2108362632709,0.445033592496918));
#42974=CARTESIAN_POINT('Ctrl Pts',(-33.8733445736998,57.7028597043182,0.55617148306496));
#42975=CARTESIAN_POINT('Ctrl Pts',(-34.4304613352259,55.9031880402636,0.667309373633001));
#42976=CARTESIAN_POINT('Ctrl Pts',(-33.2206049447144,54.4590811533792,0.778447264201042));
#42977=CARTESIAN_POINT('Ctrl Pts',(-31.3511706755799,54.6923464552708,0.889585154769085));
#42978=CARTESIAN_POINT('Ctrl Pts',(-30.5332729159539,56.3894735693294,1.00072304533713));
#42979=CARTESIAN_POINT('Ctrl Pts',(-31.5155427604288,57.9970628015172,1.11186093590517));
#42980=CARTESIAN_POINT('Ctrl Pts',(-33.3988974808522,58.0436694962151,1.22299882647321));
#42981=CARTESIAN_POINT('Ctrl Pts',(-34.4594811428284,56.4866340172583,1.33413671704125));
#42982=CARTESIAN_POINT('Ctrl Pts',(-33.7265294927624,54.7511285964951,1.44527460760929));
#42983=CARTESIAN_POINT('Ctrl Pts',(-31.8709214881723,54.4256810275324,1.55641249817734));
#42984=CARTESIAN_POINT('Ctrl Pts',(-30.5911161796977,55.808177161062,1.66755038874538));
#42985=CARTESIAN_POINT('Ctrl Pts',(-31.0585338801586,57.633202607495,1.77868827931342));
#42986=CARTESIAN_POINT('Ctrl Pts',(-32.845341867449,58.2302908785132,1.88982616988146));
#42987=CARTESIAN_POINT('Ctrl Pts',(-34.3160545270196,57.0529203082132,2.0009640604495));
#42988=CARTESIAN_POINT('Ctrl Pts',(-34.1245118825503,55.1787515318803,2.11210195101754));
#42989=CARTESIAN_POINT('Ctrl Pts',(-32.4460350887648,54.323232485012,2.22323984158559));
#42990=CARTESIAN_POINT('Ctrl Pts',(-30.8169529902366,55.2694294534524,2.33437773215363));
#42991=CARTESIAN_POINT('Ctrl Pts',(-30.7283829067961,57.1512776213849,2.44551562272167));
#42992=CARTESIAN_POINT('Ctrl Pts',(-32.2613940402695,58.2463000190907,2.55665351328971));
#42993=CARTESIAN_POINT('Ctrl Pts',(-34.0128039146597,57.5522102275515,2.66779140385775));
#42994=CARTESIAN_POINT('Ctrl Pts',(-34.3795272095987,55.7043165044764,2.77892929442579));
#42995=CARTESIAN_POINT('Ctrl Pts',(-33.0258979343037,54.3940169311364,2.89006718499384));
#42996=CARTESIAN_POINT('Ctrl Pts',(-31.1909083156522,54.8206435668173,3.00120507556188));
#42997=CARTESIAN_POINT('Ctrl Pts',(-30.5541451617937,56.5937002136053,3.11234296612992));
#42998=CARTESIAN_POINT('Ctrl Pts',(-31.6984450088403,58.0902880148654,3.22348085669796));
#42999=CARTESIAN_POINT('Ctrl Pts',(-33.5764172295469,57.9405631836441,3.334618747266));
#43000=CARTESIAN_POINT('Ctrl Pts',(-34.4691325526482,56.2815705559534,3.44575663783405));
#43001=CARTESIAN_POINT('Ctrl Pts',(-33.5594785188274,54.6318048981748,3.55689452840209));
#43002=CARTESIAN_POINT('Ctrl Pts',(-31.6800717814225,54.5013154264873,3.66803241897013));
#43003=CARTESIAN_POINT('Ctrl Pts',(-30.5511546410956,56.0095406341798,3.77917030953817));
#43004=CARTESIAN_POINT('Ctrl Pts',(-31.2060377591922,57.7759848842099,3.89030820010622));
#43005=CARTESIAN_POINT('Ctrl Pts',(-33.0452991908126,58.183801721693,4.00144609067425));
#43006=CARTESIAN_POINT('Ctrl Pts',(-34.3854420890035,56.8597117703073,4.1125839812423));
#43007=CARTESIAN_POINT('Ctrl Pts',(-33.9998184606928,55.0156695787891,4.22372187181034));
#43008=CARTESIAN_POINT('Ctrl Pts',(-32.2413939863492,54.3395478778331,4.33485976237838));
#43009=CARTESIAN_POINT('Ctrl Pts',(-30.7196745288183,55.4502085281907,4.44599765294642));
#43010=CARTESIAN_POINT('Ctrl Pts',(-30.8275071658684,57.3310512405927,4.55713554351446));
#43011=CARTESIAN_POINT('Ctrl Pts',(-32.4661914602743,58.2605193506652,4.66827343408251));
#43012=CARTESIAN_POINT('Ctrl Pts',(-34.135821096663,57.3878601553884,4.77941132465054));
#43013=CARTESIAN_POINT('Ctrl Pts',(-34.3081651275095,55.5118285147887,4.89054921521859));
#43014=CARTESIAN_POINT('Ctrl Pts',(-32.8254751197057,54.3495774612489,5.00168710578663));
#43015=CARTESIAN_POINT('Ctrl Pts',(-31.0448740266845,54.9649285726684,5.11282499635467));
#43016=CARTESIAN_POINT('Ctrl Pts',(-30.5961662731526,56.7946439827405,5.22396288692271));
#43017=CARTESIAN_POINT('Ctrl Pts',(-31.8900590533423,58.1639644570316,5.33510077749076));
#43018=CARTESIAN_POINT('Ctrl Pts',(-33.7422378333798,57.8195353749858,5.4462386680588));
#43019=CARTESIAN_POINT('Ctrl Pts',(-34.4573819695178,56.076616703484,5.55737655862684));
#43020=CARTESIAN_POINT('Ctrl Pts',(-33.3809127223489,54.5305214257639,5.66851444919489));
#43021=CARTESIAN_POINT('Ctrl Pts',(-31.4981330119909,54.5964085667956,5.77965233976292));
#43022=CARTESIAN_POINT('Ctrl Pts',(-30.532375624067,56.2139699170398,5.89079023033097));
#43023=CARTESIAN_POINT('Ctrl Pts',(-31.3676029490313,57.9026351433967,6.001928120899));
#43024=CARTESIAN_POINT('Ctrl Pts',(-33.2393344828578,58.116746001209,6.11306601146706));
#43025=CARTESIAN_POINT('Ctrl Pts',(-34.4343281672319,56.6603319824484,6.22420390203508));
#43026=CARTESIAN_POINT('Ctrl Pts',(-33.8588424113751,54.8664502505917,6.33534179260314));
#43027=CARTESIAN_POINT('Ctrl Pts',(-32.039526963185,54.3770911652606,6.44647968317117));
#43028=CARTESIAN_POINT('Ctrl Pts',(-30.6418187305185,55.640110798873,6.55761757373922));
#43029=CARTESIAN_POINT('Ctrl Pts',(-30.9446640768632,57.4995720858052,6.66875546430725));
#43030=CARTESIAN_POINT('Ctrl Pts',(-32.6716452510335,58.2532519029269,6.7798933548753));
#43031=CARTESIAN_POINT('Ctrl Pts',(-34.2404831962863,57.2117704392446,6.89103124544334));
#43032=CARTESIAN_POINT('Ctrl Pts',(-34.2183071453089,55.3274697977207,7.00216913601138));
#43033=CARTESIAN_POINT('Ctrl Pts',(-32.6190914442239,54.3269220694063,7.11330702657942));
#43034=CARTESIAN_POINT('Ctrl Pts',(-31.4873233416682,54.8574472987172,7.18739895362479));
#43035=CARTESIAN_POINT('Ctrl Pts',(-31.1587240665778,55.3034534568682,7.22444491714747));
#43036=CARTESIAN_POINT('Ctrl Pts',(-32.8235677524625,54.525462293325,-2.07481497238249));
#43037=CARTESIAN_POINT('Ctrl Pts',(-32.2362679063105,54.4178683176326,-2.03776900885981));
#43038=CARTESIAN_POINT('Ctrl Pts',(-30.9559276871686,54.8368917830921,-1.96367708181445));
#43039=CARTESIAN_POINT('Ctrl Pts',(-30.4389462976543,56.8032151562412,-1.85253919124641));
#43040=CARTESIAN_POINT('Ctrl Pts',(-31.8127163182479,58.2991210074573,-1.74140130067836));
#43041=CARTESIAN_POINT('Ctrl Pts',(-33.813479096939,57.9586056331394,-1.63026341011032));
#43042=CARTESIAN_POINT('Ctrl Pts',(-34.6130436110377,56.0917909022585,-1.51912551954228));
#43043=CARTESIAN_POINT('Ctrl Pts',(-33.477991135835,54.4081700269832,-1.40798762897424));
#43044=CARTESIAN_POINT('Ctrl Pts',(-31.4480356104804,54.448390575124,-1.29684973840619));
#43045=CARTESIAN_POINT('Ctrl Pts',(-30.3808227325528,56.1758339752236,-1.18571184783816));
#43046=CARTESIAN_POINT('Ctrl Pts',(-31.2533832993725,58.0092533532185,-1.07457395727011));
#43047=CARTESIAN_POINT('Ctrl Pts',(-33.2669528824098,58.2705485634922,-0.963436066702072));
#43048=CARTESIAN_POINT('Ctrl Pts',(-34.5785385674958,56.7205283175548,-0.85229817613403));
#43049=CARTESIAN_POINT('Ctrl Pts',(-33.9876059030427,54.7779561935981,-0.741160285565988));
#43050=CARTESIAN_POINT('Ctrl Pts',(-32.0350549182219,54.2208842229542,-0.630022394997947));
#43051=CARTESIAN_POINT('Ctrl Pts',(-30.5080713128749,55.5592098448765,-0.518884504429905));
#43052=CARTESIAN_POINT('Ctrl Pts',(-30.8043236932773,57.5679468590399,-0.407746613861863));
#43053=CARTESIAN_POINT('Ctrl Pts',(-32.6526472907505,58.4084762899819,-0.296608723293822));
#43054=CARTESIAN_POINT('Ctrl Pts',(-34.3612513615134,57.3114516183055,-0.185470832725779));
#43055=CARTESIAN_POINT('Ctrl Pts',(-34.3662308175897,55.2809921675532,-0.0743329421577381));
#43056=CARTESIAN_POINT('Ctrl Pts',(-32.6630281098851,54.1756003992724,0.0368049484103043));
#43057=CARTESIAN_POINT('Ctrl Pts',(-30.8106038901482,55.0070539855567,0.147942838978346));
#43058=CARTESIAN_POINT('Ctrl Pts',(-30.5045031059899,57.0143140041392,0.259080729546387));
#43059=CARTESIAN_POINT('Ctrl Pts',(-32.024903250764,58.3601126089029,0.370218620114429));
#43060=CARTESIAN_POINT('Ctrl Pts',(-33.9801648424124,57.8126250680988,0.48135651068247));
#43061=CARTESIAN_POINT('Ctrl Pts',(-34.5806147654118,55.8729729399783,0.592494401250512));
#43062=CARTESIAN_POINT('Ctrl Pts',(-33.2766543989477,54.3165418129426,0.703632291818553));
#43063=CARTESIAN_POINT('Ctrl Pts',(-31.2618134527171,54.5679507495101,0.814770182386596));
#43064=CARTESIAN_POINT('Ctrl Pts',(-30.3802986954812,56.3970822984609,0.925908072954637));
#43065=CARTESIAN_POINT('Ctrl Pts',(-31.4389705811804,58.1297116094828,1.03704596352268));
#43066=CARTESIAN_POINT('Ctrl Pts',(-33.4688147268869,58.1799434247416,1.14818385409072));
#43067=CARTESIAN_POINT('Ctrl Pts',(-34.6118917659325,56.5017999941153,1.25932174465876));
#43068=CARTESIAN_POINT('Ctrl Pts',(-33.8219303211561,54.6313050310708,1.3704596352268));
#43069=CARTESIAN_POINT('Ctrl Pts',(-31.8219910617071,54.2805437881517,1.48159752579485));
#43070=CARTESIAN_POINT('Ctrl Pts',(-30.4426410726264,55.7705720088982,1.59273541636289));
#43071=CARTESIAN_POINT('Ctrl Pts',(-30.9464150418056,57.737549964795,1.70387330693093));
#43072=CARTESIAN_POINT('Ctrl Pts',(-32.872202942073,58.381080425761,1.81501119749897));
#43073=CARTESIAN_POINT('Ctrl Pts',(-34.4573092683919,57.1121326627429,1.92614908806701));
#43074=CARTESIAN_POINT('Ctrl Pts',(-34.2508682239552,55.0921889540773,2.03728697863506));
#43075=CARTESIAN_POINT('Ctrl Pts',(-32.4418376379359,54.1701266840256,2.1484248692031));
#43076=CARTESIAN_POINT('Ctrl Pts',(-30.6860437215201,55.1899199052635,2.25956275977114));
#43077=CARTESIAN_POINT('Ctrl Pts',(-30.5905845584602,57.2181403171501,2.37070065033918));
#43078=CARTESIAN_POINT('Ctrl Pts',(-32.2428350032856,58.3983347751019,2.48183854090722));
#43079=CARTESIAN_POINT('Ctrl Pts',(-34.1304714860531,57.6502579074399,2.59297643147527));
#43080=CARTESIAN_POINT('Ctrl Pts',(-34.5257189268319,55.6586329549041,2.70411432204331));
#43081=CARTESIAN_POINT('Ctrl Pts',(-33.0668028606663,54.2464168231134,2.81525221261135));
#43082=CARTESIAN_POINT('Ctrl Pts',(-31.0890857081512,54.7062269531163,2.92639010317939));
#43083=CARTESIAN_POINT('Ctrl Pts',(-30.4027944078216,56.6171939183194,3.03752799374743));
#43084=CARTESIAN_POINT('Ctrl Pts',(-31.636099169942,58.2301879836331,3.14866588431547));
#43085=CARTESIAN_POINT('Ctrl Pts',(-33.660142159116,58.0688173884788,3.25980377488351));
#43086=CARTESIAN_POINT('Ctrl Pts',(-34.6222938731447,56.2807864686682,3.37094166545156));
#43087=CARTESIAN_POINT('Ctrl Pts',(-33.6418859366334,54.5027002027542,3.4820795560196));
#43088=CARTESIAN_POINT('Ctrl Pts',(-31.6162968524566,54.3620611147965,3.59321744658764));
#43089=CARTESIAN_POINT('Ctrl Pts',(-30.3995712810968,55.9875977569607,3.70435533715568));
#43090=CARTESIAN_POINT('Ctrl Pts',(-31.1053919366404,57.8914380058304,3.81549322772372));
#43091=CARTESIAN_POINT('Ctrl Pts',(-33.0877131684893,58.3309752906065,3.92663111829177));
#43092=CARTESIAN_POINT('Ctrl Pts',(-34.5320938721368,56.903896149825,4.0377690088598));
#43093=CARTESIAN_POINT('Ctrl Pts',(-34.116476009031,54.9164223052549,4.14890689942785));
#43094=CARTESIAN_POINT('Ctrl Pts',(-32.2212793229225,54.1877111062503,4.26004478999589));
#43095=CARTESIAN_POINT('Ctrl Pts',(-30.5811988331557,55.3847601775417,4.37118268056394));
#43096=CARTESIAN_POINT('Ctrl Pts',(-30.6974188126734,57.4118969284483,4.48232057113197));
#43097=CARTESIAN_POINT('Ctrl Pts',(-32.4635617944443,58.4136601021044,4.59345846170002));
#43098=CARTESIAN_POINT('Ctrl Pts',(-34.2630570813224,57.4731245038336,4.70459635226806));
#43099=CARTESIAN_POINT('Ctrl Pts',(-34.4488062226114,55.4511730352461,4.8157342428361));
#43100=CARTESIAN_POINT('Ctrl Pts',(-32.8507909365896,54.1985208018218,4.92687213340414));
#43101=CARTESIAN_POINT('Ctrl Pts',(-30.9316927097324,54.8617346072315,5.03801002397219));
#43102=CARTESIAN_POINT('Ctrl Pts',(-30.4480839679681,56.8337673173569,5.14914791454022));
#43103=CARTESIAN_POINT('Ctrl Pts',(-31.8426171679856,58.3095950614319,5.26028580510827));
#43104=CARTESIAN_POINT('Ctrl Pts',(-33.8388604739813,57.9383759022263,5.37142369567631));
#43105=CARTESIAN_POINT('Ctrl Pts',(-34.6096293165867,56.0598910775539,5.48256158624435));
#43106=CARTESIAN_POINT('Ctrl Pts',(-33.4494310938601,54.3935387891867,5.59369947681239));
#43107=CARTESIAN_POINT('Ctrl Pts',(-31.4202066831417,54.4645507053438,5.70483736738043));
#43108=CARTESIAN_POINT('Ctrl Pts',(-30.3793316112331,56.2079277768579,5.81597525794847));
#43109=CARTESIAN_POINT('Ctrl Pts',(-31.2795238466775,58.027939263068,5.92711314851652));
#43110=CARTESIAN_POINT('Ctrl Pts',(-33.2968407414035,58.2587039015876,6.03825103908456));
#43111=CARTESIAN_POINT('Ctrl Pts',(-34.5847823639128,56.6890083802673,6.1493889296526));
#43112=CARTESIAN_POINT('Ctrl Pts',(-33.9645346857694,54.7555965317121,6.26052682022065));
#43113=CARTESIAN_POINT('Ctrl Pts',(-32.0037108581305,54.2281745523389,6.37166471078868));
#43114=CARTESIAN_POINT('Ctrl Pts',(-30.4972873242539,55.5894332580934,6.48280260135673));
#43115=CARTESIAN_POINT('Ctrl Pts',(-30.823688318536,57.5935255124715,6.59394049192477));
#43116=CARTESIAN_POINT('Ctrl Pts',(-32.6849960096048,58.4058273841964,6.70507838249281));
#43117=CARTESIAN_POINT('Ctrl Pts',(-34.3758599154852,57.283338333678,6.81621627306086));
#43118=CARTESIAN_POINT('Ctrl Pts',(-34.3519589865932,55.2524746920756,6.92735416362889));
#43119=CARTESIAN_POINT('Ctrl Pts',(-32.6283545092383,54.1741032483986,7.03849205419694));
#43120=CARTESIAN_POINT('Ctrl Pts',(-31.4085562246361,54.7458933202255,7.1125839812423));
#43121=CARTESIAN_POINT('Ctrl Pts',(-31.0543981323805,55.2265903335147,7.14962994476498));
#43122=CARTESIAN_POINT('Ctrl Pts',(-32.8469189315166,54.3980002883409,-2.14962994476498));
#43123=CARTESIAN_POINT('Ctrl Pts',(-32.2172349362596,54.2826414900653,-2.1125839812423));
#43124=CARTESIAN_POINT('Ctrl Pts',(-30.8444953556861,54.7319049652148,-2.03849205419694));
#43125=CARTESIAN_POINT('Ctrl Pts',(-30.2902045467309,56.8401336080183,-1.9273541636289));
#43126=CARTESIAN_POINT('Ctrl Pts',(-31.7631165537738,58.4439957222243,-1.81621627306085));
#43127=CARTESIAN_POINT('Ctrl Pts',(-33.9082700189115,58.0789060959425,-1.70507838249281));
#43128=CARTESIAN_POINT('Ctrl Pts',(-34.7655373602912,56.0773674171098,-1.59394049192477));
#43129=CARTESIAN_POINT('Ctrl Pts',(-33.5485706232914,54.2722432949298,-1.48280260135673));
#43130=CARTESIAN_POINT('Ctrl Pts',(-31.3721176346275,54.3153664723165,-1.37166471078869));
#43131=CARTESIAN_POINT('Ctrl Pts',(-30.2278863306926,56.1674756953684,-1.26052682022064));
#43132=CARTESIAN_POINT('Ctrl Pts',(-31.1634176907274,58.1332089515266,-1.1493889296526));
#43133=CARTESIAN_POINT('Ctrl Pts',(-33.3223021993517,58.4133612672893,-1.03825103908456));
#43134=CARTESIAN_POINT('Ctrl Pts',(-34.7285421630059,56.7514794405087,-0.927113148516519));
#43135=CARTESIAN_POINT('Ctrl Pts',(-34.0949631768735,54.6687161227545,-0.815975257948477));
#43136=CARTESIAN_POINT('Ctrl Pts',(-32.0015008456287,54.0714414828596,-0.704837367380436));
#43137=CARTESIAN_POINT('Ctrl Pts',(-30.3643181635512,55.5063511462768,-0.593699476812394));
#43138=CARTESIAN_POINT('Ctrl Pts',(-30.6819504321758,57.6600543300704,-0.482561586244352));
#43139=CARTESIAN_POINT('Ctrl Pts',(-32.6636635128287,58.5612429370052,-0.371423695676311));
#43140=CARTESIAN_POINT('Ctrl Pts',(-34.4955738132308,57.3850483871807,-0.260285805108268));
#43141=CARTESIAN_POINT('Ctrl Pts',(-34.5009126257928,55.208055105922,-0.149147914540227));
#43142=CARTESIAN_POINT('Ctrl Pts',(-32.6747934930415,54.0228896243784,-0.0380100239721848));
#43143=CARTESIAN_POINT('Ctrl Pts',(-30.688683857159,54.914347402739,0.0731278665958571));
#43144=CARTESIAN_POINT('Ctrl Pts',(-30.3604924469569,57.0664669994018,0.184265757163898));
#43145=CARTESIAN_POINT('Ctrl Pts',(-31.9906165544693,58.5093889545349,0.295403647731941));
#43146=CARTESIAN_POINT('Ctrl Pts',(-34.086985111125,57.9223904318795,0.406541538299981));
#43147=CARTESIAN_POINT('Ctrl Pts',(-34.7307681955977,55.8427578396932,0.517679428868024));
#43148=CARTESIAN_POINT('Ctrl Pts',(-33.3327038531809,54.1740024725061,0.628817319436064));
#43149=CARTESIAN_POINT('Ctrl Pts',(-31.1724562298543,54.4435550437496,0.739955210004108));
#43150=CARTESIAN_POINT('Ctrl Pts',(-30.2273244750084,56.4046910275922,0.851093100572148));
#43151=CARTESIAN_POINT('Ctrl Pts',(-31.3623984019321,58.2623604174483,0.962230991140192));
#43152=CARTESIAN_POINT('Ctrl Pts',(-33.5387319729216,58.3162173532682,1.07336888170823));
#43153=CARTESIAN_POINT('Ctrl Pts',(-34.7643023890367,56.5169659709722,1.18450677227627));
#43154=CARTESIAN_POINT('Ctrl Pts',(-33.9173311495497,54.5114814656466,1.29564466284432));
#43155=CARTESIAN_POINT('Ctrl Pts',(-31.773060635242,54.135406548771,1.40678255341236));
#43156=CARTESIAN_POINT('Ctrl Pts',(-30.2941659655551,55.7329668567342,1.5179204439804));
#43157=CARTESIAN_POINT('Ctrl Pts',(-30.8342962034526,57.8418973220951,1.62905833454844));
#43158=CARTESIAN_POINT('Ctrl Pts',(-32.899064016697,58.5318699730086,1.74019622511648));
#43159=CARTESIAN_POINT('Ctrl Pts',(-34.5985640097643,57.1713450172728,1.85133411568453));
#43160=CARTESIAN_POINT('Ctrl Pts',(-34.37722456536,55.0056263762742,1.96247200625257));
#43161=CARTESIAN_POINT('Ctrl Pts',(-32.4376401871071,54.0170208830394,2.07360989682061));
#43162=CARTESIAN_POINT('Ctrl Pts',(-30.5551344528034,55.1104103570745,2.18474778738865));
#43163=CARTESIAN_POINT('Ctrl Pts',(-30.4527862101242,57.2850030129155,2.29588567795669));
#43164=CARTESIAN_POINT('Ctrl Pts',(-32.2242759663018,58.550369531113,2.40702356852473));
#43165=CARTESIAN_POINT('Ctrl Pts',(-34.2481390574465,57.7483055873284,2.51816145909278));
#43166=CARTESIAN_POINT('Ctrl Pts',(-34.6719106440651,55.6129494053317,2.62929934966082));
#43167=CARTESIAN_POINT('Ctrl Pts',(-33.107707787029,54.0988167150905,2.74043724022886));
#43168=CARTESIAN_POINT('Ctrl Pts',(-30.9872631006501,54.5918103394153,2.8515751307969));
#43169=CARTESIAN_POINT('Ctrl Pts',(-30.2514436538494,56.6406876230335,2.96271302136494));
#43170=CARTESIAN_POINT('Ctrl Pts',(-31.5737533310438,58.3700879524007,3.07385091193298));
#43171=CARTESIAN_POINT('Ctrl Pts',(-33.7438670886851,58.1970715933135,3.18498880250103));
#43172=CARTESIAN_POINT('Ctrl Pts',(-34.7754551936414,56.2800023813831,3.29612669306907));
#43173=CARTESIAN_POINT('Ctrl Pts',(-33.7242933544393,54.3735955073335,3.40726458363711));
#43174=CARTESIAN_POINT('Ctrl Pts',(-31.5525219234906,54.2228068031056,3.51840247420515));
#43175=CARTESIAN_POINT('Ctrl Pts',(-30.247987921098,55.9656548797417,3.62954036477319));
#43176=CARTESIAN_POINT('Ctrl Pts',(-31.0047461140886,58.0068911274507,3.74067825534123));
#43177=CARTESIAN_POINT('Ctrl Pts',(-33.1301271461661,58.4781488595201,3.85181614590928));
#43178=CARTESIAN_POINT('Ctrl Pts',(-34.67874565527,56.9480805293425,3.96295403647731));
#43179=CARTESIAN_POINT('Ctrl Pts',(-34.2331335573692,54.8171750317208,4.07409192704536));
#43180=CARTESIAN_POINT('Ctrl Pts',(-32.2011646594958,54.0358743346675,4.1852298176134));
#43181=CARTESIAN_POINT('Ctrl Pts',(-30.4427231374931,55.3193118268927,4.29636770818145));
#43182=CARTESIAN_POINT('Ctrl Pts',(-30.5673304594784,57.4927426163039,4.40750559874948));
#43183=CARTESIAN_POINT('Ctrl Pts',(-32.4609321286144,58.5668008535436,4.51864348931753));
#43184=CARTESIAN_POINT('Ctrl Pts',(-34.3902930659818,57.5583888522789,4.62978137988556));
#43185=CARTESIAN_POINT('Ctrl Pts',(-34.5894473177133,55.3905175557035,4.74091927045361));
#43186=CARTESIAN_POINT('Ctrl Pts',(-32.8761067534734,54.0474641423945,4.85205716102165));
#43187=CARTESIAN_POINT('Ctrl Pts',(-30.8185113927804,54.7585406417947,4.96319505158969));
#43188=CARTESIAN_POINT('Ctrl Pts',(-30.3000016627836,56.8728906519732,5.07433294215774));
#43189=CARTESIAN_POINT('Ctrl Pts',(-31.7951752826288,58.4552256658323,5.18547083272577));
#43190=CARTESIAN_POINT('Ctrl Pts',(-33.9354831145828,58.0572164294668,5.29660872329382));
#43191=CARTESIAN_POINT('Ctrl Pts',(-34.7618766636555,56.0431654516238,5.40774661386186));
#43192=CARTESIAN_POINT('Ctrl Pts',(-33.5179494653714,54.2565561526097,5.5188845044299));
#43193=CARTESIAN_POINT('Ctrl Pts',(-31.3422803542924,54.3326928438919,5.63002239499794));
#43194=CARTESIAN_POINT('Ctrl Pts',(-30.2262875983991,56.2018856366761,5.74116028556598));
#43195=CARTESIAN_POINT('Ctrl Pts',(-31.1914447443237,58.1532433827394,5.85229817613403));
#43196=CARTESIAN_POINT('Ctrl Pts',(-33.3543469999491,58.4006618019661,5.96343606670207));
#43197=CARTESIAN_POINT('Ctrl Pts',(-34.7352365605938,56.7176847780862,6.07457395727012));
#43198=CARTESIAN_POINT('Ctrl Pts',(-34.0702269601635,54.6447428128324,6.18571184783815));
#43199=CARTESIAN_POINT('Ctrl Pts',(-31.9678947530761,54.0792579394171,6.2968497384062));
#43200=CARTESIAN_POINT('Ctrl Pts',(-30.3527559179892,55.5387557173139,6.40798762897423));
#43201=CARTESIAN_POINT('Ctrl Pts',(-30.7027125602087,57.687478939138,6.51912551954228));
#43202=CARTESIAN_POINT('Ctrl Pts',(-32.6983467681761,58.5584028654659,6.63026341011033));
#43203=CARTESIAN_POINT('Ctrl Pts',(-34.5112366346841,57.3549062281114,6.74140130067836));
#43204=CARTESIAN_POINT('Ctrl Pts',(-34.4856108278775,55.1774795864306,6.85253919124641));
#43205=CARTESIAN_POINT('Ctrl Pts',(-32.6376175742527,54.0212844273909,6.96367708181445));
#43206=CARTESIAN_POINT('Ctrl Pts',(-31.329789107604,54.6343393417337,7.03776900885981));
#43207=CARTESIAN_POINT('Ctrl Pts',(-30.9500721981832,55.1497272101613,7.07481497238249));
#43208=CARTESIAN_POINT('Ctrl Pts',(-32.8702701105707,54.2705382833568,-2.22444491714747));
#43209=CARTESIAN_POINT('Ctrl Pts',(-32.1982019662087,54.147414662498,-2.18739895362479));
#43210=CARTESIAN_POINT('Ctrl Pts',(-30.7330630242036,54.6269181473375,-2.11330702657943));
#43211=CARTESIAN_POINT('Ctrl Pts',(-30.1414627958074,56.8770520597955,-2.00216913601138));
#43212=CARTESIAN_POINT('Ctrl Pts',(-31.7135167892996,58.5888704369912,-1.89103124544334));
#43213=CARTESIAN_POINT('Ctrl Pts',(-34.003060940884,58.1992065587457,-1.7798933548753));
#43214=CARTESIAN_POINT('Ctrl Pts',(-34.9180311095446,56.062943931961,-1.66875546430726));
#43215=CARTESIAN_POINT('Ctrl Pts',(-33.6191501107478,54.1363165628764,-1.55761757373921));
#43216=CARTESIAN_POINT('Ctrl Pts',(-31.2961996587746,54.182342369509,-1.44647968317118));
#43217=CARTESIAN_POINT('Ctrl Pts',(-30.0749499288325,56.1591174155132,-1.33534179260313));
#43218=CARTESIAN_POINT('Ctrl Pts',(-31.0734520820823,58.2571645498346,-1.22420390203509));
#43219=CARTESIAN_POINT('Ctrl Pts',(-33.3776515162936,58.5561739710865,-1.11306601146705));
#43220=CARTESIAN_POINT('Ctrl Pts',(-34.878545758516,56.7824305634625,-1.00192812089901));
#43221=CARTESIAN_POINT('Ctrl Pts',(-34.2023204507042,54.559476051911,-0.890790230330966));
#43222=CARTESIAN_POINT('Ctrl Pts',(-31.9679467730355,53.921998742765,-0.779652339762925));
#43223=CARTESIAN_POINT('Ctrl Pts',(-30.2205650142274,55.453492447677,-0.668514449194883));
#43224=CARTESIAN_POINT('Ctrl Pts',(-30.5595771710743,57.752161801101,-0.557376558626841));
#43225=CARTESIAN_POINT('Ctrl Pts',(-32.6746797349068,58.7140095840284,-0.4462386680588));
#43226=CARTESIAN_POINT('Ctrl Pts',(-34.6298962649481,57.4586451560558,-0.335100777490757));
#43227=CARTESIAN_POINT('Ctrl Pts',(-34.6355944339958,55.1351180442908,-0.223962886922716));
#43228=CARTESIAN_POINT('Ctrl Pts',(-32.6865588761979,53.8701788494842,-0.112824996354674));
#43229=CARTESIAN_POINT('Ctrl Pts',(-30.5667638241697,54.8216408199214,-0.00168710578663194));
#43230=CARTESIAN_POINT('Ctrl Pts',(-30.2164817879238,57.1186199946645,0.109450784781409));
#43231=CARTESIAN_POINT('Ctrl Pts',(-31.9563298581746,58.6586653001668,0.220588675349452));
#43232=CARTESIAN_POINT('Ctrl Pts',(-34.1938053798377,58.0321557956601,0.331726565917493));
#43233=CARTESIAN_POINT('Ctrl Pts',(-34.8809216257836,55.8125427394079,0.442864456485535));
#43234=CARTESIAN_POINT('Ctrl Pts',(-33.3887533074142,54.0314631320695,0.554002347053576));
#43235=CARTESIAN_POINT('Ctrl Pts',(-31.0830990069914,54.3191593379889,0.665140237621618));
#43236=CARTESIAN_POINT('Ctrl Pts',(-30.0743502545356,56.4122997567237,0.77627812818966));
#43237=CARTESIAN_POINT('Ctrl Pts',(-31.2858262226837,58.3950092254139,0.887416018757703));
#43238=CARTESIAN_POINT('Ctrl Pts',(-33.6086492189563,58.4524912817947,0.998553909325743));
#43239=CARTESIAN_POINT('Ctrl Pts',(-34.9167130121408,56.5321319478293,1.10969179989379));
#43240=CARTESIAN_POINT('Ctrl Pts',(-34.0127319779434,54.3916579002222,1.22082969046183));
#43241=CARTESIAN_POINT('Ctrl Pts',(-31.7241302087768,53.9902693093903,1.33196758102987));
#43242=CARTESIAN_POINT('Ctrl Pts',(-30.1456908584837,55.6953617045703,1.44310547159791));
#43243=CARTESIAN_POINT('Ctrl Pts',(-30.7221773650996,57.9462446793952,1.55424336216595));
#43244=CARTESIAN_POINT('Ctrl Pts',(-32.9259250913211,58.6826595202563,1.66538125273399));
#43245=CARTESIAN_POINT('Ctrl Pts',(-34.7398187511365,57.2305573718025,1.77651914330204));
#43246=CARTESIAN_POINT('Ctrl Pts',(-34.5035809067649,54.9190637984713,1.88765703387008));
#43247=CARTESIAN_POINT('Ctrl Pts',(-32.4334427362781,53.863915082053,1.99879492443812));
#43248=CARTESIAN_POINT('Ctrl Pts',(-30.4242251840869,55.0309008088856,2.10993281500616));
#43249=CARTESIAN_POINT('Ctrl Pts',(-30.3149878617883,57.3518657086808,2.22107070557421));
#43250=CARTESIAN_POINT('Ctrl Pts',(-32.2057169293179,58.7024042871241,2.33220859614224));
#43251=CARTESIAN_POINT('Ctrl Pts',(-34.3658066288398,57.8463532672169,2.44334648671029));
#43252=CARTESIAN_POINT('Ctrl Pts',(-34.8181023612983,55.5672658557593,2.55448437727833));
#43253=CARTESIAN_POINT('Ctrl Pts',(-33.1486127133916,53.9512166070675,2.66562226784637));
#43254=CARTESIAN_POINT('Ctrl Pts',(-30.8854404931491,54.4773937257141,2.77676015841441));
#43255=CARTESIAN_POINT('Ctrl Pts',(-30.1000928998773,56.6641813277477,2.88789804898245));
#43256=CARTESIAN_POINT('Ctrl Pts',(-31.5114074921456,58.5099879211684,2.99903593955049));
#43257=CARTESIAN_POINT('Ctrl Pts',(-33.8275920182542,58.3253257981482,3.11017383011854));
#43258=CARTESIAN_POINT('Ctrl Pts',(-34.9286165141379,56.2792182940979,3.22131172068658));
#43259=CARTESIAN_POINT('Ctrl Pts',(-33.8067007722453,54.2444908119128,3.33244961125462));
#43260=CARTESIAN_POINT('Ctrl Pts',(-31.4887469945246,54.0835524914147,3.44358750182266));
#43261=CARTESIAN_POINT('Ctrl Pts',(-30.0964045610992,55.9437120025227,3.5547253923907));
#43262=CARTESIAN_POINT('Ctrl Pts',(-30.9041002915367,58.1223442490711,3.66586328295875));
#43263=CARTESIAN_POINT('Ctrl Pts',(-33.1725411238429,58.6253224284337,3.77700117352679));
#43264=CARTESIAN_POINT('Ctrl Pts',(-34.8253974384033,56.9922649088601,3.88813906409483));
#43265=CARTESIAN_POINT('Ctrl Pts',(-34.3497911057075,54.7179277581866,3.99927695466287));
#43266=CARTESIAN_POINT('Ctrl Pts',(-32.1810499960691,53.8840375630848,4.11041484523091));
#43267=CARTESIAN_POINT('Ctrl Pts',(-30.3042474418304,55.2538634762437,4.22155273579896));
#43268=CARTESIAN_POINT('Ctrl Pts',(-30.4372421062834,57.5735883041595,4.332690626367));
#43269=CARTESIAN_POINT('Ctrl Pts',(-32.4583024627843,58.7199416049828,4.44382851693504));
#43270=CARTESIAN_POINT('Ctrl Pts',(-34.5175290506412,57.6436532007241,4.55496640750308));
#43271=CARTESIAN_POINT('Ctrl Pts',(-34.7300884128152,55.3298620761609,4.66610429807112));
#43272=CARTESIAN_POINT('Ctrl Pts',(-32.9014225703573,53.8964074829672,4.77724218863916));
#43273=CARTESIAN_POINT('Ctrl Pts',(-30.7053300758283,54.6553466763578,4.88838007920721));
#43274=CARTESIAN_POINT('Ctrl Pts',(-30.1519193575992,56.9120139865896,4.99951796977524));
#43275=CARTESIAN_POINT('Ctrl Pts',(-31.747733397272,58.6008562702326,5.11065586034329));
#43276=CARTESIAN_POINT('Ctrl Pts',(-34.0321057551843,58.1760569567072,5.22179375091132));
#43277=CARTESIAN_POINT('Ctrl Pts',(-34.9141240107244,56.0264398256936,5.33293164147938));
#43278=CARTESIAN_POINT('Ctrl Pts',(-33.5864678368826,54.1195735160326,5.44406953204741));
#43279=CARTESIAN_POINT('Ctrl Pts',(-31.2643540254432,54.2008349824401,5.55520742261546));
#43280=CARTESIAN_POINT('Ctrl Pts',(-30.0732435855652,56.1958434964943,5.66634531318349));
#43281=CARTESIAN_POINT('Ctrl Pts',(-31.10336564197,58.2785475024108,5.77748320375154));
#43282=CARTESIAN_POINT('Ctrl Pts',(-33.4118532584947,58.5426197023447,5.88862109431958));
#43283=CARTESIAN_POINT('Ctrl Pts',(-34.8856907572748,56.746361175905,5.99975898488762));
#43284=CARTESIAN_POINT('Ctrl Pts',(-34.1759192345577,54.5338890939528,6.11089687545567));
#43285=CARTESIAN_POINT('Ctrl Pts',(-31.9320786480218,53.9303413264953,6.2220347660237));
#43286=CARTESIAN_POINT('Ctrl Pts',(-30.2082245117245,55.4880781765344,6.33317265659175));
#43287=CARTESIAN_POINT('Ctrl Pts',(-30.5817368018815,57.7814323658043,6.44431054715979));
#43288=CARTESIAN_POINT('Ctrl Pts',(-32.7116975267474,58.7109783467354,6.55544843772783));
#43289=CARTESIAN_POINT('Ctrl Pts',(-34.646613353883,57.4264741225448,6.66658632829587));
#43290=CARTESIAN_POINT('Ctrl Pts',(-34.6192626691618,55.1024844807855,6.77772421886391));
#43291=CARTESIAN_POINT('Ctrl Pts',(-32.6468806392671,53.8684656063832,6.88886210943196));
#43292=CARTESIAN_POINT('Ctrl Pts',(-31.2510219905719,54.522785363242,6.96295403647732));
#43293=CARTESIAN_POINT('Ctrl Pts',(-30.845746263986,55.0728640868079,7.));
#43294=CARTESIAN_POINT('Ctrl Pts',(-32.8002165734084,54.652924298309,-2.));
#43295=CARTESIAN_POINT('Ctrl Pts',(-32.7409294910782,54.6348115493311,-2.));
#43296=CARTESIAN_POINT('Ctrl Pts',(-32.6807825146657,54.6203475870771,-2.));
#43297=CARTESIAN_POINT('Ctrl Pts',(-32.6200737029466,54.6093586318097,-2.));
#43298=CARTESIAN_POINT('Ctrl Pts',(-32.5553553259177,54.5976439016081,-2.));
#43299=CARTESIAN_POINT('Ctrl Pts',(-32.4899978846727,54.589877844864,-2.));
#43300=CARTESIAN_POINT('Ctrl Pts',(-32.4243295074668,54.5859022602815,-2.));
#43301=CARTESIAN_POINT('Ctrl Pts',(-32.3668696774116,54.5824236237718,-2.));
#43302=CARTESIAN_POINT('Ctrl Pts',(-32.3091708471323,54.5818478912345,-2.));
#43303=CARTESIAN_POINT('Ctrl Pts',(-32.2514404192194,54.5841026889814,-2.));
#43304=CARTESIAN_POINT('Ctrl Pts',(-32.2224739676372,54.5852340419286,-2.));
#43305=CARTESIAN_POINT('Ctrl Pts',(-32.193499433327,54.5870784902624,-2.));
#43306=CARTESIAN_POINT('Ctrl Pts',(-32.1645425913577,54.5896298423984,-2.));
#43307=CARTESIAN_POINT('Ctrl Pts',(-32.1513153330279,54.5907952800462,-2.));
#43308=CARTESIAN_POINT('Ctrl Pts',(-32.138090039214,54.5921085587763,-2.));
#43309=CARTESIAN_POINT('Ctrl Pts',(-32.1248906604564,54.5935664859841,-2.));
#43310=CARTESIAN_POINT('Ctrl Pts',(-32.058315745723,54.6009199668814,-2.));
#43311=CARTESIAN_POINT('Ctrl Pts',(-31.9922802588103,54.6119586521809,-2.));
#43312=CARTESIAN_POINT('Ctrl Pts',(-31.9271057840949,54.6265240331791,-2.));
#43313=CARTESIAN_POINT('Ctrl Pts',(-31.8607754217491,54.6413477353037,-2.));
#43314=CARTESIAN_POINT('Ctrl Pts',(-31.7953358755736,54.6598242742457,-2.));
#43315=CARTESIAN_POINT('Ctrl Pts',(-31.7311141838629,54.6818388621519,-2.));
#43316=CARTESIAN_POINT('Ctrl Pts',(-31.6773947912169,54.7002533613681,-2.));
#43317=CARTESIAN_POINT('Ctrl Pts',(-31.6245269677682,54.7211443093799,-2.));
#43318=CARTESIAN_POINT('Ctrl Pts',(-31.5727038894035,54.744472176156,-2.));
#43319=CARTESIAN_POINT('Ctrl Pts',(-31.5488262835586,54.7552205459106,-2.));
#43320=CARTESIAN_POINT('Ctrl Pts',(-31.5251705391772,54.7664866028715,-2.));
#43321=CARTESIAN_POINT('Ctrl Pts',(-31.5017561059839,54.7782682438534,-2.));
#43322=CARTESIAN_POINT('Ctrl Pts',(-31.4915364297196,54.783410565929,-2.));
#43323=CARTESIAN_POINT('Ctrl Pts',(-31.4813629900352,54.788651093074,-2.));
#43324=CARTESIAN_POINT('Ctrl Pts',(-31.4712497594445,54.7939828998655,-2.));
#43325=CARTESIAN_POINT('Ctrl Pts',(-31.4091712444154,54.8267113781765,-2.));
#43326=CARTESIAN_POINT('Ctrl Pts',(-31.3492415725568,54.8629343648207,-2.));
#43327=CARTESIAN_POINT('Ctrl Pts',(-31.2918005106532,54.9025187988196,-2.));
#43328=CARTESIAN_POINT('Ctrl Pts',(-31.2404435140348,54.9379105129636,-2.));
#43329=CARTESIAN_POINT('Ctrl Pts',(-31.1910752071313,54.9759900914521,-2.));
#43330=CARTESIAN_POINT('Ctrl Pts',(-31.1439444839342,55.0166972030901,-2.));
#43331=CARTESIAN_POINT('Ctrl Pts',(-31.0925988211627,55.0610447854056,-2.));
#43332=CARTESIAN_POINT('Ctrl Pts',(-31.043907590923,55.1085103565088,-2.));
#43333=CARTESIAN_POINT('Ctrl Pts',(-30.9979331337683,55.1587747363345,-2.));
#43334=CARTESIAN_POINT('Ctrl Pts',(-30.9801952413171,55.1781677693066,-2.));
#43335=CARTESIAN_POINT('Ctrl Pts',(-30.9628620787172,55.1979778819355,-2.));
#43336=CARTESIAN_POINT('Ctrl Pts',(-30.9459385065311,55.2181883203223,-2.));
#43337=CARTESIAN_POINT('Ctrl Pts',(-30.9385143505228,55.2270543827546,-2.));
#43338=CARTESIAN_POINT('Ctrl Pts',(-30.9311694717142,55.2359970996698,-2.));
#43339=CARTESIAN_POINT('Ctrl Pts',(-30.9239125746492,55.2450044081202,-2.));
#43340=CARTESIAN_POINT('Ctrl Pts',(-30.8800390053309,55.2994605714266,-2.));
#43341=CARTESIAN_POINT('Ctrl Pts',(-30.839297247442,55.3563704442389,-2.));
#43342=CARTESIAN_POINT('Ctrl Pts',(-30.8017204449776,55.4153538312132,-2.));
#43343=CARTESIAN_POINT('Ctrl Pts',(-30.7632731033033,55.4757036822749,-2.));
#43344=CARTESIAN_POINT('Ctrl Pts',(-30.7281385018958,55.5382249056899,-2.));
#43345=CARTESIAN_POINT('Ctrl Pts',(-30.6963834281772,55.6025570259723,-2.));
#43346=CARTESIAN_POINT('Ctrl Pts',(-30.6720872116827,55.6517783609874,-2.));
#43347=CARTESIAN_POINT('Ctrl Pts',(-30.6497699435193,55.7020608595674,-2.));
#43348=CARTESIAN_POINT('Ctrl Pts',(-30.6294765723463,55.7532569215852,-2.));
#43349=CARTESIAN_POINT('Ctrl Pts',(-30.6168451594751,55.7851234158808,-2.));
#43350=CARTESIAN_POINT('Ctrl Pts',(-30.6049981367031,55.817344072298,-2.));
#43351=CARTESIAN_POINT('Ctrl Pts',(-30.5939492528789,55.8498849658821,-2.));
#43352=CARTESIAN_POINT('Ctrl Pts',(-30.5877508307633,55.868140402147,-2.));
#43353=CARTESIAN_POINT('Ctrl Pts',(-30.5818018934048,55.8865028064712,-2.));
#43354=CARTESIAN_POINT('Ctrl Pts',(-30.576115080405,55.9049328084138,-2.));
#43355=CARTESIAN_POINT('Ctrl Pts',(-30.5540602837242,55.9764086852689,-2.));
#43356=CARTESIAN_POINT('Ctrl Pts',(-30.5359175198242,56.0489705581354,-2.));
#43357=CARTESIAN_POINT('Ctrl Pts',(-30.5217728584387,56.1222396610165,-2.));
#43358=CARTESIAN_POINT('Ctrl Pts',(-30.5111932477239,56.1770418626931,-2.));
#43359=CARTESIAN_POINT('Ctrl Pts',(-30.5028510892941,56.2322406204016,-2.));
#43360=CARTESIAN_POINT('Ctrl Pts',(-30.4967990447163,56.2876867713324,-2.));
#43361=CARTESIAN_POINT('Ctrl Pts',(-30.4949111210757,56.3049830912424,-2.));
#43362=CARTESIAN_POINT('Ctrl Pts',(-30.4932461646214,56.3223035269554,-2.));
#43363=CARTESIAN_POINT('Ctrl Pts',(-30.4918060890528,56.3396436454805,-2.));
#43364=CARTESIAN_POINT('Ctrl Pts',(-30.4904160490458,56.3563812799502,-2.));
#43365=CARTESIAN_POINT('Ctrl Pts',(-30.4892362965357,56.3731287080283,-2.));
#43366=CARTESIAN_POINT('Ctrl Pts',(-30.4882682431297,56.3898758527382,-2.));
#43367=CARTESIAN_POINT('Ctrl Pts',(-30.4839212193133,56.4650785600099,-2.));
#43368=CARTESIAN_POINT('Ctrl Pts',(-30.4838360419502,56.5403117892544,-2.));
#43369=CARTESIAN_POINT('Ctrl Pts',(-30.4881238107199,56.6152096419697,-2.));
#43370=CARTESIAN_POINT('Ctrl Pts',(-30.4914053519387,56.6725309211904,-2.));
#43371=CARTESIAN_POINT('Ctrl Pts',(-30.4972490710547,56.729656403295,-2.));
#43372=CARTESIAN_POINT('Ctrl Pts',(-30.5057249894129,56.7864264638425,-2.));
#43373=CARTESIAN_POINT('Ctrl Pts',(-30.5076920210892,56.799601261268,-2.));
#43374=CARTESIAN_POINT('Ctrl Pts',(-30.5098008972608,56.8127569211081,-2.));
#43375=CARTESIAN_POINT('Ctrl Pts',(-30.5120501580915,56.825892077386,-2.));
#43376=CARTESIAN_POINT('Ctrl Pts',(-33.3325354057627,57.7362457052863,-0.87148036339022));
#43377=CARTESIAN_POINT('Ctrl Pts',(-33.2590763562246,57.7795019958594,-0.877193940366678));
#43378=CARTESIAN_POINT('Ctrl Pts',(-33.1823540930372,57.8169005192734,-0.882907517343135));
#43379=CARTESIAN_POINT('Ctrl Pts',(-33.1030496903125,57.8476363980486,-0.888621094319593));
#43380=CARTESIAN_POINT('Ctrl Pts',(-32.5888520129845,58.0469231581002,-0.925667057842273));
#43381=CARTESIAN_POINT('Ctrl Pts',(-31.966100460501,57.9661104565053,-0.962713021364954));
#43382=CARTESIAN_POINT('Ctrl Pts',(-31.5197930553252,57.6421865224026,-0.999758984887635));
#43383=CARTESIAN_POINT('Ctrl Pts',(-31.0734856501493,57.3182625882999,-1.03680494841032));
#43384=CARTESIAN_POINT('Ctrl Pts',(-30.8036223922811,56.7512274216893,-1.073850911933));
#43385=CARTESIAN_POINT('Ctrl Pts',(-30.8337231720004,56.2005802421929,-1.11089687545568));
#43386=CARTESIAN_POINT('Ctrl Pts',(-30.8638239517197,55.6499330626964,-1.14794283897836));
#43387=CARTESIAN_POINT('Ctrl Pts',(-31.1938887690265,55.115673870314,-1.18498880250104));
#43388=CARTESIAN_POINT('Ctrl Pts',(-31.6728308546875,54.8423246209736,-1.22203476602372));
#43389=CARTESIAN_POINT('Ctrl Pts',(-32.1517729403484,54.5689753716332,-1.2590807295464));
#43390=CARTESIAN_POINT('Ctrl Pts',(-32.7795922943635,54.5565360653349,-1.29612669306908));
#43391=CARTESIAN_POINT('Ctrl Pts',(-33.2690250069387,54.8106693502475,-1.33317265659176));
#43392=CARTESIAN_POINT('Ctrl Pts',(-33.7584577195138,55.0648026351601,-1.37021862011444));
#43393=CARTESIAN_POINT('Ctrl Pts',(-34.1095037906491,55.5855085112837,-1.40726458363712));
#43394=CARTESIAN_POINT('Ctrl Pts',(-34.1613832117471,56.1345432465003,-1.4443105471598));
#43395=CARTESIAN_POINT('Ctrl Pts',(-34.2132626328451,56.6835779817169,-1.48135651068248));
#43396=CARTESIAN_POINT('Ctrl Pts',(-33.9659754039059,57.2609415760266,-1.51840247420516));
#43397=CARTESIAN_POINT('Ctrl Pts',(-33.5329364407288,57.6022802269071,-1.55544843772784));
#43398=CARTESIAN_POINT('Ctrl Pts',(-33.4704694600161,57.6515192024594,-1.56079241294864));
#43399=CARTESIAN_POINT('Ctrl Pts',(-33.4041372082081,57.6958467816506,-1.56613638816943));
#43400=CARTESIAN_POINT('Ctrl Pts',(-33.3347882996638,57.7351190113229,-1.57148036339022));
#43401=CARTESIAN_POINT('Ctrl Pts',(-31.045873711622,57.7433792852396,-2.));
#43402=CARTESIAN_POINT('Ctrl Pts',(-31.5286078227265,58.2269108712356,-1.96295403647732));
#43403=CARTESIAN_POINT('Ctrl Pts',(-33.0063987810959,58.6658791894418,-1.88886210943196));
#43404=CARTESIAN_POINT('Ctrl Pts',(-34.7728277550873,57.1516769644331,-1.77772421886392));
#43405=CARTESIAN_POINT('Ctrl Pts',(-34.4535014835806,54.8495668967864,-1.66658632829587));
#43406=CARTESIAN_POINT('Ctrl Pts',(-32.3487507516394,53.8677941230741,-1.55544843772783));
#43407=CARTESIAN_POINT('Ctrl Pts',(-30.3811218874153,55.1044118987673,-1.44431054715979));
#43408=CARTESIAN_POINT('Ctrl Pts',(-30.3535878576005,57.4278205885651,-1.33317265659175));
#43409=CARTESIAN_POINT('Ctrl Pts',(-32.2903568834191,58.7112317202032,-1.22203476602371));
#43410=CARTESIAN_POINT('Ctrl Pts',(-34.4191815551847,57.7799979545239,-1.11089687545567));
#43411=CARTESIAN_POINT('Ctrl Pts',(-34.7912737376158,55.4864512354733,-0.999758984887624));
#43412=CARTESIAN_POINT('Ctrl Pts',(-33.0661792001092,53.929919412126,-0.888621094319583));
#43413=CARTESIAN_POINT('Ctrl Pts',(-30.822833264184,54.5351044086333,-0.77748320375154));
#43414=CARTESIAN_POINT('Ctrl Pts',(-30.114627688562,56.7480782089187,-0.666345313183499));
#43415=CARTESIAN_POINT('Ctrl Pts',(-31.5897751037144,58.543278448718,-0.555207422615458));
#43416=CARTESIAN_POINT('Ctrl Pts',(-33.8980643703311,58.2775391690227,-0.444069532047415));
#43417=CARTESIAN_POINT('Ctrl Pts',(-34.926688116847,56.1940939537868,-0.332931641479374));
#43418=CARTESIAN_POINT('Ctrl Pts',(-33.7341373860101,54.1999441339785,-0.221793750911332));
#43419=CARTESIAN_POINT('Ctrl Pts',(-31.4119663698709,54.1203575053851,-0.110655860343291));
#43420=CARTESIAN_POINT('Ctrl Pts',(-30.0856850452223,56.0281806868171,0.000482030224751779));
#43421=CARTESIAN_POINT('Ctrl Pts',(-30.9692534931352,58.1771614464074,0.111619920792793));
#43422=CARTESIAN_POINT('Ctrl Pts',(-33.2539316216956,58.6003133427487,0.222757811360835));
#43423=CARTESIAN_POINT('Ctrl Pts',(-34.8485275651184,56.9103206367346,0.333895701928877));
#43424=CARTESIAN_POINT('Ctrl Pts',(-34.2934896049409,54.6540528227808,0.445033592496919));
#43425=CARTESIAN_POINT('Ctrl Pts',(-32.0968502643471,53.8966974164155,0.55617148306496));
#43426=CARTESIAN_POINT('Ctrl Pts',(-30.2692184515671,55.3314704112852,0.667309373633001));
#43427=CARTESIAN_POINT('Ctrl Pts',(-30.4834462874739,57.6451078131478,0.778447264201044));
#43428=CARTESIAN_POINT('Ctrl Pts',(-32.5434486064222,58.7199110699496,0.889585154769085));
#43429=CARTESIAN_POINT('Ctrl Pts',(-34.563681922824,57.5721005714895,1.00072304533713));
#43430=CARTESIAN_POINT('Ctrl Pts',(-34.6950037716947,55.2522802841409,1.11186093590517));
#43431=CARTESIAN_POINT('Ctrl Pts',(-32.8172137752098,53.883808025427,1.22299882647321));
#43432=CARTESIAN_POINT('Ctrl Pts',(-30.6490744128705,54.7192619732989,1.33413671704125));
#43433=CARTESIAN_POINT('Ctrl Pts',(-30.1751082313325,56.9939416545675,1.44527460760929));
#43434=CARTESIAN_POINT('Ctrl Pts',(-31.8291418517329,58.6258069603505,1.55641249817734));
#43435=CARTESIAN_POINT('Ctrl Pts',(-34.0972195432855,58.1211930696509,1.66755038874538));
#43436=CARTESIAN_POINT('Ctrl Pts',(-34.90334407317,55.9419787993381,1.77868827931342));
#43437=CARTESIAN_POINT('Ctrl Pts',(-33.5096605171051,54.0828236849994,1.88982616988146));
#43438=CARTESIAN_POINT('Ctrl Pts',(-31.1918232394055,54.2454334870425,2.0009640604495));
#43439=CARTESIAN_POINT('Ctrl Pts',(-30.0713749864112,56.2809696095364,2.11210195101755));
#43440=CARTESIAN_POINT('Ctrl Pts',(-31.1738747508359,58.326282755013,2.22323984158559));
#43441=CARTESIAN_POINT('Ctrl Pts',(-33.4901919951035,58.5092746059888,2.33437773215363));
#43442=CARTESIAN_POINT('Ctrl Pts',(-34.900175276712,56.6624506459969,2.44551562272167));
#43443=CARTESIAN_POINT('Ctrl Pts',(-34.113250907707,54.4762297900261,2.55665351328971));
#43444=CARTESIAN_POINT('Ctrl Pts',(-31.8496996873681,53.9516847809774,2.66779140385775));
#43445=CARTESIAN_POINT('Ctrl Pts',(-30.1813757180884,55.5689376143778,2.7789292944258));
#43446=CARTESIAN_POINT('Ctrl Pts',(-30.6353148490301,57.8476984309217,2.89006718499383));
#43447=CARTESIAN_POINT('Ctrl Pts',(-32.7960214456225,58.7021916123208,3.00120507556188));
#43448=CARTESIAN_POINT('Ctrl Pts',(-34.6857762559251,57.350289859029,3.11234296612992));
#43449=CARTESIAN_POINT('Ctrl Pts',(-34.5748652707907,55.0294041774427,3.22348085669796));
#43450=CARTESIAN_POINT('Ctrl Pts',(-32.5648065727292,53.8638675525518,3.334618747266));
#43451=CARTESIAN_POINT('Ctrl Pts',(-30.4954296836916,54.9205088752031,3.44575663783405));
#43452=CARTESIAN_POINT('Ctrl Pts',(-30.2608587385459,57.2321723596468,3.55689452840209));
#43453=CARTESIAN_POINT('Ctrl Pts',(-32.0757991835955,58.6829662025232,3.66803241897013));
#43454=CARTESIAN_POINT('Ctrl Pts',(-34.2790154466699,57.9449623463291,3.77917030953817));
#43455=CARTESIAN_POINT('Ctrl Pts',(-34.8538786959893,55.6936640901667,3.89030820010621));
#43456=CARTESIAN_POINT('Ctrl Pts',(-33.2742100800909,53.9897102593704,4.00144609067426));
#43457=CARTESIAN_POINT('Ctrl Pts',(-30.9858981977034,54.3927491193984,4.1125839812423));
#43458=CARTESIAN_POINT('Ctrl Pts',(-30.0834608661247,56.5338746309361,4.22372187181034));
#43459=CARTESIAN_POINT('Ctrl Pts',(-31.3929092090317,58.4532903311776,4.33485976237838));
#43460=CARTESIAN_POINT('Ctrl Pts',(-33.7156903085101,58.3941332621978,4.44599765294642));
#43461=CARTESIAN_POINT('Ctrl Pts',(-34.9257362810773,56.410550559801,4.55713554351447));
#43462=CARTESIAN_POINT('Ctrl Pts',(-33.91547832718,54.3181379674856,4.6682734340825));
#43463=CARTESIAN_POINT('Ctrl Pts',(-31.6096170051591,54.0321044593028,4.77941132465055));
#43464=CARTESIAN_POINT('Ctrl Pts',(-30.1187333412011,55.8142597516568,4.89054921521859));
#43465=CARTESIAN_POINT('Ctrl Pts',(-30.8074500449804,58.033376889416,5.00168710578664));
#43466=CARTESIAN_POINT('Ctrl Pts',(-33.045376938239,58.6582727998918,5.11282499635467));
#43467=CARTESIAN_POINT('Ctrl Pts',(-34.7841140934679,57.1169731495112,5.22396288692271));
#43468=CARTESIAN_POINT('Ctrl Pts',(-34.4321757978777,54.8202470274371,5.33510077749076));
#43469=CARTESIAN_POINT('Ctrl Pts',(-32.3116949177892,53.8703138209288,5.44623866805879));
#43470=CARTESIAN_POINT('Ctrl Pts',(-30.3635721421369,55.1366583239951,5.55737655862684));
#43471=CARTESIAN_POINT('Ctrl Pts',(-30.3709453622051,57.4601807388668,5.66851444919488));
#43472=CARTESIAN_POINT('Ctrl Pts',(-32.3270677340268,58.7141352713796,5.77965233976292));
#43473=CARTESIAN_POINT('Ctrl Pts',(-34.4414743886772,57.7507618774264,5.89079023033096));
#43474=CARTESIAN_POINT('Ctrl Pts',(-34.7788326566387,55.451849617872,6.00192812089901));
#43475=CARTESIAN_POINT('Ctrl Pts',(-33.0303393193103,53.921614042038,6.11306601146705));
#43476=CARTESIAN_POINT('Ctrl Pts',(-30.79644075645,54.5607069079647,6.22420390203509));
#43477=CARTESIAN_POINT('Ctrl Pts',(-30.1217887402557,56.7841397946825,6.33534179260313));
#43478=CARTESIAN_POINT('Ctrl Pts',(-31.6240211855661,58.5568181325983,6.44647968317118));
#43479=CARTESIAN_POINT('Ctrl Pts',(-33.9278862659328,58.2561121571831,6.55761757373921));
#43480=CARTESIAN_POINT('Ctrl Pts',(-34.9251107981772,56.1574151102239,6.66875546430726));
#43481=CARTESIAN_POINT('Ctrl Pts',(-33.7019669024841,54.1813822458926,6.77989335487529));
#43482=CARTESIAN_POINT('Ctrl Pts',(-31.3799180340502,54.137308723055,6.89103124544334));
#43483=CARTESIAN_POINT('Ctrl Pts',(-30.0805564955409,56.0643114795338,7.00216913601138));
#43484=CARTESIAN_POINT('Ctrl Pts',(-31.0009129766989,58.2011370798035,7.11330702657943));
#43485=CARTESIAN_POINT('Ctrl Pts',(-32.5211546805143,58.4569191413474,7.18739895362479));
#43486=CARTESIAN_POINT('Ctrl Pts',(-33.1673657555108,58.2350041503452,7.22444491714747));
#43487=CARTESIAN_POINT('Ctrl Pts',(-31.137578557241,57.6518256858141,-2.07481497238249));
#43488=CARTESIAN_POINT('Ctrl Pts',(-31.5898689183853,58.1048632288922,-2.03776900885981));
#43489=CARTESIAN_POINT('Ctrl Pts',(-32.9744626126811,58.5161478980409,-1.96367708181445));
#43490=CARTESIAN_POINT('Ctrl Pts',(-34.6294912924535,57.0974392229325,-1.85253919124641));
#43491=CARTESIAN_POINT('Ctrl Pts',(-34.3303034137843,54.9405123144369,-1.74140130067836));
#43492=CARTESIAN_POINT('Ctrl Pts',(-32.3582893241016,54.0206552913481,-1.63026341011032));
#43493=CARTESIAN_POINT('Ctrl Pts',(-30.5147494765409,55.1792854513053,-1.51912551954228));
#43494=CARTESIAN_POINT('Ctrl Pts',(-30.4889518873458,57.3561677789083,-1.40798762897424));
#43495=CARTESIAN_POINT('Ctrl Pts',(-32.3035780800888,58.5586402598713,-1.2968497384062));
#43496=CARTESIAN_POINT('Ctrl Pts',(-34.2981478804346,57.686134989371,-1.18571184783815));
#43497=CARTESIAN_POINT('Ctrl Pts',(-34.6467739743846,55.5372313797062,-1.07457395727011));
#43498=CARTESIAN_POINT('Ctrl Pts',(-33.0304729643072,54.0788626331852,-0.963436066702071));
#43499=CARTESIAN_POINT('Ctrl Pts',(-30.9286042125635,54.6458814833823,-0.852298176134029));
#43500=CARTESIAN_POINT('Ctrl Pts',(-30.2650618023749,56.7192935259745,-0.741160285565988));
#43501=CARTESIAN_POINT('Ctrl Pts',(-31.6471786691816,58.4012790043313,-0.630022394997946));
#43502=CARTESIAN_POINT('Ctrl Pts',(-33.8098950838865,58.1522986401539,-0.518884504429904));
#43503=CARTESIAN_POINT('Ctrl Pts',(-34.7736484112179,56.2002464293262,-0.407746613861863));
#43504=CARTESIAN_POINT('Ctrl Pts',(-33.6563061966827,54.331858177016,-0.296608723293821));
#43505=CARTESIAN_POINT('Ctrl Pts',(-31.480583488533,54.2572906994736,-0.185470832725779));
#43506=CARTESIAN_POINT('Ctrl Pts',(-30.2379444342266,56.044796524896,-0.0743329421577371));
#43507=CARTESIAN_POINT('Ctrl Pts',(-31.0657904123945,58.0582512642421,0.0368049484103043));
#43508=CARTESIAN_POINT('Ctrl Pts',(-33.2063847314925,58.4547169782087,0.147942838978346));
#43509=CARTESIAN_POINT('Ctrl Pts',(-34.7004170746387,56.8713040936592,0.259080729546388));
#43510=CARTESIAN_POINT('Ctrl Pts',(-34.1803827251225,54.7573283854237,0.37021862011443));
#43511=CARTESIAN_POINT('Ctrl Pts',(-32.1222750053513,54.0477357911158,0.481356510682471));
#43512=CARTESIAN_POINT('Ctrl Pts',(-30.4099032594437,55.3920244607626,0.592494401250513));
#43513=CARTESIAN_POINT('Ctrl Pts',(-30.6106207621861,57.5597517291987,0.703632291818555));
#43514=CARTESIAN_POINT('Ctrl Pts',(-32.5407085089656,58.5667722442101,0.814770182386597));
#43515=CARTESIAN_POINT('Ctrl Pts',(-34.4335352954974,57.4913487078745,0.925908072954637));
#43516=CARTESIAN_POINT('Ctrl Pts',(-34.5565752984423,55.3178284792041,1.03704596352268));
#43517=CARTESIAN_POINT('Ctrl Pts',(-32.7972086074906,54.0356592728607,1.14818385409072));
#43518=CARTESIAN_POINT('Ctrl Pts',(-30.7658035075692,54.8184251042164,1.25932174465876));
#43519=CARTESIAN_POINT('Ctrl Pts',(-30.3217281242748,56.9496515306538,1.3704596352268));
#43520=CARTESIAN_POINT('Ctrl Pts',(-31.8714496921254,58.4786028343079,1.48159752579485));
#43521=CARTESIAN_POINT('Ctrl Pts',(-33.9964904850136,58.0058125474546,1.59273541636289));
#43522=CARTESIAN_POINT('Ctrl Pts',(-34.7517765656152,55.9640309814584,1.70387330693093));
#43523=CARTESIAN_POINT('Ctrl Pts',(-33.4459860188247,54.222123959053,1.81501119749897));
#43524=CARTESIAN_POINT('Ctrl Pts',(-31.2743237407936,54.3744787324154,1.92614908806701));
#43525=CARTESIAN_POINT('Ctrl Pts',(-30.2245368429279,56.2816432496664,2.03728697863506));
#43526=CARTESIAN_POINT('Ctrl Pts',(-31.2575071782378,58.1979681994493,2.1484248692031));
#43527=CARTESIAN_POINT('Ctrl Pts',(-33.4277452841336,58.3694196226251,2.25956275977114));
#43528=CARTESIAN_POINT('Ctrl Pts',(-34.7488076101148,56.6390660871692,2.37070065033918));
#43529=CARTESIAN_POINT('Ctrl Pts',(-34.0115108273451,54.5907198076286,2.48183854090722));
#43530=CARTESIAN_POINT('Ctrl Pts',(-31.8907110426077,54.0992553634931,2.59297643147526));
#43531=CARTESIAN_POINT('Ctrl Pts',(-30.3276003503783,55.6145157340662,2.70411432204331));
#43532=CARTESIAN_POINT('Ctrl Pts',(-30.7529116941353,57.7495659179407,2.81525221261135));
#43533=CARTESIAN_POINT('Ctrl Pts',(-32.7773527775792,58.5501702687005,2.92639010317939));
#43534=CARTESIAN_POINT('Ctrl Pts',(-34.5479297183105,57.2835265446242,3.03752799374743));
#43535=CARTESIAN_POINT('Ctrl Pts',(-34.4440133627694,55.1090081110757,3.14866588431548));
#43536=CARTESIAN_POINT('Ctrl Pts',(-32.5607195296748,54.0169763509983,3.25980377488351));
#43537=CARTESIAN_POINT('Ctrl Pts',(-30.6218484224619,55.0069803188732,3.37094166545156));
#43538=CARTESIAN_POINT('Ctrl Pts',(-30.4020707538584,57.1728581554962,3.4820795560196));
#43539=CARTESIAN_POINT('Ctrl Pts',(-32.1025515163817,58.5321573142801,3.59321744658764));
#43540=CARTESIAN_POINT('Ctrl Pts',(-34.1668213833381,57.8406958596912,3.70435533715568));
#43541=CARTESIAN_POINT('Ctrl Pts',(-34.705430735075,55.7313763028164,3.81549322772372));
#43542=CARTESIAN_POINT('Ctrl Pts',(-33.225384323732,54.1348827553833,3.92663111829177));
#43543=CARTESIAN_POINT('Ctrl Pts',(-31.0813854144196,54.5125038668068,4.0377690088598));
#43544=CARTESIAN_POINT('Ctrl Pts',(-30.2358605235516,56.5185987513241,4.14890689942785));
#43545=CARTESIAN_POINT('Ctrl Pts',(-31.4627281724074,58.3169660103977,4.26004478999589));
#43546=CARTESIAN_POINT('Ctrl Pts',(-33.6390224888348,58.2615396970761,4.37118268056393));
#43547=CARTESIAN_POINT('Ctrl Pts',(-34.772756603214,56.4030521442201,4.48232057113198));
#43548=CARTESIAN_POINT('Ctrl Pts',(-33.8262108251009,54.4425980862377,4.59345846170001));
#43549=CARTESIAN_POINT('Ctrl Pts',(-31.6657692360459,54.1746033542736,4.70459635226806));
#43550=CARTESIAN_POINT('Ctrl Pts',(-30.2689085309823,55.8443665681263,4.8157342428361));
#43551=CARTESIAN_POINT('Ctrl Pts',(-30.9141911400064,57.9235345170459,4.92687213340414));
#43552=CARTESIAN_POINT('Ctrl Pts',(-33.0109826023927,58.5090212073898,5.03801002397218));
#43553=CARTESIAN_POINT('Ctrl Pts',(-34.6400658550227,57.0649240129586,5.14914791454022));
#43554=CARTESIAN_POINT('Ctrl Pts',(-34.3103226378947,54.9130415101336,5.26028580510827));
#43555=CARTESIAN_POINT('Ctrl Pts',(-32.3235704258736,54.0230160838143,5.3714236956763));
#43556=CARTESIAN_POINT('Ctrl Pts',(-30.498306510429,55.2094982474935,5.48256158624435));
#43557=CARTESIAN_POINT('Ctrl Pts',(-30.5052147364911,57.3864871280696,5.59369947681239));
#43558=CARTESIAN_POINT('Ctrl Pts',(-32.3379737515306,58.5613606978515,5.70483736738044));
#43559=CARTESIAN_POINT('Ctrl Pts',(-34.3190348106915,57.6587426929398,5.81597525794847));
#43560=CARTESIAN_POINT('Ctrl Pts',(-34.6351174933556,55.5048119219529,5.92711314851652));
#43561=CARTESIAN_POINT('Ctrl Pts',(-32.9968933347409,54.0710810433821,6.03825103908456));
#43562=CARTESIAN_POINT('Ctrl Pts',(-30.9038761550678,54.669869354557,6.1493889296526));
#43563=CARTESIAN_POINT('Ctrl Pts',(-30.2717712405154,56.7530808786254,6.26052682022064));
#43564=CARTESIAN_POINT('Ctrl Pts',(-31.6792650131382,58.413964804591,6.37166471078869));
#43565=CARTESIAN_POINT('Ctrl Pts',(-33.8378362540284,58.1322229282863,6.48280260135671));
#43566=CARTESIAN_POINT('Ctrl Pts',(-34.7721705665527,56.1658807463967,6.59394049192478));
#43567=CARTESIAN_POINT('Ctrl Pts',(-33.6261645529135,54.3144668991412,6.70507838249281));
#43568=CARTESIAN_POINT('Ctrl Pts',(-31.4505562891928,54.2731728842734,6.81621627306085));
#43569=CARTESIAN_POINT('Ctrl Pts',(-30.2331393178402,56.0786487199457,6.92735416362889));
#43570=CARTESIAN_POINT('Ctrl Pts',(-31.0954532825444,58.0807148681969,7.03849205419693));
#43571=CARTESIAN_POINT('Ctrl Pts',(-32.5198205551868,58.3203659687277,7.1125839812423));
#43572=CARTESIAN_POINT('Ctrl Pts',(-33.1252781637592,58.1124461032886,7.14962994476498));
#43573=CARTESIAN_POINT('Ctrl Pts',(-31.22928340286,57.5602720863885,-2.14962994476498));
#43574=CARTESIAN_POINT('Ctrl Pts',(-31.6511300140442,57.9828155865489,-2.1125839812423));
#43575=CARTESIAN_POINT('Ctrl Pts',(-32.9425264442663,58.3664166066401,-2.03849205419693));
#43576=CARTESIAN_POINT('Ctrl Pts',(-34.4861548298197,57.0432014814318,-1.9273541636289));
#43577=CARTESIAN_POINT('Ctrl Pts',(-34.207105343988,55.0314577320876,-1.81621627306085));
#43578=CARTESIAN_POINT('Ctrl Pts',(-32.3678278965638,54.1735164596221,-1.70507838249281));
#43579=CARTESIAN_POINT('Ctrl Pts',(-30.6483770656664,55.2541590038433,-1.59394049192477));
#43580=CARTESIAN_POINT('Ctrl Pts',(-30.6243159170911,57.2845149692516,-1.48280260135673));
#43581=CARTESIAN_POINT('Ctrl Pts',(-32.3167992767584,58.4060487995394,-1.37166471078869));
#43582=CARTESIAN_POINT('Ctrl Pts',(-34.1771142056845,57.5922720242182,-1.26052682022064));
#43583=CARTESIAN_POINT('Ctrl Pts',(-34.5022742111534,55.5880115239391,-1.1493889296526));
#43584=CARTESIAN_POINT('Ctrl Pts',(-32.9947667285052,54.2278058542443,-1.03825103908456));
#43585=CARTESIAN_POINT('Ctrl Pts',(-31.034375160943,54.7566585581314,-0.927113148516518));
#43586=CARTESIAN_POINT('Ctrl Pts',(-30.4154959161879,56.6905088430302,-0.815975257948476));
#43587=CARTESIAN_POINT('Ctrl Pts',(-31.7045822346488,58.2592795599445,-0.704837367380436));
#43588=CARTESIAN_POINT('Ctrl Pts',(-33.7217257974419,58.0270581112851,-0.593699476812393));
#43589=CARTESIAN_POINT('Ctrl Pts',(-34.6206087055888,56.2063989048655,-0.482561586244352));
#43590=CARTESIAN_POINT('Ctrl Pts',(-33.5784750073553,54.4637722200535,-0.37142369567631));
#43591=CARTESIAN_POINT('Ctrl Pts',(-31.5492006071951,54.394223893562,-0.260285805108268));
#43592=CARTESIAN_POINT('Ctrl Pts',(-30.3902038232309,56.0614123629749,-0.149147914540226));
#43593=CARTESIAN_POINT('Ctrl Pts',(-31.1623273316537,57.9393410820767,-0.0380100239721846));
#43594=CARTESIAN_POINT('Ctrl Pts',(-33.1588378412895,58.3091206136687,0.0731278665958569));
#43595=CARTESIAN_POINT('Ctrl Pts',(-34.5523065841589,56.8322875505838,0.184265757163899));
#43596=CARTESIAN_POINT('Ctrl Pts',(-34.067275845304,54.8606039480668,0.295403647731941));
#43597=CARTESIAN_POINT('Ctrl Pts',(-32.1476997463555,54.1987741658161,0.406541538299982));
#43598=CARTESIAN_POINT('Ctrl Pts',(-30.5505880673203,55.45257851024,0.517679428868024));
#43599=CARTESIAN_POINT('Ctrl Pts',(-30.7377952368983,57.4743956452495,0.628817319436066));
#43600=CARTESIAN_POINT('Ctrl Pts',(-32.5379684115091,58.4136334184706,0.739955210004107));
#43601=CARTESIAN_POINT('Ctrl Pts',(-34.3033886681708,57.4105968442595,0.85109310057215));
#43602=CARTESIAN_POINT('Ctrl Pts',(-34.4181468251899,55.3833766742673,0.962230991140191));
#43603=CARTESIAN_POINT('Ctrl Pts',(-32.7772034397714,54.1875105202944,1.07336888170823));
#43604=CARTESIAN_POINT('Ctrl Pts',(-30.8825326022679,54.9175882351338,1.18450677227627));
#43605=CARTESIAN_POINT('Ctrl Pts',(-30.4683480172171,56.9053614067402,1.29564466284432));
#43606=CARTESIAN_POINT('Ctrl Pts',(-31.9137575325177,58.3313987082652,1.40678255341236));
#43607=CARTESIAN_POINT('Ctrl Pts',(-33.8957614267418,57.8904320252583,1.5179204439804));
#43608=CARTESIAN_POINT('Ctrl Pts',(-34.6002090580604,55.9860831635788,1.62905833454844));
#43609=CARTESIAN_POINT('Ctrl Pts',(-33.3823115205443,54.3614242331065,1.74019622511648));
#43610=CARTESIAN_POINT('Ctrl Pts',(-31.3568242421816,54.5035239777884,1.85133411568453));
#43611=CARTESIAN_POINT('Ctrl Pts',(-30.3776986994445,56.2823168897962,1.96247200625257));
#43612=CARTESIAN_POINT('Ctrl Pts',(-31.3411396056398,58.0696536438857,2.07360989682061));
#43613=CARTESIAN_POINT('Ctrl Pts',(-33.3652985731636,58.2295646392612,2.18474778738865));
#43614=CARTESIAN_POINT('Ctrl Pts',(-34.5974399435175,56.6156815283416,2.29588567795669));
#43615=CARTESIAN_POINT('Ctrl Pts',(-33.9097707469831,54.7052098252308,2.40702356852473));
#43616=CARTESIAN_POINT('Ctrl Pts',(-31.9317223978473,54.246825946009,2.51816145909278));
#43617=CARTESIAN_POINT('Ctrl Pts',(-30.4738249826682,55.6600938537544,2.62929934966082));
#43618=CARTESIAN_POINT('Ctrl Pts',(-30.8705085392404,57.6514334049598,2.74043724022886));
#43619=CARTESIAN_POINT('Ctrl Pts',(-32.7586841095359,58.3981489250801,2.8515751307969));
#43620=CARTESIAN_POINT('Ctrl Pts',(-34.4100831806959,57.2167632302195,2.96271302136494));
#43621=CARTESIAN_POINT('Ctrl Pts',(-34.3131614547482,55.1886120447087,3.07385091193299));
#43622=CARTESIAN_POINT('Ctrl Pts',(-32.5566324866203,54.1700851494448,3.18498880250102));
#43623=CARTESIAN_POINT('Ctrl Pts',(-30.7482671612322,55.0934517625431,3.29612669306907));
#43624=CARTESIAN_POINT('Ctrl Pts',(-30.543282769171,57.1135439513457,3.40726458363711));
#43625=CARTESIAN_POINT('Ctrl Pts',(-32.1293038491678,58.381348426037,3.51840247420515));
#43626=CARTESIAN_POINT('Ctrl Pts',(-34.0546273200064,57.7364293730534,3.6295403647732));
#43627=CARTESIAN_POINT('Ctrl Pts',(-34.5569827741607,55.769088515466,3.74067825534123));
#43628=CARTESIAN_POINT('Ctrl Pts',(-33.1765585673731,54.2800552513962,3.85181614590928));
#43629=CARTESIAN_POINT('Ctrl Pts',(-31.1768726311358,54.6322586142151,3.96295403647732));
#43630=CARTESIAN_POINT('Ctrl Pts',(-30.3882601809786,56.5033228717121,4.07409192704536));
#43631=CARTESIAN_POINT('Ctrl Pts',(-31.5325471357832,58.1806416896178,4.1852298176134));
#43632=CARTESIAN_POINT('Ctrl Pts',(-33.5623546691595,58.1289461319544,4.29636770818144));
#43633=CARTESIAN_POINT('Ctrl Pts',(-34.6197769253507,56.3955537286392,4.40750559874949));
#43634=CARTESIAN_POINT('Ctrl Pts',(-33.7369433230218,54.5670582049899,4.51864348931753));
#43635=CARTESIAN_POINT('Ctrl Pts',(-31.7219214669328,54.3171022492445,4.62978137988557));
#43636=CARTESIAN_POINT('Ctrl Pts',(-30.4190837207633,55.8744733845956,4.74091927045361));
#43637=CARTESIAN_POINT('Ctrl Pts',(-31.0209322350324,57.8136921446758,4.85205716102165));
#43638=CARTESIAN_POINT('Ctrl Pts',(-32.9765882665465,58.359769614888,4.9631950515897));
#43639=CARTESIAN_POINT('Ctrl Pts',(-34.4960176165775,57.0128748764059,5.07433294215773));
#43640=CARTESIAN_POINT('Ctrl Pts',(-34.1884694779118,55.0058359928301,5.18547083272579));
#43641=CARTESIAN_POINT('Ctrl Pts',(-32.335445933958,54.1757183466999,5.29660872329381));
#43642=CARTESIAN_POINT('Ctrl Pts',(-30.6330408787211,55.2823381709918,5.40774661386187));
#43643=CARTESIAN_POINT('Ctrl Pts',(-30.6394841107772,57.3127935172725,5.51888450442989));
#43644=CARTESIAN_POINT('Ctrl Pts',(-32.3488797690342,58.4085861243233,5.63002239499795));
#43645=CARTESIAN_POINT('Ctrl Pts',(-34.1965952327058,57.5667235084533,5.74116028556598));
#43646=CARTESIAN_POINT('Ctrl Pts',(-34.4914023300724,55.5577742260337,5.85229817613403));
#43647=CARTESIAN_POINT('Ctrl Pts',(-32.9634473501715,54.2205480447262,5.96343606670206));
#43648=CARTESIAN_POINT('Ctrl Pts',(-31.0113115536856,54.7790318011494,6.07457395727011));
#43649=CARTESIAN_POINT('Ctrl Pts',(-30.4217537407751,56.7220219625683,6.18571184783815));
#43650=CARTESIAN_POINT('Ctrl Pts',(-31.7345088407103,58.2711114765837,6.29684973840619));
#43651=CARTESIAN_POINT('Ctrl Pts',(-33.7477862421241,58.0083336993895,6.40798762897424));
#43652=CARTESIAN_POINT('Ctrl Pts',(-34.6192303349282,56.1743463825696,6.51912551954228));
#43653=CARTESIAN_POINT('Ctrl Pts',(-33.5503622033428,54.4475515523897,6.63026341011032));
#43654=CARTESIAN_POINT('Ctrl Pts',(-31.5211945443355,54.4090370454918,6.74140130067836));
#43655=CARTESIAN_POINT('Ctrl Pts',(-30.3857221401394,56.0929859603577,6.8525391912464));
#43656=CARTESIAN_POINT('Ctrl Pts',(-31.18999358839,57.9602926565904,6.96367708181445));
#43657=CARTESIAN_POINT('Ctrl Pts',(-32.5184864298593,58.1838127961081,7.03776900885981));
#43658=CARTESIAN_POINT('Ctrl Pts',(-33.0831905720076,57.989888056232,7.07481497238249));
#43659=CARTESIAN_POINT('Ctrl Pts',(-31.320988248479,57.468718486963,-2.22444491714747));
#43660=CARTESIAN_POINT('Ctrl Pts',(-31.712391109703,57.8607679442056,-2.18739895362479));
#43661=CARTESIAN_POINT('Ctrl Pts',(-32.9105902758514,58.2166853152393,-2.11330702657943));
#43662=CARTESIAN_POINT('Ctrl Pts',(-34.342818367186,56.9889637399312,-2.00216913601138));
#43663=CARTESIAN_POINT('Ctrl Pts',(-34.0839072741916,55.122403149738,-1.89103124544334));
#43664=CARTESIAN_POINT('Ctrl Pts',(-32.377366469026,54.3263776278961,-1.7798933548753));
#43665=CARTESIAN_POINT('Ctrl Pts',(-30.782004654792,55.3290325563813,-1.66875546430726));
#43666=CARTESIAN_POINT('Ctrl Pts',(-30.7596799468365,57.2128621595948,-1.55761757373922));
#43667=CARTESIAN_POINT('Ctrl Pts',(-32.330020473428,58.2534573392075,-1.44647968317117));
#43668=CARTESIAN_POINT('Ctrl Pts',(-34.0560805309345,57.4984090590654,-1.33534179260313));
#43669=CARTESIAN_POINT('Ctrl Pts',(-34.3577744479221,55.6387916681721,-1.22420390203509));
#43670=CARTESIAN_POINT('Ctrl Pts',(-32.9590604927032,54.3767490753035,-1.11306601146705));
#43671=CARTESIAN_POINT('Ctrl Pts',(-31.1401461093226,54.8674356328804,-1.00192812089901));
#43672=CARTESIAN_POINT('Ctrl Pts',(-30.5659300300008,56.6617241600859,-0.890790230330966));
#43673=CARTESIAN_POINT('Ctrl Pts',(-31.761985800116,58.1172801155577,-0.779652339762924));
#43674=CARTESIAN_POINT('Ctrl Pts',(-33.6335565109972,57.9018175824163,-0.668514449194882));
#43675=CARTESIAN_POINT('Ctrl Pts',(-34.4675689999597,56.2125513804048,-0.557376558626841));
#43676=CARTESIAN_POINT('Ctrl Pts',(-33.5006438180279,54.595686263091,-0.446238668058798));
#43677=CARTESIAN_POINT('Ctrl Pts',(-31.6178177258571,54.5311570876504,-0.335100777490758));
#43678=CARTESIAN_POINT('Ctrl Pts',(-30.5424632122353,56.0780282010538,-0.223962886922715));
#43679=CARTESIAN_POINT('Ctrl Pts',(-31.2588642509129,57.8204308999113,-0.112824996354674));
#43680=CARTESIAN_POINT('Ctrl Pts',(-33.1112909510864,58.1635242491288,-0.00168710578663204));
#43681=CARTESIAN_POINT('Ctrl Pts',(-34.4041960936792,56.7932710075084,0.10945078478141));
#43682=CARTESIAN_POINT('Ctrl Pts',(-33.9541689654856,54.9638795107097,0.220588675349452));
#43683=CARTESIAN_POINT('Ctrl Pts',(-32.1731244873597,54.3498125405165,0.331726565917494));
#43684=CARTESIAN_POINT('Ctrl Pts',(-30.6912728751969,55.5131325597174,0.442864456485535));
#43685=CARTESIAN_POINT('Ctrl Pts',(-30.8649697116105,57.3890395613005,0.554002347053577));
#43686=CARTESIAN_POINT('Ctrl Pts',(-32.5352283140525,58.260494592731,0.665140237621618));
#43687=CARTESIAN_POINT('Ctrl Pts',(-34.1732420408443,57.3298449806446,0.776278128189661));
#43688=CARTESIAN_POINT('Ctrl Pts',(-34.2797183519374,55.4489248693305,0.887416018757701));
#43689=CARTESIAN_POINT('Ctrl Pts',(-32.7571982720523,54.3393617677281,0.998553909325745));
#43690=CARTESIAN_POINT('Ctrl Pts',(-30.9992616969666,55.0167513660514,1.10969179989379));
#43691=CARTESIAN_POINT('Ctrl Pts',(-30.6149679101594,56.8610712828264,1.22082969046183));
#43692=CARTESIAN_POINT('Ctrl Pts',(-31.9560653729101,58.1841945822227,1.33196758102987));
#43693=CARTESIAN_POINT('Ctrl Pts',(-33.7950323684699,57.7750515030619,1.44310547159791));
#43694=CARTESIAN_POINT('Ctrl Pts',(-34.4486415505055,56.0081353456992,1.55424336216596));
#43695=CARTESIAN_POINT('Ctrl Pts',(-33.318637022264,54.5007245071601,1.66538125273399));
#43696=CARTESIAN_POINT('Ctrl Pts',(-31.4393247435696,54.6325692231613,1.77651914330204));
#43697=CARTESIAN_POINT('Ctrl Pts',(-30.5308605559611,56.2829905299262,1.88765703387008));
#43698=CARTESIAN_POINT('Ctrl Pts',(-31.4247720330417,57.941339088322,1.99879492443812));
#43699=CARTESIAN_POINT('Ctrl Pts',(-33.3028518621937,58.0897096558975,2.10993281500616));
#43700=CARTESIAN_POINT('Ctrl Pts',(-34.4460722769204,56.592296969514,2.2210707055742));
#43701=CARTESIAN_POINT('Ctrl Pts',(-33.8080306666211,54.8196998428332,2.33220859614224));
#43702=CARTESIAN_POINT('Ctrl Pts',(-31.9727337530869,54.3943965285248,2.44334648671029));
#43703=CARTESIAN_POINT('Ctrl Pts',(-30.6200496149581,55.7056719734427,2.55448437727833));
#43704=CARTESIAN_POINT('Ctrl Pts',(-30.9881053843456,57.5533008919789,2.66562226784637));
#43705=CARTESIAN_POINT('Ctrl Pts',(-32.7400154414926,58.2461275814598,2.77676015841441));
#43706=CARTESIAN_POINT('Ctrl Pts',(-34.2722366430812,57.1499999158148,2.88789804898245));
#43707=CARTESIAN_POINT('Ctrl Pts',(-34.182309546727,55.2682159783416,2.99903593955049));
#43708=CARTESIAN_POINT('Ctrl Pts',(-32.5525454435658,54.3231939478913,3.11017383011854));
#43709=CARTESIAN_POINT('Ctrl Pts',(-30.8746859000025,55.1799232062131,3.22131172068657));
#43710=CARTESIAN_POINT('Ctrl Pts',(-30.6844947844836,57.0542297471953,3.33244961125463));
#43711=CARTESIAN_POINT('Ctrl Pts',(-32.156056181954,58.2305395377937,3.44358750182265));
#43712=CARTESIAN_POINT('Ctrl Pts',(-33.9424332566746,57.6321628864156,3.55472539239071));
#43713=CARTESIAN_POINT('Ctrl Pts',(-34.4085348132464,55.8068007281157,3.66586328295874));
#43714=CARTESIAN_POINT('Ctrl Pts',(-33.1277328110143,54.4252277474092,3.77700117352679));
#43715=CARTESIAN_POINT('Ctrl Pts',(-31.2723598478519,54.7520133616234,3.88813906409483));
#43716=CARTESIAN_POINT('Ctrl Pts',(-30.5406598384056,56.4880469921002,3.99927695466287));
#43717=CARTESIAN_POINT('Ctrl Pts',(-31.6023660991589,58.0443173688379,4.11041484523092));
#43718=CARTESIAN_POINT('Ctrl Pts',(-33.4856868494843,57.9963525668328,4.22155273579895));
#43719=CARTESIAN_POINT('Ctrl Pts',(-34.4667972474874,56.3880553130583,4.332690626367));
#43720=CARTESIAN_POINT('Ctrl Pts',(-33.6476758209426,54.691518323742,4.44382851693504));
#43721=CARTESIAN_POINT('Ctrl Pts',(-31.7780736978197,54.4596011442154,4.55496640750308));
#43722=CARTESIAN_POINT('Ctrl Pts',(-30.5692589105444,55.904580201065,4.66610429807112));
#43723=CARTESIAN_POINT('Ctrl Pts',(-31.1276733300584,57.7038497723057,4.77724218863916));
#43724=CARTESIAN_POINT('Ctrl Pts',(-32.9421939307002,58.210518022386,4.8883800792072));
#43725=CARTESIAN_POINT('Ctrl Pts',(-34.3519693781323,56.9608257398534,4.99951796977525));
#43726=CARTESIAN_POINT('Ctrl Pts',(-34.0666163179288,55.0986304755265,5.11065586034328));
#43727=CARTESIAN_POINT('Ctrl Pts',(-32.3473214420425,54.3284206095854,5.22179375091133));
#43728=CARTESIAN_POINT('Ctrl Pts',(-30.7677752470131,55.3551780944902,5.33293164147937));
#43729=CARTESIAN_POINT('Ctrl Pts',(-30.7737534850632,57.2390999064754,5.44406953204741));
#43730=CARTESIAN_POINT('Ctrl Pts',(-32.3597857865379,58.2558115507951,5.55520742261546));
#43731=CARTESIAN_POINT('Ctrl Pts',(-34.0741556547201,57.4747043239667,5.66634531318349));
#43732=CARTESIAN_POINT('Ctrl Pts',(-34.3476871667892,55.6107365301145,5.77748320375154));
#43733=CARTESIAN_POINT('Ctrl Pts',(-32.9300013656021,54.3700150460704,5.88862109431958));
#43734=CARTESIAN_POINT('Ctrl Pts',(-31.1187469523035,54.8881942477416,5.99975898488762));
#43735=CARTESIAN_POINT('Ctrl Pts',(-30.5717362410347,56.6909630465113,6.11089687545566));
#43736=CARTESIAN_POINT('Ctrl Pts',(-31.7897526682824,58.1282581485762,6.2220347660237));
#43737=CARTESIAN_POINT('Ctrl Pts',(-33.6577362302198,57.8844444704929,6.33317265659175));
#43738=CARTESIAN_POINT('Ctrl Pts',(-34.4662901033036,56.1828120187424,6.44431054715979));
#43739=CARTESIAN_POINT('Ctrl Pts',(-33.4745598537722,54.5806362056383,6.55544843772783));
#43740=CARTESIAN_POINT('Ctrl Pts',(-31.5918327994781,54.5449012067101,6.66658632829588));
#43741=CARTESIAN_POINT('Ctrl Pts',(-30.5383049624388,56.1073232007697,6.77772421886391));
#43742=CARTESIAN_POINT('Ctrl Pts',(-31.2845338942355,57.8398704449838,6.88886210943196));
#43743=CARTESIAN_POINT('Ctrl Pts',(-32.5171523045318,58.0472596234884,6.96295403647732));
#43744=CARTESIAN_POINT('Ctrl Pts',(-33.041102980256,57.8673300091754,7.));
#43745=CARTESIAN_POINT('Ctrl Pts',(-33.3327354544031,57.732107437543,-1.37851963660978));
#43746=CARTESIAN_POINT('Ctrl Pts',(-33.5202555818622,57.6251326319317,-1.36412702194089));
#43747=CARTESIAN_POINT('Ctrl Pts',(-33.6873867521344,57.4836168424902,-1.34973440727201));
#43748=CARTESIAN_POINT('Ctrl Pts',(-33.8186861741814,57.3143142072735,-1.33534179260312));
#43749=CARTESIAN_POINT('Ctrl Pts',(-34.1566451699304,56.8785365954343,-1.29829582908044));
#43750=CARTESIAN_POINT('Ctrl Pts',(-34.2572098089263,56.2586641318032,-1.26124986555776));
#43751=CARTESIAN_POINT('Ctrl Pts',(-34.0743731358877,55.7383874678429,-1.22420390203508));
#43752=CARTESIAN_POINT('Ctrl Pts',(-33.8915364628492,55.2181108038826,-1.1871579385124));
#43753=CARTESIAN_POINT('Ctrl Pts',(-33.4252984777762,54.797429939593,-1.15011197498972));
#43754=CARTESIAN_POINT('Ctrl Pts',(-32.8890270880096,54.6688706003777,-1.11306601146704));
#43755=CARTESIAN_POINT('Ctrl Pts',(-32.352755698243,54.5403112611624,-1.07602004794436));
#43756=CARTESIAN_POINT('Ctrl Pts',(-31.7464509037828,54.7038734470214,-1.03897408442168));
#43757=CARTESIAN_POINT('Ctrl Pts',(-31.3475958266657,55.0847026278185,-1.001928120899));
#43758=CARTESIAN_POINT('Ctrl Pts',(-30.9487407495486,55.4655318086156,-0.964882157376315));
#43759=CARTESIAN_POINT('Ctrl Pts',(-30.7573353897747,56.0636279843508,-0.927836193853635));
#43760=CARTESIAN_POINT('Ctrl Pts',(-30.8609753382403,56.6052687314637,-0.890790230330955));
#43761=CARTESIAN_POINT('Ctrl Pts',(-30.9646152867058,57.1469094785765,-0.853744266808274));
#43762=CARTESIAN_POINT('Ctrl Pts',(-31.3633005434109,57.6320947970672,-0.816698303285594));
#43763=CARTESIAN_POINT('Ctrl Pts',(-31.874571623577,57.8387770341222,-0.779652339762913));
#43764=CARTESIAN_POINT('Ctrl Pts',(-32.3398155301955,58.0268527049873,-0.74594143871187));
#43765=CARTESIAN_POINT('Ctrl Pts',(-32.8982866368194,57.9843126404343,-0.712230537660827));
#43766=CARTESIAN_POINT('Ctrl Pts',(-33.3348489584778,57.7359240281238,-0.678519636609784));
#43767=CARTESIAN_POINT('Ctrl Pts',(-31.045873711622,57.7433792852396,-2.));
#43768=CARTESIAN_POINT('Ctrl Pts',(-31.1022242475567,57.7901329641039,-2.));
#43769=CARTESIAN_POINT('Ctrl Pts',(-31.16109162216,57.8334666739882,-2.));
#43770=CARTESIAN_POINT('Ctrl Pts',(-31.2221267441946,57.8733637960052,-2.));
#43771=CARTESIAN_POINT('Ctrl Pts',(-31.2848602944931,57.9143711378008,-2.));
#43772=CARTESIAN_POINT('Ctrl Pts',(-31.3498848969729,57.9517482942041,-2.));
#43773=CARTESIAN_POINT('Ctrl Pts',(-31.4168445551528,57.9854278643736,-2.));
#43774=CARTESIAN_POINT('Ctrl Pts',(-31.4734239519064,58.0138863394451,-2.));
#43775=CARTESIAN_POINT('Ctrl Pts',(-31.5313856959223,58.039703972078,-2.));
#43776=CARTESIAN_POINT('Ctrl Pts',(-31.5905192436898,58.0628113946312,-2.));
#43777=CARTESIAN_POINT('Ctrl Pts',(-31.616790719774,58.0730774131924,-2.));
#43778=CARTESIAN_POINT('Ctrl Pts',(-31.6432934887177,58.0828081409933,-2.));
#43779=CARTESIAN_POINT('Ctrl Pts',(-31.6700089381812,58.0919957886042,-2.));
#43780=CARTESIAN_POINT('Ctrl Pts',(-31.684687964188,58.0970440180343,-2.));
#43781=CARTESIAN_POINT('Ctrl Pts',(-31.6994311962734,58.1019282705382,-2.));
#43782=CARTESIAN_POINT('Ctrl Pts',(-31.7142355159233,58.1066471169469,-2.));
#43783=CARTESIAN_POINT('Ctrl Pts',(-31.7278877153671,58.110998727412,-2.));
#43784=CARTESIAN_POINT('Ctrl Pts',(-31.7415938959784,58.1152101596117,-2.));
#43785=CARTESIAN_POINT('Ctrl Pts',(-31.7553302775655,58.119274259497,-2.));
#43786=CARTESIAN_POINT('Ctrl Pts',(-31.8255274332731,58.1400430660888,-2.));
#43787=CARTESIAN_POINT('Ctrl Pts',(-31.8966328017533,58.1570081793261,-2.));
#43788=CARTESIAN_POINT('Ctrl Pts',(-31.9683123621953,58.170109952811,-2.));
#43789=CARTESIAN_POINT('Ctrl Pts',(-32.0394355875927,58.1831100379529,-2.));
#43790=CARTESIAN_POINT('Ctrl Pts',(-32.1111251456288,58.1923065191834,-2.));
#43791=CARTESIAN_POINT('Ctrl Pts',(-32.1830533294103,58.1975902176944,-2.));
#43792=CARTESIAN_POINT('Ctrl Pts',(-32.2428321680078,58.2019814499469,-2.));
#43793=CARTESIAN_POINT('Ctrl Pts',(-32.3027760709099,58.203669194572,-2.));
#43794=CARTESIAN_POINT('Ctrl Pts',(-32.3626887231027,58.2025636252019,-2.));
#43795=CARTESIAN_POINT('Ctrl Pts',(-32.3876963771335,58.2021021584615,-2.));
#43796=CARTESIAN_POINT('Ctrl Pts',(-32.412698459505,58.201153730257,-2.));
#43797=CARTESIAN_POINT('Ctrl Pts',(-32.4376800452459,58.1997105189459,-2.));
#43798=CARTESIAN_POINT('Ctrl Pts',(-32.4492432419443,58.1990425014532,-2.));
#43799=CARTESIAN_POINT('Ctrl Pts',(-32.46080204105,58.198268467185,-2.));
#43800=CARTESIAN_POINT('Ctrl Pts',(-32.4723549281043,58.1973875849115,-2.));
#43801=CARTESIAN_POINT('Ctrl Pts',(-32.4844044306665,58.1964688367959,-2.));
#43802=CARTESIAN_POINT('Ctrl Pts',(-32.4964392274819,58.1954344592299,-2.));
#43803=CARTESIAN_POINT('Ctrl Pts',(-32.5084532356201,58.1942844547161,-2.));
#43804=CARTESIAN_POINT('Ctrl Pts',(-32.576878307084,58.187734672151,-2.));
#43805=CARTESIAN_POINT('Ctrl Pts',(-32.644677403631,58.1774344901198,-2.));
#43806=CARTESIAN_POINT('Ctrl Pts',(-32.7115617527711,58.1632926068264,-2.));
#43807=CARTESIAN_POINT('Ctrl Pts',(-32.7721836417578,58.1504748446728,-2.));
#43808=CARTESIAN_POINT('Ctrl Pts',(-32.8320544200173,58.1345005317114,-2.));
#43809=CARTESIAN_POINT('Ctrl Pts',(-32.8909448795169,58.1152674430859,-2.));
#43810=CARTESIAN_POINT('Ctrl Pts',(-32.9606152109761,58.0925137462918,-2.));
#43811=CARTESIAN_POINT('Ctrl Pts',(-33.0289150978522,58.0651988064951,-2.));
#43812=CARTESIAN_POINT('Ctrl Pts',(-33.0955156401827,58.0335993051752,-2.));
#43813=CARTESIAN_POINT('Ctrl Pts',(-33.1101787046012,58.0266422218357,-2.));
#43814=CARTESIAN_POINT('Ctrl Pts',(-33.1247592149198,58.0194773027427,-2.));
#43815=CARTESIAN_POINT('Ctrl Pts',(-33.1392533337008,58.0121072627471,-2.));
#43816=CARTESIAN_POINT('Ctrl Pts',(-33.1542086549745,58.0045027082655,-2.));
#43817=CARTESIAN_POINT('Ctrl Pts',(-33.1690773275701,57.9966767059895,-2.));
#43818=CARTESIAN_POINT('Ctrl Pts',(-33.1838253281019,57.9886488037328,-2.));
#43819=CARTESIAN_POINT('Ctrl Pts',(-33.2440619540896,57.9558596982087,-2.));
#43820=CARTESIAN_POINT('Ctrl Pts',(-33.3023667325631,57.9196691076086,-2.));
#43821=CARTESIAN_POINT('Ctrl Pts',(-33.3585069616797,57.8803506668497,-2.));
#43822=CARTESIAN_POINT('Ctrl Pts',(-33.4146358505063,57.8410401683904,-2.));
#43823=CARTESIAN_POINT('Ctrl Pts',(-33.4686017656045,57.7986021545295,-2.));
#43824=CARTESIAN_POINT('Ctrl Pts',(-33.5201343260632,57.753274648848,-2.));
#43825=CARTESIAN_POINT('Ctrl Pts',(-33.5574338655409,57.720466360796,-2.));
#43826=CARTESIAN_POINT('Ctrl Pts',(-33.5934578303088,57.6861435081364,-2.));
#43827=CARTESIAN_POINT('Ctrl Pts',(-33.6280882156071,57.650388864236,-2.));
#43828=CARTESIAN_POINT('Ctrl Pts',(-33.6540651537613,57.6235685974292,-2.));
#43829=CARTESIAN_POINT('Ctrl Pts',(-33.679257693834,57.5959425521655,-2.));
#43830=CARTESIAN_POINT('Ctrl Pts',(-33.7036104503286,57.5675443622685,-2.));
#43831=CARTESIAN_POINT('Ctrl Pts',(-33.7117026688921,57.558107879811,-2.));
#43832=CARTESIAN_POINT('Ctrl Pts',(-33.719695777907,57.5485935240877,-2.));
#43833=CARTESIAN_POINT('Ctrl Pts',(-33.7275879316845,57.5390030774341,-2.));
#43834=CARTESIAN_POINT('Ctrl Pts',(-33.769451093524,57.4881314862703,-2.));
#43835=CARTESIAN_POINT('Ctrl Pts',(-33.8084798256294,57.4351175562881,-2.));
#43836=CARTESIAN_POINT('Ctrl Pts',(-33.8444097934601,57.3801716628579,-2.));
#43837=CARTESIAN_POINT('Ctrl Pts',(-33.8696919535345,57.3415089265126,-2.));
#43838=CARTESIAN_POINT('Ctrl Pts',(-33.8934389530086,57.3018891510271,-2.));
#43839=CARTESIAN_POINT('Ctrl Pts',(-33.9155436487734,57.2613822920624,-2.));
#43840=CARTESIAN_POINT('Ctrl Pts',(-33.9226388854327,57.2483802696082,-2.));
#43841=CARTESIAN_POINT('Ctrl Pts',(-33.9295657376833,57.2352850255484,-2.));
#43842=CARTESIAN_POINT('Ctrl Pts',(-33.936317410013,57.2221046384805,-2.));
#43843=CARTESIAN_POINT('Ctrl Pts',(-33.9650804421564,57.1659544169675,-2.));
#43844=CARTESIAN_POINT('Ctrl Pts',(-33.9906110254719,57.1083731118225,-2.));
#43845=CARTESIAN_POINT('Ctrl Pts',(-34.012653283144,57.0495480070843,-2.));
#43846=CARTESIAN_POINT('Ctrl Pts',(-34.0329745304356,56.9953158354927,-2.));
#43847=CARTESIAN_POINT('Ctrl Pts',(-34.0503306992892,56.9400259525903,-2.));
#43848=CARTESIAN_POINT('Ctrl Pts',(-34.0644820150771,56.8838229928237,-2.));
#43849=CARTESIAN_POINT('Ctrl Pts',(-34.0671303463503,56.8733049563223,-2.));
#43850=CARTESIAN_POINT('Ctrl Pts',(-34.0696663195691,56.8627549469952,-2.));
#43851=CARTESIAN_POINT('Ctrl Pts',(-34.0720901513885,56.8521746541717,-2.));
#43852=CARTESIAN_POINT('Origin',(-32.5,56.2916512459885,3.));
#43853=CARTESIAN_POINT('Origin',(32.5,56.2916512459885,7.));
#43854=CARTESIAN_POINT('Ctrl Pts',(33.5940263469955,57.5480995545471,7.));
#43855=CARTESIAN_POINT('Ctrl Pts',(33.6455781063593,57.5127482049878,7.));
#43856=CARTESIAN_POINT('Ctrl Pts',(33.6948218851594,57.4743678095804,7.));
#43857=CARTESIAN_POINT('Ctrl Pts',(33.7416962543858,57.4332901552688,7.));
#43858=CARTESIAN_POINT('Ctrl Pts',(33.7714300138311,57.4072334186761,7.));
#43859=CARTESIAN_POINT('Ctrl Pts',(33.8002101106111,57.3800903098691,7.));
#43860=CARTESIAN_POINT('Ctrl Pts',(33.8280169256125,57.3519357929662,7.));
#43861=CARTESIAN_POINT('Ctrl Pts',(33.8470314137092,57.3326835439585,7.));
#43862=CARTESIAN_POINT('Ctrl Pts',(33.8655907373089,57.3129582157456,7.));
#43863=CARTESIAN_POINT('Ctrl Pts',(33.8836875902375,57.2927820229205,7.));
#43864=CARTESIAN_POINT('Ctrl Pts',(33.8932692328479,57.2820994434879,7.));
#43865=CARTESIAN_POINT('Ctrl Pts',(33.9027209653718,57.2712905497247,7.));
#43866=CARTESIAN_POINT('Ctrl Pts',(33.9120326403695,57.2603695725943,7.));
#43867=CARTESIAN_POINT('Ctrl Pts',(33.9548352574687,57.2101695384892,7.));
#43868=CARTESIAN_POINT('Ctrl Pts',(33.9947314180079,57.1575493208277,7.));
#43869=CARTESIAN_POINT('Ctrl Pts',(34.031636585354,57.1028515984669,7.));
#43870=CARTESIAN_POINT('Ctrl Pts',(34.0582554673164,57.0633993396144,7.));
#43871=CARTESIAN_POINT('Ctrl Pts',(34.0833178687179,57.0228651366186,7.));
#43872=CARTESIAN_POINT('Ctrl Pts',(34.1067823368899,56.9813639740226,7.));
#43873=CARTESIAN_POINT('Ctrl Pts',(34.1132255644837,56.96996795882,7.));
#43874=CARTESIAN_POINT('Ctrl Pts',(34.1195482501362,56.9584989754116,7.));
#43875=CARTESIAN_POINT('Ctrl Pts',(34.1257494083041,56.9469592819649,7.));
#43876=CARTESIAN_POINT('Ctrl Pts',(34.132058329377,56.9352190532546,7.));
#43877=CARTESIAN_POINT('Ctrl Pts',(34.1382375554008,56.9234128300226,7.));
#43878=CARTESIAN_POINT('Ctrl Pts',(34.1442842648129,56.9115477360727,7.));
#43879=CARTESIAN_POINT('Ctrl Pts',(34.1750933789438,56.8510928657025,7.));
#43880=CARTESIAN_POINT('Ctrl Pts',(34.2024838357259,56.7890775489765,7.));
#43881=CARTESIAN_POINT('Ctrl Pts',(34.2263706779214,56.7258494465016,7.));
#43882=CARTESIAN_POINT('Ctrl Pts',(34.2506031311489,56.6617065169613,7.));
#43883=CARTESIAN_POINT('Ctrl Pts',(34.2712305305803,56.5963146347364,7.));
#43884=CARTESIAN_POINT('Ctrl Pts',(34.2881270715367,56.5299991239702,7.));
#43885=CARTESIAN_POINT('Ctrl Pts',(34.2985953641974,56.4889131894921,7.));
#43886=CARTESIAN_POINT('Ctrl Pts',(34.3076308155221,56.447472028122,7.));
#43887=CARTESIAN_POINT('Ctrl Pts',(34.3151947514802,56.4057480907575,7.));
#43888=CARTESIAN_POINT('Ctrl Pts',(34.3213914047376,56.3715663137289,7.));
#43889=CARTESIAN_POINT('Ctrl Pts',(34.3266003410567,56.337194665163,7.));
#43890=CARTESIAN_POINT('Ctrl Pts',(34.3307964558936,56.3026718436529,7.));
#43891=CARTESIAN_POINT('Ctrl Pts',(34.3325110302053,56.2885654749698,7.));
#43892=CARTESIAN_POINT('Ctrl Pts',(34.3340565736349,56.2744313049453,7.));
#43893=CARTESIAN_POINT('Ctrl Pts',(34.3354292580617,56.2602960057088,7.));
#43894=CARTESIAN_POINT('Ctrl Pts',(34.3422420688248,56.1901406831141,7.));
#43895=CARTESIAN_POINT('Ctrl Pts',(34.3448171217661,56.11983645962,7.));
#43896=CARTESIAN_POINT('Ctrl Pts',(34.3430393002862,56.0497278065194,7.));
#43897=CARTESIAN_POINT('Ctrl Pts',(34.3428417470465,56.0419372652815,7.));
#43898=CARTESIAN_POINT('Ctrl Pts',(34.3425903992446,56.0341491123532,7.));
#43899=CARTESIAN_POINT('Ctrl Pts',(34.3422850635953,56.0263638020432,7.));
#43900=CARTESIAN_POINT('Ctrl Pts',(34.3396426913258,55.958989788811,7.));
#43901=CARTESIAN_POINT('Ctrl Pts',(34.3329614085344,55.8918294784504,7.));
#43902=CARTESIAN_POINT('Ctrl Pts',(34.3224781325172,55.825128323823,7.));
#43903=CARTESIAN_POINT('Ctrl Pts',(34.3112000078435,55.7533698452192,7.));
#43904=CARTESIAN_POINT('Ctrl Pts',(34.295521853206,55.6821418491415,7.));
#43905=CARTESIAN_POINT('Ctrl Pts',(34.2756745307237,55.6117461590107,7.));
#43906=CARTESIAN_POINT('Ctrl Pts',(34.2720417379785,55.5988611488225,7.));
#43907=CARTESIAN_POINT('Ctrl Pts',(34.2682690982962,55.5860040374986,7.));
#43908=CARTESIAN_POINT('Ctrl Pts',(34.2643578039031,55.5731767059407,7.));
#43909=CARTESIAN_POINT('Ctrl Pts',(34.2609943803684,55.5621461507044,7.));
#43910=CARTESIAN_POINT('Ctrl Pts',(34.2575311416983,55.5511465596784,7.));
#43911=CARTESIAN_POINT('Ctrl Pts',(34.2539698126456,55.5401805084982,7.));
#43912=CARTESIAN_POINT('Ctrl Pts',(34.2320182881598,55.4725873326265,7.));
#43913=CARTESIAN_POINT('Ctrl Pts',(34.2063390659048,55.4062514118632,7.));
#43914=CARTESIAN_POINT('Ctrl Pts',(34.1772031613691,55.3414402689902,7.));
#43915=CARTESIAN_POINT('Ctrl Pts',(34.1474529584126,55.2752626546329,7.));
#43916=CARTESIAN_POINT('Ctrl Pts',(34.1140985514797,55.2106738828667,7.));
#43917=CARTESIAN_POINT('Ctrl Pts',(34.077373335558,55.1479588365199,7.));
#43918=CARTESIAN_POINT('Ctrl Pts',(34.0404255619581,55.0848637320919,7.));
#43919=CARTESIAN_POINT('Ctrl Pts',(34.0000656099289,55.0236641322245,7.));
#43920=CARTESIAN_POINT('Ctrl Pts',(33.956480802391,54.9646647044169,7.));
#43921=CARTESIAN_POINT('Ctrl Pts',(33.9457092802779,54.9500836226779,7.));
#43922=CARTESIAN_POINT('Ctrl Pts',(33.9347405676772,54.9356370332213,7.));
#43923=CARTESIAN_POINT('Ctrl Pts',(33.9235770658016,54.9213297824322,7.));
#43924=CARTESIAN_POINT('Ctrl Pts',(33.9148444637425,54.9101379961009,7.));
#43925=CARTESIAN_POINT('Ctrl Pts',(33.9059915495185,54.8990302860272,7.));
#43926=CARTESIAN_POINT('Ctrl Pts',(33.89703329402,54.888025539777,7.));
#43927=CARTESIAN_POINT('Ctrl Pts',(33.8494695085346,54.8295959281122,7.));
#43928=CARTESIAN_POINT('Ctrl Pts',(33.7988575667886,54.7739598964368,6.99999999999999));
#43929=CARTESIAN_POINT('Ctrl Pts',(33.7454538505468,54.7214122178166,6.99999999999999));
#43930=CARTESIAN_POINT('Ctrl Pts',(33.691992046168,54.6688073821863,6.99999999999999));
#43931=CARTESIAN_POINT('Ctrl Pts',(33.6357318981107,54.6192966067137,7.));
#43932=CARTESIAN_POINT('Ctrl Pts',(33.5768824664943,54.5731951202135,7.));
#43933=CARTESIAN_POINT('Ctrl Pts',(33.5193724813759,54.5281429297379,7.));
#43934=CARTESIAN_POINT('Ctrl Pts',(33.4593891252722,54.4863457605992,7.));
#43935=CARTESIAN_POINT('Ctrl Pts',(33.3970899729434,54.4481299155973,7.));
#43936=CARTESIAN_POINT('Ctrl Pts',(33.3836932590424,54.4399120390638,7.));
#43937=CARTESIAN_POINT('Ctrl Pts',(33.3701893373732,54.4318599153263,6.99999999999999));
#43938=CARTESIAN_POINT('Ctrl Pts',(33.356579582449,54.4239770468377,6.99999999999999));
#43939=CARTESIAN_POINT('Ctrl Pts',(33.3450551424613,54.417302007843,6.99999999999999));
#43940=CARTESIAN_POINT('Ctrl Pts',(33.3334548151719,54.4107483324245,7.));
#43941=CARTESIAN_POINT('Ctrl Pts',(33.3217804591137,54.4043158724519,7.));
#43942=CARTESIAN_POINT('Ctrl Pts',(32.2716262263503,54.2496319067047,7.));
#43943=CARTESIAN_POINT('Ctrl Pts',(32.1985421824179,54.2648284787425,7.));
#43944=CARTESIAN_POINT('Ctrl Pts',(32.1265185433355,54.2843049160475,7.));
#43945=CARTESIAN_POINT('Ctrl Pts',(32.055814870235,54.3078098414778,7.));
#43946=CARTESIAN_POINT('Ctrl Pts',(31.9869629438864,54.3306991670755,7.));
#43947=CARTESIAN_POINT('Ctrl Pts',(31.9193621916298,54.3574095812603,7.));
#43948=CARTESIAN_POINT('Ctrl Pts',(31.8532778586936,54.3877469743405,7.));
#43949=CARTESIAN_POINT('Ctrl Pts',(31.8385281518176,54.3945181353016,7.));
#43950=CARTESIAN_POINT('Ctrl Pts',(31.8238521664773,54.4014710565443,7.));
#43951=CARTESIAN_POINT('Ctrl Pts',(31.8092592839734,54.4086007384021,7.));
#43952=CARTESIAN_POINT('Ctrl Pts',(31.7422937925777,54.4413182394836,7.));
#43953=CARTESIAN_POINT('Ctrl Pts',(31.6772081434645,54.4776886922259,7.));
#43954=CARTESIAN_POINT('Ctrl Pts',(31.6142783996461,54.517480847036,7.));
#43955=CARTESIAN_POINT('Ctrl Pts',(31.5700975700385,54.5454175635187,7.));
#43956=CARTESIAN_POINT('Ctrl Pts',(31.5269799621108,54.5750417874127,7.));
#43957=CARTESIAN_POINT('Ctrl Pts',(31.4850325699083,54.6062837165385,7.));
#43958=CARTESIAN_POINT('Ctrl Pts',(31.469084365258,54.6181617536036,7.));
#43959=CARTESIAN_POINT('Ctrl Pts',(31.4533054234991,54.6302737013537,7.));
#43960=CARTESIAN_POINT('Ctrl Pts',(31.4377020513635,54.6426159722202,7.));
#43961=CARTESIAN_POINT('Ctrl Pts',(31.422843223124,54.6543693086974,7.));
#43962=CARTESIAN_POINT('Ctrl Pts',(31.4081391342014,54.6663354488099,7.));
#43963=CARTESIAN_POINT('Ctrl Pts',(31.393620803187,54.6784895995769,7.));
#43964=CARTESIAN_POINT('Ctrl Pts',(31.3379553553849,54.7250904274836,7.));
#43965=CARTESIAN_POINT('Ctrl Pts',(31.284955832515,54.7744982188359,7.));
#43966=CARTESIAN_POINT('Ctrl Pts',(31.2348792621311,54.8265005113593,7.));
#43967=CARTESIAN_POINT('Ctrl Pts',(31.1858781212174,54.8773860181788,7.));
#43968=CARTESIAN_POINT('Ctrl Pts',(31.1396752549895,54.9307565896115,7.));
#43969=CARTESIAN_POINT('Ctrl Pts',(31.096553263567,54.98643879979,7.));
#43970=CARTESIAN_POINT('Ctrl Pts',(31.0543769959643,55.0408998234981,7.));
#43971=CARTESIAN_POINT('Ctrl Pts',(31.0151475677328,55.0975728716066,7.));
#43972=CARTESIAN_POINT('Ctrl Pts',(30.9791760533412,55.1563097700117,7.));
#43973=CARTESIAN_POINT('Ctrl Pts',(30.9674871681413,55.175396229786,7.));
#43974=CARTESIAN_POINT('Ctrl Pts',(30.9561426884268,55.19470068603,7.));
#43975=CARTESIAN_POINT('Ctrl Pts',(30.9451544834666,55.2142182090717,7.));
#43976=CARTESIAN_POINT('Ctrl Pts',(30.9389559539872,55.2252281913552,7.));
#43977=CARTESIAN_POINT('Ctrl Pts',(30.9328702746375,55.2363071799956,7.));
#43978=CARTESIAN_POINT('Ctrl Pts',(30.9269078404286,55.2474384077617,7.));
#43979=CARTESIAN_POINT('Ctrl Pts',(30.8946567101692,55.3076478229186,7.));
#43980=CARTESIAN_POINT('Ctrl Pts',(30.8659479670597,55.369487708999,6.99999999999999));
#43981=CARTESIAN_POINT('Ctrl Pts',(30.8410371124974,55.4327943982586,7.));
#43982=CARTESIAN_POINT('Ctrl Pts',(30.8374416945958,55.4419315397919,7.));
#43983=CARTESIAN_POINT('Ctrl Pts',(30.8339254772762,55.4510992636488,7.));
#43984=CARTESIAN_POINT('Ctrl Pts',(30.8304893165614,55.4602971020132,7.));
#43985=CARTESIAN_POINT('Ctrl Pts',(30.8062112767742,55.5252840174394,7.));
#43986=CARTESIAN_POINT('Ctrl Pts',(30.7859254272867,55.5917741516785,7.));
#43987=CARTESIAN_POINT('Ctrl Pts',(30.7695892422456,55.6594016433533,7.));
#43988=CARTESIAN_POINT('Ctrl Pts',(30.7543489013094,55.7224926298468,7.));
#43989=CARTESIAN_POINT('Ctrl Pts',(30.7425467760767,55.7865743173607,7.));
#43990=CARTESIAN_POINT('Ctrl Pts',(30.734187897611,55.8513431276599,7.));
#43991=CARTESIAN_POINT('Ctrl Pts',(30.7323430806899,55.8656377005129,7.));
#43992=CARTESIAN_POINT('Ctrl Pts',(30.7306661227445,55.8799656905854,7.));
#43993=CARTESIAN_POINT('Ctrl Pts',(30.7291573147969,55.8943237311442,7.));
#43994=CARTESIAN_POINT('Ctrl Pts',(30.7279778703883,55.905547499339,7.));
#43995=CARTESIAN_POINT('Ctrl Pts',(30.7269013312022,55.9167889367441,7.));
#43996=CARTESIAN_POINT('Ctrl Pts',(30.7259287166033,55.9280334135351,7.));
#43997=CARTESIAN_POINT('Ctrl Pts',(30.7200365397314,55.9961533514445,7.));
#43998=CARTESIAN_POINT('Ctrl Pts',(30.7179403223651,56.0645103688077,7.));
#43999=CARTESIAN_POINT('Ctrl Pts',(30.7195810692469,56.1327563915374,7.));
#44000=CARTESIAN_POINT('Ctrl Pts',(30.7212142396031,56.200687272582,7.));
#44001=CARTESIAN_POINT('Ctrl Pts',(30.7265502690293,56.2685092691059,7.));
#44002=CARTESIAN_POINT('Ctrl Pts',(30.7355805426662,56.3358665627088,7.));
#44003=CARTESIAN_POINT('Ctrl Pts',(30.7444173748676,56.4017809663077,7.));
#44004=CARTESIAN_POINT('Ctrl Pts',(30.7567922827814,56.4672512456727,7.));
#44005=CARTESIAN_POINT('Ctrl Pts',(30.7727391548109,56.5319175329114,7.));
#44006=CARTESIAN_POINT('Ctrl Pts',(30.7760991369442,56.5455426231072,7.));
#44007=CARTESIAN_POINT('Ctrl Pts',(30.7796178314759,56.5591318993402,7.));
#44008=CARTESIAN_POINT('Ctrl Pts',(30.7832957743544,56.5726817859276,7.));
#44009=CARTESIAN_POINT('Ctrl Pts',(30.786782084737,56.5855256804234,7.));
#44010=CARTESIAN_POINT('Ctrl Pts',(30.790412102401,56.5983358605448,7.));
#44011=CARTESIAN_POINT('Ctrl Pts',(30.7941799174142,56.6110887259411,7.));
#44012=CARTESIAN_POINT('Ctrl Pts',(30.8126945730391,56.6737549954412,7.));
#44013=CARTESIAN_POINT('Ctrl Pts',(30.8345622313707,56.7351520398133,7.));
#44014=CARTESIAN_POINT('Ctrl Pts',(30.8597663050147,56.794960649957,7.));
#44015=CARTESIAN_POINT('Ctrl Pts',(30.8844910320025,56.8536317829735,7.));
#44016=CARTESIAN_POINT('Ctrl Pts',(30.9124268768565,56.9107751110938,7.));
#44017=CARTESIAN_POINT('Ctrl Pts',(30.9435976955446,56.9660591311284,7.));
#44018=CARTESIAN_POINT('Ctrl Pts',(30.97375602352,57.019547415305,7.));
#44019=CARTESIAN_POINT('Ctrl Pts',(31.0069429903275,57.0712957445369,7.));
#44020=CARTESIAN_POINT('Ctrl Pts',(31.0432115503434,57.1209660580098,7.));
#44021=CARTESIAN_POINT('Ctrl Pts',(31.0492497805401,57.1292355009257,7.));
#44022=CARTESIAN_POINT('Ctrl Pts',(31.055373490492,57.1374472482377,7.));
#44023=CARTESIAN_POINT('Ctrl Pts',(31.0615830007349,57.1455996184164,7.));
#44024=CARTESIAN_POINT('Ctrl Pts',(31.0681540675971,57.1542266707015,7.));
#44025=CARTESIAN_POINT('Ctrl Pts',(31.0748212184917,57.1627872296297,7.));
#44026=CARTESIAN_POINT('Ctrl Pts',(31.0815830733444,57.1712803260696,7.));
#44027=CARTESIAN_POINT('Origin',(32.5,56.2916512459885,-3.54592528053767));
#44028=CARTESIAN_POINT('Ctrl Pts',(33.5269872402601,58.0734398505124,-1.79592528053768));
#44029=CARTESIAN_POINT('Ctrl Pts',(33.4422748054587,58.1232938101479,-1.79058130531689));
#44030=CARTESIAN_POINT('Ctrl Pts',(32.7422362990183,58.4684621317491,-1.74819136657341));
#44031=CARTESIAN_POINT('Ctrl Pts',(31.0929180917129,58.2713739433872,-1.66875546430726));
#44032=CARTESIAN_POINT('Ctrl Pts',(30.0738503853477,56.1831963302234,-1.55761757373922));
#44033=CARTESIAN_POINT('Ctrl Pts',(31.2751851021384,54.1944751483927,-1.44647968317118));
#44034=CARTESIAN_POINT('Ctrl Pts',(33.5977473666623,54.1252293793916,-1.33534179260313));
#44035=CARTESIAN_POINT('Ctrl Pts',(34.9154583912003,56.0389811637256,-1.22420390203509));
#44036=CARTESIAN_POINT('Ctrl Pts',(34.2741084270659,57.5792551456252,-1.14439839801327));
#44037=CARTESIAN_POINT('Ctrl Pts',(33.6210824061175,58.0199411501776,-1.10163885751414));
#44038=CARTESIAN_POINT('Ctrl Pts',(33.5295799600394,58.0717283210701,-1.09592528053768));
#44039=CARTESIAN_POINT('Ctrl Pts',(33.5283546803393,58.0681541983481,-1.85407471946233));
#44040=CARTESIAN_POINT('Ctrl Pts',(33.1193657433931,58.3001842134597,-1.82862455259619));
#44041=CARTESIAN_POINT('Ctrl Pts',(31.9170343357855,58.5410390719137,-1.76612842220737));
#44042=CARTESIAN_POINT('Ctrl Pts',(30.2743670907292,57.2623912321518,-1.66658632829588));
#44043=CARTESIAN_POINT('Ctrl Pts',(30.4765028746713,54.9487367869863,-1.55544843772783));
#44044=CARTESIAN_POINT('Ctrl Pts',(32.5312595152502,53.8630292597192,-1.44431054715979));
#44045=CARTESIAN_POINT('Ctrl Pts',(34.5571577499754,55.0008883544572,-1.33317265659175));
#44046=CARTESIAN_POINT('Ctrl Pts',(34.6817103419942,57.0195698185232,-1.23642738069259));
#44047=CARTESIAN_POINT('Ctrl Pts',(33.8868873402924,57.8579713309385,-1.17672806831612));
#44048=CARTESIAN_POINT('Ctrl Pts',(33.5250365419916,58.0693901510839,-1.15407471946233));
#44049=CARTESIAN_POINT('Ctrl Pts',(30.9307125467392,55.7322829513575,-2.));
#44050=CARTESIAN_POINT('Ctrl Pts',(31.116715812632,55.2104575382394,-1.96295403647732));
#44051=CARTESIAN_POINT('Ctrl Pts',(32.0473824090187,54.3760622611663,-1.88886210943196));
#44052=CARTESIAN_POINT('Ctrl Pts',(33.8672110770871,54.8728632770318,-1.77772421886392));
#44053=CARTESIAN_POINT('Ctrl Pts',(34.4318965215284,56.6706982888814,-1.66658632829588));
#44054=CARTESIAN_POINT('Ctrl Pts',(33.2300975250658,58.1203931132112,-1.55544843772783));
#44055=CARTESIAN_POINT('Ctrl Pts',(31.3591320310469,57.8968187913669,-1.44431054715979));
#44056=CARTESIAN_POINT('Ctrl Pts',(30.5328676198999,56.2037155410781,-1.33317265659175));
#44057=CARTESIAN_POINT('Ctrl Pts',(31.5069148948352,54.5912519864218,-1.22203476602371));
#44058=CARTESIAN_POINT('Ctrl Pts',(33.3900582128528,54.5351072237228,-1.11089687545567));
#44059=CARTESIAN_POINT('Ctrl Pts',(34.4584638908577,56.0867852734614,-0.999758984887625));
#44060=CARTESIAN_POINT('Ctrl Pts',(33.7342941276566,57.825960305992,-0.888621094319583));
#44061=CARTESIAN_POINT('Ctrl Pts',(31.8803464986039,58.1607744839985,-0.777483203751541));
#44062=CARTESIAN_POINT('Ctrl Pts',(30.5935820077055,56.7847541278007,-0.6663453131835));
#44063=CARTESIAN_POINT('Ctrl Pts',(31.0517798775846,54.9573935418363,-0.555207422615458));
#44064=CARTESIAN_POINT('Ctrl Pts',(32.8355518820609,54.3512929431319,-0.444069532047416));
#44065=CARTESIAN_POINT('Ctrl Pts',(34.3121885227868,55.521224917537,-0.332931641479374));
#44066=CARTESIAN_POINT('Ctrl Pts',(34.1301089195293,57.3963365394661,-0.221793750911333));
#44067=CARTESIAN_POINT('Ctrl Pts',(32.4559719031607,58.2603173390956,-0.110655860343291));
#44068=CARTESIAN_POINT('Ctrl Pts',(30.822134419883,57.3223556597407,0.000482030224751112));
#44069=CARTESIAN_POINT('Ctrl Pts',(30.724066271727,55.4409785805668,0.111619920792792));
#44070=CARTESIAN_POINT('Ctrl Pts',(32.2515304349822,54.3382318197086,0.222757811360835));
#44071=CARTESIAN_POINT('Ctrl Pts',(34.0064215941321,55.0234720228687,0.333895701928877));
#44072=CARTESIAN_POINT('Ctrl Pts',(34.3824679916267,56.8694910461269,0.445033592496917));
#44073=CARTESIAN_POINT('Ctrl Pts',(33.0354700840103,58.1866067496581,0.55617148306496));
#44074=CARTESIAN_POINT('Ctrl Pts',(31.1983503377324,57.7692481891733,0.667309373633001));
#44075=CARTESIAN_POINT('Ctrl Pts',(30.5526452880963,55.9994283901304,0.778447264201044));
#44076=CARTESIAN_POINT('Ctrl Pts',(31.6893760912438,54.4970834847716,0.889585154769084));
#44077=CARTESIAN_POINT('Ctrl Pts',(33.5680801509383,54.6373268031956,1.00072304533713));
#44078=CARTESIAN_POINT('Ctrl Pts',(34.4691583357458,56.2917920453437,1.11186093590517));
#44079=CARTESIAN_POINT('Ctrl Pts',(33.5678435640106,57.9461284122851,1.22299882647321));
#44080=CARTESIAN_POINT('Ctrl Pts',(31.6891194679972,58.086103065848,1.33413671704125));
#44081=CARTESIAN_POINT('Ctrl Pts',(30.5526035189213,56.5835956182358,1.44527460760929));
#44082=CARTESIAN_POINT('Ctrl Pts',(31.1985616539627,54.8138681758263,1.55641249817734));
#44083=CARTESIAN_POINT('Ctrl Pts',(33.0357410664428,54.3967723367386,1.66755038874538));
#44084=CARTESIAN_POINT('Ctrl Pts',(34.3825506050928,55.7140806526746,1.77868827931342));
#44085=CARTESIAN_POINT('Ctrl Pts',(34.0062402253245,57.5600458827673,1.88982616988146));
#44086=CARTESIAN_POINT('Ctrl Pts',(32.2512510853912,58.2450351172428,2.0009640604495));
#44087=CARTESIAN_POINT('Ctrl Pts',(30.7239446480036,57.1420699414794,2.11210195101754));
#44088=CARTESIAN_POINT('Ctrl Pts',(30.8222818161361,55.2607068893292,2.22323984158559));
#44089=CARTESIAN_POINT('Ctrl Pts',(32.4562534645774,54.3229788985336,2.33437773215363));
#44090=CARTESIAN_POINT('Ctrl Pts',(34.1302668130106,55.1871990336262,2.44551562272167));
#44091=CARTESIAN_POINT('Ctrl Pts',(34.3120784590119,57.0623368040342,2.55665351328971));
#44092=CARTESIAN_POINT('Ctrl Pts',(32.8352741411123,58.2320573429941,2.66779140385776));
#44093=CARTESIAN_POINT('Ctrl Pts',(31.0515895995852,57.6257021756631,2.77892929442579));
#44094=CARTESIAN_POINT('Ctrl Pts',(30.5936515236489,55.7982750632342,2.89006718499384));
#44095=CARTESIAN_POINT('Ctrl Pts',(31.8806158275789,54.4224407661471,3.00120507556188));
#44096=CARTESIAN_POINT('Ctrl Pts',(33.7345094888202,54.757516019547,3.11234296612992));
#44097=CARTESIAN_POINT('Ctrl Pts',(34.4584426146545,56.4968026439861,3.22348085669796));
#44098=CARTESIAN_POINT('Ctrl Pts',(33.3897910050459,58.0483118672624,3.33461874726601));
#44099=CARTESIAN_POINT('Ctrl Pts',(31.506703597602,57.9919297020009,3.44575663783404));
#44100=CARTESIAN_POINT('Ctrl Pts',(30.5327916520213,56.3792633834812,3.55689452840209));
#44101=CARTESIAN_POINT('Ctrl Pts',(31.3594878170038,54.6864046819268,3.66803241897013));
#44102=CARTESIAN_POINT('Ctrl Pts',(33.230107717374,54.4628463651893,3.77917030953817));
#44103=CARTESIAN_POINT('Ctrl Pts',(34.4324517440404,55.9132138959114,3.89030820010621));
#44104=CARTESIAN_POINT('Ctrl Pts',(33.8660007739066,57.7099694249182,4.00144609067425));
#44105=CARTESIAN_POINT('Ctrl Pts',(32.0492338038872,58.2085222399532,4.1125839812423));
#44106=CARTESIAN_POINT('Ctrl Pts',(30.6450582452589,56.9525412953675,4.22372187181034));
#44107=CARTESIAN_POINT('Ctrl Pts',(30.9387319111105,55.0916401936804,4.33485976237839));
#44108=CARTESIAN_POINT('Ctrl Pts',(32.6614519649159,54.3291228170264,4.44599765294642));
#44109=CARTESIAN_POINT('Ctrl Pts',(34.2363932038283,55.3629299683766,4.55713554351447));
#44110=CARTESIAN_POINT('Ctrl Pts',(34.2219940520658,57.2468062367664,4.6682734340825));
#44111=CARTESIAN_POINT('Ctrl Pts',(32.6314342140598,58.2564183114437,4.77941132465055));
#44112=CARTESIAN_POINT('Ctrl Pts',(30.9205711526377,57.4676568060689,4.89054921521858));
#44113=CARTESIAN_POINT('Ctrl Pts',(30.6553772206223,55.602484080847,5.00168710578663));
#44114=CARTESIAN_POINT('Ctrl Pts',(32.0785874510053,54.3681138654151,5.11282499635467));
#44115=CARTESIAN_POINT('Ctrl Pts',(33.8875213407722,54.8943792530066,5.22396288692271));
#44116=CARTESIAN_POINT('Ctrl Pts',(34.426441263231,56.6995834937723,5.33510077749076));
#44117=CARTESIAN_POINT('Ctrl Pts',(33.2020675476878,58.1314028177064,5.44623866805879));
#44118=CARTESIAN_POINT('Ctrl Pts',(31.3350836476587,57.8792764730932,5.55737655862684));
#44119=CARTESIAN_POINT('Ctrl Pts',(30.5343604901146,56.173979132908,5.66851444919488));
#44120=CARTESIAN_POINT('Ctrl Pts',(31.5328102757061,54.5763876565426,5.77965233976292));
#44121=CARTESIAN_POINT('Ctrl Pts',(33.4165381765593,54.5487979003783,5.89079023033096));
#44122=CARTESIAN_POINT('Ctrl Pts',(34.4613514910016,56.116458582309,6.001928120899));
#44123=CARTESIAN_POINT('Ctrl Pts',(33.7109111712192,57.8444810565579,6.11306601146705));
#44124=CARTESIAN_POINT('Ctrl Pts',(31.8521228057562,58.1511689306776,6.22420390203508));
#44125=CARTESIAN_POINT('Ctrl Pts',(30.5863185401119,56.7558427953566,6.33534179260314));
#44126=CARTESIAN_POINT('Ctrl Pts',(31.07217886447,54.9355898635396,6.44647968317117));
#44127=CARTESIAN_POINT('Ctrl Pts',(32.8648400497806,54.3566488617232,6.55761757373922));
#44128=CARTESIAN_POINT('Ctrl Pts',(34.3237580856512,55.5486512349918,6.66875546430725));
#44129=CARTESIAN_POINT('Ctrl Pts',(34.1129733567612,57.4211007417247,6.7798933548753));
#44130=CARTESIAN_POINT('Ctrl Pts',(32.4266050042152,58.2590134407084,6.89103124544334));
#44131=CARTESIAN_POINT('Ctrl Pts',(30.805840812616,57.2976582429663,7.00216913601138));
#44132=CARTESIAN_POINT('Ctrl Pts',(30.7389488982073,55.4124226867889,7.11330702657943));
#44133=CARTESIAN_POINT('Ctrl Pts',(31.764281276621,54.697545560418,7.18739895362479));
#44134=CARTESIAN_POINT('Ctrl Pts',(32.3148335773693,54.6359733196,7.22444491714747));
#44135=CARTESIAN_POINT('Ctrl Pts',(30.8086516228787,55.6887746631347,-2.07481497238249));
#44136=CARTESIAN_POINT('Ctrl Pts',(31.0091224297109,55.1263610888822,-2.03776900885981));
#44137=CARTESIAN_POINT('Ctrl Pts',(32.01217730928,54.2270656189395,-1.96367708181445));
#44138=CARTESIAN_POINT('Ctrl Pts',(33.97355427561,54.7625083704828,-1.85253919124641));
#44139=CARTESIAN_POINT('Ctrl Pts',(34.5821615821015,56.7001809895466,-1.74140130067836));
#44140=CARTESIAN_POINT('Ctrl Pts',(33.2868853227587,58.2626346900185,-1.63026341011032));
#44141=CARTESIAN_POINT('Ctrl Pts',(31.2703940512689,58.021670508707,-1.51912551954228));
#44142=CARTESIAN_POINT('Ctrl Pts',(30.3798618750492,56.1968758041265,-1.40798762897424));
#44143=CARTESIAN_POINT('Ctrl Pts',(31.4296716306029,54.4589930404121,-1.2968497384062));
#44144=CARTESIAN_POINT('Ctrl Pts',(33.4592879307893,54.3984812756124,-1.18571184783816));
#44145=CARTESIAN_POINT('Ctrl Pts',(34.6107953909719,56.0708505702161,-1.07457395727011));
#44146=CARTESIAN_POINT('Ctrl Pts',(33.83029889799,57.9453005715135,-0.963436066702072));
#44147=CARTESIAN_POINT('Ctrl Pts',(31.8321491599349,58.3061569687477,-0.85229817613403));
#44148=CARTESIAN_POINT('Ctrl Pts',(30.4452986954797,56.8231082184979,-0.741160285565988));
#44149=CARTESIAN_POINT('Ctrl Pts',(30.939135705398,54.853613493319,-0.630022394997946));
#44150=CARTESIAN_POINT('Ctrl Pts',(32.8616514807306,54.2003697157939,-0.518884504429905));
#44151=CARTESIAN_POINT('Ctrl Pts',(34.4531425620492,55.4613003006532,-0.407746613861863));
#44152=CARTESIAN_POINT('Ctrl Pts',(34.2569006046969,57.4822601904945,-0.296608723293822));
#44153=CARTESIAN_POINT('Ctrl Pts',(32.4525473488096,58.4134423778501,-0.185470832725779));
#44154=CARTESIAN_POINT('Ctrl Pts',(30.6916281685284,57.4025249956444,-0.0743329421577379));
#44155=CARTESIAN_POINT('Ctrl Pts',(30.5859321707133,55.3748123143236,0.0368049484103036));
#44156=CARTESIAN_POINT('Ctrl Pts',(32.2322041958065,54.1862926836609,0.147942838978346));
#44157=CARTESIAN_POINT('Ctrl Pts',(34.1235927415348,54.9248316321149,0.259080729546388));
#44158=CARTESIAN_POINT('Ctrl Pts',(34.5288884461575,56.9144360685965,0.370218620114429));
#44159=CARTESIAN_POINT('Ctrl Pts',(33.0771195428256,58.3339984967674,0.48135651068247));
#44160=CARTESIAN_POINT('Ctrl Pts',(31.0971065789877,57.8841773231595,0.592494401250512));
#44161=CARTESIAN_POINT('Ctrl Pts',(30.4011778722794,55.97669897132,0.703632291818555));
#44162=CARTESIAN_POINT('Ctrl Pts',(31.6263248618463,54.3575000079461,0.814770182386596));
#44163=CARTESIAN_POINT('Ctrl Pts',(33.6511566132586,54.5086516076904,0.925908072954639));
#44164=CARTESIAN_POINT('Ctrl Pts',(34.6223216616804,56.2918029968741,1.03704596352268));
#44165=CARTESIAN_POINT('Ctrl Pts',(33.6509016243366,58.0748154867945,1.14818385409072));
#44166=CARTESIAN_POINT('Ctrl Pts',(31.626048278158,58.2256775246255,1.25932174465876));
#44167=CARTESIAN_POINT('Ctrl Pts',(30.4011328542516,56.6063033762813,1.3704596352268));
#44168=CARTESIAN_POINT('Ctrl Pts',(31.0973343316293,54.6989245646766,1.48159752579485));
#44169=CARTESIAN_POINT('Ctrl Pts',(33.0774116025732,54.2493865472286,1.59273541636289));
#44170=CARTESIAN_POINT('Ctrl Pts',(34.5289774853909,55.6691565694111,1.70387330693093));
#44171=CARTESIAN_POINT('Ctrl Pts',(34.1233972656597,57.6587030286353,1.81501119749897));
#44172=CARTESIAN_POINT('Ctrl Pts',(32.2319031180934,58.396971487781,1.92614908806701));
#44173=CARTESIAN_POINT('Ctrl Pts',(30.5858010869615,57.2082164536586,2.03728697863506));
#44174=CARTESIAN_POINT('Ctrl Pts',(30.691787029426,55.1805188903994,2.1484248692031));
#44175=CARTESIAN_POINT('Ctrl Pts',(32.4528508103866,54.1698533733088,2.25956275977114));
#44176=CARTESIAN_POINT('Ctrl Pts',(34.2570707793086,55.1012935119064,2.37070065033918));
#44177=CARTESIAN_POINT('Ctrl Pts',(34.4530239373915,57.1222815840842,2.48183854090722));
#44178=CARTESIAN_POINT('Ctrl Pts',(32.8613521367821,58.3829842878143,2.59297643147526));
#44179=CARTESIAN_POINT('Ctrl Pts',(30.938930627364,57.7294661410314,2.7041143220433));
#44180=CARTESIAN_POINT('Ctrl Pts',(30.4453736184505,55.7598997148858,2.81525221261135));
#44181=CARTESIAN_POINT('Ctrl Pts',(31.8324394376172,54.2770514956311,2.92639010317939));
#44182=CARTESIAN_POINT('Ctrl Pts',(33.8305310101845,54.6381892749935,3.03752799374743));
#44183=CARTESIAN_POINT('Ctrl Pts',(34.610772459882,56.5127595479419,3.14866588431547));
#44184=CARTESIAN_POINT('Ctrl Pts',(33.4589999392618,58.1849468845734,3.25980377488351));
#44185=CARTESIAN_POINT('Ctrl Pts',(31.4294438984359,58.1241792517757,3.37094166545156));
#44186=CARTESIAN_POINT('Ctrl Pts',(30.3797799983044,56.3860779529991,3.4820795560196));
#44187=CARTESIAN_POINT('Ctrl Pts',(31.2707775106533,54.5615468184256,3.59321744658764));
#44188=CARTESIAN_POINT('Ctrl Pts',(33.2868963078361,54.3205998871158,3.70435533715568));
#44189=CARTESIAN_POINT('Ctrl Pts',(34.5827599904381,55.8837786178317,3.81549322772373));
#44190=CARTESIAN_POINT('Ctrl Pts',(33.9722498337018,57.8202877906762,3.92663111829177));
#44191=CARTESIAN_POINT('Ctrl Pts',(32.0141727077009,58.3576185982774,4.03776900885981));
#44192=CARTESIAN_POINT('Ctrl Pts',(30.5007788120545,57.0039460586119,4.14890689942785));
#44193=CARTESIAN_POINT('Ctrl Pts',(30.8172947423318,54.9983019990856,4.2600447899959));
#44194=CARTESIAN_POINT('Ctrl Pts',(32.6740098783534,54.1764751726168,4.37118268056393));
#44195=CARTESIAN_POINT('Ctrl Pts',(34.371451798864,55.2906929942526,4.48232057113198));
#44196=CARTESIAN_POINT('Ctrl Pts',(34.3559326650591,57.3210992545065,4.59345846170002));
#44197=CARTESIAN_POINT('Ctrl Pts',(32.6416573134427,58.4092400794901,4.70459635226806));
#44198=CARTESIAN_POINT('Ctrl Pts',(30.7977214198622,57.5591278267734,4.8157342428361));
#44199=CARTESIAN_POINT('Ctrl Pts',(30.511900408801,55.5488798920818,4.92687213340414));
#44200=CARTESIAN_POINT('Ctrl Pts',(32.0458095141462,54.2184989881246,5.03801002397218));
#44201=CARTESIAN_POINT('Ctrl Pts',(33.9954442941986,54.7856978830043,5.14914791454023));
#44202=CARTESIAN_POINT('Ctrl Pts',(34.576282007745,56.731312917807,5.26028580510826));
#44203=CARTESIAN_POINT('Ctrl Pts',(33.2566751425584,58.274500741577,5.37142369567632));
#44204=CARTESIAN_POINT('Ctrl Pts',(31.2444751578682,58.0027637294031,5.48256158624434));
#44205=CARTESIAN_POINT('Ctrl Pts',(30.38147086237,56.1648264650488,5.5936994768124));
#44206=CARTESIAN_POINT('Ctrl Pts',(31.4575811830052,54.4429725464192,5.70483736738043));
#44207=CARTESIAN_POINT('Ctrl Pts',(33.4878275355304,54.4132368283282,5.81597525794848));
#44208=CARTESIAN_POINT('Ctrl Pts',(34.6139075918673,56.1028319020359,5.92711314851651));
#44209=CARTESIAN_POINT('Ctrl Pts',(33.8050971891886,57.9652618866617,6.03825103908456));
#44210=CARTESIAN_POINT('Ctrl Pts',(31.8017301968603,58.2958042848038,6.1493889296526));
#44211=CARTESIAN_POINT('Ctrl Pts',(30.4374702672965,56.7919481304539,6.26052682022064));
#44212=CARTESIAN_POINT('Ctrl Pts',(30.961121348176,54.8301139006692,6.37166471078869));
#44213=CARTESIAN_POINT('Ctrl Pts',(32.893217714717,54.2061422236913,6.48280260135672));
#44214=CARTESIAN_POINT('Ctrl Pts',(34.4656120183837,55.4908598675899,6.59394049192477));
#44215=CARTESIAN_POINT('Ctrl Pts',(34.2384322187942,57.5089505799534,6.70507838249281));
#44216=CARTESIAN_POINT('Ctrl Pts',(32.4208962597951,58.4120370607959,6.81621627306085));
#44217=CARTESIAN_POINT('Ctrl Pts',(30.6740672263624,57.3759065863185,6.92735416362889));
#44218=CARTESIAN_POINT('Ctrl Pts',(30.6019723844373,55.344035311361,7.03849205419694));
#44219=CARTESIAN_POINT('Ctrl Pts',(31.70705625587,54.5735542468394,7.1125839812423));
#44220=CARTESIAN_POINT('Ctrl Pts',(32.3004311270297,54.5071928486349,7.14962994476498));
#44221=CARTESIAN_POINT('Ctrl Pts',(30.6865906990181,55.6452663749118,-2.14962994476498));
#44222=CARTESIAN_POINT('Ctrl Pts',(30.9015290467899,55.042264639525,-2.1125839812423));
#44223=CARTESIAN_POINT('Ctrl Pts',(31.9769722095413,54.0780689767127,-2.03849205419694));
#44224=CARTESIAN_POINT('Ctrl Pts',(34.0798974741329,54.6521534639338,-1.9273541636289));
#44225=CARTESIAN_POINT('Ctrl Pts',(34.7324266426746,56.7296636902118,-1.81621627306085));
#44226=CARTESIAN_POINT('Ctrl Pts',(33.3436731204516,58.4048762668258,-1.70507838249281));
#44227=CARTESIAN_POINT('Ctrl Pts',(31.1816560714909,58.1465222260471,-1.59394049192477));
#44228=CARTESIAN_POINT('Ctrl Pts',(30.2268561301985,56.1900360671749,-1.48280260135673));
#44229=CARTESIAN_POINT('Ctrl Pts',(31.3524283663706,54.3267340944024,-1.37166471078869));
#44230=CARTESIAN_POINT('Ctrl Pts',(33.5285176487258,54.261855327502,-1.26052682022064));
#44231=CARTESIAN_POINT('Ctrl Pts',(34.7631268910861,56.0549158669708,-1.1493889296526));
#44232=CARTESIAN_POINT('Ctrl Pts',(33.9263036683235,58.064640837035,-1.03825103908456));
#44233=CARTESIAN_POINT('Ctrl Pts',(31.7839518212659,58.4515394534968,-0.927113148516518));
#44234=CARTESIAN_POINT('Ctrl Pts',(30.2970153832539,56.8614623091951,-0.815975257948478));
#44235=CARTESIAN_POINT('Ctrl Pts',(30.8264915332113,54.7498334448017,-0.704837367380435));
#44236=CARTESIAN_POINT('Ctrl Pts',(32.8877510794003,54.0494464884559,-0.593699476812394));
#44237=CARTESIAN_POINT('Ctrl Pts',(34.5940966013115,55.4013756837693,-0.482561586244352));
#44238=CARTESIAN_POINT('Ctrl Pts',(34.3836922898643,57.5681838415229,-0.371423695676311));
#44239=CARTESIAN_POINT('Ctrl Pts',(32.4491227944586,58.5665674166047,-0.260285805108268));
#44240=CARTESIAN_POINT('Ctrl Pts',(30.5611219171738,57.4826943315479,-0.149147914540227));
#44241=CARTESIAN_POINT('Ctrl Pts',(30.4477980696997,55.3086460480807,-0.0380100239721852));
#44242=CARTESIAN_POINT('Ctrl Pts',(32.2128779566306,54.0343535476132,0.0731278665958569));
#44243=CARTESIAN_POINT('Ctrl Pts',(34.2407638889375,54.826191241361,0.184265757163899));
#44244=CARTESIAN_POINT('Ctrl Pts',(34.6753089006883,56.9593810910663,0.29540364773194));
#44245=CARTESIAN_POINT('Ctrl Pts',(33.1187690016409,58.4813902438765,0.406541538299981));
#44246=CARTESIAN_POINT('Ctrl Pts',(30.9958628202428,57.9991064571457,0.517679428868024));
#44247=CARTESIAN_POINT('Ctrl Pts',(30.2497104564626,55.9539695525095,0.628817319436065));
#44248=CARTESIAN_POINT('Ctrl Pts',(31.5632736324487,54.2179165311208,0.739955210004108));
#44249=CARTESIAN_POINT('Ctrl Pts',(33.7342330755791,54.379976412185,0.851093100572149));
#44250=CARTESIAN_POINT('Ctrl Pts',(34.7754849876149,56.2918139484046,0.962230991140192));
#44251=CARTESIAN_POINT('Ctrl Pts',(33.7339596846626,58.2035025613039,1.07336888170823));
#44252=CARTESIAN_POINT('Ctrl Pts',(31.5629770883188,58.3652519834031,1.18450677227628));
#44253=CARTESIAN_POINT('Ctrl Pts',(30.2496621895819,56.6290111343267,1.29564466284432));
#44254=CARTESIAN_POINT('Ctrl Pts',(30.996107009296,54.5839809535271,1.40678255341236));
#44255=CARTESIAN_POINT('Ctrl Pts',(33.1190821387036,54.1020007577187,1.5179204439804));
#44256=CARTESIAN_POINT('Ctrl Pts',(34.675404365689,55.6242324861475,1.62905833454844));
#44257=CARTESIAN_POINT('Ctrl Pts',(34.2405543059947,57.7573601745033,1.74019622511648));
#44258=CARTESIAN_POINT('Ctrl Pts',(32.2125551507957,58.5489078583191,1.85133411568452));
#44259=CARTESIAN_POINT('Ctrl Pts',(30.4476575259193,57.274362965838,1.96247200625257));
#44260=CARTESIAN_POINT('Ctrl Pts',(30.5612922427159,55.1003308914695,2.07360989682061));
#44261=CARTESIAN_POINT('Ctrl Pts',(32.4494481561958,54.0167278480842,2.18474778738865));
#44262=CARTESIAN_POINT('Ctrl Pts',(34.3838747456067,55.0153879901866,2.29588567795669));
#44263=CARTESIAN_POINT('Ctrl Pts',(34.593969415771,57.1822263641343,2.40702356852473));
#44264=CARTESIAN_POINT('Ctrl Pts',(32.8874301324519,58.5339112326344,2.51816145909278));
#44265=CARTESIAN_POINT('Ctrl Pts',(30.8262716551429,57.8332301063997,2.62929934966082));
#44266=CARTESIAN_POINT('Ctrl Pts',(30.2970957132522,55.7215243665374,2.74043724022886));
#44267=CARTESIAN_POINT('Ctrl Pts',(31.7842630476554,54.1316622251152,2.8515751307969));
#44268=CARTESIAN_POINT('Ctrl Pts',(33.9265525315489,54.5188625304399,2.96271302136494));
#44269=CARTESIAN_POINT('Ctrl Pts',(34.7631023051095,56.5287164518977,3.07385091193299));
#44270=CARTESIAN_POINT('Ctrl Pts',(33.5282088734779,58.3215819018844,3.18498880250102));
#44271=CARTESIAN_POINT('Ctrl Pts',(31.3521841992698,58.2564288015506,3.29612669306907));
#44272=CARTESIAN_POINT('Ctrl Pts',(30.2267683445876,56.3928925225169,3.40726458363711));
#44273=CARTESIAN_POINT('Ctrl Pts',(31.1820672043028,54.4366889549244,3.51840247420515));
#44274=CARTESIAN_POINT('Ctrl Pts',(33.343684898298,54.1783534090425,3.62954036477319));
#44275=CARTESIAN_POINT('Ctrl Pts',(34.7330682368358,55.8543433397519,3.74067825534124));
#44276=CARTESIAN_POINT('Ctrl Pts',(34.0784988934969,57.9306061564344,3.85181614590927));
#44277=CARTESIAN_POINT('Ctrl Pts',(31.9791116115147,58.5067149566014,3.96295403647732));
#44278=CARTESIAN_POINT('Ctrl Pts',(30.3564993788501,57.0553508218565,4.07409192704536));
#44279=CARTESIAN_POINT('Ctrl Pts',(30.6958575735531,54.9049638044908,4.18522981761341));
#44280=CARTESIAN_POINT('Ctrl Pts',(32.686567791791,54.0238275282073,4.29636770818144));
#44281=CARTESIAN_POINT('Ctrl Pts',(34.5065103938996,55.2184560201287,4.40750559874949));
#44282=CARTESIAN_POINT('Ctrl Pts',(34.4898712780524,57.3953922722465,4.51864348931753));
#44283=CARTESIAN_POINT('Ctrl Pts',(32.6518804128256,58.5620618475365,4.62978137988557));
#44284=CARTESIAN_POINT('Ctrl Pts',(30.6748716870867,57.650598847478,4.74091927045361));
#44285=CARTESIAN_POINT('Ctrl Pts',(30.3684235969797,55.4952757033166,4.85205716102166));
#44286=CARTESIAN_POINT('Ctrl Pts',(32.0130315772872,54.068884110834,4.96319505158969));
#44287=CARTESIAN_POINT('Ctrl Pts',(34.103367247625,54.677016513002,5.07433294215774));
#44288=CARTESIAN_POINT('Ctrl Pts',(34.726122752259,56.7630423418418,5.18547083272577));
#44289=CARTESIAN_POINT('Ctrl Pts',(33.3112827374291,58.4175986654477,5.29660872329383));
#44290=CARTESIAN_POINT('Ctrl Pts',(31.1538666680778,58.126250985713,5.40774661386186));
#44291=CARTESIAN_POINT('Ctrl Pts',(30.2285812346253,56.1556737971897,5.51888450442991));
#44292=CARTESIAN_POINT('Ctrl Pts',(31.3823520903042,54.3095574362957,5.63002239499793));
#44293=CARTESIAN_POINT('Ctrl Pts',(33.5591168945015,54.2776757562781,5.741160285566));
#44294=CARTESIAN_POINT('Ctrl Pts',(34.766463692733,56.0892052217627,5.85229817613402));
#44295=CARTESIAN_POINT('Ctrl Pts',(33.8992832071581,58.0860427167655,5.96343606670208));
#44296=CARTESIAN_POINT('Ctrl Pts',(31.7513375879643,58.4404396389301,6.0745739572701));
#44297=CARTESIAN_POINT('Ctrl Pts',(30.288621994481,56.8280534655513,6.18571184783816));
#44298=CARTESIAN_POINT('Ctrl Pts',(30.850063831882,54.7246379377987,6.29684973840619));
#44299=CARTESIAN_POINT('Ctrl Pts',(32.9215953796534,54.0556355856594,6.40798762897423));
#44300=CARTESIAN_POINT('Ctrl Pts',(34.6074659511161,55.433068500188,6.51912551954228));
#44301=CARTESIAN_POINT('Ctrl Pts',(34.3638910808273,57.5968004181821,6.63026341011032));
#44302=CARTESIAN_POINT('Ctrl Pts',(32.4151875153751,58.5650606808835,6.74140130067835));
#44303=CARTESIAN_POINT('Ctrl Pts',(30.5422936401087,57.4541549296709,6.85253919124641));
#44304=CARTESIAN_POINT('Ctrl Pts',(30.4649958706675,55.2756479359331,6.96367708181444));
#44305=CARTESIAN_POINT('Ctrl Pts',(31.649831235119,54.4495629332609,7.03776900885981));
#44306=CARTESIAN_POINT('Ctrl Pts',(32.28602867669,54.3784123776698,7.07481497238249));
#44307=CARTESIAN_POINT('Ctrl Pts',(30.5645297751575,55.601758086689,-2.22444491714747));
#44308=CARTESIAN_POINT('Ctrl Pts',(30.7939356638689,54.9581681901677,-2.18739895362479));
#44309=CARTESIAN_POINT('Ctrl Pts',(31.9417671098026,53.9290723344859,-2.11330702657942));
#44310=CARTESIAN_POINT('Ctrl Pts',(34.1862406726559,54.5417985573848,-2.00216913601139));
#44311=CARTESIAN_POINT('Ctrl Pts',(34.8826917032476,56.7591463908769,-1.89103124544334));
#44312=CARTESIAN_POINT('Ctrl Pts',(33.4004609181445,58.5471178436331,-1.7798933548753));
#44313=CARTESIAN_POINT('Ctrl Pts',(31.0929180917129,58.2713739433872,-1.66875546430726));
#44314=CARTESIAN_POINT('Ctrl Pts',(30.0738503853477,56.1831963302234,-1.55761757373922));
#44315=CARTESIAN_POINT('Ctrl Pts',(31.2751851021384,54.1944751483927,-1.44647968317118));
#44316=CARTESIAN_POINT('Ctrl Pts',(33.5977473666623,54.1252293793916,-1.33534179260313));
#44317=CARTESIAN_POINT('Ctrl Pts',(34.9154583912003,56.0389811637256,-1.22420390203509));
#44318=CARTESIAN_POINT('Ctrl Pts',(34.0223084386569,58.1839811025564,-1.11306601146705));
#44319=CARTESIAN_POINT('Ctrl Pts',(31.7357544825969,58.596921938246,-1.00192812089901));
#44320=CARTESIAN_POINT('Ctrl Pts',(30.1487320710281,56.8998163998922,-0.890790230330966));
#44321=CARTESIAN_POINT('Ctrl Pts',(30.7138473610246,54.6460533962845,-0.779652339762924));
#44322=CARTESIAN_POINT('Ctrl Pts',(32.9138506780699,53.8985232611178,-0.668514449194883));
#44323=CARTESIAN_POINT('Ctrl Pts',(34.7350506405739,55.3414510668855,-0.55737655862684));
#44324=CARTESIAN_POINT('Ctrl Pts',(34.5104839750318,57.654107492551,-0.4462386680588));
#44325=CARTESIAN_POINT('Ctrl Pts',(32.4456982401076,58.7196924553593,-0.335100777490757));
#44326=CARTESIAN_POINT('Ctrl Pts',(30.4306156658191,57.5628636674516,-0.223962886922716));
#44327=CARTESIAN_POINT('Ctrl Pts',(30.309663968686,55.2424797818377,-0.112824996354674));
#44328=CARTESIAN_POINT('Ctrl Pts',(32.1935517174548,53.8824144115655,-0.00168710578663204));
#44329=CARTESIAN_POINT('Ctrl Pts',(34.3579350363403,54.7275508506072,0.10945078478141));
#44330=CARTESIAN_POINT('Ctrl Pts',(34.8217293552191,57.004326113536,0.220588675349451));
#44331=CARTESIAN_POINT('Ctrl Pts',(33.1604184604563,58.6287819909857,0.331726565917493));
#44332=CARTESIAN_POINT('Ctrl Pts',(30.894619061498,58.1140355911319,0.442864456485535));
#44333=CARTESIAN_POINT('Ctrl Pts',(30.0982430406458,55.931240133699,0.554002347053577));
#44334=CARTESIAN_POINT('Ctrl Pts',(31.5002224030512,54.0783330542954,0.665140237621618));
#44335=CARTESIAN_POINT('Ctrl Pts',(33.8173095378994,54.2513012166796,0.776278128189661));
#44336=CARTESIAN_POINT('Ctrl Pts',(34.9286483135496,56.2918248999351,0.887416018757702));
#44337=CARTESIAN_POINT('Ctrl Pts',(33.8170177449885,58.3321896358132,0.998553909325745));
#44338=CARTESIAN_POINT('Ctrl Pts',(31.4999058984797,58.5048264421807,1.10969179989378));
#44339=CARTESIAN_POINT('Ctrl Pts',(30.0981915249122,56.6517188923722,1.22082969046183));
#44340=CARTESIAN_POINT('Ctrl Pts',(30.8948796869627,54.4690373423775,1.33196758102987));
#44341=CARTESIAN_POINT('Ctrl Pts',(33.1607526748339,53.9546149682086,1.44310547159791));
#44342=CARTESIAN_POINT('Ctrl Pts',(34.8218312459871,55.5793084028842,1.55424336216595));
#44343=CARTESIAN_POINT('Ctrl Pts',(34.3577113463298,57.8560173203711,1.665381252734));
#44344=CARTESIAN_POINT('Ctrl Pts',(32.1932071834979,58.7008442288574,1.77651914330203));
#44345=CARTESIAN_POINT('Ctrl Pts',(30.3095139648772,57.3405094780172,1.88765703387008));
#44346=CARTESIAN_POINT('Ctrl Pts',(30.4307974560058,55.0201428925398,1.99879492443812));
#44347=CARTESIAN_POINT('Ctrl Pts',(32.4460455020051,53.8636023228594,2.10993281500616));
#44348=CARTESIAN_POINT('Ctrl Pts',(34.5106787119048,54.9294824684667,2.2210707055742));
#44349=CARTESIAN_POINT('Ctrl Pts',(34.7349148941506,57.2421711441843,2.33220859614224));
#44350=CARTESIAN_POINT('Ctrl Pts',(32.9135081281216,58.6848381774545,2.44334648671029));
#44351=CARTESIAN_POINT('Ctrl Pts',(30.7136126829218,57.9369940717681,2.55448437727833));
#44352=CARTESIAN_POINT('Ctrl Pts',(30.1488178080538,55.6831490181888,2.66562226784637));
#44353=CARTESIAN_POINT('Ctrl Pts',(31.7360866576937,53.9862729545993,2.77676015841441));
#44354=CARTESIAN_POINT('Ctrl Pts',(34.0225740529132,54.3995357858862,2.88789804898245));
#44355=CARTESIAN_POINT('Ctrl Pts',(34.9154321503369,56.5446733558537,2.9990359395505));
#44356=CARTESIAN_POINT('Ctrl Pts',(33.5974178076939,58.4582169191954,3.11017383011853));
#44357=CARTESIAN_POINT('Ctrl Pts',(31.2749245001037,58.3886783513255,3.22131172068658));
#44358=CARTESIAN_POINT('Ctrl Pts',(30.0737566908708,56.3997070920348,3.33244961125462));
#44359=CARTESIAN_POINT('Ctrl Pts',(31.0933568979523,54.3118310914232,3.44358750182266));
#44360=CARTESIAN_POINT('Ctrl Pts',(33.40047348876,54.0361069309691,3.5547253923907));
#44361=CARTESIAN_POINT('Ctrl Pts',(34.8833764832335,55.8249080616723,3.66586328295875));
#44362=CARTESIAN_POINT('Ctrl Pts',(34.1847479532921,58.0409245221924,3.77700117352678));
#44363=CARTESIAN_POINT('Ctrl Pts',(31.9440505153284,58.6558113149256,3.88813906409484));
#44364=CARTESIAN_POINT('Ctrl Pts',(30.2122199456457,57.1067555851009,3.99927695466286));
#44365=CARTESIAN_POINT('Ctrl Pts',(30.5744204047745,54.811625609896,4.11041484523092));
#44366=CARTESIAN_POINT('Ctrl Pts',(32.6991257052286,53.8711798837977,4.22155273579895));
#44367=CARTESIAN_POINT('Ctrl Pts',(34.6415689889353,55.1462190460046,4.332690626367));
#44368=CARTESIAN_POINT('Ctrl Pts',(34.6238098910458,57.4696852899866,4.44382851693504));
#44369=CARTESIAN_POINT('Ctrl Pts',(32.6621035122085,58.7148836155828,4.55496640750308));
#44370=CARTESIAN_POINT('Ctrl Pts',(30.5520219543112,57.7420698681825,4.66610429807112));
#44371=CARTESIAN_POINT('Ctrl Pts',(30.2249467851584,55.4416715145514,4.77724218863916));
#44372=CARTESIAN_POINT('Ctrl Pts',(31.980253640428,53.9192692335435,4.8883800792072));
#44373=CARTESIAN_POINT('Ctrl Pts',(34.2112902010514,54.5683351429997,4.99951796977525));
#44374=CARTESIAN_POINT('Ctrl Pts',(34.8759634967729,56.7947717658766,5.11065586034329));
#44375=CARTESIAN_POINT('Ctrl Pts',(33.3658903322998,58.5606965893184,5.22179375091133));
#44376=CARTESIAN_POINT('Ctrl Pts',(31.0632581782873,58.2497382420229,5.33293164147937));
#44377=CARTESIAN_POINT('Ctrl Pts',(30.0756916068806,56.1465211293306,5.44406953204742));
#44378=CARTESIAN_POINT('Ctrl Pts',(31.3071229976033,54.1761423261722,5.55520742261545));
#44379=CARTESIAN_POINT('Ctrl Pts',(33.6304062534725,54.1421146842281,5.6663453131835));
#44380=CARTESIAN_POINT('Ctrl Pts',(34.9190197935988,56.0755785414894,5.77748320375153));
#44381=CARTESIAN_POINT('Ctrl Pts',(33.9934692251276,58.2068235468693,5.88862109431959));
#44382=CARTESIAN_POINT('Ctrl Pts',(31.7009449790683,58.5850749930563,5.99975898488761));
#44383=CARTESIAN_POINT('Ctrl Pts',(30.1397737216656,56.8641588006487,6.11089687545567));
#44384=CARTESIAN_POINT('Ctrl Pts',(30.7390063155881,54.6191619749282,6.2220347660237));
#44385=CARTESIAN_POINT('Ctrl Pts',(32.9499730445898,53.9051289476276,6.33317265659175));
#44386=CARTESIAN_POINT('Ctrl Pts',(34.7493198838486,55.375277132786,6.44431054715978));
#44387=CARTESIAN_POINT('Ctrl Pts',(34.4893499428603,57.684650256411,6.55544843772784));
#44388=CARTESIAN_POINT('Ctrl Pts',(32.409478770955,58.718084300971,6.66658632829587));
#44389=CARTESIAN_POINT('Ctrl Pts',(30.4105200538552,57.5324032730233,6.77772421886391));
#44390=CARTESIAN_POINT('Ctrl Pts',(30.3280193568976,55.2072605605051,6.88886210943196));
#44391=CARTESIAN_POINT('Ctrl Pts',(31.592606214368,54.3255716196824,6.96295403647732));
#44392=CARTESIAN_POINT('Ctrl Pts',(32.2716262263503,54.2496319067047,7.));
#44393=CARTESIAN_POINT('Ctrl Pts',(30.9307125467392,55.7322829513575,-2.));
#44394=CARTESIAN_POINT('Ctrl Pts',(30.9446699885302,55.6718824515121,-2.));
#44395=CARTESIAN_POINT('Ctrl Pts',(30.9622173189429,55.6125616548499,-2.));
#44396=CARTESIAN_POINT('Ctrl Pts',(30.9830550110871,55.5544917980879,-2.));
#44397=CARTESIAN_POINT('Ctrl Pts',(31.0052689439607,55.4925866748543,-2.));
#44398=CARTESIAN_POINT('Ctrl Pts',(31.031222059362,55.4321024422535,-2.));
#44399=CARTESIAN_POINT('Ctrl Pts',(31.0606132871183,55.373244167107,-2.));
#44400=CARTESIAN_POINT('Ctrl Pts',(31.0863306114051,55.3217431763537,-2.));
#44401=CARTESIAN_POINT('Ctrl Pts',(31.1146814237683,55.271486657179,-2.));
#44402=CARTESIAN_POINT('Ctrl Pts',(31.1454993456467,55.2226180386923,-2.));
#44403=CARTESIAN_POINT('Ctrl Pts',(31.1609623517183,55.1980980289605,-2.));
#44404=CARTESIAN_POINT('Ctrl Pts',(31.1770469579252,55.1739275671393,-2.));
#44405=CARTESIAN_POINT('Ctrl Pts',(31.1937349146798,55.1501258793134,-2.));
#44406=CARTESIAN_POINT('Ctrl Pts',(31.201357838137,55.1392534611306,-2.));
#44407=CARTESIAN_POINT('Ctrl Pts',(31.2091078133333,55.1284566647485,-2.));
#44408=CARTESIAN_POINT('Ctrl Pts',(31.2169701001442,55.1177546356172,-2.));
#44409=CARTESIAN_POINT('Ctrl Pts',(31.2566258561271,55.0637758040171,-2.));
#44410=CARTESIAN_POINT('Ctrl Pts',(31.2992033789151,55.0121067330646,-2.));
#44411=CARTESIAN_POINT('Ctrl Pts',(31.3444046039735,54.9629466687563,-2.));
#44412=CARTESIAN_POINT('Ctrl Pts',(31.3904074837357,54.9129147387687,-2.));
#44413=CARTESIAN_POINT('Ctrl Pts',(31.4391284050012,54.8654806967995,-2.));
#44414=CARTESIAN_POINT('Ctrl Pts',(31.4903044396858,54.8208703724848,-2.));
#44415=CARTESIAN_POINT('Ctrl Pts',(31.5331115544079,54.7835552642998,-2.));
#44416=CARTESIAN_POINT('Ctrl Pts',(31.5776375521365,54.7482158610042,-2.));
#44417=CARTESIAN_POINT('Ctrl Pts',(31.6237516110946,54.7149996928349,-2.));
#44418=CARTESIAN_POINT('Ctrl Pts',(31.6449987764552,54.6996952621757,-2.));
#44419=CARTESIAN_POINT('Ctrl Pts',(31.666583341519,54.684841812932,-2.));
#44420=CARTESIAN_POINT('Ctrl Pts',(31.6884937600232,54.6704551374775,-2.));
#44421=CARTESIAN_POINT('Ctrl Pts',(31.6980569752198,54.6641758017675,-2.));
#44422=CARTESIAN_POINT('Ctrl Pts',(31.7076821201642,54.6579856105882,-2.));
#44423=CARTESIAN_POINT('Ctrl Pts',(31.7173562110341,54.6518932017638,-2.));
#44424=CARTESIAN_POINT('Ctrl Pts',(31.7767391575644,54.6144958698259,-2.));
#44425=CARTESIAN_POINT('Ctrl Pts',(31.8380740161593,54.5807067449847,-2.));
#44426=CARTESIAN_POINT('Ctrl Pts',(31.9010756695341,54.5507535434866,-2.));
#44427=CARTESIAN_POINT('Ctrl Pts',(31.9574042849217,54.5239729389083,-2.));
#44428=CARTESIAN_POINT('Ctrl Pts',(32.0150663148412,54.5002585220861,-2.));
#44429=CARTESIAN_POINT('Ctrl Pts',(32.073885064195,54.4797956759537,-2.));
#44430=CARTESIAN_POINT('Ctrl Pts',(32.1379640249064,54.4575028198872,-2.));
#44431=CARTESIAN_POINT('Ctrl Pts',(32.2034160279184,54.4390677641941,-2.));
#44432=CARTESIAN_POINT('Ctrl Pts',(32.2699334847327,54.4243849072974,-2.));
#44433=CARTESIAN_POINT('Ctrl Pts',(32.2955972920822,54.418719958143,-2.));
#44434=CARTESIAN_POINT('Ctrl Pts',(32.3214199362483,54.4136140552492,-2.));
#44435=CARTESIAN_POINT('Ctrl Pts',(32.3473844776328,54.4090630310332,-2.));
#44436=CARTESIAN_POINT('Ctrl Pts',(32.3587747917572,54.4070665545832,-2.));
#44437=CARTESIAN_POINT('Ctrl Pts',(32.370191852042,54.4051770614586,-2.));
#44438=CARTESIAN_POINT('Ctrl Pts',(32.3816208593905,54.4033960585417,-2.));
#44439=CARTESIAN_POINT('Ctrl Pts',(32.4507180638397,54.3926285160141,-2.));
#44440=CARTESIAN_POINT('Ctrl Pts',(32.5203743381692,54.3858000563277,-2.));
#44441=CARTESIAN_POINT('Ctrl Pts',(32.5902438513676,54.3827492853088,-2.));
#44442=CARTESIAN_POINT('Ctrl Pts',(32.6617320285806,54.3796278372087,-2.));
#44443=CARTESIAN_POINT('Ctrl Pts',(32.7334442999622,54.3804609924871,-2.));
#44444=CARTESIAN_POINT('Ctrl Pts',(32.8050350906587,54.3851263529449,-2.));
#44445=CARTESIAN_POINT('Ctrl Pts',(32.8598101377162,54.3886958810382,-2.));
#44446=CARTESIAN_POINT('Ctrl Pts',(32.9145147054626,54.3945098111843,-2.));
#44447=CARTESIAN_POINT('Ctrl Pts',(32.9689984939366,54.4025332699551,-2.));
#44448=CARTESIAN_POINT('Ctrl Pts',(33.0029113987617,54.4075273939191,-2.));
#44449=CARTESIAN_POINT('Ctrl Pts',(33.036738821977,54.4133779008128,-2.));
#44450=CARTESIAN_POINT('Ctrl Pts',(33.0704445092544,54.4200797350036,-2.));
#44451=CARTESIAN_POINT('Ctrl Pts',(33.089353388944,54.4238394618227,-2.));
#44452=CARTESIAN_POINT('Ctrl Pts',(33.1082301633356,54.427868732682,-2.));
#44453=CARTESIAN_POINT('Ctrl Pts',(33.1270344168394,54.4321588085794,-2.));
#44454=CARTESIAN_POINT('Ctrl Pts',(33.1999617463517,54.4487967345966,-2.));
#44455=CARTESIAN_POINT('Ctrl Pts',(33.2718735596778,54.4693655783697,-2.));
#44456=CARTESIAN_POINT('Ctrl Pts',(33.3423988007245,54.4937504954065,-2.));
#44457=CARTESIAN_POINT('Ctrl Pts',(33.3951487097983,54.5119893860131,-2.));
#44458=CARTESIAN_POINT('Ctrl Pts',(33.4471233202134,54.5323642451401,-2.));
#44459=CARTESIAN_POINT('Ctrl Pts',(33.4981671222966,54.5548460976078,-2.));
#44460=CARTESIAN_POINT('Ctrl Pts',(33.5140901369429,54.5618592676991,-2.));
#44461=CARTESIAN_POINT('Ctrl Pts',(33.5299225528842,54.5690775909089,-2.));
#44462=CARTESIAN_POINT('Ctrl Pts',(33.5456595741859,54.5765005080531,-2.));
#44463=CARTESIAN_POINT('Ctrl Pts',(33.5608498129668,54.5836655160752,-2.));
#44464=CARTESIAN_POINT('Ctrl Pts',(33.5759433894836,54.5910175352326,-2.));
#44465=CARTESIAN_POINT('Ctrl Pts',(33.5909308710043,54.5985527495203,-2.));
#44466=CARTESIAN_POINT('Ctrl Pts',(33.6582318432482,54.6323894716492,-2.));
#44467=CARTESIAN_POINT('Ctrl Pts',(33.7234283245458,54.6699323219049,-2.));
#44468=CARTESIAN_POINT('Ctrl Pts',(33.7861478874081,54.7110945661111,-2.));
#44469=CARTESIAN_POINT('Ctrl Pts',(33.8341488046729,54.7425971051658,-2.));
#44470=CARTESIAN_POINT('Ctrl Pts',(33.8806990672136,54.7762206567448,-2.));
#44471=CARTESIAN_POINT('Ctrl Pts',(33.9256254254142,54.8119460488582,-2.));
#44472=CARTESIAN_POINT('Ctrl Pts',(33.9360516193134,54.8202369471242,-2.));
#44473=CARTESIAN_POINT('Ctrl Pts',(33.9463903172992,54.8286411175249,-2.));
#44474=CARTESIAN_POINT('Ctrl Pts',(33.9566410663199,54.8371566128168,-2.));
#44475=CARTESIAN_POINT('Ctrl Pts',(33.3347877909358,57.7349452754743,-0.871480363390197));
#44476=CARTESIAN_POINT('Ctrl Pts',(33.4089783616458,57.6929560180431,-0.877193940366654));
#44477=CARTESIAN_POINT('Ctrl Pts',(33.4797275640263,57.6452118511612,-0.882907517343111));
#44478=CARTESIAN_POINT('Ctrl Pts',(33.5459978166813,57.5919001635713,-0.888621094319568));
#44479=CARTESIAN_POINT('Ctrl Pts',(33.9756840487236,57.2462352951484,-0.925667057842249));
#44480=CARTESIAN_POINT('Ctrl Pts',(34.2170739697906,56.6665102843049,-0.96271302136493));
#44481=CARTESIAN_POINT('Ctrl Pts',(34.1597013173233,56.1180347705934,-0.99975898488761));
#44482=CARTESIAN_POINT('Ctrl Pts',(34.102328664856,55.5695592568819,-1.03680494841029));
#44483=CARTESIAN_POINT('Ctrl Pts',(33.7461934388544,55.0523332403023,-1.07385091193297));
#44484=CARTESIAN_POINT('Ctrl Pts',(33.254268606184,54.8030776924624,-1.11089687545565));
#44485=CARTESIAN_POINT('Ctrl Pts',(32.7623437735136,54.5538221446225,-1.14794283897833));
#44486=CARTESIAN_POINT('Ctrl Pts',(32.1346293341744,54.5725370655222,-1.18498880250101));
#44487=CARTESIAN_POINT('Ctrl Pts',(31.6584309020156,54.8506384517481,-1.22203476602369));
#44488=CARTESIAN_POINT('Ctrl Pts',(31.1822324698568,55.1287398379739,-1.25908072954638));
#44489=CARTESIAN_POINT('Ctrl Pts',(30.8575500448783,55.666227689526,-1.29612669306906));
#44490=CARTESIAN_POINT('Ctrl Pts',(30.8329195675803,56.2171554903502,-1.33317265659174));
#44491=CARTESIAN_POINT('Ctrl Pts',(30.8082890902823,56.7680832911743,-1.37021862011442));
#44492=CARTESIAN_POINT('Ctrl Pts',(31.0837105606646,57.3324510412706,-1.4072645836371));
#44493=CARTESIAN_POINT('Ctrl Pts',(31.5332488781922,57.6518973032928,-1.44431054715978));
#44494=CARTESIAN_POINT('Ctrl Pts',(31.9827871957199,57.971343565315,-1.48135651068246));
#44495=CARTESIAN_POINT('Ctrl Pts',(32.6064423603928,58.0458683392631,-1.51840247420514));
#44496=CARTESIAN_POINT('Ctrl Pts',(33.1185697754731,57.8415149221822,-1.55544843772782));
#44497=CARTESIAN_POINT('Ctrl Pts',(33.1924454681488,57.8120364178238,-1.56079241294861));
#44498=CARTESIAN_POINT('Ctrl Pts',(33.2640004019439,57.7767547923516,-1.56613638816941));
#44499=CARTESIAN_POINT('Ctrl Pts',(33.332685602761,57.7363329907929,-1.5714803633902));
#44500=CARTESIAN_POINT('Ctrl Pts',(34.4842965055667,55.7582049595679,-2.));
#44501=CARTESIAN_POINT('Ctrl Pts',(34.6616800870191,56.4180307560557,-1.96295403647732));
#44502=CARTESIAN_POINT('Ctrl Pts',(34.3029408546812,57.9173199920237,-1.88886210943196));
#44503=CARTESIAN_POINT('Ctrl Pts',(32.1083909227282,58.6899905331758,-1.77772421886392));
#44504=CARTESIAN_POINT('Ctrl Pts',(30.2743670907292,57.2623912321518,-1.66658632829588));
#44505=CARTESIAN_POINT('Ctrl Pts',(30.4765028746713,54.9487367869863,-1.55544843772783));
#44506=CARTESIAN_POINT('Ctrl Pts',(32.5312595152502,53.8630292597192,-1.44431054715979));
#44507=CARTESIAN_POINT('Ctrl Pts',(34.5571577499754,55.0008883544572,-1.33317265659175));
#44508=CARTESIAN_POINT('Ctrl Pts',(34.7002397993375,57.3198853035068,-1.22203476602371));
#44509=CARTESIAN_POINT('Ctrl Pts',(32.8293553152893,58.6978846888631,-1.11089687545567));
#44510=CARTESIAN_POINT('Ctrl Pts',(30.6570393620672,57.873352597378,-0.999758984887625));
#44511=CARTESIAN_POINT('Ctrl Pts',(30.1715905180572,55.6011108576298,-0.888621094319582));
#44512=CARTESIAN_POINT('Ctrl Pts',(31.817369145763,53.960908709333,-0.777483203751541));
#44513=CARTESIAN_POINT('Ctrl Pts',(34.087963584719,54.4540716106361,-0.666345313183499));
#44514=CARTESIAN_POINT('Ctrl Pts',(34.9050789303496,56.6291869825843,-0.555207422615458));
#44515=CARTESIAN_POINT('Ctrl Pts',(33.5207972588595,58.4953545827796,-0.444069532047415));
#44516=CARTESIAN_POINT('Ctrl Pts',(31.2021687803137,58.344446263511,-0.332931641479374));
#44517=CARTESIAN_POINT('Ctrl Pts',(30.0714596841225,56.3145920190741,-0.221793750911332));
#44518=CARTESIAN_POINT('Ctrl Pts',(31.1636212068566,54.2637395061115,-0.110655860343291));
#44519=CARTESIAN_POINT('Ctrl Pts',(33.4789853310955,54.0690577668369,0.000482030224751639));
#44520=CARTESIAN_POINT('Ctrl Pts',(34.8982731111897,55.908740964546,0.111619920792793));
#44521=CARTESIAN_POINT('Ctrl Pts',(34.1223942983453,58.0989063257425,0.222757811360834));
#44522=CARTESIAN_POINT('Ctrl Pts',(31.8615195930587,58.6348705964901,0.333895701928877));
#44523=CARTESIAN_POINT('Ctrl Pts',(30.1850532410697,57.0260596319961,0.445033592496918));
#44524=CARTESIAN_POINT('Ctrl Pts',(30.6274839128385,54.7450363379153,0.55617148306496));
#44525=CARTESIAN_POINT('Ctrl Pts',(32.783849793945,53.8796472115696,0.667309373633002));
#44526=CARTESIAN_POINT('Ctrl Pts',(34.6804047400893,55.2219927306231,0.778447264201043));
#44527=CARTESIAN_POINT('Ctrl Pts',(34.5812104999016,57.5434088201914,0.889585154769087));
#44528=CARTESIAN_POINT('Ctrl Pts',(32.5770606867505,58.7190770058698,1.00072304533713));
#44529=CARTESIAN_POINT('Ctrl Pts',(30.5023763530244,57.672894864812,1.11186093590517));
#44530=CARTESIAN_POINT('Ctrl Pts',(30.2561395980005,55.3624447749947,1.22299882647321));
#44531=CARTESIAN_POINT('Ctrl Pts',(32.0637337160182,53.9025079060376,1.33413671704125));
#44532=CARTESIAN_POINT('Ctrl Pts',(34.2706473113688,54.6293810308449,1.44527460760929));
#44533=CARTESIAN_POINT('Ctrl Pts',(34.8568673421132,56.8777489350101,1.55641249817734));
#44534=CARTESIAN_POINT('Ctrl Pts',(33.2858199659299,58.5896549776087,1.66755038874538));
#44535=CARTESIAN_POINT('Ctrl Pts',(30.9955026631254,58.198172143523,1.77868827931342));
#44536=CARTESIAN_POINT('Ctrl Pts',(30.082268834923,56.0616291105053,1.88982616988146));
#44537=CARTESIAN_POINT('Ctrl Pts',(31.3820117610517,54.1356279467244,2.0009640604495));
#44538=CARTESIAN_POINT('Ctrl Pts',(33.7050620011388,54.1830593597268,2.11210195101754));
#44539=CARTESIAN_POINT('Ctrl Pts',(34.9251053252509,56.1605088392832,2.22323984158559));
#44540=CARTESIAN_POINT('Ctrl Pts',(33.925422242596,58.2579944509529,2.33437773215363));
#44541=CARTESIAN_POINT('Ctrl Pts',(31.6210340159052,58.5556638272701,2.44551562272167));
#44542=CARTESIAN_POINT('Ctrl Pts',(30.1211733226086,56.7810568122913,2.55665351328971));
#44543=CARTESIAN_POINT('Ctrl Pts',(30.7986796648578,54.558491332239,2.66779140385775));
#44544=CARTESIAN_POINT('Ctrl Pts',(33.0334238041474,53.9223067766118,2.7789292944258));
#44545=CARTESIAN_POINT('Ctrl Pts',(34.7799190860636,55.4548100839991,2.89006718499383));
#44546=CARTESIAN_POINT('Ctrl Pts',(34.4395785724648,57.7532835973794,3.00120507556188));
#44547=CARTESIAN_POINT('Ctrl Pts',(32.3239197951718,58.7139084434936,3.11234296612992));
#44548=CARTESIAN_POINT('Ctrl Pts',(30.3694292262435,57.4574138064661,3.22348085669796));
#44549=CARTESIAN_POINT('Ctrl Pts',(30.3650742488504,55.1338834771873,3.33461874726601));
#44550=CARTESIAN_POINT('Ctrl Pts',(32.3148410231894,53.870071116671,3.44575663783404));
#44551=CARTESIAN_POINT('Ctrl Pts',(34.4340859088485,54.822758511107,3.55689452840209));
#44552=CARTESIAN_POINT('Ctrl Pts',(34.7830400281131,57.1199400841538,3.66803241897013));
#44553=CARTESIAN_POINT('Ctrl Pts',(33.0423017182097,58.6589794901992,3.77917030953818));
#44554=CARTESIAN_POINT('Ctrl Pts',(30.8051884955116,58.0311765069792,3.89030820010621));
#44555=CARTESIAN_POINT('Ctrl Pts',(30.1193554633367,55.8111663248381,4.00144609067426));
#44556=CARTESIAN_POINT('Ctrl Pts',(31.6125533739245,54.0309494400521,4.11258398124229));
#44557=CARTESIAN_POINT('Ctrl Pts',(33.9180412456697,54.3199785564283,4.22372187181034));
#44558=CARTESIAN_POINT('Ctrl Pts',(34.9255798836093,56.4137020456761,4.33485976237838));
#44559=CARTESIAN_POINT('Ctrl Pts',(33.7129577460601,58.3957110541619,4.44599765294642));
#44560=CARTESIAN_POINT('Ctrl Pts',(31.390101627814,58.451850257884,4.55713554351446));
#44561=CARTESIAN_POINT('Ctrl Pts',(30.0831480764379,56.5307348090518,4.66827343408251));
#44562=CARTESIAN_POINT('Ctrl Pts',(30.9883665002516,54.3907834608547,4.77941132465054));
#44563=CARTESIAN_POINT('Ctrl Pts',(33.2772002083032,53.9907179590751,4.89054921521859));
#44564=CARTESIAN_POINT('Ctrl Pts',(34.8546537539781,55.6967227784588,5.00168710578663));
#44565=CARTESIAN_POINT('Ctrl Pts',(34.2768660104017,57.9472723924375,5.11282499635467));
#44566=CARTESIAN_POINT('Ctrl Pts',(32.0726926657226,58.6824131526073,5.22396288692271));
#44567=CARTESIAN_POINT('Ctrl Pts',(30.2596385516873,57.2292625110706,5.33510077749076));
#44568=CARTESIAN_POINT('Ctrl Pts',(30.4972127153845,54.9179054771161,5.44623866805879));
#44569=CARTESIAN_POINT('Ctrl Pts',(32.5679607208418,53.8639538597437,5.55737655862684));
#44570=CARTESIAN_POINT('Ctrl Pts',(34.5765036531329,55.0321005249752,5.66851444919487));
#44571=CARTESIAN_POINT('Ctrl Pts',(34.684398953168,57.3531295774156,5.77965233976293));
#44572=CARTESIAN_POINT('Ctrl Pts',(32.7928896947834,58.7025728310562,5.89079023033095));
#44573=CARTESIAN_POINT('Ctrl Pts',(30.6332940299706,57.8452774805726,6.00192812089902));
#44574=CARTESIAN_POINT('Ctrl Pts',(30.1823177935136,55.5659199366929,6.11306601146704));
#44575=CARTESIAN_POINT('Ctrl Pts',(31.8527378172473,53.9508533596396,6.2242039020351));
#44576=CARTESIAN_POINT('Ctrl Pts',(34.1156133119216,54.4783040835128,6.33534179260312));
#44577=CARTESIAN_POINT('Ctrl Pts',(34.8996815919165,56.6656147589771,6.44647968317118));
#44578=CARTESIAN_POINT('Ctrl Pts',(33.4873299906744,58.5104676737159,6.55761757373921));
#44579=CARTESIAN_POINT('Ctrl Pts',(31.1711925871668,58.3247407101007,6.66875546430726));
#44580=CARTESIAN_POINT('Ctrl Pts',(30.0714699489351,56.2774508415846,6.77989335487529));
#44581=CARTESIAN_POINT('Ctrl Pts',(31.1943253650081,54.2444600690086,6.89103124544334));
#44582=CARTESIAN_POINT('Ctrl Pts',(33.5128402220711,54.0826823257856,7.00216913601138));
#44583=CARTESIAN_POINT('Ctrl Pts',(34.903205848792,55.948145429959,7.11330702657943));
#44584=CARTESIAN_POINT('Ctrl Pts',(34.3645996631225,57.3926056844023,7.18739895362479));
#44585=CARTESIAN_POINT('Ctrl Pts',(33.8493101059358,57.841283396055,7.22444491714747));
#44586=CARTESIAN_POINT('Ctrl Pts',(34.3591563398468,55.7918468858113,-2.07481497238249));
#44587=CARTESIAN_POINT('Ctrl Pts',(34.5253531804484,56.4100605999883,-2.03776900885981));
#44588=CARTESIAN_POINT('Ctrl Pts',(34.189237929385,57.8147967775173,-1.96367708181445));
#44589=CARTESIAN_POINT('Ctrl Pts',(32.1330878491652,58.5387386537266,-1.8525391912464));
#44590=CARTESIAN_POINT('Ctrl Pts',(30.4147271983626,57.2011712670919,-1.74140130067837));
#44591=CARTESIAN_POINT('Ctrl Pts',(30.6041152374845,55.033428030193,-1.63026341011032));
#44592=CARTESIAN_POINT('Ctrl Pts',(32.5292881259403,54.0161909253172,-1.51912551954228));
#44593=CARTESIAN_POINT('Ctrl Pts',(34.4274225712752,55.0822906457469,-1.40798762897424));
#44594=CARTESIAN_POINT('Ctrl Pts',(34.561481114665,57.2550394601585,-1.2968497384062));
#44595=CARTESIAN_POINT('Ctrl Pts',(32.8085844382453,58.5461349624701,-1.18571184783816));
#44596=CARTESIAN_POINT('Ctrl Pts',(30.7732661452114,57.77360219784,-1.07457395727011));
#44597=CARTESIAN_POINT('Ctrl Pts',(30.3184322564853,55.6446599635185,-0.963436066702072));
#44598=CARTESIAN_POINT('Ctrl Pts',(31.860419434863,54.1078975824522,-0.852298176134029));
#44599=CARTESIAN_POINT('Ctrl Pts',(33.9878182558372,54.5699590394786,-0.741160285565988));
#44600=CARTESIAN_POINT('Ctrl Pts',(34.7534020135838,56.6079002051822,-0.630022394997946));
#44601=CARTESIAN_POINT('Ctrl Pts',(33.4564204191172,58.3563774692333,-0.518884504429904));
#44602=CARTESIAN_POINT('Ctrl Pts',(31.2840168375231,58.2149862216468,-0.407746613861862));
#44603=CARTESIAN_POINT('Ctrl Pts',(30.2246161991563,56.3131452533626,-0.296608723293821));
#44604=CARTESIAN_POINT('Ctrl Pts',(31.2479002766274,54.3916302777182,-0.185470832725779));
#44605=CARTESIAN_POINT('Ctrl Pts',(33.4172453712523,54.2092261920339,-0.0743329421577372));
#44606=CARTESIAN_POINT('Ctrl Pts',(34.7470254051468,55.9328892992031,0.0368049484103043));
#44607=CARTESIAN_POINT('Ctrl Pts',(34.0200775877185,57.9849313227406,0.147942838978346));
#44608=CARTESIAN_POINT('Ctrl Pts',(31.9017855229282,58.4870948699203,0.259080729546388));
#44609=CARTESIAN_POINT('Ctrl Pts',(30.3310459494339,56.9797439796362,0.37021862011443));
#44610=CARTESIAN_POINT('Ctrl Pts',(30.7455746179339,54.8425740019479,0.481356510682471));
#44611=CARTESIAN_POINT('Ctrl Pts',(32.7659487342222,54.0317608617915,0.592494401250513));
#44612=CARTESIAN_POINT('Ctrl Pts',(34.5428969584923,55.2894510179814,0.703632291818555));
#44613=CARTESIAN_POINT('Ctrl Pts',(34.4499584283865,57.4644664091972,0.814770182386596));
#44614=CARTESIAN_POINT('Ctrl Pts',(32.5722008348668,58.5659907805944,0.925908072954638));
#44615=CARTESIAN_POINT('Ctrl Pts',(30.6283569983197,57.5857863833556,1.03704596352268));
#44616=CARTESIAN_POINT('Ctrl Pts',(30.3976492271163,55.4210454183169,1.14818385409072));
#44617=CARTESIAN_POINT('Ctrl Pts',(32.0912469605975,54.0531798407264,1.25932174465876));
#44618=CARTESIAN_POINT('Ctrl Pts',(34.1589809866262,54.7342125263452,1.3704596352268));
#44619=CARTESIAN_POINT('Ctrl Pts',(34.7082309014681,56.8407865346196,1.48159752579485));
#44620=CARTESIAN_POINT('Ctrl Pts',(33.2362620291565,58.4447307855874,1.59273541636289));
#44621=CARTESIAN_POINT('Ctrl Pts',(31.0903841717777,58.07793691638,1.70387330693093));
#44622=CARTESIAN_POINT('Ctrl Pts',(30.234743668102,56.0761355152048,1.81501119749897));
#44623=CARTESIAN_POINT('Ctrl Pts',(31.4525179747664,54.2715981065311,1.92614908806701));
#44624=CARTESIAN_POINT('Ctrl Pts',(33.6290644583814,54.3160382453632,2.03728697863505));
#44625=CARTESIAN_POINT('Ctrl Pts',(34.7721654387779,56.1687793686431,2.1484248692031));
#44626=CARTESIAN_POINT('Ctrl Pts',(33.8355276249525,58.133986514719,2.25956275977114));
#44627=CARTESIAN_POINT('Ctrl Pts',(31.6764662300946,58.4128832958229,2.37070065033918));
#44628=CARTESIAN_POINT('Ctrl Pts',(30.2711946343393,56.7501923253058,2.48183854090722));
#44629=CARTESIAN_POINT('Ctrl Pts',(30.9059738661453,54.6677935046801,2.59297643147527));
#44630=CARTESIAN_POINT('Ctrl Pts',(32.9997832957543,54.0717300904732,2.7041143220433));
#44631=CARTESIAN_POINT('Ctrl Pts',(34.6361354068314,55.5075856855278,2.81525221261135));
#44632=CARTESIAN_POINT('Ctrl Pts',(34.3172585546125,57.6611053799801,2.92639010317939));
#44633=CARTESIAN_POINT('Ctrl Pts',(32.3350243382431,58.561148174924,3.03752799374743));
#44634=CARTESIAN_POINT('Ctrl Pts',(30.503794216031,57.3838946929671,3.14866588431547));
#44635=CARTESIAN_POINT('Ctrl Pts',(30.4997138863991,55.206898397108,3.25980377488352));
#44636=CARTESIAN_POINT('Ctrl Pts',(32.3265181213336,54.0227886857625,3.37094166545156));
#44637=CARTESIAN_POINT('Ctrl Pts',(34.3121122872296,54.9153946064446,3.4820795560196));
#44638=CARTESIAN_POINT('Ctrl Pts',(34.6390595258737,57.0677038371105,3.59321744658764));
#44639=CARTESIAN_POINT('Ctrl Pts',(33.0081013218997,58.5096833300926,3.70435533715569));
#44640=CARTESIAN_POINT('Ctrl Pts',(30.9120722157322,57.9214729022892,3.81549322772372));
#44641=CARTESIAN_POINT('Ctrl Pts',(30.2694914188265,55.8414682290596,3.92663111829177));
#44642=CARTESIAN_POINT('Ctrl Pts',(31.6685204219654,54.1735211766069,4.0377690088598));
#44643=CARTESIAN_POINT('Ctrl Pts',(33.8286121124817,54.4443225979689,4.14890689942785));
#44644=CARTESIAN_POINT('Ctrl Pts',(34.7726100689922,56.4060048808339,4.26004478999589));
#44645=CARTESIAN_POINT('Ctrl Pts',(33.6364622561334,58.2630179851872,4.37118268056393));
#44646=CARTESIAN_POINT('Ctrl Pts',(31.460097652016,58.315616755694,4.48232057113198));
#44647=CARTESIAN_POINT('Ctrl Pts',(30.2355674600263,56.5156569431085,4.59345846170002));
#44648=CARTESIAN_POINT('Ctrl Pts',(31.0836980528375,54.5106621730209,4.70459635226806));
#44649=CARTESIAN_POINT('Ctrl Pts',(33.2281858787452,54.1358269042489,4.8157342428361));
#44650=CARTESIAN_POINT('Ctrl Pts',(34.7061569138339,55.7342420941504,4.92687213340414));
#44651=CARTESIAN_POINT('Ctrl Pts',(34.164807501817,57.8428602221521,5.03801002397219));
#44652=CARTESIAN_POINT('Ctrl Pts',(32.0996409118515,58.5316391425983,5.14914791454022));
#44653=CARTESIAN_POINT('Ctrl Pts',(30.4009275183955,57.1701318172634,5.26028580510827));
#44654=CARTESIAN_POINT('Ctrl Pts',(30.6235190068059,55.0045411047512,5.37142369567631));
#44655=CARTESIAN_POINT('Ctrl Pts',(32.5636747606314,54.017057215205,5.48256158624435));
#44656=CARTESIAN_POINT('Ctrl Pts',(34.4455484201109,55.1115344127627,5.59369947681239));
#44657=CARTESIAN_POINT('Ctrl Pts',(34.5466392755035,57.2861871754458,5.70483736738044));
#44658=CARTESIAN_POINT('Ctrl Pts',(32.7744185314064,58.550527445779,5.81597525794847));
#44659=CARTESIAN_POINT('Ctrl Pts',(30.7510183185457,57.7472976454435,5.92711314851652));
#44660=CARTESIAN_POINT('Ctrl Pts',(30.3284830135763,55.6116883669947,6.03825103908455));
#44661=CARTESIAN_POINT('Ctrl Pts',(31.8935575720505,54.0984763759544,6.1493889296526));
#44662=CARTESIAN_POINT('Ctrl Pts',(34.0137242459347,54.5926632852668,6.26052682022064));
#44663=CARTESIAN_POINT('Ctrl Pts',(34.748345059677,56.6420306545566,6.37166471078869));
#44664=CARTESIAN_POINT('Ctrl Pts',(33.4250637727444,58.3705374492314,6.48280260135672));
#44665=CARTESIAN_POINT('Ctrl Pts',(31.2549941659053,58.1965234039931,6.59394049192477));
#44666=CARTESIAN_POINT('Ctrl Pts',(30.2246258166159,56.2783463937137,6.70507838249281));
#44667=CARTESIAN_POINT('Ctrl Pts',(31.2766680692062,54.3735667032384,6.81621627306085));
#44668=CARTESIAN_POINT('Ctrl Pts',(33.4489651948853,54.221991514694,6.92735416362889));
#44669=CARTESIAN_POINT('Ctrl Pts',(34.7516470583929,55.9698087119448,7.03849205419693));
#44670=CARTESIAN_POINT('Ctrl Pts',(34.2470082093303,57.323173711667,7.1125839812423));
#44671=CARTESIAN_POINT('Ctrl Pts',(33.7642155196223,57.7435554488857,7.14962994476498));
#44672=CARTESIAN_POINT('Ctrl Pts',(34.2340161741268,55.8254888120548,-2.14962994476498));
#44673=CARTESIAN_POINT('Ctrl Pts',(34.3890262738776,56.4020904439209,-2.1125839812423));
#44674=CARTESIAN_POINT('Ctrl Pts',(34.0755350040887,57.7122735630109,-2.03849205419694));
#44675=CARTESIAN_POINT('Ctrl Pts',(32.1577847756023,58.3874867742776,-1.92735416362889));
#44676=CARTESIAN_POINT('Ctrl Pts',(30.5550873059959,57.1399513020318,-1.81621627306085));
#44677=CARTESIAN_POINT('Ctrl Pts',(30.7317276002978,55.1181192733998,-1.70507838249281));
#44678=CARTESIAN_POINT('Ctrl Pts',(32.5273167366304,54.169352590915,-1.59394049192477));
#44679=CARTESIAN_POINT('Ctrl Pts',(34.297687392575,55.1636929370367,-1.48280260135673));
#44680=CARTESIAN_POINT('Ctrl Pts',(34.4227224299926,57.19019361681,-1.37166471078869));
#44681=CARTESIAN_POINT('Ctrl Pts',(32.7878135612012,58.3943852360772,-1.26052682022064));
#44682=CARTESIAN_POINT('Ctrl Pts',(30.8894929283555,57.6738517983019,-1.1493889296526));
#44683=CARTESIAN_POINT('Ctrl Pts',(30.4652739949134,55.6882090694071,-1.03825103908456));
#44684=CARTESIAN_POINT('Ctrl Pts',(31.903469723963,54.2548864555714,-0.927113148516518));
#44685=CARTESIAN_POINT('Ctrl Pts',(33.8876729269554,54.6858464683213,-0.815975257948477));
#44686=CARTESIAN_POINT('Ctrl Pts',(34.6017250968181,56.5866134277799,-0.704837367380434));
#44687=CARTESIAN_POINT('Ctrl Pts',(33.3920435793748,58.2174003556871,-0.593699476812394));
#44688=CARTESIAN_POINT('Ctrl Pts',(31.3658648947325,58.0855261797825,-0.482561586244351));
#44689=CARTESIAN_POINT('Ctrl Pts',(30.3777727141902,56.3116984876511,-0.37142369567631));
#44690=CARTESIAN_POINT('Ctrl Pts',(31.3321793463981,54.519521049325,-0.260285805108268));
#44691=CARTESIAN_POINT('Ctrl Pts',(33.3555054114091,54.3493946172309,-0.149147914540226));
#44692=CARTESIAN_POINT('Ctrl Pts',(34.5957776991039,55.9570376338603,-0.0380100239721845));
#44693=CARTESIAN_POINT('Ctrl Pts',(33.9177608770916,57.8709563197388,0.0731278665958568));
#44694=CARTESIAN_POINT('Ctrl Pts',(31.9420514527978,58.3393191433506,0.184265757163899));
#44695=CARTESIAN_POINT('Ctrl Pts',(30.4770386577981,56.9334283272761,0.295403647731941));
#44696=CARTESIAN_POINT('Ctrl Pts',(30.8636653230292,54.9401116659806,0.406541538299983));
#44697=CARTESIAN_POINT('Ctrl Pts',(32.7480476744994,54.1838745120134,0.517679428868023));
#44698=CARTESIAN_POINT('Ctrl Pts',(34.4053891768952,55.3569093053397,0.628817319436067));
#44699=CARTESIAN_POINT('Ctrl Pts',(34.3187063568714,57.3855239982029,0.739955210004107));
#44700=CARTESIAN_POINT('Ctrl Pts',(32.5673409829831,58.4129045553191,0.85109310057215));
#44701=CARTESIAN_POINT('Ctrl Pts',(30.754337643615,57.4986779018991,0.962230991140189));
#44702=CARTESIAN_POINT('Ctrl Pts',(30.5391588562322,55.4796460616392,1.07336888170823));
#44703=CARTESIAN_POINT('Ctrl Pts',(32.1187602051768,54.2038517754153,1.18450677227627));
#44704=CARTESIAN_POINT('Ctrl Pts',(34.0473146618836,54.8390440218454,1.29564466284432));
#44705=CARTESIAN_POINT('Ctrl Pts',(34.559594460823,56.8038241342291,1.40678255341236));
#44706=CARTESIAN_POINT('Ctrl Pts',(33.1867040923831,58.299806593566,1.5179204439804));
#44707=CARTESIAN_POINT('Ctrl Pts',(31.18526568043,57.957701689237,1.62905833454844));
#44708=CARTESIAN_POINT('Ctrl Pts',(30.387218501281,56.0906419199043,1.74019622511648));
#44709=CARTESIAN_POINT('Ctrl Pts',(31.5230241884812,54.4075682663379,1.85133411568453));
#44710=CARTESIAN_POINT('Ctrl Pts',(33.5530669156239,54.4490171309996,1.96247200625256));
#44711=CARTESIAN_POINT('Ctrl Pts',(34.6192255523049,56.177049898003,2.07360989682061));
#44712=CARTESIAN_POINT('Ctrl Pts',(33.7456330073089,58.009978578485,2.18474778738865));
#44713=CARTESIAN_POINT('Ctrl Pts',(31.731898444284,58.2701027643758,2.29588567795669));
#44714=CARTESIAN_POINT('Ctrl Pts',(30.42121594607,56.7193278383203,2.40702356852473));
#44715=CARTESIAN_POINT('Ctrl Pts',(31.0132680674328,54.7770956771211,2.51816145909278));
#44716=CARTESIAN_POINT('Ctrl Pts',(32.9661427873612,54.2211534043346,2.62929934966082));
#44717=CARTESIAN_POINT('Ctrl Pts',(34.4923517275991,55.5603612870565,2.74043724022886));
#44718=CARTESIAN_POINT('Ctrl Pts',(34.1949385367603,57.568927162581,2.8515751307969));
#44719=CARTESIAN_POINT('Ctrl Pts',(32.3461288813143,58.4083879063544,2.96271302136494));
#44720=CARTESIAN_POINT('Ctrl Pts',(30.6381592058186,57.3103755794683,3.07385091193298));
#44721=CARTESIAN_POINT('Ctrl Pts',(30.6343535239477,55.2799133170288,3.18498880250103));
#44722=CARTESIAN_POINT('Ctrl Pts',(32.3381952194777,54.175506254854,3.29612669306906));
#44723=CARTESIAN_POINT('Ctrl Pts',(34.1901386656106,55.0080307017823,3.40726458363711));
#44724=CARTESIAN_POINT('Ctrl Pts',(34.4950790236344,57.0154675900672,3.51840247420515));
#44725=CARTESIAN_POINT('Ctrl Pts',(32.9739009255897,58.360387169986,3.6295403647732));
#44726=CARTESIAN_POINT('Ctrl Pts',(31.0189559359528,57.8117692975994,3.74067825534123));
#44727=CARTESIAN_POINT('Ctrl Pts',(30.4196273743162,55.8717701332809,3.85181614590928));
#44728=CARTESIAN_POINT('Ctrl Pts',(31.7244874700065,54.3160929131618,3.96295403647732));
#44729=CARTESIAN_POINT('Ctrl Pts',(33.7391829792937,54.5686666395094,4.07409192704536));
#44730=CARTESIAN_POINT('Ctrl Pts',(34.6196402543752,56.3983077159918,4.1852298176134));
#44731=CARTESIAN_POINT('Ctrl Pts',(33.5599667662066,58.1303249162124,4.29636770818144));
#44732=CARTESIAN_POINT('Ctrl Pts',(31.530093676218,58.1793832535041,4.40750559874948));
#44733=CARTESIAN_POINT('Ctrl Pts',(30.3879868436147,56.5005790771652,4.51864348931753));
#44734=CARTESIAN_POINT('Ctrl Pts',(31.1790296054233,54.6305408851872,4.62978137988557));
#44735=CARTESIAN_POINT('Ctrl Pts',(33.1791715491872,54.2809358494227,4.74091927045361));
#44736=CARTESIAN_POINT('Ctrl Pts',(34.5576600736896,55.771761409842,4.85205716102165));
#44737=CARTESIAN_POINT('Ctrl Pts',(34.0527489932322,57.7384480518666,4.9631950515897));
#44738=CARTESIAN_POINT('Ctrl Pts',(32.1265891579804,58.3808651325893,5.07433294215774));
#44739=CARTESIAN_POINT('Ctrl Pts',(30.5422164851039,57.1110011234562,5.18547083272578));
#44740=CARTESIAN_POINT('Ctrl Pts',(30.7498252982272,55.0911767323862,5.29660872329382));
#44741=CARTESIAN_POINT('Ctrl Pts',(32.5593888004209,54.1701605706663,5.40774661386186));
#44742=CARTESIAN_POINT('Ctrl Pts',(34.314593187089,55.1909683005501,5.5188845044299));
#44743=CARTESIAN_POINT('Ctrl Pts',(34.4088795978388,57.219244773476,5.63002239499794));
#44744=CARTESIAN_POINT('Ctrl Pts',(32.7559473680293,58.3984820605018,5.74116028556599));
#44745=CARTESIAN_POINT('Ctrl Pts',(30.8687426071207,57.6493178103144,5.85229817613403));
#44746=CARTESIAN_POINT('Ctrl Pts',(30.474648233639,55.6574567972967,5.96343606670207));
#44747=CARTESIAN_POINT('Ctrl Pts',(31.9343773268536,54.2460993922691,6.0745739572701));
#44748=CARTESIAN_POINT('Ctrl Pts',(33.9118351799479,54.7070224870208,6.18571184783815));
#44749=CARTESIAN_POINT('Ctrl Pts',(34.5970085274374,56.6184465501361,6.29684973840619));
#44750=CARTESIAN_POINT('Ctrl Pts',(33.3627975548145,58.2306072247468,6.40798762897424));
#44751=CARTESIAN_POINT('Ctrl Pts',(31.3387957446438,58.0683060978856,6.51912551954227));
#44752=CARTESIAN_POINT('Ctrl Pts',(30.3777816842967,56.2792419458429,6.63026341011033));
#44753=CARTESIAN_POINT('Ctrl Pts',(31.3590107734043,54.5026733374682,6.74140130067836));
#44754=CARTESIAN_POINT('Ctrl Pts',(33.3850901676995,54.3613007036024,6.8525391912464));
#44755=CARTESIAN_POINT('Ctrl Pts',(34.6000882679938,55.9914719939308,6.96367708181444));
#44756=CARTESIAN_POINT('Ctrl Pts',(34.129416755538,57.2537417389318,7.03776900885981));
#44757=CARTESIAN_POINT('Ctrl Pts',(33.6791209333089,57.6458275017164,7.07481497238249));
#44758=CARTESIAN_POINT('Ctrl Pts',(34.1088760084069,55.8591307382982,-2.22444491714747));
#44759=CARTESIAN_POINT('Ctrl Pts',(34.2526993673069,56.3941202878534,-2.18739895362479));
#44760=CARTESIAN_POINT('Ctrl Pts',(33.9618320787925,57.6097503485044,-2.11330702657943));
#44761=CARTESIAN_POINT('Ctrl Pts',(32.1824817020393,58.2362348948285,-2.00216913601138));
#44762=CARTESIAN_POINT('Ctrl Pts',(30.6954474136293,57.0787313369719,-1.89103124544334));
#44763=CARTESIAN_POINT('Ctrl Pts',(30.859339963111,55.2028105166065,-1.7798933548753));
#44764=CARTESIAN_POINT('Ctrl Pts',(32.5253453473205,54.3225142565131,-1.66875546430726));
#44765=CARTESIAN_POINT('Ctrl Pts',(34.1679522138747,55.2450952283263,-1.55761757373922));
#44766=CARTESIAN_POINT('Ctrl Pts',(34.28396374532,57.1253477734617,-1.44647968317117));
#44767=CARTESIAN_POINT('Ctrl Pts',(32.7670426841572,58.2426355096843,-1.33534179260313));
#44768=CARTESIAN_POINT('Ctrl Pts',(31.0057197114997,57.5741013987638,-1.22420390203509));
#44769=CARTESIAN_POINT('Ctrl Pts',(30.6121157333414,55.7317581752959,-1.11306601146705));
#44770=CARTESIAN_POINT('Ctrl Pts',(31.946520013063,54.4018753286905,-1.00192812089901));
#44771=CARTESIAN_POINT('Ctrl Pts',(33.7875275980737,54.801733897164,-0.890790230330966));
#44772=CARTESIAN_POINT('Ctrl Pts',(34.4500481800523,56.5653266503777,-0.779652339762923));
#44773=CARTESIAN_POINT('Ctrl Pts',(33.3276667396325,58.0784232421408,-0.668514449194882));
#44774=CARTESIAN_POINT('Ctrl Pts',(31.4477129519419,57.9560661379182,-0.55737655862684));
#44775=CARTESIAN_POINT('Ctrl Pts',(30.530929229224,56.3102517219396,-0.446238668058799));
#44776=CARTESIAN_POINT('Ctrl Pts',(31.4164584161689,54.6474118209319,-0.335100777490757));
#44777=CARTESIAN_POINT('Ctrl Pts',(33.2937654515659,54.4895630424277,-0.223962886922715));
#44778=CARTESIAN_POINT('Ctrl Pts',(34.444529993061,55.9811859685177,-0.112824996354674));
#44779=CARTESIAN_POINT('Ctrl Pts',(33.8154441664647,57.7569813167368,-0.00168710578663197));
#44780=CARTESIAN_POINT('Ctrl Pts',(31.9823173826673,58.1915434167809,0.10945078478141));
#44781=CARTESIAN_POINT('Ctrl Pts',(30.6230313661623,56.887112674916,0.220588675349452));
#44782=CARTESIAN_POINT('Ctrl Pts',(30.9817560281246,55.0376493300133,0.331726565917493));
#44783=CARTESIAN_POINT('Ctrl Pts',(32.7301466147766,54.3359881622353,0.442864456485535));
#44784=CARTESIAN_POINT('Ctrl Pts',(34.2678813952981,55.424367592698,0.554002347053577));
#44785=CARTESIAN_POINT('Ctrl Pts',(34.1874542853563,57.3065815872086,0.665140237621619));
#44786=CARTESIAN_POINT('Ctrl Pts',(32.5624811310993,58.2598183300436,0.776278128189661));
#44787=CARTESIAN_POINT('Ctrl Pts',(30.8803182889104,57.4115694204428,0.887416018757702));
#44788=CARTESIAN_POINT('Ctrl Pts',(30.680668485348,55.5382467049613,0.998553909325744));
#44789=CARTESIAN_POINT('Ctrl Pts',(32.1462734497561,54.3545237101042,1.10969179989378));
#44790=CARTESIAN_POINT('Ctrl Pts',(33.935648337141,54.9438755173456,1.22082969046183));
#44791=CARTESIAN_POINT('Ctrl Pts',(34.4109580201779,56.7668617338386,1.33196758102987));
#44792=CARTESIAN_POINT('Ctrl Pts',(33.1371461556097,58.1548824015447,1.44310547159791));
#44793=CARTESIAN_POINT('Ctrl Pts',(31.2801471890823,57.8374664620939,1.55424336216595));
#44794=CARTESIAN_POINT('Ctrl Pts',(30.53969333446,56.1051483246038,1.66538125273399));
#44795=CARTESIAN_POINT('Ctrl Pts',(31.593530402196,54.5435384261447,1.77651914330204));
#44796=CARTESIAN_POINT('Ctrl Pts',(33.4770693728664,54.581996016636,1.88765703387008));
#44797=CARTESIAN_POINT('Ctrl Pts',(34.4662856658319,56.1853204273628,1.99879492443812));
#44798=CARTESIAN_POINT('Ctrl Pts',(33.6557383896653,57.8859706422512,2.10993281500616));
#44799=CARTESIAN_POINT('Ctrl Pts',(31.7873306584734,58.1273222329285,2.2210707055742));
#44800=CARTESIAN_POINT('Ctrl Pts',(30.5712372578007,56.6884633513348,2.33220859614224));
#44801=CARTESIAN_POINT('Ctrl Pts',(31.1205622687203,54.8863978495623,2.44334648671029));
#44802=CARTESIAN_POINT('Ctrl Pts',(32.9325022789681,54.370576718196,2.55448437727833));
#44803=CARTESIAN_POINT('Ctrl Pts',(34.3485680483669,55.6131368885852,2.66562226784637));
#44804=CARTESIAN_POINT('Ctrl Pts',(34.0726185189081,57.4767489451818,2.77676015841441));
#44805=CARTESIAN_POINT('Ctrl Pts',(32.3572334243856,58.2556276377848,2.88789804898245));
#44806=CARTESIAN_POINT('Ctrl Pts',(30.7725241956061,57.2368564659694,2.99903593955049));
#44807=CARTESIAN_POINT('Ctrl Pts',(30.7689931614964,55.3529282369496,3.11017383011854));
#44808=CARTESIAN_POINT('Ctrl Pts',(32.3498723176219,54.3282238239454,3.22131172068658));
#44809=CARTESIAN_POINT('Ctrl Pts',(34.0681650439915,55.10066679712,3.33244961125462));
#44810=CARTESIAN_POINT('Ctrl Pts',(34.351098521395,56.9632313430239,3.44358750182266));
#44811=CARTESIAN_POINT('Ctrl Pts',(32.9397005292797,58.2110910098795,3.5547253923907));
#44812=CARTESIAN_POINT('Ctrl Pts',(31.1258396561734,57.7020656929093,3.66586328295875));
#44813=CARTESIAN_POINT('Ctrl Pts',(30.569763329806,55.9020720375025,3.77700117352679));
#44814=CARTESIAN_POINT('Ctrl Pts',(31.7804545180475,54.4586646497164,3.88813906409483));
#44815=CARTESIAN_POINT('Ctrl Pts',(33.6497538461057,54.6930106810501,3.99927695466287));
#44816=CARTESIAN_POINT('Ctrl Pts',(34.4666704397582,56.3906105511495,4.11041484523091));
#44817=CARTESIAN_POINT('Ctrl Pts',(33.4834712762799,57.9976318472377,4.22155273579896));
#44818=CARTESIAN_POINT('Ctrl Pts',(31.60008970042,58.0431497513142,4.33269062636699));
#44819=CARTESIAN_POINT('Ctrl Pts',(30.5404062272031,56.4855012112219,4.44382851693505));
#44820=CARTESIAN_POINT('Ctrl Pts',(31.2743611580091,54.7504195973535,4.55496640750307));
#44821=CARTESIAN_POINT('Ctrl Pts',(33.1301572196292,54.4260447945964,4.66610429807113));
#44822=CARTESIAN_POINT('Ctrl Pts',(34.4091632335454,55.8092807255337,4.77724218863916));
#44823=CARTESIAN_POINT('Ctrl Pts',(33.9406904846474,57.6340358815812,4.88838007920721));
#44824=CARTESIAN_POINT('Ctrl Pts',(32.1535374041094,58.2300911225802,4.99951796977524));
#44825=CARTESIAN_POINT('Ctrl Pts',(30.6835054518121,57.0518704296491,5.11065586034329));
#44826=CARTESIAN_POINT('Ctrl Pts',(30.8761315896486,55.1778123600212,5.22179375091132));
#44827=CARTESIAN_POINT('Ctrl Pts',(32.5551028402105,54.3232639261277,5.33293164147937));
#44828=CARTESIAN_POINT('Ctrl Pts',(34.1836379540671,55.2704021883376,5.44406953204741));
#44829=CARTESIAN_POINT('Ctrl Pts',(34.2711199201742,57.1523023715063,5.55520742261546));
#44830=CARTESIAN_POINT('Ctrl Pts',(32.7374762046522,58.2464366752245,5.66634531318349));
#44831=CARTESIAN_POINT('Ctrl Pts',(30.9864668956958,57.5513379751854,5.77748320375154));
#44832=CARTESIAN_POINT('Ctrl Pts',(30.6208134537018,55.7032252275986,5.88862109431957));
#44833=CARTESIAN_POINT('Ctrl Pts',(31.9751970816566,54.3937224085839,5.99975898488763));
#44834=CARTESIAN_POINT('Ctrl Pts',(33.809946113961,54.8213816887749,6.11089687545565));
#44835=CARTESIAN_POINT('Ctrl Pts',(34.4456719951979,56.5948624457155,6.22203476602371));
#44836=CARTESIAN_POINT('Ctrl Pts',(33.3005313368845,58.0906770002622,6.33317265659174));
#44837=CARTESIAN_POINT('Ctrl Pts',(31.4225973233824,57.940088791778,6.4443105471598));
#44838=CARTESIAN_POINT('Ctrl Pts',(30.5309375519775,56.280137497972,6.55544843772783));
#44839=CARTESIAN_POINT('Ctrl Pts',(31.4413534776024,54.631779971698,6.66658632829587));
#44840=CARTESIAN_POINT('Ctrl Pts',(33.3212151405137,54.5006098925109,6.77772421886391));
#44841=CARTESIAN_POINT('Ctrl Pts',(34.4485294775946,56.0131352759167,6.88886210943196));
#44842=CARTESIAN_POINT('Ctrl Pts',(34.0118253017458,57.1843097661965,6.96295403647732));
#44843=CARTESIAN_POINT('Ctrl Pts',(33.5940263469955,57.5480995545471,7.));
#44844=CARTESIAN_POINT('Ctrl Pts',(33.3311039683456,57.7330494773494,-1.3785196366098));
#44845=CARTESIAN_POINT('Ctrl Pts',(33.1447009981387,57.8419592717116,-1.36412702194092));
#44846=CARTESIAN_POINT('Ctrl Pts',(32.9385791362006,57.9159412173671,-1.34973440727203));
#44847=CARTESIAN_POINT('Ctrl Pts',(32.7263090322414,57.9449985351604,-1.33534179260314));
#44848=CARTESIAN_POINT('Ctrl Pts',(32.1799350266047,58.0197908060441,-1.29829582908046));
#44849=CARTESIAN_POINT('Ctrl Pts',(31.5928273690522,57.796946102404,-1.26124986555778));
#44850=CARTESIAN_POINT('Ctrl Pts',(31.2336728772496,57.3784665466726,-1.2242039020351));
#44851=CARTESIAN_POINT('Ctrl Pts',(30.874518385447,56.9599869909412,-1.18715793851242));
#44852=CARTESIAN_POINT('Ctrl Pts',(30.7433170593942,56.3458725831185,-1.15011197498974));
#44853=CARTESIAN_POINT('Ctrl Pts',(30.9001171096548,55.8171682381063,-1.11306601146706));
#44854=CARTESIAN_POINT('Ctrl Pts',(31.0569171599153,55.2884638930941,-1.07602004794438));
#44855=CARTESIAN_POINT('Ctrl Pts',(31.5017185864892,54.8451696108923,-1.0389740844217));
#44856=CARTESIAN_POINT('Ctrl Pts',(32.0309538972778,54.690165564537,-1.00192812089902));
#44857=CARTESIAN_POINT('Ctrl Pts',(32.5601892080665,54.5351615181817,-0.964882157376335));
#44858=CARTESIAN_POINT('Ctrl Pts',(33.1738584030701,54.6684477076728,-0.927836193853654));
#44859=CARTESIAN_POINT('Ctrl Pts',(33.5911130975683,55.029022927954,-0.890790230330973));
#44860=CARTESIAN_POINT('Ctrl Pts',(34.0083677920665,55.3895981482352,-0.853744266808293));
#44861=CARTESIAN_POINT('Ctrl Pts',(34.2292079860594,55.9774623993064,-0.816698303285612));
#44862=CARTESIAN_POINT('Ctrl Pts',(34.1525645096526,56.5235772901359,-0.779652339762931));
#44863=CARTESIAN_POINT('Ctrl Pts',(34.0828208613931,57.0205281937339,-0.745941438711888));
#44864=CARTESIAN_POINT('Ctrl Pts',(33.7667445152314,57.4829083508763,-0.712230537660845));
#44865=CARTESIAN_POINT('Ctrl Pts',(33.3333524836119,57.7367881187288,-0.678519636609802));
#44866=CARTESIAN_POINT('Ctrl Pts',(34.4842965055667,55.7582049595679,-2.));
#44867=CARTESIAN_POINT('Ctrl Pts',(34.4966111053925,55.830382760503,-2.));
#44868=CARTESIAN_POINT('Ctrl Pts',(34.5047055015068,55.9030302259432,-2.));
#44869=CARTESIAN_POINT('Ctrl Pts',(34.5087398487957,55.975836724312,-2.));
#44870=CARTESIAN_POINT('Ctrl Pts',(34.5128864619034,56.0506692458705,-2.));
#44871=CARTESIAN_POINT('Ctrl Pts',(34.5127437096053,56.1256707869282,-2.));
#44872=CARTESIAN_POINT('Ctrl Pts',(34.5084312212538,56.2004993443966,-2.));
#44873=CARTESIAN_POINT('Ctrl Pts',(34.5047872656982,56.2637277905931,-2.));
#44874=CARTESIAN_POINT('Ctrl Pts',(34.4981650958835,56.3268329649118,-2.));
#44875=CARTESIAN_POINT('Ctrl Pts',(34.4886099106143,56.3895978470293,-2.));
#44876=CARTESIAN_POINT('Ctrl Pts',(34.4843647905613,56.4174826501174,-2.));
#44877=CARTESIAN_POINT('Ctrl Pts',(34.4795404472607,56.4453001134182,-2.));
#44878=CARTESIAN_POINT('Ctrl Pts',(34.4741394411489,56.4730302233705,-2.));
#44879=CARTESIAN_POINT('Ctrl Pts',(34.4711718179616,56.4882667396007,-2.));
#44880=CARTESIAN_POINT('Ctrl Pts',(34.4680300836907,56.5034768715482,-2.));
#44881=CARTESIAN_POINT('Ctrl Pts',(34.4647145599138,56.5186572039168,-2.));
#44882=CARTESIAN_POINT('Ctrl Pts',(34.4616570554946,56.5326561785654,-2.));
#44883=CARTESIAN_POINT('Ctrl Pts',(34.45845116215,56.5466318131546,-2.));
#44884=CARTESIAN_POINT('Ctrl Pts',(34.4551025744278,56.5605599363288,-2.));
#44885=CARTESIAN_POINT('Ctrl Pts',(34.4379902743583,56.631736875066,-2.));
#44886=CARTESIAN_POINT('Ctrl Pts',(34.417129771285,56.7017985031124,-2.));
#44887=CARTESIAN_POINT('Ctrl Pts',(34.3926364221807,56.7704257260637,-2.));
#44888=CARTESIAN_POINT('Ctrl Pts',(34.3683331729278,56.8385203136112,-2.));
#44889=CARTESIAN_POINT('Ctrl Pts',(34.3404527390893,56.9052035572333,-2.));
#44890=CARTESIAN_POINT('Ctrl Pts',(34.3090644243563,56.9701370642033,-2.));
#44891=CARTESIAN_POINT('Ctrl Pts',(34.2829778948777,57.0241026835151,-2.));
#44892=CARTESIAN_POINT('Ctrl Pts',(34.2544675459293,57.0768595084347,-2.));
#44893=CARTESIAN_POINT('Ctrl Pts',(34.2235537441951,57.1281926115957,-2.));
#44894=CARTESIAN_POINT('Ctrl Pts',(34.2106502677927,57.1496191411115,-2.));
#44895=CARTESIAN_POINT('Ctrl Pts',(34.197327856878,57.1707973646537,-2.));
#44896=CARTESIAN_POINT('Ctrl Pts',(34.1835872002777,57.191710445978,-2.));
#44897=CARTESIAN_POINT('Ctrl Pts',(34.1772270825051,57.2013904535701,-2.));
#44898=CARTESIAN_POINT('Ctrl Pts',(34.1707773505651,57.2110136443968,-2.));
#44899=CARTESIAN_POINT('Ctrl Pts',(34.1642380418293,57.2205782912845,-2.));
#44900=CARTESIAN_POINT('Ctrl Pts',(34.1574176230365,57.2305541006574,-2.));
#44901=CARTESIAN_POINT('Ctrl Pts',(34.1505044190796,57.2404593596496,-2.));
#44902=CARTESIAN_POINT('Ctrl Pts',(34.1435014736337,57.2502888014871,-2.));
#44903=CARTESIAN_POINT('Ctrl Pts',(34.1036166313874,57.3062717789476,-2.));
#44904=CARTESIAN_POINT('Ctrl Pts',(34.0607968393012,57.3598374440895,-2.));
#44905=CARTESIAN_POINT('Ctrl Pts',(34.0151074156251,57.4106900609547,-2.));
#44906=CARTESIAN_POINT('Ctrl Pts',(33.9736959571629,57.4567812755417,-2.));
#44907=CARTESIAN_POINT('Ctrl Pts',(33.9299264067014,57.5006437323277,-2.));
#44908=CARTESIAN_POINT('Ctrl Pts',(33.8838248402233,57.5420278185054,-2.));
#44909=CARTESIAN_POINT('Ctrl Pts',(33.8292843968241,57.5909872483519,-2.));
#44910=CARTESIAN_POINT('Ctrl Pts',(33.7714790326439,57.6364792135475,-2.));
#44911=CARTESIAN_POINT('Ctrl Pts',(33.7108128089775,57.6783572197639,-2.));
#44912=CARTESIAN_POINT('Ctrl Pts',(33.6974562676307,57.6875772649183,-2.));
#44913=CARTESIAN_POINT('Ctrl Pts',(33.6839610126013,57.6966218980588,-2.));
#44914=CARTESIAN_POINT('Ctrl Pts',(33.6703313137203,57.7054891532984,-2.));
#44915=CARTESIAN_POINT('Ctrl Pts',(33.6562679227742,57.7146385613772,-2.));
#44916=CARTESIAN_POINT('Ctrl Pts',(33.6420560771616,57.7236022055282,-2.));
#44917=CARTESIAN_POINT('Ctrl Pts',(33.6277297174338,57.7323603945594,-2.));
#44918=CARTESIAN_POINT('Ctrl Pts',(33.569215230037,57.7681322829823,-2.));
#44919=CARTESIAN_POINT('Ctrl Pts',(33.5087208994645,57.8005303979702,-2.));
#44920=CARTESIAN_POINT('Ctrl Pts',(33.4466000497757,57.8294900318497,-2.));
#44921=CARTESIAN_POINT('Ctrl Pts',(33.3844917461018,57.8584438170004,-2.));
#44922=CARTESIAN_POINT('Ctrl Pts',(33.3207564252846,57.8839606526941,-2.));
#44923=CARTESIAN_POINT('Ctrl Pts',(33.2557354106676,57.905925394536,-2.));
#44924=CARTESIAN_POINT('Ctrl Pts',(33.2086728278312,57.9218236005007,-2.));
#44925=CARTESIAN_POINT('Ctrl Pts',(33.1609363812474,57.9358598412383,-2.));
#44926=CARTESIAN_POINT('Ctrl Pts',(33.1126567567704,57.9479733084058,-2.));
#44927=CARTESIAN_POINT('Ctrl Pts',(33.0764412556209,57.9570598596971,-2.));
#44928=CARTESIAN_POINT('Ctrl Pts',(33.0399201289053,57.9650642116641,-2.));
#44929=CARTESIAN_POINT('Ctrl Pts',(33.0031501969537,57.9719552160039,-2.));
#44930=CARTESIAN_POINT('Ctrl Pts',(32.9909318989143,57.9742450310877,-2.));
#44931=CARTESIAN_POINT('Ctrl Pts',(32.9786957157085,57.9764100788818,-2.));
#44932=CARTESIAN_POINT('Ctrl Pts',(32.9664441134471,57.9784496521969,-2.));
#44933=CARTESIAN_POINT('Ctrl Pts',(32.9014564692835,57.9892684056971,-2.));
#44934=CARTESIAN_POINT('Ctrl Pts',(32.8360307197705,57.996561300293,-2.));
#44935=CARTESIAN_POINT('Ctrl Pts',(32.7704812212897,58.0002046036744,-2.));
#44936=CARTESIAN_POINT('Ctrl Pts',(32.7243572374919,58.0027682185003,-2.));
#44937=CARTESIAN_POINT('Ctrl Pts',(32.678172012929,58.0035238244839,-2.));
#44938=CARTESIAN_POINT('Ctrl Pts',(32.6320397021384,58.0024136109102,-2.));
#44939=CARTESIAN_POINT('Ctrl Pts',(32.6172320120056,58.0020572511636,-2.));
#44940=CARTESIAN_POINT('Ctrl Pts',(32.6024277816188,58.0015084555323,-2.));
#44941=CARTESIAN_POINT('Ctrl Pts',(32.5876374051397,58.0007653782458,-2.));
#44942=CARTESIAN_POINT('Ctrl Pts',(32.5246283833708,57.9975997676214,-2.));
#44943=CARTESIAN_POINT('Ctrl Pts',(32.4619962285916,57.9909192311175,-2.));
#44944=CARTESIAN_POINT('Ctrl Pts',(32.4000310708476,57.9805958152549,-2.));
#44945=CARTESIAN_POINT('Ctrl Pts',(32.3429040942577,57.9710784419796,-2.));
#44946=CARTESIAN_POINT('Ctrl Pts',(32.2863436472675,57.9584643876278,-2.));
#44947=CARTESIAN_POINT('Ctrl Pts',(32.2305948723589,57.942618319326,-2.));
#44948=CARTESIAN_POINT('Ctrl Pts',(32.2201618224275,57.9396528223787,-2.));
#44949=CARTESIAN_POINT('Ctrl Pts',(32.2097572620709,57.9365740341467,-2.));
#44950=CARTESIAN_POINT('Ctrl Pts',(32.1993825459687,57.9333829869217,-2.));
#44951=CARTESIAN_POINT('Origin',(32.5,56.2916512459885,3.));
#44952=CARTESIAN_POINT('Origin',(32.5,-56.2916512459885,8.));
#44953=CARTESIAN_POINT('Origin',(-32.5,-56.2916512459885,8.));
#44954=CARTESIAN_POINT('Origin',(-65.,8.88178419700125E-15,8.));
#44955=CARTESIAN_POINT('Origin',(-32.5,56.2916512459885,8.));
#44956=CARTESIAN_POINT('Origin',(32.5,56.2916512459885,8.));
#44957=CARTESIAN_POINT('Origin',(32.5,-56.2916512459885,13.));
#44958=CARTESIAN_POINT('Ctrl Pts',(31.4059736530044,-55.03520293743,13.));
#44959=CARTESIAN_POINT('Ctrl Pts',(31.3544234714672,-55.070553205003,13.));
#44960=CARTESIAN_POINT('Ctrl Pts',(31.3051813503374,-55.1089326491051,13.));
#44961=CARTESIAN_POINT('Ctrl Pts',(31.2583086630398,-55.1500094432322,13.));
#44962=CARTESIAN_POINT('Ctrl Pts',(31.2285772761546,-55.1760644899685,13.));
#44963=CARTESIAN_POINT('Ctrl Pts',(31.1997994780201,-55.2032058502151,13.));
#44964=CARTESIAN_POINT('Ctrl Pts',(31.1719948710937,-55.2313585593622,13.));
#44965=CARTESIAN_POINT('Ctrl Pts',(31.1530079463075,-55.2505831926225,13.));
#44966=CARTESIAN_POINT('Ctrl Pts',(31.1344748974185,-55.2702795821264,13.));
#44967=CARTESIAN_POINT('Ctrl Pts',(31.1164029944547,-55.2904256030864,13.));
#44968=CARTESIAN_POINT('Ctrl Pts',(31.10680688574,-55.3011230602213,13.));
#44969=CARTESIAN_POINT('Ctrl Pts',(31.097341027084,-55.311947259576,13.));
#44970=CARTESIAN_POINT('Ctrl Pts',(31.0880156367974,-55.3228838799501,13.));
#44971=CARTESIAN_POINT('Ctrl Pts',(31.0452129481991,-55.373081967301,13.));
#44972=CARTESIAN_POINT('Ctrl Pts',(31.0053166517631,-55.4257004118496,13.));
#44973=CARTESIAN_POINT('Ctrl Pts',(30.9684112137071,-55.4803964712117,13.));
#44974=CARTESIAN_POINT('Ctrl Pts',(30.9417896431645,-55.5198512258336,13.));
#44975=CARTESIAN_POINT('Ctrl Pts',(30.916724774461,-55.5603881845169,13.));
#44976=CARTESIAN_POINT('Ctrl Pts',(30.8932580445526,-55.6018923080322,13.));
#44977=CARTESIAN_POINT('Ctrl Pts',(30.8868285874191,-55.6132636829126,13.));
#44978=CARTESIAN_POINT('Ctrl Pts',(30.8805191498619,-55.6247077158807,13.));
#44979=CARTESIAN_POINT('Ctrl Pts',(30.8743307104748,-55.636222162741,13.));
#44980=CARTESIAN_POINT('Ctrl Pts',(30.8680004795506,-55.648000432355,13.));
#44981=CARTESIAN_POINT('Ctrl Pts',(30.8618007209708,-55.6598452663792,13.));
#44982=CARTESIAN_POINT('Ctrl Pts',(30.8557343742871,-55.6717493028589,13.));
#44983=CARTESIAN_POINT('Ctrl Pts',(30.824926284678,-55.732204242495,13.));
#44984=CARTESIAN_POINT('Ctrl Pts',(30.7975367125457,-55.794219620245,13.));
#44985=CARTESIAN_POINT('Ctrl Pts',(30.7736505522206,-55.8574477163192,13.));
#44986=CARTESIAN_POINT('Ctrl Pts',(30.7494182331566,-55.9215921152943,13.));
#44987=CARTESIAN_POINT('Ctrl Pts',(30.72879092513,-55.9869854550098,13.));
#44988=CARTESIAN_POINT('Ctrl Pts',(30.7118943736091,-56.0533023281135,13.));
#44989=CARTESIAN_POINT('Ctrl Pts',(30.7014256021216,-56.094390960278,13.));
#44990=CARTESIAN_POINT('Ctrl Pts',(30.6923897620677,-56.1358348149116,13.));
#44991=CARTESIAN_POINT('Ctrl Pts',(30.6848255186051,-56.1775614118862,13.));
#44992=CARTESIAN_POINT('Ctrl Pts',(30.6786294263779,-56.2117408832985,13.));
#44993=CARTESIAN_POINT('Ctrl Pts',(30.6734208465555,-56.2461101538938,13.));
#44994=CARTESIAN_POINT('Ctrl Pts',(30.66922486922,-56.2806305243324,13.));
#44995=CARTESIAN_POINT('Ctrl Pts',(30.6675094773901,-56.2947430794491,13.));
#44996=CARTESIAN_POINT('Ctrl Pts',(30.6659632509475,-56.3088834624587,13.));
#44997=CARTESIAN_POINT('Ctrl Pts',(30.6645900225892,-56.3230249696056,13.));
#44998=CARTESIAN_POINT('Ctrl Pts',(30.657777408341,-56.3931812786421,13.));
#44999=CARTESIAN_POINT('Ctrl Pts',(30.6552023639046,-56.4634862436646,13.));
#45000=CARTESIAN_POINT('Ctrl Pts',(30.6569799481117,-56.5335953127025,13.));
#45001=CARTESIAN_POINT('Ctrl Pts',(30.6571775468159,-56.5413887331989,13.));
#45002=CARTESIAN_POINT('Ctrl Pts',(30.6574289761761,-56.5491797596255,13.));
#45003=CARTESIAN_POINT('Ctrl Pts',(30.6577344296099,-56.5569679370674,13.));
#45004=CARTESIAN_POINT('Ctrl Pts',(30.6603769077943,-56.6243434735914,13.));
#45005=CARTESIAN_POINT('Ctrl Pts',(30.6670582139719,-56.6915049782437,13.));
#45006=CARTESIAN_POINT('Ctrl Pts',(30.677541462644,-56.7582070441068,13.));
#45007=CARTESIAN_POINT('Ctrl Pts',(30.6888193174907,-56.8299649733815,13.));
#45008=CARTESIAN_POINT('Ctrl Pts',(30.7044969561434,-56.9011921151434,13.));
#45009=CARTESIAN_POINT('Ctrl Pts',(30.7243435713018,-56.9715867176043,13.));
#45010=CARTESIAN_POINT('Ctrl Pts',(30.72797807261,-56.9844780480751,13.));
#45011=CARTESIAN_POINT('Ctrl Pts',(30.731752555977,-56.9973414436069,13.));
#45012=CARTESIAN_POINT('Ctrl Pts',(30.7356658277082,-57.0101750208647,13.));
#45013=CARTESIAN_POINT('Ctrl Pts',(30.7390274224034,-57.0211993729146,13.));
#45014=CARTESIAN_POINT('Ctrl Pts',(30.7424887108225,-57.0321927628317,13.));
#45015=CARTESIAN_POINT('Ctrl Pts',(30.7460479825644,-57.0431526566225,13.));
#45016=CARTESIAN_POINT('Ctrl Pts',(30.7679991292784,-57.1107457638707,13.));
#45017=CARTESIAN_POINT('Ctrl Pts',(30.7936779402928,-57.177081381741,13.));
#45018=CARTESIAN_POINT('Ctrl Pts',(30.8228134385709,-57.2418920410565,13.));
#45019=CARTESIAN_POINT('Ctrl Pts',(30.8525629753419,-57.3080686025165,13.));
#45020=CARTESIAN_POINT('Ctrl Pts',(30.8859166603802,-57.3726561598101,13.));
#45021=CARTESIAN_POINT('Ctrl Pts',(30.9226411455397,-57.4353698900493,13.));
#45022=CARTESIAN_POINT('Ctrl Pts',(30.9595879478473,-57.4984632672077,13.));
#45023=CARTESIAN_POINT('Ctrl Pts',(30.9999468759528,-57.5596610610251,13.));
#45024=CARTESIAN_POINT('Ctrl Pts',(31.0435306577909,-57.618658668117,13.));
#45025=CARTESIAN_POINT('Ctrl Pts',(31.0543033138896,-57.6332411780565,13.));
#45026=CARTESIAN_POINT('Ctrl Pts',(31.0652732111657,-57.6476891601633,13.));
#45027=CARTESIAN_POINT('Ctrl Pts',(31.0764379482539,-57.6619977671329,13.));
#45028=CARTESIAN_POINT('Ctrl Pts',(31.0851682203193,-57.6731863899133,13.));
#45029=CARTESIAN_POINT('Ctrl Pts',(31.0940187404437,-57.6842909722259,13.));
#45030=CARTESIAN_POINT('Ctrl Pts',(31.1029745495045,-57.6952926419673,13.));
#45031=CARTESIAN_POINT('Ctrl Pts',(31.1505373075081,-57.7537206133534,13.));
#45032=CARTESIAN_POINT('Ctrl Pts',(31.2011482674294,-57.8093550198619,13.));
#45033=CARTESIAN_POINT('Ctrl Pts',(31.2545510980919,-57.8619011541248,13.));
#45034=CARTESIAN_POINT('Ctrl Pts',(31.3080118293392,-57.9145042601225,13.));
#45035=CARTESIAN_POINT('Ctrl Pts',(31.3642709811015,-57.9640134083886,13.));
#45036=CARTESIAN_POINT('Ctrl Pts',(31.4231195457109,-58.010113437602,13.));
#45037=CARTESIAN_POINT('Ctrl Pts',(31.4806288821152,-58.0551643595042,13.));
#45038=CARTESIAN_POINT('Ctrl Pts',(31.5406117299258,-58.0969603997432,13.));
#45039=CARTESIAN_POINT('Ctrl Pts',(31.6029105624086,-58.1351753158739,13.));
#45040=CARTESIAN_POINT('Ctrl Pts',(31.6163051637375,-58.1433917389751,13.));
#45041=CARTESIAN_POINT('Ctrl Pts',(31.6298069488463,-58.1514424691007,13.));
#45042=CARTESIAN_POINT('Ctrl Pts',(31.6434145443376,-58.1593240060195,13.));
#45043=CARTESIAN_POINT('Ctrl Pts',(31.6549388802987,-58.1659989163223,13.));
#45044=CARTESIAN_POINT('Ctrl Pts',(31.666539109872,-58.1725524712207,13.));
#45045=CARTESIAN_POINT('Ctrl Pts',(31.6782133743559,-58.1789848186021,13.));
#45046=CARTESIAN_POINT('Ctrl Pts',(32.7283737736498,-58.3336705852723,13.));
#45047=CARTESIAN_POINT('Ctrl Pts',(32.801456501431,-58.3184742869055,13.));
#45048=CARTESIAN_POINT('Ctrl Pts',(32.8734788597396,-58.298997786029,13.));
#45049=CARTESIAN_POINT('Ctrl Pts',(32.9441813035354,-58.2754925548906,13.));
#45050=CARTESIAN_POINT('Ctrl Pts',(33.0130334318726,-58.2526024664573,13.));
#45051=CARTESIAN_POINT('Ctrl Pts',(33.0806343841287,-58.2258909044602,13.));
#45052=CARTESIAN_POINT('Ctrl Pts',(33.1467189154918,-58.1955520781492,13.));
#45053=CARTESIAN_POINT('Ctrl Pts',(33.1614684625166,-58.1887806910164,13.));
#45054=CARTESIAN_POINT('Ctrl Pts',(33.1761442888062,-58.1818275349416,13.));
#45055=CARTESIAN_POINT('Ctrl Pts',(33.1907370174276,-58.1746976086672,13.));
#45056=CARTESIAN_POINT('Ctrl Pts',(33.2577025900794,-58.1419786012548,13.));
#45057=CARTESIAN_POINT('Ctrl Pts',(33.3227883256884,-58.1056063855858,13.));
#45058=CARTESIAN_POINT('Ctrl Pts',(33.3857181635784,-58.0658123209271,13.));
#45059=CARTESIAN_POINT('Ctrl Pts',(33.4298991913055,-58.0378741800863,13.));
#45060=CARTESIAN_POINT('Ctrl Pts',(33.4730169947395,-58.0082484492559,13.));
#45061=CARTESIAN_POINT('Ctrl Pts',(33.5149645797389,-57.9770049692026,13.));
#45062=CARTESIAN_POINT('Ctrl Pts',(33.5309116525527,-57.9651272400944,13.));
#45063=CARTESIAN_POINT('Ctrl Pts',(33.5466894876595,-57.9530156292951,13.));
#45064=CARTESIAN_POINT('Ctrl Pts',(33.5622917797584,-57.9406737257053,13.));
#45065=CARTESIAN_POINT('Ctrl Pts',(33.5771528445811,-57.9289181561955,13.));
#45066=CARTESIAN_POINT('Ctrl Pts',(33.5918591265304,-57.916949716641,13.));
#45067=CARTESIAN_POINT('Ctrl Pts',(33.6063795972843,-57.9047932103788,13.));
#45068=CARTESIAN_POINT('Ctrl Pts',(33.6620452141432,-57.8581900780557,13.));
#45069=CARTESIAN_POINT('Ctrl Pts',(33.7150448946165,-57.8087799685606,13.));
#45070=CARTESIAN_POINT('Ctrl Pts',(33.7651216104469,-57.7567754487711,13.));
#45071=CARTESIAN_POINT('Ctrl Pts',(33.8141231388454,-57.7058875079175,13.));
#45072=CARTESIAN_POINT('Ctrl Pts',(33.8603263529607,-57.6525145643954,13.));
#45073=CARTESIAN_POINT('Ctrl Pts',(33.9034486471934,-57.5968301466407,13.));
#45074=CARTESIAN_POINT('Ctrl Pts',(33.9456250981648,-57.5423671094322,13.));
#45075=CARTESIAN_POINT('Ctrl Pts',(33.9848546823971,-57.485692216831,13.));
#45076=CARTESIAN_POINT('Ctrl Pts',(34.0208263213787,-57.4269537423419,13.));
#45077=CARTESIAN_POINT('Ctrl Pts',(34.0325140425975,-57.4078687372078,13.));
#45078=CARTESIAN_POINT('Ctrl Pts',(34.0438574259696,-57.3885658089128,13.));
#45079=CARTESIAN_POINT('Ctrl Pts',(34.0548446057631,-57.3690498891776,13.));
#45080=CARTESIAN_POINT('Ctrl Pts',(34.0610436454207,-57.3580388779202,13.));
#45081=CARTESIAN_POINT('Ctrl Pts',(34.0671298182374,-57.3469588596036,13.));
#45082=CARTESIAN_POINT('Ctrl Pts',(34.0730927271078,-57.3358266055139,13.));
#45083=CARTESIAN_POINT('Ctrl Pts',(34.1053441709564,-57.2756158467244,13.));
#45084=CARTESIAN_POINT('Ctrl Pts',(34.1340531807434,-57.2137749292232,13.));
#45085=CARTESIAN_POINT('Ctrl Pts',(34.1589642502906,-57.1504676174455,13.));
#45086=CARTESIAN_POINT('Ctrl Pts',(34.1625594233608,-57.1413310871163,13.));
#45087=CARTESIAN_POINT('Ctrl Pts',(34.1660754069223,-57.132163987681,13.));
#45088=CARTESIAN_POINT('Ctrl Pts',(34.1695113451333,-57.1229667871477,13.));
#45089=CARTESIAN_POINT('Ctrl Pts',(34.1937894815815,-57.05797991143,13.));
#45090=CARTESIAN_POINT('Ctrl Pts',(34.2140754401812,-56.9914902794374,13.));
#45091=CARTESIAN_POINT('Ctrl Pts',(34.2304117433295,-56.9238636615664,13.));
#45092=CARTESIAN_POINT('Ctrl Pts',(34.2456521934161,-56.8607734945421,13.));
#45093=CARTESIAN_POINT('Ctrl Pts',(34.2574544361006,-56.7966929502049,13.));
#45094=CARTESIAN_POINT('Ctrl Pts',(34.2658134374973,-56.7319255341013,13.));
#45095=CARTESIAN_POINT('Ctrl Pts',(34.2676584011698,-56.7176303421036,13.));
#45096=CARTESIAN_POINT('Ctrl Pts',(34.2693354843654,-56.7033017407798,13.));
#45097=CARTESIAN_POINT('Ctrl Pts',(34.270844395972,-56.6889430967336,13.));
#45098=CARTESIAN_POINT('Ctrl Pts',(34.2720238222348,-56.6777198005427,13.));
#45099=CARTESIAN_POINT('Ctrl Pts',(34.2731003471964,-56.6664788446859,13.));
#45100=CARTESIAN_POINT('Ctrl Pts',(34.2740729517289,-56.655234855777,13.));
#45101=CARTESIAN_POINT('Ctrl Pts',(34.2799651735089,-56.5871166493205,13.));
#45102=CARTESIAN_POINT('Ctrl Pts',(34.2820614503553,-56.5187616004217,13.));
#45103=CARTESIAN_POINT('Ctrl Pts',(34.2804207734115,-56.4505176925959,13.));
#45104=CARTESIAN_POINT('Ctrl Pts',(34.2787876667758,-56.3825886715075,13.));
#45105=CARTESIAN_POINT('Ctrl Pts',(34.2734516847404,-56.3147686810319,13.));
#45106=CARTESIAN_POINT('Ctrl Pts',(34.2644214383682,-56.2474134550015,13.));
#45107=CARTESIAN_POINT('Ctrl Pts',(34.2555845575225,-56.1815005128466,13.));
#45108=CARTESIAN_POINT('Ctrl Pts',(34.2432095214319,-56.1160317615425,13.));
#45109=CARTESIAN_POINT('Ctrl Pts',(34.2272624366034,-56.0513669972495,13.));
#45110=CARTESIAN_POINT('Ctrl Pts',(34.2239018011631,-56.037739760613,13.));
#45111=CARTESIAN_POINT('Ctrl Pts',(34.2203823920739,-56.0241483506747,13.));
#45112=CARTESIAN_POINT('Ctrl Pts',(34.2167036730317,-56.0105963443819,13.));
#45113=CARTESIAN_POINT('Ctrl Pts',(34.2132180506299,-55.9977556853967,13.));
#45114=CARTESIAN_POINT('Ctrl Pts',(34.2095887842124,-55.9849487305413,13.));
#45115=CARTESIAN_POINT('Ctrl Pts',(34.2058217802463,-55.972199063853,13.));
#45116=CARTESIAN_POINT('Ctrl Pts',(34.1873069910902,-55.9095345716819,13.));
#45117=CARTESIAN_POINT('Ctrl Pts',(34.165439151763,-55.8481392502423,13.));
#45118=CARTESIAN_POINT('Ctrl Pts',(34.1402348458363,-55.7883322343982,13.));
#45119=CARTESIAN_POINT('Ctrl Pts',(34.1155097070053,-55.7296622287999,13.));
#45120=CARTESIAN_POINT('Ctrl Pts',(34.0875733532055,-55.6725199271447,13.));
#45121=CARTESIAN_POINT('Ctrl Pts',(34.0564019231628,-55.6172367681066,13.));
#45122=CARTESIAN_POINT('Ctrl Pts',(34.0262427202374,-55.5637488142492,13.));
#45123=CARTESIAN_POINT('Ctrl Pts',(33.9930547257087,-55.512000693163,13.));
#45124=CARTESIAN_POINT('Ctrl Pts',(33.9567849769708,-55.4623304145165,13.));
#45125=CARTESIAN_POINT('Ctrl Pts',(33.9507490318898,-55.4540643778192,13.));
#45126=CARTESIAN_POINT('Ctrl Pts',(33.9446276728718,-55.4458559844853,13.));
#45127=CARTESIAN_POINT('Ctrl Pts',(33.9384205797355,-55.4377069137228,13.));
#45128=CARTESIAN_POINT('Ctrl Pts',(33.931849519021,-55.4290800029336,13.));
#45129=CARTESIAN_POINT('Ctrl Pts',(33.9251823737702,-55.4205195760218,13.));
#45130=CARTESIAN_POINT('Ctrl Pts',(33.9184205240576,-55.4120266023845,13.));
#45131=CARTESIAN_POINT('Origin',(32.5,-56.2916512459885,23.5459252805377));
#45132=CARTESIAN_POINT('Ctrl Pts',(31.4730118547325,-54.5098571360138,21.7959252805377));
#45133=CARTESIAN_POINT('Ctrl Pts',(31.5577251735551,-54.4600031121465,21.7905813053169));
#45134=CARTESIAN_POINT('Ctrl Pts',(32.2577698823492,-54.1148344325097,21.7481913665734));
#45135=CARTESIAN_POINT('Ctrl Pts',(33.9070787897524,-54.3119235461293,21.6687554643073));
#45136=CARTESIAN_POINT('Ctrl Pts',(34.9261604045136,-56.4001058936205,21.5576175737392));
#45137=CARTESIAN_POINT('Ctrl Pts',(33.7248161346881,-58.3888336702692,21.4464796831712));
#45138=CARTESIAN_POINT('Ctrl Pts',(31.4022507610405,-58.458078910143,21.3353417926031));
#45139=CARTESIAN_POINT('Ctrl Pts',(30.0845341595457,-56.5443222204949,21.2242039020351));
#45140=CARTESIAN_POINT('Ctrl Pts',(30.7258866583526,-55.0040437006141,21.1443983980133));
#45141=CARTESIAN_POINT('Ctrl Pts',(31.3789145578642,-54.5633564487824,21.1016388575141));
#45142=CARTESIAN_POINT('Ctrl Pts',(31.4704172621348,-54.5115691325664,21.0959252805377));
#45143=CARTESIAN_POINT('Ctrl Pts',(31.4716734168817,-54.5151354051885,21.8540747194623));
#45144=CARTESIAN_POINT('Ctrl Pts',(31.8806518858733,-54.2831085316556,21.8286245525962));
#45145=CARTESIAN_POINT('Ctrl Pts',(33.082939422317,-54.0422681540074,21.7661284222074));
#45146=CARTESIAN_POINT('Ctrl Pts',(34.7256560234758,-55.3208993649632,21.6665863282959));
#45147=CARTESIAN_POINT('Ctrl Pts',(34.5234929724835,-57.6345755616839,21.5554484377278));
#45148=CARTESIAN_POINT('Ctrl Pts',(32.4687454188576,-58.7202753686332,21.4443105471598));
#45149=CARTESIAN_POINT('Ctrl Pts',(30.4428342940784,-57.5824199368056,21.3331726565917));
#45150=CARTESIAN_POINT('Ctrl Pts',(30.3182849616345,-55.5637298511605,21.2364273806926));
#45151=CARTESIAN_POINT('Ctrl Pts',(31.1131094829785,-54.725326778543,21.1767280683161));
#45152=CARTESIAN_POINT('Ctrl Pts',(31.4749609874599,-54.5139076530798,21.1540747194623));
#45153=CARTESIAN_POINT('Ctrl Pts',(34.0692874532607,-56.8510195406194,22.));
#45154=CARTESIAN_POINT('Ctrl Pts',(33.8832841873681,-57.3728449537375,21.9629540364773));
#45155=CARTESIAN_POINT('Ctrl Pts',(32.9525520823054,-58.2072244344894,21.888862109432));
#45156=CARTESIAN_POINT('Ctrl Pts',(31.1328156874419,-57.7104505124287,21.7777242188639));
#45157=CARTESIAN_POINT('Ctrl Pts',(30.5680805647129,-55.9126012127397,21.6665863282959));
#45158=CARTESIAN_POINT('Ctrl Pts',(31.7699104961033,-54.4629042731491,21.5554484377278));
#45159=CARTESIAN_POINT('Ctrl Pts',(33.6408654404319,-54.686479644594,21.4443105471598));
#45160=CARTESIAN_POINT('Ctrl Pts',(34.4671411285654,-56.3795867334955,21.3331726565917));
#45161=CARTESIAN_POINT('Ctrl Pts',(33.493086107989,-57.992055635258,21.2220347660237));
#45162=CARTESIAN_POINT('Ctrl Pts',(31.6099402690807,-58.0481999689384,21.1108968754557));
#45163=CARTESIAN_POINT('Ctrl Pts',(30.5415300692557,-56.4965179419503,20.9997589848876));
#45164=CARTESIAN_POINT('Ctrl Pts',(31.2657026944405,-54.7573377854331,20.8886210943196));
#45165=CARTESIAN_POINT('Ctrl Pts',(33.1196550861101,-54.4225228075052,20.7774832037515));
#45166=CARTESIAN_POINT('Ctrl Pts',(34.4064234335583,-55.7985469486803,20.6663453131835));
#45167=CARTESIAN_POINT('Ctrl Pts',(33.9482241472934,-57.6259127164007,20.5552074226154));
#45168=CARTESIAN_POINT('Ctrl Pts',(32.1644471988301,-58.2320149921633,20.4440695320474));
#45169=CARTESIAN_POINT('Ctrl Pts',(30.6878063720739,-57.0620797446065,20.3329316414794));
#45170=CARTESIAN_POINT('Ctrl Pts',(30.8698865063133,-55.1869628453693,20.2217937509113));
#45171=CARTESIAN_POINT('Ctrl Pts',(32.5440282170451,-54.3229796221854,20.1106558603433));
#45172=CARTESIAN_POINT('Ctrl Pts',(34.1778702970045,-55.2609439349858,19.9995179697752));
#45173=CARTESIAN_POINT('Ctrl Pts',(34.2759387179252,-57.1423263023633,19.8883800792072));
#45174=CARTESIAN_POINT('Ctrl Pts',(32.7484702637603,-58.2450761614138,19.7772421886392));
#45175=CARTESIAN_POINT('Ctrl Pts',(30.9935741723466,-57.559834032996,19.6661042980711));
#45176=CARTESIAN_POINT('Ctrl Pts',(30.6175267185128,-55.7138098219726,19.5549664075031));
#45177=CARTESIAN_POINT('Ctrl Pts',(31.9645284111714,-54.3966904172637,19.443828516935));
#45178=CARTESIAN_POINT('Ctrl Pts',(33.801653320123,-54.8140501505305,19.332690626367));
#45179=CARTESIAN_POINT('Ctrl Pts',(34.4473601842239,-56.5838749230435,19.221552735799));
#45180=CARTESIAN_POINT('Ctrl Pts',(33.3106261867332,-58.0862240501872,19.1104148452309));
#45181=CARTESIAN_POINT('Ctrl Pts',(31.4319168476016,-57.9459803376678,18.9992769546629));
#45182=CARTESIAN_POINT('Ctrl Pts',(30.530836130646,-56.2915104462365,18.8881390640948));
#45183=CARTESIAN_POINT('Ctrl Pts',(31.4321534351977,-54.63716943038,18.7770011735268));
#45184=CARTESIAN_POINT('Ctrl Pts',(33.3108828106914,-54.4971943834675,18.6658632829587));
#45185=CARTESIAN_POINT('Ctrl Pts',(34.4474019535353,-55.9997060533367,18.5547253923907));
#45186=CARTESIAN_POINT('Ctrl Pts',(33.8014420032617,-57.7694384689282,18.4435875018227));
#45187=CARTESIAN_POINT('Ctrl Pts',(31.9642574280497,-58.1865354801138,18.3324496112546));
#45188=CARTESIAN_POINT('Ctrl Pts',(30.6174441046761,-56.869223462357,18.2213117206866));
#45189=CARTESIAN_POINT('Ctrl Pts',(30.9937555419292,-55.023253044843,18.1101738301185));
#45190=CARTESIAN_POINT('Ctrl Pts',(32.748749613628,-54.3382618854519,17.9990359395505));
#45191=CARTESIAN_POINT('Ctrl Pts',(34.2760603429607,-55.4412301607017,17.8878980489824));
#45192=CARTESIAN_POINT('Ctrl Pts',(34.1777228984872,-57.3225984997459,17.7767601584144));
#45193=CARTESIAN_POINT('Ctrl Pts',(32.5437466583565,-58.2603291256887,17.6656222678464));
#45194=CARTESIAN_POINT('Ctrl Pts',(30.8697286057113,-57.3961065620164,17.5544843772783));
#45195=CARTESIAN_POINT('Ctrl Pts',(30.6879164487935,-55.5209635222086,17.4433464867103));
#45196=CARTESIAN_POINT('Ctrl Pts',(32.1647249167202,-54.3512396961697,17.3322085961422));
#45197=CARTESIAN_POINT('Ctrl Pts',(33.9484144706509,-54.9575965674439,17.2210707055742));
#45198=CARTESIAN_POINT('Ctrl Pts',(34.4063538334575,-56.7850288151988,17.1099328150062));
#45199=CARTESIAN_POINT('Ctrl Pts',(33.1193859129775,-58.1608669785735,16.9987949244381));
#45200=CARTESIAN_POINT('Ctrl Pts',(31.2654870420352,-57.825790783565,16.8876570338701));
#45201=CARTESIAN_POINT('Ctrl Pts',(30.5415518818472,-56.086499271487,16.776519143302));
#45202=CARTESIAN_POINT('Ctrl Pts',(31.6102064945166,-54.534985688252,16.665381252734));
#45203=CARTESIAN_POINT('Ctrl Pts',(33.4932991936999,-54.5913680119554,16.5542433621659));
#45204=CARTESIAN_POINT('Ctrl Pts',(34.46721387611,-56.2040388622933,16.4431054715979));
#45205=CARTESIAN_POINT('Ctrl Pts',(33.6405153879952,-57.8969023210181,16.3319675810299));
#45206=CARTESIAN_POINT('Ctrl Pts',(31.7698902309213,-58.1204612659856,16.2208296904618));
#45207=CARTESIAN_POINT('Ctrl Pts',(30.5675428254988,-56.6700896595285,16.1096917998938));
#45208=CARTESIAN_POINT('Ctrl Pts',(31.1339953874406,-54.8733290813849,15.9985539093257));
#45209=CARTESIAN_POINT('Ctrl Pts',(32.9507674628268,-54.3747748653499,15.8874160187577));
#45210=CARTESIAN_POINT('Ctrl Pts',(34.3549469673911,-55.6307593394112,15.7762781281896));
#45211=CARTESIAN_POINT('Ctrl Pts',(34.0612724762645,-57.4916656705044,15.6651402376216));
#45212=CARTESIAN_POINT('Ctrl Pts',(32.3385475813956,-58.2541851899138,15.5540023470536));
#45213=CARTESIAN_POINT('Ctrl Pts',(30.7636019166367,-57.2203751334699,15.4428644564855));
#45214=CARTESIAN_POINT('Ctrl Pts',(30.7780011089404,-55.3364935710292,15.3317265659175));
#45215=CARTESIAN_POINT('Ctrl Pts',(32.3685654164946,-54.326878659382,15.2205886753495));
#45216=CARTESIAN_POINT('Ctrl Pts',(34.0794332859622,-55.1156423809379,15.1094507847814));
#45217=CARTESIAN_POINT('Ctrl Pts',(34.344627962679,-56.9808203482265,14.9983128942134));
#45218=CARTESIAN_POINT('Ctrl Pts',(32.9214137338773,-58.2151940311284,14.8871750036453));
#45219=CARTESIAN_POINT('Ctrl Pts',(31.1124747588703,-57.6889271671124,14.7760371130773));
#45220=CARTESIAN_POINT('Ctrl Pts',(30.5735533254956,-55.8837178487831,14.6648992225092));
#45221=CARTESIAN_POINT('Ctrl Pts',(31.7979304751287,-54.4518945101648,14.5537613319412));
#45222=CARTESIAN_POINT('Ctrl Pts',(33.6649196338359,-54.7040215463161,14.4426234413732));
#45223=CARTESIAN_POINT('Ctrl Pts',(34.4656450190372,-56.4093237108058,14.3314855508051));
#45224=CARTESIAN_POINT('Ctrl Pts',(33.4671924688587,-58.0069196157817,14.2203476602371));
#45225=CARTESIAN_POINT('Ctrl Pts',(31.5834591995985,-58.0345095641669,14.109209769669));
#45226=CARTESIAN_POINT('Ctrl Pts',(30.5386430838269,-56.4668442614587,13.998071879101));
#45227=CARTESIAN_POINT('Ctrl Pts',(31.289085272834,-54.7388173343014,13.886933988533));
#45228=CARTESIAN_POINT('Ctrl Pts',(33.1478792814865,-54.4321278475435,13.7757960979649));
#45229=CARTESIAN_POINT('Ctrl Pts',(34.4136863832883,-55.8274592952636,13.6646582073969));
#45230=CARTESIAN_POINT('Ctrl Pts',(33.9278258993098,-57.6477147792301,13.5535203168288));
#45231=CARTESIAN_POINT('Ctrl Pts',(32.135157735345,-58.2266620964951,13.4423824262608));
#45232=CARTESIAN_POINT('Ctrl Pts',(30.6762385450867,-57.0346478668883,13.3312445356927));
#45233=CARTESIAN_POINT('Ctrl Pts',(30.8870198365664,-55.1622083892051,13.2201066451247));
#45234=CARTESIAN_POINT('Ctrl Pts',(32.5733973317359,-54.3242660615775,13.1089687545567));
#45235=CARTESIAN_POINT('Ctrl Pts',(34.1941640560837,-55.2856728893477,12.9978308639886));
#45236=CARTESIAN_POINT('Ctrl Pts',(34.2610507255277,-57.170812419961,12.8866929734206));
#45237=CARTESIAN_POINT('Ctrl Pts',(33.2357187233791,-57.885756931559,12.8126010463752));
#45238=CARTESIAN_POINT('Ctrl Pts',(32.6851664226308,-57.947329172377,12.7755550828525));
#45239=CARTESIAN_POINT('Ctrl Pts',(34.1913483771213,-56.8945278288423,22.0748149723825));
#45240=CARTESIAN_POINT('Ctrl Pts',(33.9908775702891,-57.4569414030947,22.0377690088598));
#45241=CARTESIAN_POINT('Ctrl Pts',(32.9877520867064,-58.3562198480608,21.9636770818145));
#45242=CARTESIAN_POINT('Ctrl Pts',(31.0264745706938,-57.8208062977085,21.8525391912464));
#45243=CARTESIAN_POINT('Ctrl Pts',(30.4178137218822,-55.8831182794814,21.7414013006784));
#45244=CARTESIAN_POINT('Ctrl Pts',(31.7131233223058,-54.3206622992213,21.6302634101103));
#45245=CARTESIAN_POINT('Ctrl Pts',(33.7296032235388,-54.5616276117725,21.5191255195423));
#45246=CARTESIAN_POINT('Ctrl Pts',(34.6201475538814,-56.386426453537,21.4079876289742));
#45247=CARTESIAN_POINT('Ctrl Pts',(33.570329450222,-58.1243149802618,21.2968497384062));
#45248=CARTESIAN_POINT('Ctrl Pts',(31.5407104330672,-58.1848262826732,21.1857118478381));
#45249=CARTESIAN_POINT('Ctrl Pts',(30.3891980993524,-56.5124527014652,21.0745739572701));
#45250=CARTESIAN_POINT('Ctrl Pts',(31.1696976769262,-54.6379971776318,20.9634360667021));
#45251=CARTESIAN_POINT('Ctrl Pts',(33.16785254804,-54.2771399182574,20.852298176134));
#45252=CARTESIAN_POINT('Ctrl Pts',(34.5547071690116,-55.7601927478843,20.741160285566));
#45253=CARTESIAN_POINT('Ctrl Pts',(34.0608686325396,-57.7296930578618,20.6300223949979));
#45254=CARTESIAN_POINT('Ctrl Pts',(32.1383475286711,-58.3829386428887,20.5188845044299));
#45255=CARTESIAN_POINT('Ctrl Pts',(30.546851935728,-57.1220045302883,20.4077466138619));
#45256=CARTESIAN_POINT('Ctrl Pts',(30.7430944653628,-55.1010389526641,20.2966087232938));
#45257=CARTESIAN_POINT('Ctrl Pts',(32.5474527807459,-54.1698541532471,20.1854708327258));
#45258=CARTESIAN_POINT('Ctrl Pts',(34.3083769152439,-55.1807743737309,20.0743329421578));
#45259=CARTESIAN_POINT('Ctrl Pts',(34.4140732070395,-57.2084927545773,19.9631950515897));
#45260=CARTESIAN_POINT('Ctrl Pts',(32.7677965572851,-58.3970157244133,19.8520571610217));
#45261=CARTESIAN_POINT('Ctrl Pts',(30.8764026956559,-57.6584747009531,19.7409192704536));
#45262=CARTESIAN_POINT('Ctrl Pts',(30.4711058525308,-55.6688646731958,19.6297813798856));
#45263=CARTESIAN_POINT('Ctrl Pts',(31.9228788353096,-54.2492982559659,19.5186434893175));
#45264=CARTESIAN_POINT('Ctrl Pts',(33.9028973633798,-54.6991206935759,19.4075055987495));
#45265=CARTESIAN_POINT('Ctrl Pts',(34.5988280256839,-56.6066044057275,19.2963677081814));
#45266=CARTESIAN_POINT('Ctrl Pts',(33.3736775933143,-58.2258079192614,19.1852298176134));
#45267=CARTESIAN_POINT('Ctrl Pts',(31.3488401518243,-58.0746558947686,19.0740919270453));
#45268=CARTESIAN_POINT('Ctrl Pts',(30.3776723743012,-56.2914994946751,18.9629540364773));
#45269=CARTESIAN_POINT('Ctrl Pts',(31.3490951414668,-54.5084819942419,18.8518161459093));
#45270=CARTESIAN_POINT('Ctrl Pts',(33.3739541777695,-54.357619532466,18.7406782553412));
#45271=CARTESIAN_POINT('Ctrl Pts',(34.5988730438588,-55.9769982314793,18.6295403647732));
#45272=CARTESIAN_POINT('Ctrl Pts',(33.9026696100581,-57.8843824030853,18.5184024742052));
#45273=CARTESIAN_POINT('Ctrl Pts',(31.9225867748193,-58.3339216837986,18.4072645836371));
#45274=CARTESIAN_POINT('Ctrl Pts',(30.471016812898,-56.9141476718634,18.2961266930691));
#45275=CARTESIAN_POINT('Ctrl Pts',(30.8765981723663,-54.9245956217347,18.184988802501));
#45276=CARTESIAN_POINT('Ctrl Pts',(32.7680976352963,-54.1863250879512,18.073850911933));
#45277=CARTESIAN_POINT('Ctrl Pts',(34.4142042922056,-55.3750834626415,17.9627130213649));
#45278=CARTESIAN_POINT('Ctrl Pts',(34.308218051906,-57.4027867240152,17.8515751307969));
#45279=CARTESIAN_POINT('Ctrl Pts',(32.5471493221093,-58.4134550812175,17.7404372402289));
#45280=CARTESIAN_POINT('Ctrl Pts',(30.7429242830762,-57.4820123251428,17.6292993496608));
#45281=CARTESIAN_POINT('Ctrl Pts',(30.5469705743374,-55.4610185737053,17.5181614590928));
#45282=CARTESIAN_POINT('Ctrl Pts',(32.1386468477676,-54.2003123272238,17.4070235685247));
#45283=CARTESIAN_POINT('Ctrl Pts',(34.0610737594595,-54.8538323104842,17.2958856779567));
#45284=CARTESIAN_POINT('Ctrl Pts',(34.5546321553376,-56.8234042713874,17.1847477873886));
#45285=CARTESIAN_POINT('Ctrl Pts',(33.1675624383217,-58.3062566576536,17.0736098968206));
#45286=CARTESIAN_POINT('Ctrl Pts',(31.1694652508369,-57.9451178634435,16.9624720062526));
#45287=CARTESIAN_POINT('Ctrl Pts',(30.3892216085515,-56.07054232269,16.8513341156845));
#45288=CARTESIAN_POINT('Ctrl Pts',(31.5409973658137,-54.3983502869775,16.7401962251165));
#45289=CARTESIAN_POINT('Ctrl Pts',(33.5705591099766,-54.4591180905408,16.6290583345485));
#45290=CARTESIAN_POINT('Ctrl Pts',(34.620225959811,-56.1972242736255,16.5179204439804));
#45291=CARTESIAN_POINT('Ctrl Pts',(33.7292259436341,-58.0217605353874,16.4067825534124));
#45292=CARTESIAN_POINT('Ctrl Pts',(31.7131014808755,-58.2627081437915,16.2956446628443));
#45293=CARTESIAN_POINT('Ctrl Pts',(30.4172341567137,-56.6995250203255,16.1845067722763));
#45294=CARTESIAN_POINT('Ctrl Pts',(31.0277460290708,-54.7630104056167,16.0733688817082));
#45295=CARTESIAN_POINT('Ctrl Pts',(32.9858286575395,-54.2256780880444,15.9622309911402));
#45296=CARTESIAN_POINT('Ctrl Pts',(34.4992268060413,-55.5793544317117,15.8510931005721));
#45297=CARTESIAN_POINT('Ctrl Pts',(34.182709986298,-57.5850041273934,15.7399552100041));
#45298=CARTESIAN_POINT('Ctrl Pts',(32.3259896326697,-58.4068332632833,15.628817319436));
#45299=CARTESIAN_POINT('Ctrl Pts',(30.6285429420654,-57.2926123105924,15.517679428868));
#45300=CARTESIAN_POINT('Ctrl Pts',(30.6440621195648,-55.2622003445105,15.4065415382999));
#45301=CARTESIAN_POINT('Ctrl Pts',(32.3583422883757,-54.1740564618944,15.295403647732));
#45302=CARTESIAN_POINT('Ctrl Pts',(34.202283363977,-55.0241711031691,15.1842657571639));
#45303=CARTESIAN_POINT('Ctrl Pts',(34.4881051776633,-57.0344246876612,15.0731278665959));
#45304=CARTESIAN_POINT('Ctrl Pts',(32.9541917628979,-58.3648093287921,14.9619899760278));
#45305=CARTESIAN_POINT('Ctrl Pts',(31.0045515020698,-57.7976088426501,14.8508520854598));
#45306=CARTESIAN_POINT('Ctrl Pts',(30.4237121600868,-55.8519883353451,14.7397141948917));
#45307=CARTESIAN_POINT('Ctrl Pts',(31.7433227264704,-54.3087961846243,14.6285763043237));
#45308=CARTESIAN_POINT('Ctrl Pts',(33.7555283788647,-54.5805339421248,14.5174384137556));
#45309=CARTESIAN_POINT('Ctrl Pts',(34.6185350752899,-56.4184764060235,14.4063005231876));
#45310=CARTESIAN_POINT('Ctrl Pts',(33.542421775035,-58.1403350977259,14.2951626326195));
#45311=CARTESIAN_POINT('Ctrl Pts',(31.5121696365421,-58.1700710229889,14.1840247420515));
#45312=CARTESIAN_POINT('Ctrl Pts',(30.3860865609853,-56.4804709690946,14.0728868514835));
#45313=CARTESIAN_POINT('Ctrl Pts',(31.194898978279,-54.6180361852081,13.9617489609154));
#45314=CARTESIAN_POINT('Ctrl Pts',(33.1982720527306,-54.2874920489951,13.8506110703474));
#45315=CARTESIAN_POINT('Ctrl Pts',(34.5625350390512,-55.7913539289481,13.7394731797794));
#45316=CARTESIAN_POINT('Ctrl Pts',(34.0388837861359,-57.7531909093917,13.6283352892113));
#45317=CARTESIAN_POINT('Ctrl Pts',(32.1067798981332,-58.3771693930406,13.5171973986433));
#45318=CARTESIAN_POINT('Ctrl Pts',(30.5343843502893,-57.0924389706047,13.4060595080752));
#45319=CARTESIAN_POINT('Ctrl Pts',(30.7615604451028,-55.0743590673614,13.2949216175072));
#45320=CARTESIAN_POINT('Ctrl Pts',(32.5791062578488,-54.1712406533262,13.1837837269391));
#45321=CARTESIAN_POINT('Ctrl Pts',(34.3259380210302,-55.2074267736726,13.0726458363711));
#45322=CARTESIAN_POINT('Ctrl Pts',(34.3980272100312,-57.239194554091,12.9615079458031));
#45323=CARTESIAN_POINT('Ctrl Pts',(33.2929437441301,-58.0097482451375,12.8874160187577));
#45324=CARTESIAN_POINT('Ctrl Pts',(32.6995688729705,-58.0761096433421,12.850370055235));
#45325=CARTESIAN_POINT('Ctrl Pts',(34.3134093009819,-56.9380361170651,22.149629944765));
#45326=CARTESIAN_POINT('Ctrl Pts',(34.0984709532101,-57.541037852452,22.1125839812423));
#45327=CARTESIAN_POINT('Ctrl Pts',(33.0229520911074,-58.5052152616321,22.0384920541969));
#45328=CARTESIAN_POINT('Ctrl Pts',(30.9201334539457,-57.9311620829884,21.9273541636289));
#45329=CARTESIAN_POINT('Ctrl Pts',(30.2675468790515,-55.8536353462229,21.8162162730609));
#45330=CARTESIAN_POINT('Ctrl Pts',(31.6563361485083,-54.1784203252935,21.7050783824928));
#45331=CARTESIAN_POINT('Ctrl Pts',(33.8183410066456,-54.4367755789509,21.5939404919248));
#45332=CARTESIAN_POINT('Ctrl Pts',(34.7731539791975,-56.3932661735788,21.4828026013567));
#45333=CARTESIAN_POINT('Ctrl Pts',(33.6475727924551,-58.2565743252654,21.3716647107887));
#45334=CARTESIAN_POINT('Ctrl Pts',(31.4714805970539,-58.3214525964081,21.2605268202207));
#45335=CARTESIAN_POINT('Ctrl Pts',(30.236866129449,-56.52838746098,21.1493889296526));
#45336=CARTESIAN_POINT('Ctrl Pts',(31.0736926594119,-54.5186565698304,21.0382510390846));
#45337=CARTESIAN_POINT('Ctrl Pts',(33.2160500099698,-54.1317570290097,20.9271131485165));
#45338=CARTESIAN_POINT('Ctrl Pts',(34.702990904465,-55.7218385470882,20.8159752579485));
#45339=CARTESIAN_POINT('Ctrl Pts',(34.1735131177857,-57.8334733993231,20.7048373673804));
#45340=CARTESIAN_POINT('Ctrl Pts',(32.112247858512,-58.5338622936139,20.5936994768124));
#45341=CARTESIAN_POINT('Ctrl Pts',(30.4058974993822,-57.1819293159701,20.4825615862443));
#45342=CARTESIAN_POINT('Ctrl Pts',(30.6163024244123,-55.0151150599589,20.3714236956763));
#45343=CARTESIAN_POINT('Ctrl Pts',(32.5508773444466,-54.0167286843088,20.2602858051082));
#45344=CARTESIAN_POINT('Ctrl Pts',(34.4388835334834,-55.1006048124759,20.1491479145403));
#45345=CARTESIAN_POINT('Ctrl Pts',(34.5522076961538,-57.2746592067913,20.0380100239721));
#45346=CARTESIAN_POINT('Ctrl Pts',(32.7871228508099,-58.5489552874128,19.9268721334042));
#45347=CARTESIAN_POINT('Ctrl Pts',(30.7592312189651,-57.75711536891,19.8157342428361));
#45348=CARTESIAN_POINT('Ctrl Pts',(30.3246849865488,-55.6239195244191,19.7045963522681));
#45349=CARTESIAN_POINT('Ctrl Pts',(31.8812292594478,-54.1019060946679,19.5934584617));
#45350=CARTESIAN_POINT('Ctrl Pts',(34.0041414066367,-54.5841912366213,19.482320571132));
#45351=CARTESIAN_POINT('Ctrl Pts',(34.7502958671438,-56.6293338884116,19.3711826805639));
#45352=CARTESIAN_POINT('Ctrl Pts',(33.4367289998955,-58.3653917883354,19.2600447899959));
#45353=CARTESIAN_POINT('Ctrl Pts',(31.265763456047,-58.2033314518695,19.1489068994278));
#45354=CARTESIAN_POINT('Ctrl Pts',(30.2245086179564,-56.2914885431138,19.0377690088598));
#45355=CARTESIAN_POINT('Ctrl Pts',(31.2660368477359,-54.379794558104,18.9266311182918));
#45356=CARTESIAN_POINT('Ctrl Pts',(33.4370255448476,-54.2180446814646,18.8154932277237));
#45357=CARTESIAN_POINT('Ctrl Pts',(34.7503441341823,-55.9542904096218,18.7043553371557));
#45358=CARTESIAN_POINT('Ctrl Pts',(34.0038972168544,-57.9993263372426,18.5932174465876));
#45359=CARTESIAN_POINT('Ctrl Pts',(31.8809161215888,-58.4813078874833,18.4820795560196));
#45360=CARTESIAN_POINT('Ctrl Pts',(30.3245895211199,-56.9590718813699,18.3709416654516));
#45361=CARTESIAN_POINT('Ctrl Pts',(30.7594408028035,-54.8259381986264,18.2598037748835));
#45362=CARTESIAN_POINT('Ctrl Pts',(32.7874456569645,-54.0343882904504,18.1486658843155));
#45363=CARTESIAN_POINT('Ctrl Pts',(34.5523482414506,-55.3089367645812,18.0375279937474));
#45364=CARTESIAN_POINT('Ctrl Pts',(34.4387132053247,-57.4829749482845,17.9263901031794));
#45365=CARTESIAN_POINT('Ctrl Pts',(32.550551985862,-58.5665810367465,17.8152522126113));
#45366=CARTESIAN_POINT('Ctrl Pts',(30.6161199604412,-57.5679180882693,17.7041143220433));
#45367=CARTESIAN_POINT('Ctrl Pts',(30.4060246998813,-55.4010736252019,17.5929764314753));
#45368=CARTESIAN_POINT('Ctrl Pts',(32.112568778815,-54.0493849582779,17.4818385409072));
#45369=CARTESIAN_POINT('Ctrl Pts',(34.1737330482682,-54.7500680535245,17.3707006503392));
#45370=CARTESIAN_POINT('Ctrl Pts',(34.7029104772176,-56.861779727576,17.2595627597711));
#45371=CARTESIAN_POINT('Ctrl Pts',(33.2157389636658,-58.4516463367337,17.1484248692031));
#45372=CARTESIAN_POINT('Ctrl Pts',(31.0734434596386,-58.0644449433221,17.037286978635));
#45373=CARTESIAN_POINT('Ctrl Pts',(30.2368913352558,-56.054585373893,16.926149088067));
#45374=CARTESIAN_POINT('Ctrl Pts',(31.4717882371109,-54.261714885703,16.815011197499));
#45375=CARTESIAN_POINT('Ctrl Pts',(33.6478190262533,-54.3268681691261,16.7038733069309));
#45376=CARTESIAN_POINT('Ctrl Pts',(34.773238043512,-56.1904096849576,16.5927354163629));
#45377=CARTESIAN_POINT('Ctrl Pts',(33.8179364992731,-58.1466187497568,16.4815975257948));
#45378=CARTESIAN_POINT('Ctrl Pts',(31.6563127308296,-58.4049550215973,16.3704596352268));
#45379=CARTESIAN_POINT('Ctrl Pts',(30.2669254879288,-56.7289603811226,16.2593217446588));
#45380=CARTESIAN_POINT('Ctrl Pts',(30.9214966707009,-54.6526917298483,16.1481838540907));
#45381=CARTESIAN_POINT('Ctrl Pts',(33.0208898522522,-54.0765813107389,16.0370459635227));
#45382=CARTESIAN_POINT('Ctrl Pts',(34.6435066446914,-55.5279495240122,15.9259080729546));
#45383=CARTESIAN_POINT('Ctrl Pts',(34.3041474963316,-57.6783425842823,15.8147701823866));
#45384=CARTESIAN_POINT('Ctrl Pts',(32.3134316839437,-58.5594813366529,15.7036322918185));
#45385=CARTESIAN_POINT('Ctrl Pts',(30.4934839674941,-57.364849487715,15.5924944012505));
#45386=CARTESIAN_POINT('Ctrl Pts',(30.5101231301891,-55.1879071179918,15.4813565106825));
#45387=CARTESIAN_POINT('Ctrl Pts',(32.3481191602569,-54.0212342644067,15.3702186201144));
#45388=CARTESIAN_POINT('Ctrl Pts',(34.3251334419918,-54.9326998254003,15.2590807295464));
#45389=CARTESIAN_POINT('Ctrl Pts',(34.6315823926476,-57.0880290270961,15.1479428389784));
#45390=CARTESIAN_POINT('Ctrl Pts',(32.9869697919185,-58.5144246264557,15.0368049484103));
#45391=CARTESIAN_POINT('Ctrl Pts',(30.8966282452692,-57.9062905181877,14.9256670578423));
#45392=CARTESIAN_POINT('Ctrl Pts',(30.2738709946779,-55.8202588219069,14.8145291672742));
#45393=CARTESIAN_POINT('Ctrl Pts',(31.6887149778122,-54.1656978590839,14.7033912767062));
#45394=CARTESIAN_POINT('Ctrl Pts',(33.8461371238934,-54.4570463379336,14.5922533861381));
#45395=CARTESIAN_POINT('Ctrl Pts',(34.7714251315425,-56.4276291012412,14.4811154955701));
#45396=CARTESIAN_POINT('Ctrl Pts',(33.6176510812112,-58.2737505796701,14.369977605002));
#45397=CARTESIAN_POINT('Ctrl Pts',(31.4408800734857,-58.3056324818108,14.258839714434));
#45398=CARTESIAN_POINT('Ctrl Pts',(30.2335300381437,-56.4940976767304,14.147701823866));
#45399=CARTESIAN_POINT('Ctrl Pts',(31.1007126837241,-54.4972550361148,14.0365639332979));
#45400=CARTESIAN_POINT('Ctrl Pts',(33.2486648239746,-54.1428562504465,13.9254260427299));
#45401=CARTESIAN_POINT('Ctrl Pts',(34.7113836948142,-55.7552485626328,13.8142881521619));
#45402=CARTESIAN_POINT('Ctrl Pts',(34.149941672962,-57.8586670395533,13.7031502615938));
#45403=CARTESIAN_POINT('Ctrl Pts',(32.0784020609214,-58.5276766895861,13.5920123710258));
#45404=CARTESIAN_POINT('Ctrl Pts',(30.3925301554919,-57.1502300743212,13.4808744804577));
#45405=CARTESIAN_POINT('Ctrl Pts',(30.6361010536393,-54.9865097455178,13.3697365898897));
#45406=CARTESIAN_POINT('Ctrl Pts',(32.5848151839618,-54.0182152450749,13.2585986993216));
#45407=CARTESIAN_POINT('Ctrl Pts',(34.4577119859767,-55.1291806579975,13.1474608087536));
#45408=CARTESIAN_POINT('Ctrl Pts',(34.5350036945349,-57.3075766882209,13.0363229181856));
#45409=CARTESIAN_POINT('Ctrl Pts',(33.3501687648811,-58.133739558716,12.9622309911402));
#45410=CARTESIAN_POINT('Ctrl Pts',(32.7139713233101,-58.2048901143072,12.9251850276175));
#45411=CARTESIAN_POINT('Ctrl Pts',(34.4354702248424,-56.9815444052879,22.2244449171475));
#45412=CARTESIAN_POINT('Ctrl Pts',(34.2060643361312,-57.6251343018092,22.1873989536248));
#45413=CARTESIAN_POINT('Ctrl Pts',(33.0581520955084,-58.6542106752035,22.1133070265794));
#45414=CARTESIAN_POINT('Ctrl Pts',(30.8137923371976,-58.0415178682682,22.0021691360114));
#45415=CARTESIAN_POINT('Ctrl Pts',(30.1172800362208,-55.8241524129646,21.8910312454434));
#45416=CARTESIAN_POINT('Ctrl Pts',(31.5995489747108,-54.0361783513656,21.7798933548753));
#45417=CARTESIAN_POINT('Ctrl Pts',(33.9070787897524,-54.3119235461293,21.6687554643073));
#45418=CARTESIAN_POINT('Ctrl Pts',(34.9261604045136,-56.4001058936205,21.5576175737392));
#45419=CARTESIAN_POINT('Ctrl Pts',(33.7248161346881,-58.3888336702692,21.4464796831712));
#45420=CARTESIAN_POINT('Ctrl Pts',(31.4022507610405,-58.458078910143,21.3353417926031));
#45421=CARTESIAN_POINT('Ctrl Pts',(30.0845341595457,-56.5443222204949,21.2242039020351));
#45422=CARTESIAN_POINT('Ctrl Pts',(30.9776876418977,-54.3993159620292,21.113066011467));
#45423=CARTESIAN_POINT('Ctrl Pts',(33.2642474718997,-53.9863741397619,21.001928120899));
#45424=CARTESIAN_POINT('Ctrl Pts',(34.8512746399183,-55.6834843462923,20.890790230331));
#45425=CARTESIAN_POINT('Ctrl Pts',(34.2861576030319,-57.9372537407841,20.7796523397629));
#45426=CARTESIAN_POINT('Ctrl Pts',(32.086148188353,-58.6847859443394,20.6685144491949));
#45427=CARTESIAN_POINT('Ctrl Pts',(30.2649430630364,-57.2418541016519,20.5573765586268));
#45428=CARTESIAN_POINT('Ctrl Pts',(30.4895103834618,-54.9291911672537,20.4462386680588));
#45429=CARTESIAN_POINT('Ctrl Pts',(32.5543019081473,-53.8636032153705,20.3351007774907));
#45430=CARTESIAN_POINT('Ctrl Pts',(34.5693901517228,-55.0204352512209,20.2239628869227));
#45431=CARTESIAN_POINT('Ctrl Pts',(34.6903421852681,-57.3408256590054,20.1128249963547));
#45432=CARTESIAN_POINT('Ctrl Pts',(32.8064491443347,-58.7008948504122,20.0016871057866));
#45433=CARTESIAN_POINT('Ctrl Pts',(30.6420597422744,-57.8557560368671,19.8905492152186));
#45434=CARTESIAN_POINT('Ctrl Pts',(30.1782641205668,-55.5789743756423,19.7794113246505));
#45435=CARTESIAN_POINT('Ctrl Pts',(31.8395796835861,-53.9545139333701,19.6682734340825));
#45436=CARTESIAN_POINT('Ctrl Pts',(34.1053854498936,-54.4692617796666,19.5571355435145));
#45437=CARTESIAN_POINT('Ctrl Pts',(34.9017637086038,-56.6520633710957,19.4459976529464));
#45438=CARTESIAN_POINT('Ctrl Pts',(33.4997804064766,-58.5049756574095,19.3348597623784));
#45439=CARTESIAN_POINT('Ctrl Pts',(31.1826867602698,-58.3320070089704,19.2237218718103));
#45440=CARTESIAN_POINT('Ctrl Pts',(30.0713448616115,-56.2914775915524,19.1125839812423));
#45441=CARTESIAN_POINT('Ctrl Pts',(31.1829785540051,-54.2511071219659,19.0014460906742));
#45442=CARTESIAN_POINT('Ctrl Pts',(33.5000969119256,-54.0784698304632,18.8903082001062));
#45443=CARTESIAN_POINT('Ctrl Pts',(34.9018152245058,-55.9315825877644,18.7791703095382));
#45444=CARTESIAN_POINT('Ctrl Pts',(34.1051248236507,-58.1142702713998,18.6680324189701));
#45445=CARTESIAN_POINT('Ctrl Pts',(31.8392454683584,-58.628694091168,18.5568945284021));
#45446=CARTESIAN_POINT('Ctrl Pts',(30.1781622293417,-57.0039960908763,18.445756637834));
#45447=CARTESIAN_POINT('Ctrl Pts',(30.6422834332407,-54.7272807755182,18.334618747266));
#45448=CARTESIAN_POINT('Ctrl Pts',(32.8067936786327,-53.8824514929497,18.2234808566979));
#45449=CARTESIAN_POINT('Ctrl Pts',(34.6904921906955,-55.242790066521,18.1123429661299));
#45450=CARTESIAN_POINT('Ctrl Pts',(34.5692083587434,-57.5631631725538,18.0012050755619));
#45451=CARTESIAN_POINT('Ctrl Pts',(32.5539546496148,-58.7197069922754,17.8900671849938));
#45452=CARTESIAN_POINT('Ctrl Pts',(30.4893156378063,-57.6538238513956,17.7789292944258));
#45453=CARTESIAN_POINT('Ctrl Pts',(30.2650788254252,-55.3411286766987,17.6677914038578));
#45454=CARTESIAN_POINT('Ctrl Pts',(32.0864907098624,-53.8984575893318,17.5566535132897));
#45455=CARTESIAN_POINT('Ctrl Pts',(34.2863923370768,-54.6463037965649,17.4455156227217));
#45456=CARTESIAN_POINT('Ctrl Pts',(34.8511887990977,-56.9001551837646,17.3343777321536));
#45457=CARTESIAN_POINT('Ctrl Pts',(33.26391548901,-58.5970360158138,17.2232398415856));
#45458=CARTESIAN_POINT('Ctrl Pts',(30.9774216684404,-58.1837720232006,17.1121019510175));
#45459=CARTESIAN_POINT('Ctrl Pts',(30.0845610619601,-56.038628425096,17.0009640604495));
#45460=CARTESIAN_POINT('Ctrl Pts',(31.4025791084081,-54.1250794844285,16.8898261698814));
#45461=CARTESIAN_POINT('Ctrl Pts',(33.7250789425299,-54.1946182477115,16.7786882793134));
#45462=CARTESIAN_POINT('Ctrl Pts',(34.9262501272131,-56.1835950962899,16.6675503887454));
#45463=CARTESIAN_POINT('Ctrl Pts',(33.9066470549119,-58.2714769641261,16.5564124981774));
#45464=CARTESIAN_POINT('Ctrl Pts',(31.5995239807838,-58.5472018994033,16.4452746076093));
#45465=CARTESIAN_POINT('Ctrl Pts',(30.1166168191438,-56.7583957419196,16.3341367170413));
#45466=CARTESIAN_POINT('Ctrl Pts',(30.8152473123311,-54.5423730540802,16.2229988264732));
#45467=CARTESIAN_POINT('Ctrl Pts',(33.0559510469649,-53.9274845334332,16.1118609359052));
#45468=CARTESIAN_POINT('Ctrl Pts',(34.7877864833415,-55.4765446163129,16.0007230453371));
#45469=CARTESIAN_POINT('Ctrl Pts',(34.4255850063652,-57.7716810411711,15.8895851547691));
#45470=CARTESIAN_POINT('Ctrl Pts',(32.3008737352177,-58.7121294100224,15.778447264201));
#45471=CARTESIAN_POINT('Ctrl Pts',(30.3584249929227,-57.4370866648374,15.667309373633));
#45472=CARTESIAN_POINT('Ctrl Pts',(30.3761841408135,-55.1136138914732,15.5561714830649));
#45473=CARTESIAN_POINT('Ctrl Pts',(32.3378960321381,-53.8684120669189,15.4450335924969));
#45474=CARTESIAN_POINT('Ctrl Pts',(34.4479835200066,-54.8412285476316,15.3338957019289));
#45475=CARTESIAN_POINT('Ctrl Pts',(34.7750596076319,-57.1416333665308,15.2227578113608));
#45476=CARTESIAN_POINT('Ctrl Pts',(33.019747820939,-58.6640399241195,15.1116199207928));
#45477=CARTESIAN_POINT('Ctrl Pts',(30.7887049884687,-58.0149721937253,15.0004820302248));
#45478=CARTESIAN_POINT('Ctrl Pts',(30.124029829269,-55.7885293084688,14.8893441396567));
#45479=CARTESIAN_POINT('Ctrl Pts',(31.634107229154,-54.0225995335434,14.7782062490887));
#45480=CARTESIAN_POINT('Ctrl Pts',(33.9367458689222,-54.3335587337424,14.6670683585206));
#45481=CARTESIAN_POINT('Ctrl Pts',(34.9243151877952,-56.4367817964588,14.5559304679526));
#45482=CARTESIAN_POINT('Ctrl Pts',(33.6928803873874,-58.4071660616143,14.4447925773845));
#45483=CARTESIAN_POINT('Ctrl Pts',(31.3695905104292,-58.4411939406326,14.3336546868165));
#45484=CARTESIAN_POINT('Ctrl Pts',(30.0809735153021,-56.5077243843663,14.2225167962484));
#45485=CARTESIAN_POINT('Ctrl Pts',(31.0065263891691,-54.3764738870214,14.1113789056804));
#45486=CARTESIAN_POINT('Ctrl Pts',(33.2990575952187,-53.9982204518981,14.0002410151124));
#45487=CARTESIAN_POINT('Ctrl Pts',(34.8602323505772,-55.7191431963173,13.8891031245444));
#45488=CARTESIAN_POINT('Ctrl Pts',(34.2609995597881,-57.9641431697149,13.7779652339763));
#45489=CARTESIAN_POINT('Ctrl Pts',(32.0500242237095,-58.6781839861316,13.6668273434083));
#45490=CARTESIAN_POINT('Ctrl Pts',(30.2506759606945,-57.2080211780376,13.5556894528402));
#45491=CARTESIAN_POINT('Ctrl Pts',(30.5106416621758,-54.8986604236742,13.4445515622722));
#45492=CARTESIAN_POINT('Ctrl Pts',(32.5905241100746,-53.8651898368237,13.3334136717041));
#45493=CARTESIAN_POINT('Ctrl Pts',(34.5894859509232,-55.0509345423224,13.2222757811361));
#45494=CARTESIAN_POINT('Ctrl Pts',(34.6719801790384,-57.3759588223509,13.111137890568));
#45495=CARTESIAN_POINT('Ctrl Pts',(33.4073937856322,-58.2577308722946,13.0370459635227));
#45496=CARTESIAN_POINT('Ctrl Pts',(32.7283737736498,-58.3336705852723,13.));
#45497=CARTESIAN_POINT('Ctrl Pts',(34.0692874532607,-56.8510195406194,22.));
#45498=CARTESIAN_POINT('Ctrl Pts',(34.0553305059908,-56.9114179004368,22.));
#45499=CARTESIAN_POINT('Ctrl Pts',(34.0377835201511,-56.9707365361936,22.));
#45500=CARTESIAN_POINT('Ctrl Pts',(34.0169460819157,-57.0288042521055,22.));
#45501=CARTESIAN_POINT('Ctrl Pts',(33.9947315403597,-57.0907095436108,22.));
#45502=CARTESIAN_POINT('Ctrl Pts',(33.9687774174651,-57.1511938546456,22.));
#45503=CARTESIAN_POINT('Ctrl Pts',(33.9393848899745,-57.2100521415653,22.));
#45504=CARTESIAN_POINT('Ctrl Pts',(33.9136664284202,-57.2615531426201,22.));
#45505=CARTESIAN_POINT('Ctrl Pts',(33.8853142547964,-57.311809621018,22.));
#45506=CARTESIAN_POINT('Ctrl Pts',(33.8544948148302,-57.3606781624786,22.));
#45507=CARTESIAN_POINT('Ctrl Pts',(33.8390317669678,-57.3851969920354,22.));
#45508=CARTESIAN_POINT('Ctrl Pts',(33.8229471373042,-57.4093662970867,22.));
#45509=CARTESIAN_POINT('Ctrl Pts',(33.8062591811805,-57.433166856092,22.));
#45510=CARTESIAN_POINT('Ctrl Pts',(33.7986346988524,-57.4440409823294,22.));
#45511=CARTESIAN_POINT('Ctrl Pts',(33.7908831156841,-57.4548394646073,22.));
#45512=CARTESIAN_POINT('Ctrl Pts',(33.7830191798169,-57.4655431489118,22.));
#45513=CARTESIAN_POINT('Ctrl Pts',(33.7433624663838,-57.5195203110236,22.));
#45514=CARTESIAN_POINT('Ctrl Pts',(33.7007840160683,-57.5711878026522,22.));
#45515=CARTESIAN_POINT('Ctrl Pts',(33.6555819715537,-57.6203464168852,22.));
#45516=CARTESIAN_POINT('Ctrl Pts',(33.6095776366613,-57.6703775465898,22.));
#45517=CARTESIAN_POINT('Ctrl Pts',(33.5608552987539,-57.7178108518911,22.));
#45518=CARTESIAN_POINT('Ctrl Pts',(33.5096779792476,-57.7624205360752,22.));
#45519=CARTESIAN_POINT('Ctrl Pts',(33.4668687974159,-57.7997359738536,22.));
#45520=CARTESIAN_POINT('Ctrl Pts',(33.4223407450877,-57.8350756827256,22.));
#45521=CARTESIAN_POINT('Ctrl Pts',(33.3762247079518,-57.868292142162,22.));
#45522=CARTESIAN_POINT('Ctrl Pts',(33.3549779646033,-57.883595746557,22.));
#45523=CARTESIAN_POINT('Ctrl Pts',(33.3333938801028,-57.8984484230851,22.));
#45524=CARTESIAN_POINT('Ctrl Pts',(33.3114840048116,-57.9128343832935,22.));
#45525=CARTESIAN_POINT('Ctrl Pts',(33.3019191647095,-57.9191146294054,22.));
#45526=CARTESIAN_POINT('Ctrl Pts',(33.2922923777588,-57.9253057104171,22.));
#45527=CARTESIAN_POINT('Ctrl Pts',(33.2826166374558,-57.9313989825921,22.));
#45528=CARTESIAN_POINT('Ctrl Pts',(33.2232320152038,-57.9687962932948,22.));
#45529=CARTESIAN_POINT('Ctrl Pts',(33.1618957172908,-58.0025854530623,22.));
#45530=CARTESIAN_POINT('Ctrl Pts',(33.098892967176,-58.0325387704389,22.));
#45531=CARTESIAN_POINT('Ctrl Pts',(33.042562016297,-58.0593201227882,22.));
#45532=CARTESIAN_POINT('Ctrl Pts',(32.9848978605095,-58.0830352046633,22.));
#45533=CARTESIAN_POINT('Ctrl Pts',(32.9260772832472,-58.1034986372925,22.));
#45534=CARTESIAN_POINT('Ctrl Pts',(32.8619970286521,-58.1257918896507,22.));
#45535=CARTESIAN_POINT('Ctrl Pts',(32.7965441149125,-58.1442273323774,22.));
#45536=CARTESIAN_POINT('Ctrl Pts',(32.730026067277,-58.1589105502836,22.));
#45537=CARTESIAN_POINT('Ctrl Pts',(32.7043629429453,-58.1645754376355,22.));
#45538=CARTESIAN_POINT('Ctrl Pts',(32.6785410407308,-58.1696813145168,22.));
#45539=CARTESIAN_POINT('Ctrl Pts',(32.6525772949454,-58.1742323470501,22.));
#45540=CARTESIAN_POINT('Ctrl Pts',(32.6411872717866,-58.1762288373247,22.));
#45541=CARTESIAN_POINT('Ctrl Pts',(32.6297705135365,-58.1781183496249,22.));
#45542=CARTESIAN_POINT('Ctrl Pts',(32.6183418171879,-58.1798993771494,22.));
#45543=CARTESIAN_POINT('Ctrl Pts',(32.5492442274453,-58.1906674215051,22.));
#45544=CARTESIAN_POINT('Ctrl Pts',(32.479587866051,-58.1974963222448,22.));
#45545=CARTESIAN_POINT('Ctrl Pts',(32.4097184968816,-58.2005474581315,22.));
#45546=CARTESIAN_POINT('Ctrl Pts',(32.3382311065792,-58.2036692516239,22.));
#45547=CARTESIAN_POINT('Ctrl Pts',(32.2665198680808,-58.2028364327161,22.));
#45548=CARTESIAN_POINT('Ctrl Pts',(32.1949302795595,-58.1981713779293,22.));
#45549=CARTESIAN_POINT('Ctrl Pts',(32.1401596273564,-58.1946023101568,22.));
#45550=CARTESIAN_POINT('Ctrl Pts',(32.0854595447263,-58.1887891069564,22.));
#45551=CARTESIAN_POINT('Ctrl Pts',(32.0309802701291,-58.1807666255705,22.));
#45552=CARTESIAN_POINT('Ctrl Pts',(31.9970690900463,-58.1757729502141,22.));
#45553=CARTESIAN_POINT('Ctrl Pts',(31.9632434082193,-58.1699229342579,22.));
#45554=CARTESIAN_POINT('Ctrl Pts',(31.9295394677181,-58.1632216306219,22.));
#45555=CARTESIAN_POINT('Ctrl Pts',(31.9106295175814,-58.1594617937684,22.));
#45556=CARTESIAN_POINT('Ctrl Pts',(31.891751681419,-58.155432366917,22.));
#45557=CARTESIAN_POINT('Ctrl Pts',(31.8729463795953,-58.1511420898522,22.));
#45558=CARTESIAN_POINT('Ctrl Pts',(31.8000212116739,-58.1345048043509,22.));
#45559=CARTESIAN_POINT('Ctrl Pts',(31.7281115869712,-58.1139365946325,22.));
#45560=CARTESIAN_POINT('Ctrl Pts',(31.6575884718452,-58.0895522802127,22.));
#45561=CARTESIAN_POINT('Ctrl Pts',(31.6048403101262,-58.0713138947113,22.));
#45562=CARTESIAN_POINT('Ctrl Pts',(31.5528674074715,-58.0509395358532,22.));
#45563=CARTESIAN_POINT('Ctrl Pts',(31.5018252351578,-58.0284581681729,22.));
#45564=CARTESIAN_POINT('Ctrl Pts',(31.485902371771,-58.0214449920071,22.));
#45565=CARTESIAN_POINT('Ctrl Pts',(31.4700701035634,-58.0142266520142,22.));
#45566=CARTESIAN_POINT('Ctrl Pts',(31.454333225623,-58.006803707092,22.));
#45567=CARTESIAN_POINT('Ctrl Pts',(31.4391437429471,-57.9996389636323,22.));
#45568=CARTESIAN_POINT('Ctrl Pts',(31.4240509122119,-57.9922872148314,22.));
#45569=CARTESIAN_POINT('Ctrl Pts',(31.4090641623495,-57.9847522751711,22.));
#45570=CARTESIAN_POINT('Ctrl Pts',(31.3417651306224,-57.9509161100309,22.));
#45571=CARTESIAN_POINT('Ctrl Pts',(31.2765704047207,-57.9133737616735,22.));
#45572=CARTESIAN_POINT('Ctrl Pts',(31.2138523221447,-57.8722119391925,22.));
#45573=CARTESIAN_POINT('Ctrl Pts',(31.1658528011688,-57.8407098957555,22.));
#45574=CARTESIAN_POINT('Ctrl Pts',(31.119303757925,-57.8070868161123,22.));
#45575=CARTESIAN_POINT('Ctrl Pts',(31.0743783982804,-57.7713618605751,22.));
#45576=CARTESIAN_POINT('Ctrl Pts',(31.0639523774024,-57.7630710169349,22.));
#45577=CARTESIAN_POINT('Ctrl Pts',(31.0536138415293,-57.75466689798,22.));
#45578=CARTESIAN_POINT('Ctrl Pts',(31.0433632440414,-57.7461514510325,22.));
#45579=CARTESIAN_POINT('Ctrl Pts',(31.6652099567911,-54.8483531313949,20.8714803633902));
#45580=CARTESIAN_POINT('Ctrl Pts',(31.5910191767377,-54.8903425066551,20.8771939403667));
#45581=CARTESIAN_POINT('Ctrl Pts',(31.5202697708326,-54.9380868086678,20.8829075173431));
#45582=CARTESIAN_POINT('Ctrl Pts',(31.453999322188,-54.9913986485313,20.8886210943196));
#45583=CARTESIAN_POINT('Ctrl Pts',(31.0243118193789,-55.3370645042722,20.9256670578423));
#45584=CARTESIAN_POINT('Ctrl Pts',(30.7829209443173,-55.9167912231112,20.9627130213649));
#45585=CARTESIAN_POINT('Ctrl Pts',(30.840293873424,-56.4652682536955,20.9997589848876));
#45586=CARTESIAN_POINT('Ctrl Pts',(30.8976668025307,-57.0137452842797,21.0368049484103));
#45587=CARTESIAN_POINT('Ctrl Pts',(31.2538035358057,-57.5309726266091,21.073850911933));
#45588=CARTESIAN_POINT('Ctrl Pts',(31.7457295422612,-57.780228908827,21.1108968754557));
#45589=CARTESIAN_POINT('Ctrl Pts',(32.2376555487168,-58.029485191045,21.1479428389784));
#45590=CARTESIAN_POINT('Ctrl Pts',(32.8653708283529,-58.0107704131515,21.184988802501));
#45591=CARTESIAN_POINT('Ctrl Pts',(33.3415709716003,-57.7326682072443,21.2220347660237));
#45592=CARTESIAN_POINT('Ctrl Pts',(33.8177711148478,-57.4545660013372,21.2590807295464));
#45593=CARTESIAN_POINT('Ctrl Pts',(34.1424561217066,-56.9170763674163,21.2961266930691));
#45594=CARTESIAN_POINT('Ctrl Pts',(34.1670860104471,-56.366147035639,21.3331726565918));
#45595=CARTESIAN_POINT('Ctrl Pts',(34.1917158991876,-55.8152177038616,21.3702186201144));
#45596=CARTESIAN_POINT('Ctrl Pts',(33.9162906698097,-55.2508486742278,21.4072645836371));
#45597=CARTESIAN_POINT('Ctrl Pts',(33.4667522310661,-54.9314015975034,21.4443105471598));
#45598=CARTESIAN_POINT('Ctrl Pts',(33.0172137923224,-54.611954520779,21.4813565106825));
#45599=CARTESIAN_POINT('Ctrl Pts',(32.3935621442128,-54.5374293969641,21.5184024742052));
#45600=CARTESIAN_POINT('Ctrl Pts',(31.881431331593,-54.741782991655,21.5554484377278));
#45601=CARTESIAN_POINT('Ctrl Pts',(31.8075551488135,-54.7712615216341,21.5607924129486));
#45602=CARTESIAN_POINT('Ctrl Pts',(31.7359995810404,-54.8065431837032,21.5661363881694));
#45603=CARTESIAN_POINT('Ctrl Pts',(31.6673136634551,-54.8469650373412,21.5714803633902));
#45604=CARTESIAN_POINT('Ctrl Pts',(30.5157034944333,-56.8250975324092,22.));
#45605=CARTESIAN_POINT('Ctrl Pts',(30.3383199129809,-56.1652717359215,21.9629540364773));
#45606=CARTESIAN_POINT('Ctrl Pts',(30.6971298707754,-54.6659551967235,21.888862109432));
#45607=CARTESIAN_POINT('Ctrl Pts',(32.8915770858133,-53.893318629858,21.7777242188639));
#45608=CARTESIAN_POINT('Ctrl Pts',(34.7256560234758,-55.3208993649632,21.6665863282959));
#45609=CARTESIAN_POINT('Ctrl Pts',(34.5234929724835,-57.6345755616839,21.5554484377278));
#45610=CARTESIAN_POINT('Ctrl Pts',(32.4687454188576,-58.7202753686332,21.4443105471598));
#45611=CARTESIAN_POINT('Ctrl Pts',(30.4428342940784,-57.5824199368056,21.3331726565917));
#45612=CARTESIAN_POINT('Ctrl Pts',(30.2997559892121,-55.2634130835607,21.2220347660237));
#45613=CARTESIAN_POINT('Ctrl Pts',(32.1706430815574,-53.8854124812074,21.1108968754557));
#45614=CARTESIAN_POINT('Ctrl Pts',(34.3429657642116,-54.7099453599153,20.9997589848876));
#45615=CARTESIAN_POINT('Ctrl Pts',(34.8284152391772,-56.982193672835,20.8886210943196));
#45616=CARTESIAN_POINT('Ctrl Pts',(33.18263271582,-58.6223996095028,20.7774832037515));
#45617=CARTESIAN_POINT('Ctrl Pts',(30.9120322857351,-58.1292356735021,20.6663453131835));
#45618=CARTESIAN_POINT('Ctrl Pts',(30.0949149346206,-55.954114599854,20.5552074226154));
#45619=CARTESIAN_POINT('Ctrl Pts',(31.479200108132,-54.0879422836221,20.4440695320474));
#45620=CARTESIAN_POINT('Ctrl Pts',(33.7978345552324,-54.2388509530007,20.3329316414794));
#45621=CARTESIAN_POINT('Ctrl Pts',(34.9285465373885,-56.2687104209716,20.2217937509113));
#45622=CARTESIAN_POINT('Ctrl Pts',(33.836382221401,-58.3195681810162,20.1106558603433));
#45623=CARTESIAN_POINT('Ctrl Pts',(31.5210121579647,-58.5142504249981,19.9995179697753));
#45624=CARTESIAN_POINT('Ctrl Pts',(30.101720741136,-56.674562508041,19.8883800792072));
#45625=CARTESIAN_POINT('Ctrl Pts',(30.8776015421154,-54.4843915336431,19.7772421886392));
#45626=CARTESIAN_POINT('Ctrl Pts',(33.1384820439343,-53.9484258880498,19.6661042980711));
#45627=CARTESIAN_POINT('Ctrl Pts',(34.8149526935151,-55.5572409773789,19.5549664075031));
#45628=CARTESIAN_POINT('Ctrl Pts',(34.3725208876465,-57.8382701189333,19.443828516935));
#45629=CARTESIAN_POINT('Ctrl Pts',(32.2161494783462,-58.7036614639378,19.332690626367));
#45630=CARTESIAN_POINT('Ctrl Pts',(30.3195896701685,-57.3613125035426,19.221552735799));
#45631=CARTESIAN_POINT('Ctrl Pts',(30.4187841646359,-55.039890462752,19.1104148452309));
#45632=CARTESIAN_POINT('Ctrl Pts',(32.4229391156972,-53.8642192630766,18.9992769546629));
#45633=CARTESIAN_POINT('Ctrl Pts',(34.4976287681445,-54.9104040861686,18.8881390640948));
#45634=CARTESIAN_POINT('Ctrl Pts',(34.7438661544311,-57.2208600991234,18.7770011735268));
#45635=CARTESIAN_POINT('Ctrl Pts',(32.9362674024074,-58.680800710823,18.6658632829587));
#45636=CARTESIAN_POINT('Ctrl Pts',(30.7293481493445,-57.9539257225797,18.5547253923907));
#45637=CARTESIAN_POINT('Ctrl Pts',(30.1431266157477,-55.7055520544289,18.4435875018226));
#45638=CARTESIAN_POINT('Ctrl Pts',(31.7141780195173,-53.993641623134,18.3324496112546));
#45639=CARTESIAN_POINT('Ctrl Pts',(34.004501193851,-54.3851254608373,18.2213117206866));
#45640=CARTESIAN_POINT('Ctrl Pts',(34.9177373632483,-56.5216739711635,18.1101738301186));
#45641=CARTESIAN_POINT('Ctrl Pts',(33.6179911050581,-58.4476800725016,17.9990359395505));
#45642=CARTESIAN_POINT('Ctrl Pts',(31.2949349095266,-58.4002485379024,17.8878980489825));
#45643=CARTESIAN_POINT('Ctrl Pts',(30.074888457673,-56.4227939888948,17.7767601584144));
#45644=CARTESIAN_POINT('Ctrl Pts',(31.0745741031467,-54.3253030000451,17.6656222678464));
#45645=CARTESIAN_POINT('Ctrl Pts',(33.3789682374394,-54.0276328606134,17.5544843772783));
#45646=CARTESIAN_POINT('Ctrl Pts',(34.8788327758259,-55.8022444250302,17.4433464867103));
#45647=CARTESIAN_POINT('Ctrl Pts',(34.2013246967004,-58.0248156029211,17.3322085961422));
#45648=CARTESIAN_POINT('Ctrl Pts',(31.9665748283507,-58.6610017894909,17.2210707055742));
#45649=CARTESIAN_POINT('Ctrl Pts',(30.2200750690644,-57.1284945533304,17.1099328150062));
#45650=CARTESIAN_POINT('Ctrl Pts',(30.5604164551708,-54.8300151475112,16.9987949244381));
#45651=CARTESIAN_POINT('Ctrl Pts',(32.6760806562327,-53.8693878387091,16.8876570338701));
#45652=CARTESIAN_POINT('Ctrl Pts',(34.6305762357544,-55.1258856969254,16.776519143302));
#45653=CARTESIAN_POINT('Ctrl Pts',(34.6349312243122,-57.4494219828794,16.665381252734));
#45654=CARTESIAN_POINT('Ctrl Pts',(32.68515945149,-58.7132375833447,16.5542433621659));
#45655=CARTESIAN_POINT('Ctrl Pts',(30.5659091328683,-57.7605477465697,16.4431054715979));
#45656=CARTESIAN_POINT('Ctrl Pts',(30.2169541190139,-55.4633602843959,16.3319675810299));
#45657=CARTESIAN_POINT('Ctrl Pts',(31.9576968915284,-53.9243169328214,16.2208296904618));
#45658=CARTESIAN_POINT('Ctrl Pts',(34.1948158493603,-54.5521215254954,16.1096917998938));
#45659=CARTESIAN_POINT('Ctrl Pts',(34.880650639758,-56.7721373989267,15.9985539093257));
#45660=CARTESIAN_POINT('Ctrl Pts',(33.387448901162,-58.5523588475275,15.8874160187577));
#45661=CARTESIAN_POINT('Ctrl Pts',(31.0819551189947,-58.2633289901972,15.7762781281897));
#45662=CARTESIAN_POINT('Ctrl Pts',(30.0744138980993,-56.1696001333952,15.6651402376216));
#45663=CARTESIAN_POINT('Ctrl Pts',(31.287039144361,-54.1875860438059,15.5540023470536));
#45664=CARTESIAN_POINT('Ctrl Pts',(33.6099012175602,-54.1314466960922,15.4428644564855));
#45665=CARTESIAN_POINT('Ctrl Pts',(34.9168581194719,-56.052567070093,15.3317265659175));
#45666=CARTESIAN_POINT('Ctrl Pts',(34.0116373750326,-58.1925239040739,15.2205886753494));
#45667=CARTESIAN_POINT('Ctrl Pts',(31.722797799219,-58.5925904319764,15.1094507847814));
#45668=CARTESIAN_POINT('Ctrl Pts',(30.1453402095973,-56.8865812380664,14.9983128942134));
#45669=CARTESIAN_POINT('Ctrl Pts',(30.7231294343029,-54.6360258563356,14.8871750036453));
#45670=CARTESIAN_POINT('Ctrl Pts',(32.9273084298409,-53.9008832080614,14.7760371130773));
#45671=CARTESIAN_POINT('Ctrl Pts',(34.7403671916158,-55.3540375815297,14.6648992225092));
#45672=CARTESIAN_POINT('Ctrl Pts',(34.5027924192342,-57.6654005284896,14.5537613319412));
#45673=CARTESIAN_POINT('Ctrl Pts',(32.4320391047204,-58.7193548713018,14.4426234413732));
#45674=CARTESIAN_POINT('Ctrl Pts',(30.423491023484,-57.5512051672244,14.3314855508051));
#45675=CARTESIAN_POINT('Ctrl Pts',(30.3155954476549,-55.2301702471532,14.2203476602371));
#45676=CARTESIAN_POINT('Ctrl Pts',(32.2071095510683,-53.8807233800597,14.109209769669));
#45677=CARTESIAN_POINT('Ctrl Pts',(34.3667107654437,-54.7380212138032,13.998071879101));
#45678=CARTESIAN_POINT('Ctrl Pts',(34.817688121868,-57.0173840749687,13.886933988533));
#45679=CARTESIAN_POINT('Ctrl Pts',(33.1472639077745,-58.6324557555082,13.7757960979649));
#45680=CARTESIAN_POINT('Ctrl Pts',(30.8843823888257,-58.1050019311361,13.6646582073969));
#45681=CARTESIAN_POINT('Ctrl Pts',(30.1003126229301,-55.9176887906373,13.5535203168288));
#45682=CARTESIAN_POINT('Ctrl Pts',(31.5126666412308,-54.0728255670594,13.4423824262608));
#45683=CARTESIAN_POINT('Ctrl Pts',(33.8288126996591,-54.2585627611561,13.3312445356927));
#45684=CARTESIAN_POINT('Ctrl Pts',(34.9285321027134,-56.3058411531895,13.2201066451247));
#45685=CARTESIAN_POINT('Ctrl Pts',(33.8056871835127,-58.3388651889264,13.1089687545567));
#45686=CARTESIAN_POINT('Ctrl Pts',(31.4871369476881,-58.5005967837941,12.9978308639886));
#45687=CARTESIAN_POINT('Ctrl Pts',(30.0968376198178,-56.6352191751132,12.8866929734206));
#45688=CARTESIAN_POINT('Ctrl Pts',(30.6354003368774,-55.1906968075749,12.8126010463752));
#45689=CARTESIAN_POINT('Ctrl Pts',(31.1506898940641,-54.7420190959222,12.7755550828525));
#45690=CARTESIAN_POINT('Ctrl Pts',(30.6408436601533,-56.7914556061658,22.0748149723825));
#45691=CARTESIAN_POINT('Ctrl Pts',(30.4746468195516,-56.1732418919889,22.0377690088598));
#45692=CARTESIAN_POINT('Ctrl Pts',(30.8108283357527,-54.7684801331151,21.9636770818145));
#45693=CARTESIAN_POINT('Ctrl Pts',(32.8668821769258,-54.0445700885952,21.8525391912464));
#45694=CARTESIAN_POINT('Ctrl Pts',(34.5852944581392,-55.3821200801757,21.7414013006784));
#45695=CARTESIAN_POINT('Ctrl Pts',(34.3958808715705,-57.5498836968623,21.6302634101103));
#45696=CARTESIAN_POINT('Ctrl Pts',(32.4707164969967,-58.5671135683042,21.5191255195423));
#45697=CARTESIAN_POINT('Ctrl Pts',(30.5725699745224,-57.5010172797825,21.4079876289742));
#45698=CARTESIAN_POINT('Ctrl Pts',(30.4385149394808,-55.3282591857862,21.2968497384062));
#45699=CARTESIAN_POINT('Ctrl Pts',(32.1914140597047,-54.0371625432278,21.1857118478382));
#45700=CARTESIAN_POINT('Ctrl Pts',(34.2267386577773,-54.8096960454343,21.0745739572701));
#45701=CARTESIAN_POINT('Ctrl Pts',(34.6815731376677,-56.9386444383886,20.9634360667021));
#45702=CARTESIAN_POINT('Ctrl Pts',(33.1395823093187,-58.4754103689113,20.852298176134));
#45703=CARTESIAN_POINT('Ctrl Pts',(31.0121778750478,-58.0133479424405,20.741160285566));
#45704=CARTESIAN_POINT('Ctrl Pts',(30.2465922382936,-55.9754014346165,20.6300223949979));
#45705=CARTESIAN_POINT('Ctrl Pts',(31.5435771139257,-54.2269197519468,20.5188845044299));
#45706=CARTESIAN_POINT('Ctrl Pts',(33.7159862876659,-54.3683113275636,20.4077466138618));
#45707=CARTESIAN_POINT('Ctrl Pts',(34.7753896299934,-56.2701571899581,20.2966087232938));
#45708=CARTESIAN_POINT('Ctrl Pts',(33.7521029354263,-58.1916770817759,20.1854708327258));
#45709=CARTESIAN_POINT('Ctrl Pts',(31.5827522761609,-58.3740816403382,20.0743329421578));
#45710=CARTESIAN_POINT('Ctrl Pts',(30.2529688348836,-56.6504141115414,19.9631950515897));
#45711=CARTESIAN_POINT('Ctrl Pts',(30.9799185150647,-54.5983668288006,19.8520571610217));
#45712=CARTESIAN_POINT('Ctrl Pts',(33.0982160108274,-54.0962019934801,19.7409192704536));
#45713=CARTESIAN_POINT('Ctrl Pts',(34.6689596108847,-55.6035567484657,19.6297813798856));
#45714=CARTESIAN_POINT('Ctrl Pts',(34.2544298798073,-57.7407322048549,19.5186434893175));
#45715=CARTESIAN_POINT('Ctrl Pts',(32.2340505839621,-58.5515474237501,19.4075055987495));
#45716=CARTESIAN_POINT('Ctrl Pts',(30.4570978042841,-57.2938540432475,19.2963677081814));
#45717=CARTESIAN_POINT('Ctrl Pts',(30.5500365726333,-55.1188330761249,19.1852298176134));
#45718=CARTESIAN_POINT('Ctrl Pts',(32.4277989800396,-54.017305880809,19.0740919270454));
#45719=CARTESIAN_POINT('Ctrl Pts',(34.3716477998814,-54.9975127909389,18.9629540364773));
#45720=CARTESIAN_POINT('Ctrl Pts',(34.6023561625367,-57.1622593055708,18.8518161459093));
#45721=CARTESIAN_POINT('Ctrl Pts',(32.9087540872943,-58.5301283898668,18.7406782553412));
#45722=CARTESIAN_POINT('Ctrl Pts',(30.8410147603584,-57.8490939583302,18.6295403647732));
#45723=CARTESIAN_POINT('Ctrl Pts',(30.2917634374419,-55.7425145495774,18.5184024742052));
#45724=CARTESIAN_POINT('Ctrl Pts',(31.763736083339,-54.1385661866874,18.4072645836371));
#45725=CARTESIAN_POINT('Ctrl Pts',(33.9096194419575,-54.5053609962191,18.2961266930691));
#45726=CARTESIAN_POINT('Ctrl Pts',(34.76526213918,-56.507167529275,18.184988802501));
#45727=CARTESIAN_POINT('Ctrl Pts',(33.5474847105914,-58.3117095641174,18.073850911933));
#45728=CARTESIAN_POINT('Ctrl Pts',(31.3709326471137,-58.2672693113572,17.9627130213649));
#45729=CARTESIAN_POINT('Ctrl Pts',(30.2278287362275,-56.4145234383323,17.8515751307969));
#45730=CARTESIAN_POINT('Ctrl Pts',(31.1644689512469,-54.4493112541897,17.7404372402289));
#45731=CARTESIAN_POINT('Ctrl Pts',(33.3235358811423,-54.1704137580971,17.6292993496608));
#45732=CARTESIAN_POINT('Ctrl Pts',(34.7288110794959,-55.8331089911409,17.5181614590928));
#45733=CARTESIAN_POINT('Ctrl Pts',(34.0940302203501,-57.9155131502695,17.4070235685247));
#45734=CARTESIAN_POINT('Ctrl Pts',(32.0002154229856,-58.5115780925633,17.2958856779567));
#45735=CARTESIAN_POINT('Ctrl Pts',(30.3638591169049,-57.0757188165044,17.1847477873887));
#45736=CARTESIAN_POINT('Ctrl Pts',(30.6827367866064,-54.9221936012214,17.0736098968206));
#45737=CARTESIAN_POINT('Ctrl Pts',(32.6649760846935,-54.0221484988997,16.9624720062526));
#45738=CARTESIAN_POINT('Ctrl Pts',(34.4962109015046,-55.1994049989002,16.8513341156845));
#45739=CARTESIAN_POINT('Ctrl Pts',(34.5002912415971,-57.3764068757753,16.7401962251165));
#45740=CARTESIAN_POINT('Ctrl Pts',(32.6734823234101,-58.5605196227416,16.6290583345484));
#45741=CARTESIAN_POINT('Ctrl Pts',(30.6878830671827,-57.6679114137473,16.5179204439804));
#45742=CARTESIAN_POINT('Ctrl Pts',(30.3609349903662,-55.5155966653537,16.4067825534124));
#45743=CARTESIAN_POINT('Ctrl Pts',(31.9918973755156,-54.0736134756683,16.2956446628443));
#45744=CARTESIAN_POINT('Ctrl Pts',(34.0879318551292,-54.661825411425,16.1845067722763));
#45745=CARTESIAN_POINT('Ctrl Pts',(34.730514299375,-56.7418354170223,16.0733688817082));
#45746=CARTESIAN_POINT('Ctrl Pts',(33.331481709642,-58.4097867454715,15.9622309911402));
#45747=CARTESIAN_POINT('Ctrl Pts',(31.1713844814461,-58.138984629884,15.8510931005721));
#45748=CARTESIAN_POINT('Ctrl Pts',(30.2273841048744,-56.1772973179708,15.7399552100041));
#45749=CARTESIAN_POINT('Ctrl Pts',(31.3635348303941,-54.3202794529553,15.6288173194361));
#45750=CARTESIAN_POINT('Ctrl Pts',(33.5399050139139,-54.2676805475375,15.517679428868));
#45751=CARTESIAN_POINT('Ctrl Pts',(34.7644383451369,-56.0676449746849,15.4065415383));
#45752=CARTESIAN_POINT('Ctrl Pts',(33.916305578051,-58.0726448845937,15.2954036477319));
#45753=CARTESIAN_POINT('Ctrl Pts',(31.7718122544331,-58.4474811147761,15.1842657571639));
#45754=CARTESIAN_POINT('Ctrl Pts',(30.2938374304302,-56.8490618262287,15.0731278665959));
#45755=CARTESIAN_POINT('Ctrl Pts',(30.8351882301686,-54.7404382942198,14.9619899760278));
#45756=CARTESIAN_POINT('Ctrl Pts',(32.9003601146199,-54.0516576047429,14.8508520854598));
#45757=CARTESIAN_POINT('Ctrl Pts',(34.5990778627046,-55.4131684266541,14.7397141948917));
#45758=CARTESIAN_POINT('Ctrl Pts',(34.3764858039968,-57.5787646792667,14.6285763043237));
#45759=CARTESIAN_POINT('Ctrl Pts',(32.4363250759318,-58.566251122372,14.5174384137557));
#45760=CARTESIAN_POINT('Ctrl Pts',(30.5544465922265,-57.4717710776141,14.4063005231876));
#45761=CARTESIAN_POINT('Ctrl Pts',(30.453355478433,-55.2971128173437,14.2951626326196));
#45762=CARTESIAN_POINT('Ctrl Pts',(32.2255807620059,-54.032769161441,14.1840247420515));
#45763=CARTESIAN_POINT('Ctrl Pts',(34.2489861744446,-54.8360012884289,14.0728868514835));
#45764=CARTESIAN_POINT('Ctrl Pts',(34.6715225287503,-56.9716155488275,13.9617489609154));
#45765=CARTESIAN_POINT('Ctrl Pts',(33.1064440441824,-58.4848323215015,13.8506110703474));
#45766=CARTESIAN_POINT('Ctrl Pts',(30.9862717259461,-57.9906425072238,13.7394731797794));
#45767=CARTESIAN_POINT('Ctrl Pts',(30.2516495200117,-55.9412728283577,13.6283352892113));
#45768=CARTESIAN_POINT('Ctrl Pts',(31.5749330715706,-54.2127563749734,13.5171973986433));
#45769=CARTESIAN_POINT('Ctrl Pts',(33.7450107875055,-54.386780005505,13.4060595080752));
#45770=CARTESIAN_POINT('Ctrl Pts',(34.7753761056448,-56.3049462630692,13.2949216175072));
#45771=CARTESIAN_POINT('Ctrl Pts',(33.7233436879389,-58.2097571189556,13.1837837269391));
#45772=CARTESIAN_POINT('Ctrl Pts',(31.5510134146689,-58.3612890695026,13.0726458363711));
#45773=CARTESIAN_POINT('Ctrl Pts',(30.248393668858,-56.6135519759491,12.9615079458031));
#45774=CARTESIAN_POINT('Ctrl Pts',(30.7529917906697,-55.2601287803101,12.8874160187577));
#45775=CARTESIAN_POINT('Ctrl Pts',(31.2357844803776,-54.8397470430914,12.850370055235));
#45776=CARTESIAN_POINT('Ctrl Pts',(30.7659838258732,-56.7578136799224,22.149629944765));
#45777=CARTESIAN_POINT('Ctrl Pts',(30.6109737261224,-56.1812120480563,22.1125839812423));
#45778=CARTESIAN_POINT('Ctrl Pts',(30.92452680073,-54.8710050695067,22.0384920541969));
#45779=CARTESIAN_POINT('Ctrl Pts',(32.8421872680382,-54.1958215473323,21.9273541636289));
#45780=CARTESIAN_POINT('Ctrl Pts',(34.4449328928026,-55.4433407953882,21.8162162730609));
#45781=CARTESIAN_POINT('Ctrl Pts',(34.2682687706575,-57.4651918320407,21.7050783824928));
#45782=CARTESIAN_POINT('Ctrl Pts',(32.4726875751358,-58.4139517679752,21.5939404919248));
#45783=CARTESIAN_POINT('Ctrl Pts',(30.7023056549664,-57.4196146227593,21.4828026013567));
#45784=CARTESIAN_POINT('Ctrl Pts',(30.5772738897495,-55.3931052880118,21.3716647107887));
#45785=CARTESIAN_POINT('Ctrl Pts',(32.2121850378521,-54.188912605248,21.2605268202206));
#45786=CARTESIAN_POINT('Ctrl Pts',(34.1105115513431,-54.9094467309535,21.1493889296526));
#45787=CARTESIAN_POINT('Ctrl Pts',(34.5347310361582,-56.8950952039421,21.0382510390846));
#45788=CARTESIAN_POINT('Ctrl Pts',(33.0965319028176,-58.3284211283198,20.9271131485165));
#45789=CARTESIAN_POINT('Ctrl Pts',(31.1123234643604,-57.897460211379,20.8159752579485));
#45790=CARTESIAN_POINT('Ctrl Pts',(30.3982695419666,-55.996688269379,20.7048373673804));
#45791=CARTESIAN_POINT('Ctrl Pts',(31.6079541197193,-54.3658972202713,20.5936994768124));
#45792=CARTESIAN_POINT('Ctrl Pts',(33.6341380200995,-54.4977717021264,20.4825615862443));
#45793=CARTESIAN_POINT('Ctrl Pts',(34.6222327225984,-56.2716039589447,20.3714236956763));
#45794=CARTESIAN_POINT('Ctrl Pts',(33.6678236494516,-58.0637859825356,20.2602858051083));
#45795=CARTESIAN_POINT('Ctrl Pts',(31.6444923943572,-58.2339128556783,20.1491479145402));
#45796=CARTESIAN_POINT('Ctrl Pts',(30.4042169286311,-56.6262657150416,20.0380100239722));
#45797=CARTESIAN_POINT('Ctrl Pts',(31.082235488014,-54.712342123958,19.9268721334041));
#45798=CARTESIAN_POINT('Ctrl Pts',(33.0579499777204,-54.2439780989105,19.8157342428361));
#45799=CARTESIAN_POINT('Ctrl Pts',(34.5229665282544,-55.6498725195525,19.7045963522681));
#45800=CARTESIAN_POINT('Ctrl Pts',(34.1363388719681,-57.6431942907767,19.5934584617));
#45801=CARTESIAN_POINT('Ctrl Pts',(32.251951689578,-58.3994333835621,19.482320571132));
#45802=CARTESIAN_POINT('Ctrl Pts',(30.5946059383997,-57.2263955829524,19.371182680564));
#45803=CARTESIAN_POINT('Ctrl Pts',(30.6812889806306,-55.1977756894976,19.2600447899959));
#45804=CARTESIAN_POINT('Ctrl Pts',(32.4326588443821,-54.1703924985415,19.1489068994279));
#45805=CARTESIAN_POINT('Ctrl Pts',(34.2456668316182,-55.0846214957091,19.0377690088598));
#45806=CARTESIAN_POINT('Ctrl Pts',(34.4608461706423,-57.1036585120183,18.9266311182918));
#45807=CARTESIAN_POINT('Ctrl Pts',(32.8812407721812,-58.3794560689106,18.8154932277237));
#45808=CARTESIAN_POINT('Ctrl Pts',(30.9526813713723,-57.7442621940807,18.7043553371557));
#45809=CARTESIAN_POINT('Ctrl Pts',(30.440400259136,-55.7794770447258,18.5932174465876));
#45810=CARTESIAN_POINT('Ctrl Pts',(31.8132941471606,-54.283490750241,18.4820795560196));
#45811=CARTESIAN_POINT('Ctrl Pts',(33.8147376900639,-54.625596531601,18.3709416654515));
#45812=CARTESIAN_POINT('Ctrl Pts',(34.6127869151118,-56.4926610873864,18.2598037748835));
#45813=CARTESIAN_POINT('Ctrl Pts',(33.4769783161247,-58.1757390557333,18.1486658843155));
#45814=CARTESIAN_POINT('Ctrl Pts',(31.4469303847008,-58.134290084812,18.0375279937474));
#45815=CARTESIAN_POINT('Ctrl Pts',(30.380769014782,-56.4062528877698,17.9263901031794));
#45816=CARTESIAN_POINT('Ctrl Pts',(31.2543637993471,-54.5733195083342,17.8152522126114));
#45817=CARTESIAN_POINT('Ctrl Pts',(33.2681035248451,-54.313194655581,17.7041143220433));
#45818=CARTESIAN_POINT('Ctrl Pts',(34.5787893831658,-55.8639735572515,17.5929764314753));
#45819=CARTESIAN_POINT('Ctrl Pts',(33.9867357439999,-57.8062106976179,17.4818385409072));
#45820=CARTESIAN_POINT('Ctrl Pts',(32.0338560176206,-58.3621543956356,17.3707006503392));
#45821=CARTESIAN_POINT('Ctrl Pts',(30.5076431647456,-57.0229430796785,17.2595627597712));
#45822=CARTESIAN_POINT('Ctrl Pts',(30.8050571180421,-55.0143720549317,17.1484248692031));
#45823=CARTESIAN_POINT('Ctrl Pts',(32.6538715131543,-54.1749091590902,17.0372869786351));
#45824=CARTESIAN_POINT('Ctrl Pts',(34.3618455672548,-55.2729243008751,16.926149088067));
#45825=CARTESIAN_POINT('Ctrl Pts',(34.365651258882,-57.3033917686712,16.815011197499));
#45826=CARTESIAN_POINT('Ctrl Pts',(32.6618051953302,-58.4078016621386,16.7038733069309));
#45827=CARTESIAN_POINT('Ctrl Pts',(30.809857001497,-57.5752750809248,16.5927354163629));
#45828=CARTESIAN_POINT('Ctrl Pts',(30.5049158617185,-55.5678330463115,16.4815975257948));
#45829=CARTESIAN_POINT('Ctrl Pts',(32.0260978595028,-54.2229100185152,16.3704596352268));
#45830=CARTESIAN_POINT('Ctrl Pts',(33.9810478608982,-54.7715292973546,16.2593217446587));
#45831=CARTESIAN_POINT('Ctrl Pts',(34.580377958992,-56.7115334351178,16.1481838540907));
#45832=CARTESIAN_POINT('Ctrl Pts',(33.2755145181221,-58.2672146434156,16.0370459635227));
#45833=CARTESIAN_POINT('Ctrl Pts',(31.2608138438975,-58.0146402695707,15.9259080729546));
#45834=CARTESIAN_POINT('Ctrl Pts',(30.3803543116496,-56.1849945025465,15.8147701823866));
#45835=CARTESIAN_POINT('Ctrl Pts',(31.4400305164272,-54.4529728621045,15.7036322918186));
#45836=CARTESIAN_POINT('Ctrl Pts',(33.4699088102677,-54.4039143989829,15.5924944012505));
#45837=CARTESIAN_POINT('Ctrl Pts',(34.6120185708019,-56.0827228792766,15.4813565106825));
#45838=CARTESIAN_POINT('Ctrl Pts',(33.8209737810693,-57.9527658651135,15.3702186201144));
#45839=CARTESIAN_POINT('Ctrl Pts',(31.8208267096472,-58.3023717975756,15.2590807295464));
#45840=CARTESIAN_POINT('Ctrl Pts',(30.4423346512631,-56.811542414391,15.1479428389783));
#45841=CARTESIAN_POINT('Ctrl Pts',(30.9472470260342,-54.844850732104,15.0368049484103));
#45842=CARTESIAN_POINT('Ctrl Pts',(32.873411799399,-54.2024320014244,14.9256670578423));
#45843=CARTESIAN_POINT('Ctrl Pts',(34.4577885337935,-55.4722992717786,14.8145291672742));
#45844=CARTESIAN_POINT('Ctrl Pts',(34.2501791887593,-57.4921288300438,14.7033912767062));
#45845=CARTESIAN_POINT('Ctrl Pts',(32.4406110471432,-58.4131473734422,14.5922533861381));
#45846=CARTESIAN_POINT('Ctrl Pts',(30.6854021609689,-57.3923369880037,14.4811154955701));
#45847=CARTESIAN_POINT('Ctrl Pts',(30.5911155092111,-55.3640553875343,14.3699776050021));
#45848=CARTESIAN_POINT('Ctrl Pts',(32.2440519729435,-54.1848149428223,14.258839714434));
#45849=CARTESIAN_POINT('Ctrl Pts',(34.1312615834455,-54.9339813630547,14.147701823866));
#45850=CARTESIAN_POINT('Ctrl Pts',(34.5253569356325,-56.9258470226863,14.0365639332979));
#45851=CARTESIAN_POINT('Ctrl Pts',(33.0656241805903,-58.3372088874948,13.9254260427299));
#45852=CARTESIAN_POINT('Ctrl Pts',(31.0881610630664,-57.8762830833116,13.8142881521618));
#45853=CARTESIAN_POINT('Ctrl Pts',(30.4029864170935,-55.9648568660781,13.7031502615938));
#45854=CARTESIAN_POINT('Ctrl Pts',(31.6371995019102,-54.3526871828874,13.5920123710258));
#45855=CARTESIAN_POINT('Ctrl Pts',(33.661208875352,-54.5149972498541,13.4808744804577));
#45856=CARTESIAN_POINT('Ctrl Pts',(34.6222201085763,-56.3040513729489,13.3697365898897));
#45857=CARTESIAN_POINT('Ctrl Pts',(33.6410001923651,-58.0806490489848,13.2585986993216));
#45858=CARTESIAN_POINT('Ctrl Pts',(31.6148898816497,-58.221981355211,13.1474608087536));
#45859=CARTESIAN_POINT('Ctrl Pts',(30.3999497178981,-56.591884776785,13.0363229181856));
#45860=CARTESIAN_POINT('Ctrl Pts',(30.8705832444619,-55.3295607530454,12.9622309911402));
#45861=CARTESIAN_POINT('Ctrl Pts',(31.320879066691,-54.9374749902607,12.9251850276175));
#45862=CARTESIAN_POINT('Ctrl Pts',(30.8911239915931,-56.724171753679,22.2244449171475));
#45863=CARTESIAN_POINT('Ctrl Pts',(30.7473006326931,-56.1891822041237,22.1873989536248));
#45864=CARTESIAN_POINT('Ctrl Pts',(31.0382252657072,-54.9735300058983,22.1133070265794));
#45865=CARTESIAN_POINT('Ctrl Pts',(32.8174923591507,-54.3470730060696,22.0021691360114));
#45866=CARTESIAN_POINT('Ctrl Pts',(34.3045713274659,-55.5045615106007,21.8910312454433));
#45867=CARTESIAN_POINT('Ctrl Pts',(34.1406566697445,-57.3804999672191,21.7798933548753));
#45868=CARTESIAN_POINT('Ctrl Pts',(32.474658653275,-58.2607899676461,21.6687554643073));
#45869=CARTESIAN_POINT('Ctrl Pts',(30.8320413354104,-57.3382119657362,21.5576175737392));
#45870=CARTESIAN_POINT('Ctrl Pts',(30.7160328400182,-55.4579513902373,21.4464796831712));
#45871=CARTESIAN_POINT('Ctrl Pts',(32.2329560159993,-54.3406626672684,21.3353417926031));
#45872=CARTESIAN_POINT('Ctrl Pts',(33.9942844449089,-55.0091974164724,21.2242039020351));
#45873=CARTESIAN_POINT('Ctrl Pts',(34.3878889346486,-56.8515459694957,21.1130660114671));
#45874=CARTESIAN_POINT('Ctrl Pts',(33.0534814963164,-58.1814318877282,21.001928120899));
#45875=CARTESIAN_POINT('Ctrl Pts',(31.212469053673,-57.7815724803176,20.890790230331));
#45876=CARTESIAN_POINT('Ctrl Pts',(30.5499468456396,-56.0179751041415,20.7796523397629));
#45877=CARTESIAN_POINT('Ctrl Pts',(31.672331125513,-54.504874688596,20.6685144491949));
#45878=CARTESIAN_POINT('Ctrl Pts',(33.5522897525329,-54.6272320766892,20.5573765586268));
#45879=CARTESIAN_POINT('Ctrl Pts',(34.4690758152034,-56.2730507279312,20.4462386680588));
#45880=CARTESIAN_POINT('Ctrl Pts',(33.5835443634768,-57.9358948832953,20.3351007774908));
#45881=CARTESIAN_POINT('Ctrl Pts',(31.7062325125535,-58.0937440710183,20.2239628869227));
#45882=CARTESIAN_POINT('Ctrl Pts',(30.5554650223786,-56.6021173185421,20.1128249963547));
#45883=CARTESIAN_POINT('Ctrl Pts',(31.1845524609633,-54.8263174191155,20.0016871057866));
#45884=CARTESIAN_POINT('Ctrl Pts',(33.0176839446135,-54.3917542043407,19.8905492152186));
#45885=CARTESIAN_POINT('Ctrl Pts',(34.3769734456241,-55.6961882906394,19.7794113246506));
#45886=CARTESIAN_POINT('Ctrl Pts',(34.018247864129,-57.5456563766984,19.6682734340825));
#45887=CARTESIAN_POINT('Ctrl Pts',(32.2698527951939,-58.2473193433743,19.5571355435145));
#45888=CARTESIAN_POINT('Ctrl Pts',(30.7321140725153,-57.1589371226574,19.4459976529464));
#45889=CARTESIAN_POINT('Ctrl Pts',(30.812541388628,-55.2767183028703,19.3348597623784));
#45890=CARTESIAN_POINT('Ctrl Pts',(32.4375187087245,-54.3234791162739,19.2237218718103));
#45891=CARTESIAN_POINT('Ctrl Pts',(34.119685863355,-55.1717302004793,19.1125839812423));
#45892=CARTESIAN_POINT('Ctrl Pts',(34.3193361787479,-57.0450577184658,19.0014460906742));
#45893=CARTESIAN_POINT('Ctrl Pts',(32.8537274570681,-58.2287837479543,18.8903082001062));
#45894=CARTESIAN_POINT('Ctrl Pts',(31.0643479823862,-57.6394304298313,18.7791703095382));
#45895=CARTESIAN_POINT('Ctrl Pts',(30.5890370808301,-55.8164395398742,18.6680324189701));
#45896=CARTESIAN_POINT('Ctrl Pts',(31.8628522109823,-54.4284153137945,18.5568945284021));
#45897=CARTESIAN_POINT('Ctrl Pts',(33.7198559381704,-54.7458320669827,18.4457566378341));
#45898=CARTESIAN_POINT('Ctrl Pts',(34.4603116910435,-56.4781546454979,18.334618747266));
#45899=CARTESIAN_POINT('Ctrl Pts',(33.406471921658,-58.039768547349,18.223480856698));
#45900=CARTESIAN_POINT('Ctrl Pts',(31.522928122288,-58.0013108582667,18.1123429661299));
#45901=CARTESIAN_POINT('Ctrl Pts',(30.5337092933365,-56.3979823372073,18.0012050755619));
#45902=CARTESIAN_POINT('Ctrl Pts',(31.3442586474474,-54.6973277624788,17.8900671849938));
#45903=CARTESIAN_POINT('Ctrl Pts',(33.212671168548,-54.4559755530648,17.7789292944258));
#45904=CARTESIAN_POINT('Ctrl Pts',(34.4287676868358,-55.8948381233622,17.6677914038578));
#45905=CARTESIAN_POINT('Ctrl Pts',(33.8794412676495,-57.6969082449663,17.5566535132897));
#45906=CARTESIAN_POINT('Ctrl Pts',(32.0674966122556,-58.2127306987079,17.4455156227217));
#45907=CARTESIAN_POINT('Ctrl Pts',(30.6514272125861,-56.9701673428525,17.3343777321536));
#45908=CARTESIAN_POINT('Ctrl Pts',(30.9273774494778,-55.1065505086419,17.2232398415856));
#45909=CARTESIAN_POINT('Ctrl Pts',(32.6427669416151,-54.3276698192808,17.1121019510176));
#45910=CARTESIAN_POINT('Ctrl Pts',(34.2274802330049,-55.3464436028499,17.0009640604495));
#45911=CARTESIAN_POINT('Ctrl Pts',(34.2310112761669,-57.2303766615672,16.8898261698815));
#45912=CARTESIAN_POINT('Ctrl Pts',(32.6501280672502,-58.2550837015356,16.7786882793134));
#45913=CARTESIAN_POINT('Ctrl Pts',(30.9318309358114,-57.4826387481023,16.6675503887454));
#45914=CARTESIAN_POINT('Ctrl Pts',(30.6488967330708,-55.6200694272693,16.5564124981773));
#45915=CARTESIAN_POINT('Ctrl Pts',(32.0602983434901,-54.3722065613621,16.4452746076093));
#45916=CARTESIAN_POINT('Ctrl Pts',(33.8741638666671,-54.8812331832842,16.3341367170413));
#45917=CARTESIAN_POINT('Ctrl Pts',(34.430241618609,-56.6812314532133,16.2229988264732));
#45918=CARTESIAN_POINT('Ctrl Pts',(33.2195473266021,-58.1246425413596,16.1118609359052));
#45919=CARTESIAN_POINT('Ctrl Pts',(31.3502432063489,-57.8902959092575,16.0007230453371));
#45920=CARTESIAN_POINT('Ctrl Pts',(30.5333245184248,-56.1926916871221,15.8895851547691));
#45921=CARTESIAN_POINT('Ctrl Pts',(31.5165262024604,-54.5856662712539,15.778447264201));
#45922=CARTESIAN_POINT('Ctrl Pts',(33.3999126066214,-54.5401482504283,15.667309373633));
#45923=CARTESIAN_POINT('Ctrl Pts',(34.4595987964668,-56.0978007838682,15.556171483065));
#45924=CARTESIAN_POINT('Ctrl Pts',(33.7256419840878,-57.8328868456334,15.4450335924969));
#45925=CARTESIAN_POINT('Ctrl Pts',(31.8698411648613,-58.1572624803752,15.3338957019289));
#45926=CARTESIAN_POINT('Ctrl Pts',(30.5908318720959,-56.7740230025534,15.2227578113608));
#45927=CARTESIAN_POINT('Ctrl Pts',(31.0593058218999,-54.9492631699882,15.1116199207928));
#45928=CARTESIAN_POINT('Ctrl Pts',(32.846463484178,-54.3532063981059,15.0004820302248));
#45929=CARTESIAN_POINT('Ctrl Pts',(34.3164992048823,-55.5314301169031,14.8893441396567));
#45930=CARTESIAN_POINT('Ctrl Pts',(34.1238725735219,-57.4054929808208,14.7782062490887));
#45931=CARTESIAN_POINT('Ctrl Pts',(32.4448970183546,-58.2600436245124,14.6670683585206));
#45932=CARTESIAN_POINT('Ctrl Pts',(30.8163577297114,-57.3129028983934,14.5559304679526));
#45933=CARTESIAN_POINT('Ctrl Pts',(30.7288755399893,-55.4309979577249,14.4447925773845));
#45934=CARTESIAN_POINT('Ctrl Pts',(32.2625231838811,-54.3368607242037,14.3336546868165));
#45935=CARTESIAN_POINT('Ctrl Pts',(34.0135369924464,-55.0319614376805,14.2225167962484));
#45936=CARTESIAN_POINT('Ctrl Pts',(34.3791913425147,-56.8800784965451,14.1113789056804));
#45937=CARTESIAN_POINT('Ctrl Pts',(33.0248043169983,-58.1895854534881,14.0002410151124));
#45938=CARTESIAN_POINT('Ctrl Pts',(31.1900504001867,-57.7619236593993,13.8891031245443));
#45939=CARTESIAN_POINT('Ctrl Pts',(30.5543233141752,-55.9884409037984,13.7779652339763));
#45940=CARTESIAN_POINT('Ctrl Pts',(31.69946593225,-54.4926179908013,13.6668273434083));
#45941=CARTESIAN_POINT('Ctrl Pts',(33.5774069631984,-54.6432144942032,13.5556894528402));
#45942=CARTESIAN_POINT('Ctrl Pts',(34.4690641115077,-56.3031564828284,13.4445515622722));
#45943=CARTESIAN_POINT('Ctrl Pts',(33.5586566967914,-57.9515409790141,13.3334136717041));
#45944=CARTESIAN_POINT('Ctrl Pts',(31.6787663486304,-58.0826736409194,13.2222757811361));
#45945=CARTESIAN_POINT('Ctrl Pts',(30.5515057669383,-56.5702175776209,13.111137890568));
#45946=CARTESIAN_POINT('Ctrl Pts',(30.9881746982542,-55.3989927257807,13.0370459635227));
#45947=CARTESIAN_POINT('Ctrl Pts',(31.4059736530044,-55.03520293743,13.));
#45948=CARTESIAN_POINT('Ctrl Pts',(31.6688940285232,-54.8502492137287,21.3785196366098));
#45949=CARTESIAN_POINT('Ctrl Pts',(31.8552973625104,-54.7413392620857,21.3641270219409));
#45950=CARTESIAN_POINT('Ctrl Pts',(32.061419630626,-54.6673572529873,21.349734407272));
#45951=CARTESIAN_POINT('Ctrl Pts',(32.2736902248207,-54.6382999126305,21.3353417926031));
#45952=CARTESIAN_POINT('Ctrl Pts',(32.8200654923025,-54.5635075836697,21.2982958290804));
#45953=CARTESIAN_POINT('Ctrl Pts',(33.4071749686057,-54.7863525000711,21.2612498655578));
#45954=CARTESIAN_POINT('Ctrl Pts',(33.7663304550473,-55.2048330504423,21.2242039020351));
#45955=CARTESIAN_POINT('Ctrl Pts',(34.1254859414888,-55.6233136008135,21.1871579385124));
#45956=CARTESIAN_POINT('Ctrl Pts',(34.2566874380687,-56.2374297851546,21.1501119749897));
#45957=CARTESIAN_POINT('Ctrl Pts',(34.0998869466366,-56.7661355303639,21.113066011467));
#45958=CARTESIAN_POINT('Ctrl Pts',(33.9430864552045,-57.2948412755732,21.0760200479444));
#45959=CARTESIAN_POINT('Ctrl Pts',(33.4982839757605,-57.7381365816507,21.0389740844217));
#45960=CARTESIAN_POINT('Ctrl Pts',(32.9690473289312,-57.8931410001211,21.001928120899));
#45961=CARTESIAN_POINT('Ctrl Pts',(32.4398106821019,-58.0481454185914,20.9648821573763));
#45962=CARTESIAN_POINT('Ctrl Pts',(31.8261398678875,-57.9148589494545,20.9278361938536));
#45963=CARTESIAN_POINT('Ctrl Pts',(31.4088840927747,-57.5542828188567,20.8907902303309));
#45964=CARTESIAN_POINT('Ctrl Pts',(30.9916283176618,-57.1937066882589,20.8537442668083));
#45965=CARTESIAN_POINT('Ctrl Pts',(30.7707875816507,-56.6058408962002,20.8166983032856));
#45966=CARTESIAN_POINT('Ctrl Pts',(30.8474312602907,-56.0597245975799,20.7796523397629));
#45967=CARTESIAN_POINT('Ctrl Pts',(30.9171750925773,-55.5627724129275,20.7459414387119));
#45968=CARTESIAN_POINT('Ctrl Pts',(31.2332522390469,-55.1003910850247,20.7122305376608));
#45969=CARTESIAN_POINT('Ctrl Pts',(31.6666453776089,-54.8465106722,20.6785196366098));
#45970=CARTESIAN_POINT('Ctrl Pts',(30.5157034944333,-56.8250975324092,22.));
#45971=CARTESIAN_POINT('Ctrl Pts',(30.5033891751539,-56.7529213758001,22.));
#45972=CARTESIAN_POINT('Ctrl Pts',(30.495295269616,-56.6802754208446,22.));
#45973=CARTESIAN_POINT('Ctrl Pts',(30.4912615438002,-56.6074703113041,22.));
#45974=CARTESIAN_POINT('Ctrl Pts',(30.4871154839524,-56.5326376738967,22.));
#45975=CARTESIAN_POINT('Ctrl Pts',(30.487259104724,-56.4576358814856,22.));
#45976=CARTESIAN_POINT('Ctrl Pts',(30.4915726828733,-56.3828069694724,22.));
#45977=CARTESIAN_POINT('Ctrl Pts',(30.4952175802639,-56.3195778597416,22.));
#45978=CARTESIAN_POINT('Ctrl Pts',(30.5018408843277,-56.2564719495625,22.));
#45979=CARTESIAN_POINT('Ctrl Pts',(30.5113973391132,-56.193706282076,22.));
#45980=CARTESIAN_POINT('Ctrl Pts',(30.5156431766695,-56.1658201219636,22.));
#45981=CARTESIAN_POINT('Ctrl Pts',(30.5204683060505,-56.1380012967322,22.));
#45982=CARTESIAN_POINT('Ctrl Pts',(30.5258701615124,-56.1102698241508,22.));
#45983=CARTESIAN_POINT('Ctrl Pts',(30.5288380312312,-56.0950336893986,22.));
#45984=CARTESIAN_POINT('Ctrl Pts',(30.5319800053068,-56.0798239348075,22.));
#45985=CARTESIAN_POINT('Ctrl Pts',(30.5352957613587,-56.0646439756266,22.));
#45986=CARTESIAN_POINT('Ctrl Pts',(30.5383537435175,-56.0506441386005,22.));
#45987=CARTESIAN_POINT('Ctrl Pts',(30.5415601340457,-56.0366676410971,22.));
#45988=CARTESIAN_POINT('Ctrl Pts',(30.5449092364487,-56.0227386583732,22.));
#45989=CARTESIAN_POINT('Ctrl Pts',(30.5620232882029,-55.9515609807346,22.));
#45990=CARTESIAN_POINT('Ctrl Pts',(30.5828856177102,-55.8814985818636,22.));
#45991=CARTESIAN_POINT('Ctrl Pts',(30.6073807784331,-55.8128705897493,22.));
#45992=CARTESIAN_POINT('Ctrl Pts',(30.631685982855,-55.7447747974306,22.));
#45993=CARTESIAN_POINT('Ctrl Pts',(30.6595684038277,-55.6780903688633,22.));
#45994=CARTESIAN_POINT('Ctrl Pts',(30.690958647943,-55.6131557366251,22.));
#45995=CARTESIAN_POINT('Ctrl Pts',(30.7170465723104,-55.5591896136339,22.));
#45996=CARTESIAN_POINT('Ctrl Pts',(30.7455582375761,-55.5064323069427,22.));
#45997=CARTESIAN_POINT('Ctrl Pts',(30.7764732244728,-55.4550987628706,22.));
#45998=CARTESIAN_POINT('Ctrl Pts',(30.7893770627374,-55.4336722698731,22.));
#45999=CARTESIAN_POINT('Ctrl Pts',(30.8026998040103,-55.4124940848672,22.));
#46000=CARTESIAN_POINT('Ctrl Pts',(30.816440755509,-55.3915810450006,22.));
#46001=CARTESIAN_POINT('Ctrl Pts',(30.8228008343777,-55.3819013235527,22.));
#46002=CARTESIAN_POINT('Ctrl Pts',(30.8292505148729,-55.3722784163625,22.));
#46003=CARTESIAN_POINT('Ctrl Pts',(30.8357897592244,-55.36271405055,22.));
#46004=CARTESIAN_POINT('Ctrl Pts',(30.8426105864645,-55.3527378387185,22.));
#46005=CARTESIAN_POINT('Ctrl Pts',(30.8495241989438,-55.3428321824372,22.));
#46006=CARTESIAN_POINT('Ctrl Pts',(30.8565275508842,-55.3330023511027,22.));
#46007=CARTESIAN_POINT('Ctrl Pts',(30.8964137687876,-55.2770184739693,22.));
#46008=CARTESIAN_POINT('Ctrl Pts',(30.9392347488792,-55.2234520245275,22.));
#46009=CARTESIAN_POINT('Ctrl Pts',(30.9849250921271,-55.1725987747119,22.));
#46010=CARTESIAN_POINT('Ctrl Pts',(31.0263368675565,-55.1265075613062,22.));
#46011=CARTESIAN_POINT('Ctrl Pts',(31.0701064557712,-55.0826451744781,22.));
#46012=CARTESIAN_POINT('Ctrl Pts',(31.1162077188352,-55.0412612463575,22.));
#46013=CARTESIAN_POINT('Ctrl Pts',(31.1707480896715,-54.9923017464143,22.));
#46014=CARTESIAN_POINT('Ctrl Pts',(31.2285529377194,-54.9468098709298,22.));
#46015=CARTESIAN_POINT('Ctrl Pts',(31.2892182914167,-54.9049320829474,22.));
#46016=CARTESIAN_POINT('Ctrl Pts',(31.3025747483257,-54.8957120119094,22.));
#46017=CARTESIAN_POINT('Ctrl Pts',(31.3160699039855,-54.8866673619302,22.));
#46018=CARTESIAN_POINT('Ctrl Pts',(31.3296994894169,-54.8778000986123,22.));
#46019=CARTESIAN_POINT('Ctrl Pts',(31.3437625465108,-54.8686508232411,22.));
#46020=CARTESIAN_POINT('Ctrl Pts',(31.3579740386175,-54.8596873154203,22.));
#46021=CARTESIAN_POINT('Ctrl Pts',(31.372300027318,-54.8509292655156,22.));
#46022=CARTESIAN_POINT('Ctrl Pts',(31.4308133755382,-54.8151577153271,22.));
#46023=CARTESIAN_POINT('Ctrl Pts',(31.4913062997832,-54.7827600287193,22.));
#46024=CARTESIAN_POINT('Ctrl Pts',(31.5534255550514,-54.7538008858643,22.));
#46025=CARTESIAN_POINT('Ctrl Pts',(31.6155323755402,-54.7248475399326,22.));
#46026=CARTESIAN_POINT('Ctrl Pts',(31.6792660307646,-54.6993312184063,22.));
#46027=CARTESIAN_POINT('Ctrl Pts',(31.7442852729951,-54.6773670392688,22.));
#46028=CARTESIAN_POINT('Ctrl Pts',(31.7913479559042,-54.6614687734225,22.));
#46029=CARTESIAN_POINT('Ctrl Pts',(31.8390844861912,-54.6474326076125,22.));
#46030=CARTESIAN_POINT('Ctrl Pts',(31.8873641954598,-54.6353193456966,22.));
#46031=CARTESIAN_POINT('Ctrl Pts',(31.9235796701969,-54.6262329709536,22.));
#46032=CARTESIAN_POINT('Ctrl Pts',(31.960100769596,-54.6182288635217,22.));
#46033=CARTESIAN_POINT('Ctrl Pts',(31.9968706812112,-54.6113381701337,22.));
#46034=CARTESIAN_POINT('Ctrl Pts',(32.0090868551873,-54.6090488551599,22.));
#46035=CARTESIAN_POINT('Ctrl Pts',(32.0213209007479,-54.6068842729393,22.));
#46036=CARTESIAN_POINT('Ctrl Pts',(32.033570365114,-54.6048451279827,22.));
#46037=CARTESIAN_POINT('Ctrl Pts',(32.0985567096685,-54.5940269752226,22.));
#46038=CARTESIAN_POINT('Ctrl Pts',(32.1639811762245,-54.5867347457051,22.));
#46039=CARTESIAN_POINT('Ctrl Pts',(32.2295294708195,-54.5830921510723,22.));
#46040=CARTESIAN_POINT('Ctrl Pts',(32.275653061784,-54.5805290097133,22.));
#46041=CARTESIAN_POINT('Ctrl Pts',(32.3218379338893,-54.5797739344474,22.));
#46042=CARTESIAN_POINT('Ctrl Pts',(32.3679699515865,-54.5808847307989,22.));
#46043=CARTESIAN_POINT('Ctrl Pts',(32.3827771688226,-54.5812412684858,22.));
#46044=CARTESIAN_POINT('Ctrl Pts',(32.397580934837,-54.5817902377274,22.));
#46045=CARTESIAN_POINT('Ctrl Pts',(32.4123708490296,-54.5825334834844,22.));
#46046=CARTESIAN_POINT('Ctrl Pts',(32.4753792588787,-54.5856998800343,22.));
#46047=CARTESIAN_POINT('Ctrl Pts',(32.5380109270838,-54.5923812630408,22.));
#46048=CARTESIAN_POINT('Ctrl Pts',(32.5999757761394,-54.6027055704867,22.));
#46049=CARTESIAN_POINT('Ctrl Pts',(32.6570986727354,-54.6122231333574,22.));
#46050=CARTESIAN_POINT('Ctrl Pts',(32.7136552658997,-54.6248370045754,22.));
#46051=CARTESIAN_POINT('Ctrl Pts',(32.7694005056338,-54.6406824777883,22.));
#46052=CARTESIAN_POINT('Ctrl Pts',(32.7798334333405,-54.6436480166809,22.));
#46053=CARTESIAN_POINT('Ctrl Pts',(32.7902378797118,-54.6467268441195,22.));
#46054=CARTESIAN_POINT('Ctrl Pts',(32.8006124898339,-54.6499179279035,22.));
#46055=CARTESIAN_POINT('Origin',(32.5,-56.2916512459885,17.));
#46056=CARTESIAN_POINT('Origin',(-32.5,-56.2916512459885,13.));
#46057=CARTESIAN_POINT('Ctrl Pts',(-31.9588970197441,-54.7159724828016,
13.));
#46058=CARTESIAN_POINT('Ctrl Pts',(-32.0152863485872,-54.6890038458254,
13.));
#46059=CARTESIAN_POINT('Ctrl Pts',(-32.0731449906992,-54.665548635413,13.));
#46060=CARTESIAN_POINT('Ctrl Pts',(-32.1321548892164,-54.6454940895841,
13.));
#46061=CARTESIAN_POINT('Ctrl Pts',(-32.1695849278231,-54.6327734707815,
13.));
#46062=CARTESIAN_POINT('Ctrl Pts',(-32.2074789472177,-54.6214218412685,
13.));
#46063=CARTESIAN_POINT('Ctrl Pts',(-32.2457622248769,-54.611418695037,13.));
#46064=CARTESIAN_POINT('Ctrl Pts',(-32.271904889536,-54.6045878040198,13.));
#46065=CARTESIAN_POINT('Ctrl Pts',(-32.2982291715498,-54.5983858677327,
13.));
#46066=CARTESIAN_POINT('Ctrl Pts',(-32.3247122748156,-54.592808119745,13.));
#46067=CARTESIAN_POINT('Ctrl Pts',(-32.338774499773,-54.5898463993541,13.));
#46068=CARTESIAN_POINT('Ctrl Pts',(-32.3528813607046,-54.5870608474282,
13.));
#46069=CARTESIAN_POINT('Ctrl Pts',(-32.367015346482,-54.5844531526057,13.));
#46070=CARTESIAN_POINT('Ctrl Pts',(-32.4318895175076,-54.5724839853404,
13.));
#46071=CARTESIAN_POINT('Ctrl Pts',(-32.4974065824013,-54.5642420059679,
13.));
#46072=CARTESIAN_POINT('Ctrl Pts',(-32.5632274845374,-54.5596289936312,
13.));
#46073=CARTESIAN_POINT('Ctrl Pts',(-32.6107070729831,-54.5563014195608,
13.));
#46074=CARTESIAN_POINT('Ctrl Pts',(-32.6583455261738,-54.5548630893332,
13.));
#46075=CARTESIAN_POINT('Ctrl Pts',(-32.7060224989242,-54.5552923689863,
13.));
#46076=CARTESIAN_POINT('Ctrl Pts',(-32.7190852595527,-54.5554099850392,
13.));
#46077=CARTESIAN_POINT('Ctrl Pts',(-32.7321509341772,-54.5556678729876,
13.));
#46078=CARTESIAN_POINT('Ctrl Pts',(-32.7452170898975,-54.5560657582162,
13.));
#46079=CARTESIAN_POINT('Ctrl Pts',(-32.7585822800833,-54.55647274952,13.));
#46080=CARTESIAN_POINT('Ctrl Pts',(-32.7719398800736,-54.5570260108604,
13.));
#46081=CARTESIAN_POINT('Ctrl Pts',(-32.7852820457025,-54.5577244070661,
13.));
#46082=CARTESIAN_POINT('Ctrl Pts',(-32.8530416061927,-54.5612712840324,
13.));
#46083=CARTESIAN_POINT('Ctrl Pts',(-32.9204432866946,-54.5685589036366,
13.));
#46084=CARTESIAN_POINT('Ctrl Pts',(-32.9871435059666,-54.5794869270338,
13.));
#46085=CARTESIAN_POINT('Ctrl Pts',(-33.0548103387428,-54.590573318351,13.));
#46086=CARTESIAN_POINT('Ctrl Pts',(-33.1217562803605,-54.6054062113849,
13.));
#46087=CARTESIAN_POINT('Ctrl Pts',(-33.1876366472556,-54.6239318016751,
13.));
#46088=CARTESIAN_POINT('Ctrl Pts',(-33.2284548201806,-54.6354098911825,
13.));
#46089=CARTESIAN_POINT('Ctrl Pts',(-33.2688641593019,-54.6483065466031,
13.));
#46090=CARTESIAN_POINT('Ctrl Pts',(-33.308782562507,-54.6626190129889,13.));
#46091=CARTESIAN_POINT('Ctrl Pts',(-33.3414809096879,-54.6743427784034,
13.));
#46092=CARTESIAN_POINT('Ctrl Pts',(-33.3738498713991,-54.6870166552392,
13.));
#46093=CARTESIAN_POINT('Ctrl Pts',(-33.4058433879587,-54.7006430225369,
13.));
#46094=CARTESIAN_POINT('Ctrl Pts',(-33.4189228881451,-54.7062137160015,
13.));
#46095=CARTESIAN_POINT('Ctrl Pts',(-33.431941905508,-54.7119448243305,13.));
#46096=CARTESIAN_POINT('Ctrl Pts',(-33.4448753977064,-54.7178263149142,
13.));
#46097=CARTESIAN_POINT('Ctrl Pts',(-33.5090388470795,-54.7470045691335,
13.));
#46098=CARTESIAN_POINT('Ctrl Pts',(-33.5712122519748,-54.7799269958261,
13.));
#46099=CARTESIAN_POINT('Ctrl Pts',(-33.6310396924137,-54.8165209633119,
13.));
#46100=CARTESIAN_POINT('Ctrl Pts',(-33.6376901817643,-54.8205887922091,
13.));
#46101=CARTESIAN_POINT('Ctrl Pts',(-33.6443116825685,-54.8247020426567,
13.));
#46102=CARTESIAN_POINT('Ctrl Pts',(-33.6509037041524,-54.8288606547026,
13.));
#46103=CARTESIAN_POINT('Ctrl Pts',(-33.7079313851615,-54.8648368720402,
13.));
#46104=CARTESIAN_POINT('Ctrl Pts',(-33.7627542963063,-54.9042038022182,
13.));
#46105=CARTESIAN_POINT('Ctrl Pts',(-33.8152783515972,-54.9466335926766,
13.));
#46106=CARTESIAN_POINT('Ctrl Pts',(-33.8717836154426,-54.9922794684851,
13.));
#46107=CARTESIAN_POINT('Ctrl Pts',(-33.9256293125932,-55.0414702768411,
13.));
#46108=CARTESIAN_POINT('Ctrl Pts',(-33.9766695218193,-55.0938552564662,
13.));
#46109=CARTESIAN_POINT('Ctrl Pts',(-33.98601646824,-55.1034484694492,13.));
#46110=CARTESIAN_POINT('Ctrl Pts',(-33.9952692317474,-55.113148942497,13.));
#46111=CARTESIAN_POINT('Ctrl Pts',(-34.0044267781796,-55.1229547001842,
13.));
#46112=CARTESIAN_POINT('Ctrl Pts',(-34.0122933714936,-55.1313781254359,
13.));
#46113=CARTESIAN_POINT('Ctrl Pts',(-34.0200833036472,-55.1398724074257,
13.));
#46114=CARTESIAN_POINT('Ctrl Pts',(-34.0277952351974,-55.1484347977441,
13.));
#46115=CARTESIAN_POINT('Ctrl Pts',(-34.0753570091897,-55.2012416037311,
13.));
#46116=CARTESIAN_POINT('Ctrl Pts',(-34.1199659341815,-55.2566479177152,
13.));
#46117=CARTESIAN_POINT('Ctrl Pts',(-34.1615258634594,-55.3142853318227,
13.));
#46118=CARTESIAN_POINT('Ctrl Pts',(-34.2039616811858,-55.373137472377,13.));
#46119=CARTESIAN_POINT('Ctrl Pts',(-34.2432193073455,-55.4343163954304,
13.));
#46120=CARTESIAN_POINT('Ctrl Pts',(-34.2791687520186,-55.497477603779,13.));
#46121=CARTESIAN_POINT('Ctrl Pts',(-34.3153358231374,-55.5610211698915,
13.));
#46122=CARTESIAN_POINT('Ctrl Pts',(-34.3481552082325,-55.6265719323703,
13.));
#46123=CARTESIAN_POINT('Ctrl Pts',(-34.3774567489235,-55.6938154067926,
13.));
#46124=CARTESIAN_POINT('Ctrl Pts',(-34.3846992416887,-55.7104360473981,
13.));
#46125=CARTESIAN_POINT('Ctrl Pts',(-34.3917266096161,-55.7271602398318,
13.));
#46126=CARTESIAN_POINT('Ctrl Pts',(-34.3985358555028,-55.743983480801,13.));
#46127=CARTESIAN_POINT('Ctrl Pts',(-34.4038603586072,-55.7571384468955,
13.));
#46128=CARTESIAN_POINT('Ctrl Pts',(-34.4090519561989,-55.7703555308113,
13.));
#46129=CARTESIAN_POINT('Ctrl Pts',(-34.414101784082,-55.7836123414303,13.));
#46130=CARTESIAN_POINT('Ctrl Pts',(-34.4409205169415,-55.8540168919997,
13.));
#46131=CARTESIAN_POINT('Ctrl Pts',(-34.4637958507435,-55.9256644802089,
13.));
#46132=CARTESIAN_POINT('Ctrl Pts',(-34.4826007268578,-55.9981857626967,
13.));
#46133=CARTESIAN_POINT('Ctrl Pts',(-34.5014259919704,-56.0707856756575,
13.));
#46134=CARTESIAN_POINT('Ctrl Pts',(-34.5161726005963,-56.1442621124532,
13.));
#46135=CARTESIAN_POINT('Ctrl Pts',(-34.5266721187049,-56.2182764860945,
13.));
#46136=CARTESIAN_POINT('Ctrl Pts',(-34.5369326970758,-56.290606499097,13.));
#46137=CARTESIAN_POINT('Ctrl Pts',(-34.5431377092968,-56.3634511940737,
13.));
#46138=CARTESIAN_POINT('Ctrl Pts',(-34.5450833843548,-56.4365110273052,
13.));
#46139=CARTESIAN_POINT('Ctrl Pts',(-34.5455017158062,-56.4522193162868,
13.));
#46140=CARTESIAN_POINT('Ctrl Pts',(-34.5457229607324,-56.4679375826136,
13.));
#46141=CARTESIAN_POINT('Ctrl Pts',(-34.5457447745363,-56.4836628867631,
13.));
#46142=CARTESIAN_POINT('Ctrl Pts',(-34.545763248735,-56.4969807103663,13.));
#46143=CARTESIAN_POINT('Ctrl Pts',(-34.5456386792458,-56.5103035820178,
13.));
#46144=CARTESIAN_POINT('Ctrl Pts',(-34.5453721234944,-56.52362996598,13.));
#46145=CARTESIAN_POINT('Ctrl Pts',(-34.1542537360139,-57.5104384051693,
13.));
#46146=CARTESIAN_POINT('Ctrl Pts',(-34.1045519887786,-57.5661317580893,
13.));
#46147=CARTESIAN_POINT('Ctrl Pts',(-34.0516736631806,-57.6187667033008,
13.));
#46148=CARTESIAN_POINT('Ctrl Pts',(-33.9959663128535,-57.6682442041301,
13.));
#46149=CARTESIAN_POINT('Ctrl Pts',(-33.941716853086,-57.7164268528268,13.));
#46150=CARTESIAN_POINT('Ctrl Pts',(-33.8847834892553,-57.7616152151019,
13.));
#46151=CARTESIAN_POINT('Ctrl Pts',(-33.8254670336322,-57.8036766866724,
13.));
#46152=CARTESIAN_POINT('Ctrl Pts',(-33.812228067015,-57.8130644764879,13.));
#46153=CARTESIAN_POINT('Ctrl Pts',(-33.7988685442659,-57.8222975378101,
13.));
#46154=CARTESIAN_POINT('Ctrl Pts',(-33.7853974828999,-57.8313702493365,
13.));
#46155=CARTESIAN_POINT('Ctrl Pts',(-33.7235792093242,-57.8730046349261,
13.));
#46156=CARTESIAN_POINT('Ctrl Pts',(-33.6595370838482,-57.9111844301544,
13.));
#46157=CARTESIAN_POINT('Ctrl Pts',(-33.5936094995078,-57.945786238912,13.));
#46158=CARTESIAN_POINT('Ctrl Pts',(-33.547323850303,-57.9700790625916,13.));
#46159=CARTESIAN_POINT('Ctrl Pts',(-33.5001083176739,-57.9926073121725,
13.));
#46160=CARTESIAN_POINT('Ctrl Pts',(-33.4520768824606,-58.0133132483315,
13.));
#46161=CARTESIAN_POINT('Ctrl Pts',(-33.4338169279728,-58.0211849567285,
13.));
#46162=CARTESIAN_POINT('Ctrl Pts',(-33.4154390448092,-58.0287931600018,
13.));
#46163=CARTESIAN_POINT('Ctrl Pts',(-33.3969494936981,-58.0361341920447,
13.));
#46164=CARTESIAN_POINT('Ctrl Pts',(-33.3793383498013,-58.043126464106,13.));
#46165=CARTESIAN_POINT('Ctrl Pts',(-33.3616202465966,-58.0498782554867,
13.));
#46166=CARTESIAN_POINT('Ctrl Pts',(-33.3438321785184,-58.0563750965513,
13.));
#46167=CARTESIAN_POINT('Ctrl Pts',(-33.2756398803729,-58.0812813719788,
13.));
#46168=CARTESIAN_POINT('Ctrl Pts',(-33.2063496369042,-58.1024753902403,
13.));
#46169=CARTESIAN_POINT('Ctrl Pts',(-33.1362740502616,-58.1198408416066,
13.));
#46170=CARTESIAN_POINT('Ctrl Pts',(-33.0677030440348,-58.1368334424655,
13.));
#46171=CARTESIAN_POINT('Ctrl Pts',(-32.9983791192747,-58.1501601307445,
13.));
#46172=CARTESIAN_POINT('Ctrl Pts',(-32.9285938585171,-58.1596629268823,
13.));
#46173=CARTESIAN_POINT('Ctrl Pts',(-32.860339265238,-58.1689572890207,13.));
#46174=CARTESIAN_POINT('Ctrl Pts',(-32.791642581852,-58.1745936618092,13.));
#46175=CARTESIAN_POINT('Ctrl Pts',(-32.7227877559508,-58.1763767799569,
13.));
#46176=CARTESIAN_POINT('Ctrl Pts',(-32.7004157901354,-58.1769561417914,
13.));
#46177=CARTESIAN_POINT('Ctrl Pts',(-32.6780272661539,-58.1771283364151,
13.));
#46178=CARTESIAN_POINT('Ctrl Pts',(-32.6556323878678,-58.1768855536499,
13.));
#46179=CARTESIAN_POINT('Ctrl Pts',(-32.642997056445,-58.1767485740841,13.));
#46180=CARTESIAN_POINT('Ctrl Pts',(-32.6303583965514,-58.1764793454886,
13.));
#46181=CARTESIAN_POINT('Ctrl Pts',(-32.617736131084,-58.1760772493482,13.));
#46182=CARTESIAN_POINT('Ctrl Pts',(-32.5494663667858,-58.1739024409672,
13.));
#46183=CARTESIAN_POINT('Ctrl Pts',(-32.4815560597098,-58.1678447149676,
13.));
#46184=CARTESIAN_POINT('Ctrl Pts',(-32.4142747868267,-58.1577646785827,
13.));
#46185=CARTESIAN_POINT('Ctrl Pts',(-32.4045647306857,-58.15630992431,13.));
#46186=CARTESIAN_POINT('Ctrl Pts',(-32.3948677956577,-58.1547713053032,
13.));
#46187=CARTESIAN_POINT('Ctrl Pts',(-32.3851848149705,-58.1531483143848,
13.));
#46188=CARTESIAN_POINT('Ctrl Pts',(-32.3167654615685,-58.1416803591339,
13.));
#46189=CARTESIAN_POINT('Ctrl Pts',(-32.2490407707029,-58.1260036975298,
13.));
#46190=CARTESIAN_POINT('Ctrl Pts',(-32.1823062478791,-58.1063380404035,
13.));
#46191=CARTESIAN_POINT('Ctrl Pts',(-32.1200483333854,-58.0879915722183,
13.));
#46192=CARTESIAN_POINT('Ctrl Pts',(-32.0586518297846,-58.0661723398752,
13.));
#46193=CARTESIAN_POINT('Ctrl Pts',(-31.9983820977313,-58.0410277367995,
13.));
#46194=CARTESIAN_POINT('Ctrl Pts',(-31.9850796184709,-58.0354779268115,
13.));
#46195=CARTESIAN_POINT('Ctrl Pts',(-31.9718321460664,-58.0297660234503,
13.));
#46196=CARTESIAN_POINT('Ctrl Pts',(-31.9586427416388,-58.023893457908,13.));
#46197=CARTESIAN_POINT('Ctrl Pts',(-31.9483333677394,-58.0193032222945,
13.));
#46198=CARTESIAN_POINT('Ctrl Pts',(-31.9380601507492,-58.0146150416842,
13.));
#46199=CARTESIAN_POINT('Ctrl Pts',(-31.9278362672604,-58.0098353467978,
13.));
#46200=CARTESIAN_POINT('Ctrl Pts',(-31.8658980543593,-57.9808790544257,
13.));
#46201=CARTESIAN_POINT('Ctrl Pts',(-31.8056527017084,-57.9485169556613,
13.));
#46202=CARTESIAN_POINT('Ctrl Pts',(-31.7473720765467,-57.9129741302491,
13.));
#46203=CARTESIAN_POINT('Ctrl Pts',(-31.6893603668348,-57.8775953047057,
13.));
#46204=CARTESIAN_POINT('Ctrl Pts',(-31.6332945176634,-57.8390642101102,
13.));
#46205=CARTESIAN_POINT('Ctrl Pts',(-31.5794782982672,-57.7975661709256,
13.));
#46206=CARTESIAN_POINT('Ctrl Pts',(-31.5268144521557,-57.7569567343271,
13.));
#46207=CARTESIAN_POINT('Ctrl Pts',(-31.4763043639082,-57.7135052609396,
13.));
#46208=CARTESIAN_POINT('Ctrl Pts',(-31.4282765730784,-57.6673622963473,
13.));
#46209=CARTESIAN_POINT('Ctrl Pts',(-31.4181553628237,-57.6576382878443,
13.));
#46210=CARTESIAN_POINT('Ctrl Pts',(-31.4081445660852,-57.647794690832,13.));
#46211=CARTESIAN_POINT('Ctrl Pts',(-31.3982475487379,-57.6378328293302,
13.));
#46212=CARTESIAN_POINT('Ctrl Pts',(-31.3888700148449,-57.6283938548803,
13.));
#46213=CARTESIAN_POINT('Ctrl Pts',(-31.3795934917281,-57.6188473329616,
13.));
#46214=CARTESIAN_POINT('Ctrl Pts',(-31.370435450571,-57.6092101707806,13.));
#46215=CARTESIAN_POINT('Ctrl Pts',(-31.3254237977993,-57.5618436444295,
13.));
#46216=CARTESIAN_POINT('Ctrl Pts',(-31.28318780428,-57.5122078770326,13.));
#46217=CARTESIAN_POINT('Ctrl Pts',(-31.2439955573278,-57.4604767979467,
13.));
#46218=CARTESIAN_POINT('Ctrl Pts',(-31.2055484075955,-57.4097291961098,
13.));
#46219=CARTESIAN_POINT('Ctrl Pts',(-31.1700298958942,-57.3569644529347,
13.));
#46220=CARTESIAN_POINT('Ctrl Pts',(-31.1377389873445,-57.3023276234082,
13.));
#46221=CARTESIAN_POINT('Ctrl Pts',(-31.1064966595925,-57.2494650124732,
13.));
#46222=CARTESIAN_POINT('Ctrl Pts',(-31.0782754671115,-57.1948493080738,
13.));
#46223=CARTESIAN_POINT('Ctrl Pts',(-31.0533946162939,-57.1386036481878,
13.));
#46224=CARTESIAN_POINT('Ctrl Pts',(-31.049253985217,-57.129243336156,13.));
#46225=CARTESIAN_POINT('Ctrl Pts',(-31.045205981978,-57.1198378750668,13.));
#46226=CARTESIAN_POINT('Ctrl Pts',(-31.0412522209115,-57.1103878272416,
13.));
#46227=CARTESIAN_POINT('Ctrl Pts',(-31.0370666269761,-57.1003836660893,
13.));
#46228=CARTESIAN_POINT('Ctrl Pts',(-31.032986652061,-57.0903295352429,13.));
#46229=CARTESIAN_POINT('Ctrl Pts',(-31.0290124456509,-57.0802271145803,
13.));
#46230=CARTESIAN_POINT('Origin',(-32.5,-56.2916512459885,23.5459252805377));
#46231=CARTESIAN_POINT('Ctrl Pts',(-31.4704151231923,-54.5113563798656,
21.7959252805377));
#46232=CARTESIAN_POINT('Ctrl Pts',(-31.3848836142506,-54.5597932517276,
21.7905813053169));
#46233=CARTESIAN_POINT('Ctrl Pts',(-30.7359364258277,-54.993465396867,21.7481913665734));
#46234=CARTESIAN_POINT('Ctrl Pts',(-30.0819661342964,-56.5203533893187,
21.6687554643073));
#46235=CARTESIAN_POINT('Ctrl Pts',(-31.380844296031,-58.4469950837991,21.5576175737392));
#46236=CARTESIAN_POINT('Ctrl Pts',(-33.7038051725687,-58.4009643313194,
21.4464796831712));
#46237=CARTESIAN_POINT('Ctrl Pts',(-34.9250559921582,-56.4241863460987,
21.3353417926031));
#46238=CARTESIAN_POINT('Ctrl Pts',(-33.9265523881077,-54.3261319732661,
21.2242039020351));
#46239=CARTESIAN_POINT('Ctrl Pts',(-32.2719558287363,-54.111420270443,21.1443983980133));
#46240=CARTESIAN_POINT('Ctrl Pts',(-31.5637955304719,-54.4566153915593,
21.1016388575141));
#46241=CARTESIAN_POINT('Ctrl Pts',(-31.4731950477465,-54.5099653993635,
21.0959252805377));
#46242=CARTESIAN_POINT('Ctrl Pts',(-31.4756555660462,-54.5128362942924,
21.8540747194623));
#46243=CARTESIAN_POINT('Ctrl Pts',(-31.0702251268552,-54.7510086370429,
21.8286245525962));
#46244=CARTESIAN_POINT('Ctrl Pts',(-30.2605073082537,-55.6718001447715,
21.7661284222074));
#46245=CARTESIAN_POINT('Ctrl Pts',(-30.5464763025826,-57.7337498950934,
21.6665863282958));
#46246=CARTESIAN_POINT('Ctrl Pts',(-32.6512600365403,-58.7155097146097,
21.5554484377279));
#46247=CARTESIAN_POINT('Ctrl Pts',(-34.6188774786828,-57.4788960204646,
21.4443105471598));
#46248=CARTESIAN_POINT('Ctrl Pts',(-34.6464212862449,-55.1554778495401,
21.3331726565917));
#46249=CARTESIAN_POINT('Ctrl Pts',(-32.9604590994426,-54.0382699285555,
21.2364273806926));
#46250=CARTESIAN_POINT('Ctrl Pts',(-31.8369684898523,-54.3074066165865,
21.1767280683161));
#46251=CARTESIAN_POINT('Ctrl Pts',(-31.4729484072307,-54.5150696468519,
21.1540747194623));
#46252=CARTESIAN_POINT('Ctrl Pts',(-32.1997834265916,-57.9303781936679,
22.));
#46253=CARTESIAN_POINT('Ctrl Pts',(-32.7446991236385,-58.0302073467771,
21.9629540364773));
#46254=CARTESIAN_POINT('Ctrl Pts',(-33.932658940673,-57.64135965021,21.888862109432));
#46255=CARTESIAN_POINT('Ctrl Pts',(-34.4123083746051,-55.8170344416491,
21.7777242188639));
#46256=CARTESIAN_POINT('Ctrl Pts',(-33.1376927310287,-54.4290349886999,
21.6665863282959));
#46257=CARTESIAN_POINT('Ctrl Pts',(-31.2813034436656,-54.7450016890465,
21.5554484377278));
#46258=CARTESIAN_POINT('Ctrl Pts',(-30.5394479035103,-56.4770839121465,
21.4443105471598));
#46259=CARTESIAN_POINT('Ctrl Pts',(-31.592583816614,-58.0392131556089,21.3331726565918));
#46260=CARTESIAN_POINT('Ctrl Pts',(-33.4760503309402,-58.0018912265998,
21.2220347660237));
#46261=CARTESIAN_POINT('Ctrl Pts',(-34.4662456663514,-56.3991112663237,
21.1108968754557));
#46262=CARTESIAN_POINT('Ctrl Pts',(-33.6566547164314,-54.6979998974762,
20.9997589848876));
#46263=CARTESIAN_POINT('Ctrl Pts',(-31.7883942259045,-54.4555617097706,
20.8886210943196));
#46264=CARTESIAN_POINT('Ctrl Pts',(-30.5714597638967,-55.8937240769523,
20.7774832037515));
#46265=CARTESIAN_POINT('Ctrl Pts',(-31.1197474481278,-57.6961102078823,
20.6663453131835));
#46266=CARTESIAN_POINT('Ctrl Pts',(-32.9313922508809,-58.212980865287,20.5552074226155));
#46267=CARTESIAN_POINT('Ctrl Pts',(-34.3481806801685,-56.9712358625611,
20.4440695320474));
#46268=CARTESIAN_POINT('Ctrl Pts',(-34.0733074508499,-55.1074597880137,
20.3329316414794));
#46269=CARTESIAN_POINT('Ctrl Pts',(-32.3583685299806,-54.3275873674106,
20.2217937509113));
#46270=CARTESIAN_POINT('Ctrl Pts',(-30.7730662696612,-55.3454449973685,
20.1106558603433));
#46271=CARTESIAN_POINT('Ctrl Pts',(-30.7684461524675,-57.2293758831937,
19.9995179697752));
#46272=CARTESIAN_POINT('Ctrl Pts',(-32.3487368516327,-58.2549968011428,
19.8883800792072));
#46273=CARTESIAN_POINT('Ctrl Pts',(-34.0674804546367,-57.4835452530785,
19.7772421886392));
#46274=CARTESIAN_POINT('Ctrl Pts',(-34.3514914067379,-55.6211396100853,
19.6661042980711));
#46275=CARTESIAN_POINT('Ctrl Pts',(-32.9408112840734,-54.3724608681775,
19.5549664075031));
#46276=CARTESIAN_POINT('Ctrl Pts',(-31.1266515903786,-54.8804388458658,
19.443828516935));
#46277=CARTESIAN_POINT('Ctrl Pts',(-30.569533272628,-56.680115536781,19.332690626367));
#46278=CARTESIAN_POINT('Ctrl Pts',(-31.7793930425298,-58.1242264572701,
19.2215527357989));
#46279=CARTESIAN_POINT('Ctrl Pts',(-33.6488325332889,-57.8909605038464,
19.1104148452309));
#46280=CARTESIAN_POINT('Ctrl Pts',(-34.4667325774588,-56.1938286494099,
18.9992769546628));
#46281=CARTESIAN_POINT('Ctrl Pts',(-33.4844599893276,-54.5862349269529,
18.8881390640949));
#46282=CARTESIAN_POINT('Ctrl Pts',(-31.6011000083736,-54.539628102072,18.7770011735268));
#46283=CARTESIAN_POINT('Ctrl Pts',(-30.5405133840023,-56.0966679300985,
18.6658632829588));
#46284=CARTESIAN_POINT('Ctrl Pts',(-31.2734670813295,-57.8321781984269,
18.5547253923907));
#46285=CARTESIAN_POINT('Ctrl Pts',(-33.1290802689522,-58.1576266764213,
18.4435875018227));
#46286=CARTESIAN_POINT('Ctrl Pts',(-34.4088891521439,-56.7751266813415,
18.3324496112546));
#46287=CARTESIAN_POINT('Ctrl Pts',(-33.9414701461048,-54.9500961372979,
18.2213117206866));
#46288=CARTESIAN_POINT('Ctrl Pts',(-32.1546571679518,-54.353006198509,18.1101738301185));
#46289=CARTESIAN_POINT('Ctrl Pts',(-30.6839404004271,-55.530380057408,17.9990359395505));
#46290=CARTESIAN_POINT('Ctrl Pts',(-30.8754835799079,-57.4045540686174,
17.8878980489824));
#46291=CARTESIAN_POINT('Ctrl Pts',(-32.5539650619684,-58.2600755050979,
17.7767601584144));
#46292=CARTESIAN_POINT('Ctrl Pts',(-34.1830517108038,-57.3138758937664,
17.6656222678464));
#46293=CARTESIAN_POINT('Ctrl Pts',(-34.271622041636,-55.4320224695076,17.5544843772783));
#46294=CARTESIAN_POINT('Ctrl Pts',(-32.7386066261983,-54.3369970132153,
17.4433464867103));
#46295=CARTESIAN_POINT('Ctrl Pts',(-30.9871918598182,-55.0310887434669,
17.3322085961423));
#46296=CARTESIAN_POINT('Ctrl Pts',(-30.6204675405577,-56.8789876280276,
17.2210707055742));
#46297=CARTESIAN_POINT('Ctrl Pts',(-31.9741005967727,-58.1892908612603,
17.1099328150062));
#46298=CARTESIAN_POINT('Ctrl Pts',(-33.8090953408665,-57.7626630339378,
16.9987949244381));
#46299=CARTESIAN_POINT('Ctrl Pts',(-34.4458602733144,-55.989601434697,16.8876570338701));
#46300=CARTESIAN_POINT('Ctrl Pts',(-33.3015572300412,-54.493009453209,16.776519143302));
#46301=CARTESIAN_POINT('Ctrl Pts',(-31.4235797638343,-54.6427347026375,
16.665381252734));
#46302=CARTESIAN_POINT('Ctrl Pts',(-30.5308619472252,-56.3017319641806,
16.554243362166));
#46303=CARTESIAN_POINT('Ctrl Pts',(-31.4405185218662,-57.9515022300392,
16.4431054715979));
#46304=CARTESIAN_POINT('Ctrl Pts',(-33.3199305087784,-58.0819920662062,
16.3319675810299));
#46305=CARTESIAN_POINT('Ctrl Pts',(-34.4488508023651,-56.5737626457811,
16.2208296904618));
#46306=CARTESIAN_POINT('Ctrl Pts',(-33.7939658550683,-54.8073134617672,
16.1096917998938));
#46307=CARTESIAN_POINT('Ctrl Pts',(-31.9546992860713,-54.3994954851817,
15.9985539093257));
#46308=CARTESIAN_POINT('Ctrl Pts',(-30.6145526446348,-55.7235891349781,
15.8874160187577));
#46309=CARTESIAN_POINT('Ctrl Pts',(-31.0001773500498,-57.5676364772256,
15.7762781281896));
#46310=CARTESIAN_POINT('Ctrl Pts',(-32.758606735993,-58.2437600667033,15.6651402376216));
#46311=CARTESIAN_POINT('Ctrl Pts',(-34.2803304439162,-57.1330963140847,
15.5540023470536));
#46312=CARTESIAN_POINT('Ctrl Pts',(-34.1724975057335,-55.2522483481541,
15.4428644564855));
#46313=CARTESIAN_POINT('Ctrl Pts',(-32.5338086340801,-54.3227776419367,
15.3317265659175));
#46314=CARTESIAN_POINT('Ctrl Pts',(-30.8641743343578,-55.195439274664,15.2205886753495));
#46315=CARTESIAN_POINT('Ctrl Pts',(-30.6918298216846,-57.0714761554116,
15.1094507847814));
#46316=CARTESIAN_POINT('Ctrl Pts',(-32.1745239717376,-58.2337304551948,
14.9983128942134));
#46317=CARTESIAN_POINT('Ctrl Pts',(-33.9551300366822,-57.618377625218,14.8871750036453));
#46318=CARTESIAN_POINT('Ctrl Pts',(-34.4038390465812,-55.788657104035,14.7760371130773));
#46319=CARTESIAN_POINT('Ctrl Pts',(-33.1099426465396,-54.4193328057006,
14.6648992225092));
#46320=CARTESIAN_POINT('Ctrl Pts',(-31.2577587039999,-54.7637628485765,
14.5537613319412));
#46321=CARTESIAN_POINT('Ctrl Pts',(-30.5426125496715,-56.5066863904105,
14.4426234413731));
#46322=CARTESIAN_POINT('Ctrl Pts',(-31.6190848424819,-58.0527859832772,
14.3314855508051));
#46323=CARTESIAN_POINT('Ctrl Pts',(-33.5018697389164,-57.9868986634345,
14.2203476602371));
#46324=CARTESIAN_POINT('Ctrl Pts',(-34.4676299603036,-56.3693327876153,
14.109209769669));
#46325=CARTESIAN_POINT('Ctrl Pts',(-33.6324000499911,-54.680662853446,13.998071879101));
#46326=CARTESIAN_POINT('Ctrl Pts',(-31.7606637541616,-54.466551391645,13.886933988533));
#46327=CARTESIAN_POINT('Ctrl Pts',(-30.5656658770528,-55.9229694665903,
13.7757960979649));
#46328=CARTESIAN_POINT('Ctrl Pts',(-31.141154796329,-57.7168562799665,13.6646582073969));
#46329=CARTESIAN_POINT('Ctrl Pts',(-32.9604725206547,-58.206216496256,13.5535203168288));
#46330=CARTESIAN_POINT('Ctrl Pts',(-34.358189658021,-56.9431939941263,13.4423824262608));
#46331=CARTESIAN_POINT('Ctrl Pts',(-34.0553346792797,-55.0837258210724,
13.3312445356927));
#46332=CARTESIAN_POINT('Ctrl Pts',(-32.3283638467564,-54.3300480294051,
13.2201066451247));
#46333=CARTESIAN_POINT('Ctrl Pts',(-30.7594958530052,-55.3715226379037,
13.1089687545567));
#46334=CARTESIAN_POINT('Ctrl Pts',(-30.7817150891479,-57.2558511192949,
12.9978308639886));
#46335=CARTESIAN_POINT('Ctrl Pts',(-32.3808507372123,-58.2563466091156,
12.8866929734206));
#46336=CARTESIAN_POINT('Ctrl Pts',(-33.5126766583317,-57.7258551932599,
12.8126010463752));
#46337=CARTESIAN_POINT('Ctrl Pts',(-33.8412759334222,-57.2798490351089,
12.7755550828525));
#46338=CARTESIAN_POINT('Ctrl Pts',(-32.1764322475374,-58.057840198652,22.0748149723825));
#46339=CARTESIAN_POINT('Ctrl Pts',(-32.7637320936894,-58.1654341743444,
22.0377690088598));
#46340=CARTESIAN_POINT('Ctrl Pts',(-34.0440927468328,-57.7463414713666,
21.9636770818144));
#46341=CARTESIAN_POINT('Ctrl Pts',(-34.5610498473198,-55.7801182186225,
21.8525391912464));
#46342=CARTESIAN_POINT('Ctrl Pts',(-33.1872931810462,-54.2841586241499,
21.7414013006783));
#46343=CARTESIAN_POINT('Ctrl Pts',(-31.1865118697811,-54.624701565945,21.6302634101103));
#46344=CARTESIAN_POINT('Ctrl Pts',(-30.386953980439,-56.4915070712039,21.5191255195423));
#46345=CARTESIAN_POINT('Ctrl Pts',(-31.5220039764197,-58.1751404650056,
21.4079876289743));
#46346=CARTESIAN_POINT('Ctrl Pts',(-33.551968611483,-58.1349155948397,21.2968497384062));
#46347=CARTESIAN_POINT('Ctrl Pts',(-34.6191824416203,-56.4074696262487,
21.1857118478381));
#46348=CARTESIAN_POINT('Ctrl Pts',(-33.7466206069902,-54.5740439227395,
21.0745739572701));
#46349=CARTESIAN_POINT('Ctrl Pts',(-31.7330447371731,-54.312748623095,20.963436066702));
#46350=CARTESIAN_POINT('Ctrl Pts',(-30.4214557589377,-55.8627728590726,
20.852298176134));
#46351=CARTESIAN_POINT('Ctrl Pts',(-31.0123898691881,-57.8053505883217,
20.741160285566));
#46352=CARTESIAN_POINT('Ctrl Pts',(-32.9649464200546,-58.3624240204495,
20.6300223949979));
#46353=CARTESIAN_POINT('Ctrl Pts',(-34.4919342294713,-57.0240947100386,
20.5188845044299));
#46354=CARTESIAN_POINT('Ctrl Pts',(-34.195681054595,-55.0153520590646,20.4077466138619));
#46355=CARTESIAN_POINT('Ctrl Pts',(-32.3473522766853,-54.1748202940219,
20.2966087232938));
#46356=CARTESIAN_POINT('Ctrl Pts',(-30.6387434429966,-55.2718480227484,
20.1854708327258));
#46357=CARTESIAN_POINT('Ctrl Pts',(-30.6337639679481,-57.3023131486427,
20.0743329421578));
#46358=CARTESIAN_POINT('Ctrl Pts',(-32.3369714356807,-58.4077080025365,
19.9631950515897));
#46359=CARTESIAN_POINT('Ctrl Pts',(-34.1894008281341,-57.5762520948665,
19.8520571610217));
#46360=CARTESIAN_POINT('Ctrl Pts',(-34.4955024680362,-55.5689864691375,
19.7409192704536));
#46361=CARTESIAN_POINT('Ctrl Pts',(-32.975098076127,-54.2231841055976,19.6297813798856));
#46362=CARTESIAN_POINT('Ctrl Pts',(-31.0198310233036,-54.770673175488,19.5186434893175));
#46363=CARTESIAN_POINT('Ctrl Pts',(-30.419379423035,-56.710330721464,19.4075055987495));
#46364=CARTESIAN_POINT('Ctrl Pts',(-31.7233434317422,-58.2667661958427,
19.2963677081814));
#46365=CARTESIAN_POINT('Ctrl Pts',(-33.7381900057412,-58.0153565570662,
19.1852298176134));
#46366=CARTESIAN_POINT('Ctrl Pts',(-34.6197072252153,-56.1862198990257,
19.0740919270454));
#46367=CARTESIAN_POINT('Ctrl Pts',(-33.5610323824551,-54.4535857484765,
18.9629540364773));
#46368=CARTESIAN_POINT('Ctrl Pts',(-31.5311825670481,-54.4033537929088,
18.8518161459093));
#46369=CARTESIAN_POINT('Ctrl Pts',(-30.388102335189,-56.0815019108804,18.7406782553412));
#46370=CARTESIAN_POINT('Ctrl Pts',(-31.1780659864649,-57.9520020985391,
18.6295403647732));
#46371=CARTESIAN_POINT('Ctrl Pts',(-33.1780108320884,-58.3027643211954,
18.5184024742051));
#46372=CARTESIAN_POINT('Ctrl Pts',(-34.5573646739318,-56.812731938543,18.4072645836371));
#46373=CARTESIAN_POINT('Ctrl Pts',(-34.0535892976251,-54.8457484885378,
18.296126693069));
#46374=CARTESIAN_POINT('Ctrl Pts',(-32.1277960183002,-54.20221623008,18.1849888025011));
#46375=CARTESIAN_POINT('Ctrl Pts',(-30.5426852645059,-55.4711675374879,
18.073850911933));
#46376=CARTESIAN_POINT('Ctrl Pts',(-30.749126885568,-57.4911168882046,17.962713021365));
#46377=CARTESIAN_POINT('Ctrl Pts',(-32.5581625245214,-58.4131817337352,
17.8515751307969));
#46378=CARTESIAN_POINT('Ctrl Pts',(-34.3139613451725,-57.3933856640392,
17.7404372402289));
#46379=CARTESIAN_POINT('Ctrl Pts',(-34.4094207748664,-55.3651595869832,
17.6292993496608));
#46380=CARTESIAN_POINT('Ctrl Pts',(-32.7571657150207,-54.1849618325449,
17.5181614590928));
#46381=CARTESIAN_POINT('Ctrl Pts',(-30.869523959759,-54.9330407897143,17.4070235685247));
#46382=CARTESIAN_POINT('Ctrl Pts',(-30.4742754149858,-56.9246713052021,
17.2958856779567));
#46383=CARTESIAN_POINT('Ctrl Pts',(-31.9331955561555,-58.3368913815558,
17.1847477873886));
#46384=CARTESIAN_POINT('Ctrl Pts',(-33.9109182327756,-57.8770799672243,
17.0736098968206));
#46385=CARTESIAN_POINT('Ctrl Pts',(-34.5972114500352,-55.9661076643608,
16.9624720062525));
#46386=CARTESIAN_POINT('Ctrl Pts',(-33.3639032430821,-54.3531090936767,
16.8513341156845));
#46387=CARTESIAN_POINT('Ctrl Pts',(-31.339854600407,-54.5144801395667,16.7401962251165));
#46388=CARTESIAN_POINT('Ctrl Pts',(-30.3777001989227,-56.3025160536558,
16.6290583345484));
#46389=CARTESIAN_POINT('Ctrl Pts',(-31.3581108738821,-58.0806072860715,
16.5179204439804));
#46390=CARTESIAN_POINT('Ctrl Pts',(-33.3837056158788,-58.2212467668584,
16.4067825534123));
#46391=CARTESIAN_POINT('Ctrl Pts',(-34.6004345857623,-56.5957055842903,
16.2956446628443));
#46392=CARTESIAN_POINT('Ctrl Pts',(-33.8946119587414,-54.6918600176663,
16.1845067722763));
#46393=CARTESIAN_POINT('Ctrl Pts',(-31.9122851899249,-54.252321505187,16.0733688817082));
#46394=CARTESIAN_POINT('Ctrl Pts',(-30.467900451878,-55.6794046320458,15.9622309911402));
#46395=CARTESIAN_POINT('Ctrl Pts',(-30.8835194758665,-57.6668840279746,
15.8510931005722));
#46396=CARTESIAN_POINT('Ctrl Pts',(-32.7787214556042,-58.3955972623921,
15.7399552100041));
#46397=CARTESIAN_POINT('Ctrl Pts',(-34.4188065263637,-57.1985448475426,
15.6288173194361));
#46398=CARTESIAN_POINT('Ctrl Pts',(-34.3025862222909,-55.1714024344819,
15.517679428868));
#46399=CARTESIAN_POINT('Ctrl Pts',(-32.5364383072491,-54.1696364627501,
15.4065415383));
#46400=CARTESIAN_POINT('Ctrl Pts',(-30.7369379943181,-55.1101746880588,
15.2954036477319));
#46401=CARTESIAN_POINT('Ctrl Pts',(-30.5511883337254,-57.1321318043788,
15.1842657571639));
#46402=CARTESIAN_POINT('Ctrl Pts',(-32.1492080841852,-58.3847875365432,
15.0731278665959));
#46403=CARTESIAN_POINT('Ctrl Pts',(-34.0683116696875,-57.7215718789046,
14.9619899760278));
#46404=CARTESIAN_POINT('Ctrl Pts',(-34.5519217655404,-55.7495336601205,
14.8508520854598));
#46405=CARTESIAN_POINT('Ctrl Pts',(-33.1573846641151,-54.2737017945639,
14.7397141948917));
#46406=CARTESIAN_POINT('Ctrl Pts',(-31.1611357940719,-54.644921989334,14.6285763043237));
#46407=CARTESIAN_POINT('Ctrl Pts',(-30.3903647762991,-56.5234120631583,
14.5174384137557));
#46408=CARTESIAN_POINT('Ctrl Pts',(-31.5505662815605,-58.1897690023091,
14.4063005231876));
#46409=CARTESIAN_POINT('Ctrl Pts',(-33.5797962817343,-58.1187568934328,
14.2951626326196));
#46410=CARTESIAN_POINT('Ctrl Pts',(-34.620674407496,-56.3753749443396,14.1840247420515));
#46411=CARTESIAN_POINT('Ctrl Pts',(-33.7204793856122,-54.555358384138,14.0728868514835));
#46412=CARTESIAN_POINT('Ctrl Pts',(-31.7031573584894,-54.3245930946511,
13.9617489609154));
#46413=CARTESIAN_POINT('Ctrl Pts',(-30.4152112171298,-55.8942929876505,
13.8506110703474));
#46414=CARTESIAN_POINT('Ctrl Pts',(-31.0354623047469,-57.8277103129715,
13.7394731797794));
#46415=CARTESIAN_POINT('Ctrl Pts',(-32.9962885855616,-58.3551335112703,
13.6283352892113));
#46416=CARTESIAN_POINT('Ctrl Pts',(-34.5027217167555,-56.9938717138819,
13.5171973986433));
#46417=CARTESIAN_POINT('Ctrl Pts',(-34.1763103408583,-54.9897720377718,
13.4060595080752));
#46418=CARTESIAN_POINT('Ctrl Pts',(-32.3150137958213,-54.1774723490436,
13.2949216175072));
#46419=CARTESIAN_POINT('Ctrl Pts',(-30.6241175042368,-55.2999540111744,
13.1837837269392));
#46420=CARTESIAN_POINT('Ctrl Pts',(-30.6480649772844,-57.3308476580601,
13.0726458363711));
#46421=CARTESIAN_POINT('Ctrl Pts',(-32.3715831750057,-58.4091628000751,
12.9615079458031));
#46422=CARTESIAN_POINT('Ctrl Pts',(-33.5914437753638,-57.8374091717516,
12.8874160187577));
#46423=CARTESIAN_POINT('Ctrl Pts',(-33.9456018676194,-57.3567121584624,
12.850370055235));
#46424=CARTESIAN_POINT('Ctrl Pts',(-32.1530810684833,-58.1853022036361,
22.149629944765));
#46425=CARTESIAN_POINT('Ctrl Pts',(-32.7827650637403,-58.3006610019117,
22.1125839812423));
#46426=CARTESIAN_POINT('Ctrl Pts',(-34.1555265529926,-57.8513232925233,
22.038492054197));
#46427=CARTESIAN_POINT('Ctrl Pts',(-34.7097913200344,-55.7432019955959,
21.9273541636289));
#46428=CARTESIAN_POINT('Ctrl Pts',(-33.2368936310637,-54.1392822596,21.8162162730608));
#46429=CARTESIAN_POINT('Ctrl Pts',(-31.0917202958965,-54.5044014428434,
21.7050783824928));
#46430=CARTESIAN_POINT('Ctrl Pts',(-30.2344600573677,-56.5059302302613,
21.5939404919248));
#46431=CARTESIAN_POINT('Ctrl Pts',(-31.4514241362253,-58.3110677744024,
21.4828026013567));
#46432=CARTESIAN_POINT('Ctrl Pts',(-33.6278868920259,-58.2679399630795,
21.3716647107887));
#46433=CARTESIAN_POINT('Ctrl Pts',(-34.7721192168892,-56.4158279861738,
21.2605268202206));
#46434=CARTESIAN_POINT('Ctrl Pts',(-33.836586497549,-54.4500879480027,21.1493889296526));
#46435=CARTESIAN_POINT('Ctrl Pts',(-31.6776952484417,-54.1699355364194,
21.0382510390845));
#46436=CARTESIAN_POINT('Ctrl Pts',(-30.2714517539787,-55.8318216411929,
20.9271131485165));
#46437=CARTESIAN_POINT('Ctrl Pts',(-30.9050322902485,-57.9145909687611,
20.8159752579484));
#46438=CARTESIAN_POINT('Ctrl Pts',(-32.9985005892282,-58.511867175612,20.7048373673804));
#46439=CARTESIAN_POINT('Ctrl Pts',(-34.6356877787742,-57.0769535575162,
20.5936994768124));
#46440=CARTESIAN_POINT('Ctrl Pts',(-34.3180546583401,-54.9232443301155,
20.4825615862444));
#46441=CARTESIAN_POINT('Ctrl Pts',(-32.3363360233899,-54.022053220633,20.3714236956763));
#46442=CARTESIAN_POINT('Ctrl Pts',(-30.5044206163321,-55.1982510481283,
20.2602858051083));
#46443=CARTESIAN_POINT('Ctrl Pts',(-30.4990817834286,-57.3752504140916,
20.1491479145402));
#46444=CARTESIAN_POINT('Ctrl Pts',(-32.3252060197288,-58.5604192039303,
20.0380100239722));
#46445=CARTESIAN_POINT('Ctrl Pts',(-34.3113212016315,-57.6689589366545,
19.9268721334042));
#46446=CARTESIAN_POINT('Ctrl Pts',(-34.6395135293347,-55.5168333281896,
19.8157342428361));
#46447=CARTESIAN_POINT('Ctrl Pts',(-33.0093848681805,-54.0739073430178,
19.7045963522681));
#46448=CARTESIAN_POINT('Ctrl Pts',(-30.9130104562287,-54.6609075051103,
19.5934584617));
#46449=CARTESIAN_POINT('Ctrl Pts',(-30.269225573442,-56.740545906147,19.482320571132));
#46450=CARTESIAN_POINT('Ctrl Pts',(-31.6672938209546,-58.4093059344153,
19.3711826805639));
#46451=CARTESIAN_POINT('Ctrl Pts',(-33.8275474781934,-58.1397526102859,
19.2600447899959));
#46452=CARTESIAN_POINT('Ctrl Pts',(-34.7726818729719,-56.1786111486416,
19.1489068994278));
#46453=CARTESIAN_POINT('Ctrl Pts',(-33.6376047755825,-54.3209365700001,
19.0377690088598));
#46454=CARTESIAN_POINT('Ctrl Pts',(-31.4612651257226,-54.2670794837456,
18.9266311182918));
#46455=CARTESIAN_POINT('Ctrl Pts',(-30.2356912863756,-56.0663358916622,
18.8154932277237));
#46456=CARTESIAN_POINT('Ctrl Pts',(-31.0826648916004,-58.0718259986512,
18.7043553371557));
#46457=CARTESIAN_POINT('Ctrl Pts',(-33.2269413952247,-58.4479019659694,
18.5932174465876));
#46458=CARTESIAN_POINT('Ctrl Pts',(-34.7058401957198,-56.8503371957446,
18.4820795560196));
#46459=CARTESIAN_POINT('Ctrl Pts',(-34.1657084491453,-54.7414008397775,
18.3709416654516));
#46460=CARTESIAN_POINT('Ctrl Pts',(-32.1009348686486,-54.0514262616512,
18.2598037748835));
#46461=CARTESIAN_POINT('Ctrl Pts',(-30.4014301285847,-55.4119550175678,
18.1486658843155));
#46462=CARTESIAN_POINT('Ctrl Pts',(-30.6227701912281,-57.5776797077918,
18.0375279937474));
#46463=CARTESIAN_POINT('Ctrl Pts',(-32.5623599870745,-58.5662879623725,
17.9263901031794));
#46464=CARTESIAN_POINT('Ctrl Pts',(-34.4448709795413,-57.472895434312,17.8152522126114));
#46465=CARTESIAN_POINT('Ctrl Pts',(-34.5472195080969,-55.2982967044589,
17.7041143220433));
#46466=CARTESIAN_POINT('Ctrl Pts',(-32.7757248038432,-54.0329266518745,
17.5929764314753));
#46467=CARTESIAN_POINT('Ctrl Pts',(-30.7518560596998,-54.8349928359617,
17.4818385409072));
#46468=CARTESIAN_POINT('Ctrl Pts',(-30.328083289414,-56.9703549823765,17.3707006503392));
#46469=CARTESIAN_POINT('Ctrl Pts',(-31.8922905155383,-58.4844919018513,
17.2595627597711));
#46470=CARTESIAN_POINT('Ctrl Pts',(-34.0127411246847,-57.9914969005106,
17.1484248692031));
#46471=CARTESIAN_POINT('Ctrl Pts',(-34.7485626267561,-55.9426138940248,
17.037286978635));
#46472=CARTESIAN_POINT('Ctrl Pts',(-33.426249256123,-54.2132087341443,16.926149088067));
#46473=CARTESIAN_POINT('Ctrl Pts',(-31.2561294369797,-54.3862255764959,
16.815011197499));
#46474=CARTESIAN_POINT('Ctrl Pts',(-30.2245384506201,-56.3033001431311,
16.7038733069309));
#46475=CARTESIAN_POINT('Ctrl Pts',(-31.275703225898,-58.2097123421037,16.5927354163629));
#46476=CARTESIAN_POINT('Ctrl Pts',(-33.4474807229792,-58.3605014675107,
16.4815975257949));
#46477=CARTESIAN_POINT('Ctrl Pts',(-34.7520183691595,-56.6176485227995,
16.3704596352268));
#46478=CARTESIAN_POINT('Ctrl Pts',(-33.9952580624144,-54.5764065735656,
16.2593217446588));
#46479=CARTESIAN_POINT('Ctrl Pts',(-31.8698710937785,-54.1051475251923,
16.1481838540907));
#46480=CARTESIAN_POINT('Ctrl Pts',(-30.3212482591213,-55.6352201291135,
16.0370459635227));
#46481=CARTESIAN_POINT('Ctrl Pts',(-30.7668616016832,-57.7661315787237,
15.9259080729546));
#46482=CARTESIAN_POINT('Ctrl Pts',(-32.7988361752155,-58.547434458081,15.8147701823866));
#46483=CARTESIAN_POINT('Ctrl Pts',(-34.5572826088111,-57.2639933810004,
15.7036322918185));
#46484=CARTESIAN_POINT('Ctrl Pts',(-34.4326749388483,-55.0905565208099,
15.5924944012505));
#46485=CARTESIAN_POINT('Ctrl Pts',(-32.5390679804181,-54.0164952835633,
15.4813565106825));
#46486=CARTESIAN_POINT('Ctrl Pts',(-30.6097016542784,-55.0249101014538,
15.3702186201144));
#46487=CARTESIAN_POINT('Ctrl Pts',(-30.4105468457662,-57.192787453346,15.2590807295464));
#46488=CARTESIAN_POINT('Ctrl Pts',(-32.1238921966328,-58.5358446178915,
15.1479428389784));
#46489=CARTESIAN_POINT('Ctrl Pts',(-34.1814933026927,-57.8247661325911,
15.0368049484103));
#46490=CARTESIAN_POINT('Ctrl Pts',(-34.7000044844997,-55.7104102162061,
14.9256670578423));
#46491=CARTESIAN_POINT('Ctrl Pts',(-33.2048266816906,-54.128070783427,14.8145291672742));
#46492=CARTESIAN_POINT('Ctrl Pts',(-31.064512884144,-54.5260811300915,14.7033912767062));
#46493=CARTESIAN_POINT('Ctrl Pts',(-30.2381170029267,-56.5401377359062,
14.5922533861381));
#46494=CARTESIAN_POINT('Ctrl Pts',(-31.4820477206391,-58.3267520213409,
14.4811154955701));
#46495=CARTESIAN_POINT('Ctrl Pts',(-33.6577228245522,-58.2506151234313,
14.369977605002));
#46496=CARTESIAN_POINT('Ctrl Pts',(-34.7737188546885,-56.3814171010637,
14.258839714434));
#46497=CARTESIAN_POINT('Ctrl Pts',(-33.8085587212332,-54.4300539148301,
14.147701823866));
#46498=CARTESIAN_POINT('Ctrl Pts',(-31.6456509628172,-54.182634797657,14.0365639332979));
#46499=CARTESIAN_POINT('Ctrl Pts',(-30.2647565572066,-55.8656165087107,
13.9254260427299));
#46500=CARTESIAN_POINT('Ctrl Pts',(-30.9297698131649,-57.9385643459764,
13.8142881521619));
#46501=CARTESIAN_POINT('Ctrl Pts',(-33.0321046504685,-58.5040505262846,
13.7031502615938));
#46502=CARTESIAN_POINT('Ctrl Pts',(-34.6472537754902,-57.0445494336376,
13.5920123710258));
#46503=CARTESIAN_POINT('Ctrl Pts',(-34.2972860024369,-54.8958182544712,
13.4808744804577));
#46504=CARTESIAN_POINT('Ctrl Pts',(-32.3016637448863,-54.0248966686821,
13.3697365898897));
#46505=CARTESIAN_POINT('Ctrl Pts',(-30.4887391554684,-55.2283853844451,
13.2585986993216));
#46506=CARTESIAN_POINT('Ctrl Pts',(-30.5144148654209,-57.4058441968251,
13.1474608087536));
#46507=CARTESIAN_POINT('Ctrl Pts',(-32.3623156127991,-58.5619789910346,
13.0363229181856));
#46508=CARTESIAN_POINT('Ctrl Pts',(-33.6702108923959,-57.9489631502434,
12.9622309911402));
#46509=CARTESIAN_POINT('Ctrl Pts',(-34.0499278018167,-57.4335752818158,
12.9251850276175));
#46510=CARTESIAN_POINT('Ctrl Pts',(-32.1297298894292,-58.3127642086202,
22.2244449171475));
#46511=CARTESIAN_POINT('Ctrl Pts',(-32.8017980337912,-58.4358878294791,
22.1873989536248));
#46512=CARTESIAN_POINT('Ctrl Pts',(-34.2669603591524,-57.95630511368,22.1133070265794));
#46513=CARTESIAN_POINT('Ctrl Pts',(-34.858532792749,-55.7062857725693,22.0021691360114));
#46514=CARTESIAN_POINT('Ctrl Pts',(-33.2864940810812,-53.9944058950499,
21.8910312454434));
#46515=CARTESIAN_POINT('Ctrl Pts',(-30.9969287220119,-54.384101319742,21.7798933548753));
#46516=CARTESIAN_POINT('Ctrl Pts',(-30.0819661342964,-56.5203533893187,
21.6687554643073));
#46517=CARTESIAN_POINT('Ctrl Pts',(-31.380844296031,-58.4469950837991,21.5576175737392));
#46518=CARTESIAN_POINT('Ctrl Pts',(-33.7038051725687,-58.4009643313194,
21.4464796831712));
#46519=CARTESIAN_POINT('Ctrl Pts',(-34.9250559921582,-56.4241863460987,
21.3353417926031));
#46520=CARTESIAN_POINT('Ctrl Pts',(-33.9265523881077,-54.3261319732661,
21.2242039020351));
#46521=CARTESIAN_POINT('Ctrl Pts',(-31.6223457597103,-54.0271224497437,
21.113066011467));
#46522=CARTESIAN_POINT('Ctrl Pts',(-30.1214477490197,-55.8008704233132,
21.001928120899));
#46523=CARTESIAN_POINT('Ctrl Pts',(-30.7976747113088,-58.0238313492005,
20.890790230331));
#46524=CARTESIAN_POINT('Ctrl Pts',(-33.0320547584019,-58.6613103307746,
20.7796523397629));
#46525=CARTESIAN_POINT('Ctrl Pts',(-34.779441328077,-57.1298124049937,20.6685144491949));
#46526=CARTESIAN_POINT('Ctrl Pts',(-34.4404282620852,-54.8311366011663,
20.5573765586268));
#46527=CARTESIAN_POINT('Ctrl Pts',(-32.3253197700946,-53.8692861472442,
20.4462386680588));
#46528=CARTESIAN_POINT('Ctrl Pts',(-30.3700977896676,-55.1246540735083,
20.3351007774907));
#46529=CARTESIAN_POINT('Ctrl Pts',(-30.3643995989091,-57.4481876795404,
20.2239628869227));
#46530=CARTESIAN_POINT('Ctrl Pts',(-32.3134406037768,-58.7131304053242,
20.1128249963547));
#46531=CARTESIAN_POINT('Ctrl Pts',(-34.4332415751289,-57.7616657784424,
20.0016871057866));
#46532=CARTESIAN_POINT('Ctrl Pts',(-34.7835245906331,-55.4646801872418,
19.8905492152186));
#46533=CARTESIAN_POINT('Ctrl Pts',(-33.043671660234,-53.924630580438,19.7794113246506));
#46534=CARTESIAN_POINT('Ctrl Pts',(-30.8061898891539,-54.5511418347326,
19.6682734340825));
#46535=CARTESIAN_POINT('Ctrl Pts',(-30.1190717238489,-56.77076109083,19.5571355435145));
#46536=CARTESIAN_POINT('Ctrl Pts',(-31.611244210167,-58.5518456729879,19.4459976529464));
#46537=CARTESIAN_POINT('Ctrl Pts',(-33.9169049506455,-58.2641486635056,
19.3348597623784));
#46538=CARTESIAN_POINT('Ctrl Pts',(-34.9256565207284,-56.1710023982575,
19.2237218718104));
#46539=CARTESIAN_POINT('Ctrl Pts',(-33.71417716871,-54.1882873915237,19.1125839812423));
#46540=CARTESIAN_POINT('Ctrl Pts',(-31.3913476843971,-54.1308051745824,
19.0014460906743));
#46541=CARTESIAN_POINT('Ctrl Pts',(-30.0832802375623,-56.0511698724442,
18.8903082001062));
#46542=CARTESIAN_POINT('Ctrl Pts',(-30.9872637967358,-58.1916498987633,
18.7791703095382));
#46543=CARTESIAN_POINT('Ctrl Pts',(-33.2758719583609,-58.5930396107435,
18.6680324189701));
#46544=CARTESIAN_POINT('Ctrl Pts',(-34.8543157175077,-56.8879424529461,
18.5568945284021));
#46545=CARTESIAN_POINT('Ctrl Pts',(-34.2778276006655,-54.6370531910174,
18.445756637834));
#46546=CARTESIAN_POINT('Ctrl Pts',(-32.074073718997,-53.9006362932222,18.334618747266));
#46547=CARTESIAN_POINT('Ctrl Pts',(-30.2601749926636,-55.3527424976477,
18.223480856698));
#46548=CARTESIAN_POINT('Ctrl Pts',(-30.4964134968882,-57.664242527379,18.1123429661299));
#46549=CARTESIAN_POINT('Ctrl Pts',(-32.5665574496276,-58.7193941910097,
18.0012050755619));
#46550=CARTESIAN_POINT('Ctrl Pts',(-34.57578061391,-57.5524052045849,17.8900671849938));
#46551=CARTESIAN_POINT('Ctrl Pts',(-34.6850182413274,-55.2314338219344,
17.7789292944258));
#46552=CARTESIAN_POINT('Ctrl Pts',(-32.7942838926656,-53.8808914712041,
17.6677914038577));
#46553=CARTESIAN_POINT('Ctrl Pts',(-30.6341881596407,-54.7369448822092,
17.5566535132897));
#46554=CARTESIAN_POINT('Ctrl Pts',(-30.1818911638421,-57.0160386595509,
17.4455156227217));
#46555=CARTESIAN_POINT('Ctrl Pts',(-31.8513854749211,-58.6320924221469,
17.3343777321536));
#46556=CARTESIAN_POINT('Ctrl Pts',(-34.1145640165938,-58.1059138337969,
17.2232398415856));
#46557=CARTESIAN_POINT('Ctrl Pts',(-34.899913803477,-55.9191201236888,17.1121019510176));
#46558=CARTESIAN_POINT('Ctrl Pts',(-33.4885952691639,-54.0733083746118,
17.0009640604495));
#46559=CARTESIAN_POINT('Ctrl Pts',(-31.1724042735525,-54.2579710134251,
16.8898261698815));
#46560=CARTESIAN_POINT('Ctrl Pts',(-30.0713767023175,-56.3040842326063,
16.7786882793134));
#46561=CARTESIAN_POINT('Ctrl Pts',(-31.1932955779139,-58.3388173981362,
16.6675503887454));
#46562=CARTESIAN_POINT('Ctrl Pts',(-33.5112558300796,-58.4997561681628,
16.5564124981773));
#46563=CARTESIAN_POINT('Ctrl Pts',(-34.9036021525567,-56.6395914613089,
16.4452746076093));
#46564=CARTESIAN_POINT('Ctrl Pts',(-34.0959041660875,-54.4609531294646,
16.3341367170413));
#46565=CARTESIAN_POINT('Ctrl Pts',(-31.8274569976321,-53.9579735451976,
16.2229988264732));
#46566=CARTESIAN_POINT('Ctrl Pts',(-30.1745960663645,-55.5910356261813,
16.1118609359052));
#46567=CARTESIAN_POINT('Ctrl Pts',(-30.6502037274999,-57.8653791294726,
16.0007230453371));
#46568=CARTESIAN_POINT('Ctrl Pts',(-32.8189508948268,-58.6992716537698,
15.8895851547691));
#46569=CARTESIAN_POINT('Ctrl Pts',(-34.6957586912586,-57.3294419144583,
15.778447264201));
#46570=CARTESIAN_POINT('Ctrl Pts',(-34.5627636554057,-55.0097106071377,
15.667309373633));
#46571=CARTESIAN_POINT('Ctrl Pts',(-32.5416976535871,-53.8633541043767,
15.556171483065));
#46572=CARTESIAN_POINT('Ctrl Pts',(-30.4824653142387,-54.9396455148486,
15.4450335924969));
#46573=CARTESIAN_POINT('Ctrl Pts',(-30.269905357807,-57.2534431023133,15.3338957019289));
#46574=CARTESIAN_POINT('Ctrl Pts',(-32.0985763090804,-58.6869016992398,
15.2227578113608));
#46575=CARTESIAN_POINT('Ctrl Pts',(-34.2946749356979,-57.9279603862777,
15.1116199207928));
#46576=CARTESIAN_POINT('Ctrl Pts',(-34.848087203459,-55.6712867722916,15.0004820302248));
#46577=CARTESIAN_POINT('Ctrl Pts',(-33.2522686992661,-53.9824397722902,
14.8893441396567));
#46578=CARTESIAN_POINT('Ctrl Pts',(-30.967889974216,-54.407240270849,14.7782062490887));
#46579=CARTESIAN_POINT('Ctrl Pts',(-30.0858692295543,-56.5568634086542,
14.6670683585206));
#46580=CARTESIAN_POINT('Ctrl Pts',(-31.4135291597177,-58.4637350403727,
14.5559304679526));
#46581=CARTESIAN_POINT('Ctrl Pts',(-33.73564936737,-58.3824733534297,14.4447925773845));
#46582=CARTESIAN_POINT('Ctrl Pts',(-34.926763301881,-56.3874592577879,14.3336546868165));
#46583=CARTESIAN_POINT('Ctrl Pts',(-33.8966380568543,-54.3047494455222,
14.2225167962484));
#46584=CARTESIAN_POINT('Ctrl Pts',(-31.5881445671451,-54.0406765006631,
14.1113789056804));
#46585=CARTESIAN_POINT('Ctrl Pts',(-30.1143018972835,-55.8369400297709,
14.0002410151124));
#46586=CARTESIAN_POINT('Ctrl Pts',(-30.8240773215828,-58.0494183789814,
13.8891031245444));
#46587=CARTESIAN_POINT('Ctrl Pts',(-33.0679207153753,-58.6529675412989,
13.7779652339763));
#46588=CARTESIAN_POINT('Ctrl Pts',(-34.7917858342248,-57.0952271533932,
13.6668273434083));
#46589=CARTESIAN_POINT('Ctrl Pts',(-34.4182616640155,-54.8018644711707,
13.5556894528402));
#46590=CARTESIAN_POINT('Ctrl Pts',(-32.2883136939512,-53.8723209883206,
13.4445515622722));
#46591=CARTESIAN_POINT('Ctrl Pts',(-30.3533608067001,-55.1568167577159,
13.3334136717041));
#46592=CARTESIAN_POINT('Ctrl Pts',(-30.3807647535574,-57.4808407355902,
13.2222757811361));
#46593=CARTESIAN_POINT('Ctrl Pts',(-32.3530480505925,-58.7147951819942,
13.1111378905681));
#46594=CARTESIAN_POINT('Ctrl Pts',(-33.748978009428,-58.0605171287351,13.0370459635227));
#46595=CARTESIAN_POINT('Ctrl Pts',(-34.1542537360139,-57.5104384051693,
13.));
#46596=CARTESIAN_POINT('Ctrl Pts',(-32.1997834265916,-57.9303781936679,
22.));
#46597=CARTESIAN_POINT('Ctrl Pts',(-32.2590684210029,-57.9484903047675,
22.));
#46598=CARTESIAN_POINT('Ctrl Pts',(-32.3192133660472,-57.9629534896913,
22.));
#46599=CARTESIAN_POINT('Ctrl Pts',(-32.3799202087205,-57.9739415995515,
22.));
#46600=CARTESIAN_POINT('Ctrl Pts',(-32.4446390331051,-57.9856558894247,
22.));
#46601=CARTESIAN_POINT('Ctrl Pts',(-32.5099970425764,-57.9934211178936,
22.));
#46602=CARTESIAN_POINT('Ctrl Pts',(-32.5756660758662,-57.997395589509,22.));
#46603=CARTESIAN_POINT('Ctrl Pts',(-32.6331264799947,-58.0008732521725,
22.));
#46604=CARTESIAN_POINT('Ctrl Pts',(-32.6908259517003,-58.0014477926638,
22.));
#46605=CARTESIAN_POINT('Ctrl Pts',(-32.7485570677765,-57.9991916498581,
22.));
#46606=CARTESIAN_POINT('Ctrl Pts',(-32.7775225242267,-57.9980596744067,
22.));
#46607=CARTESIAN_POINT('Ctrl Pts',(-32.8064960744402,-57.9962146309827,
22.));
#46608=CARTESIAN_POINT('Ctrl Pts',(-32.8354519444006,-57.9936627183816,
22.));
#46609=CARTESIAN_POINT('Ctrl Pts',(-32.8486814477492,-57.992496787731,22.));
#46610=CARTESIAN_POINT('Ctrl Pts',(-32.8619089919099,-57.9911829627194,
22.));
#46611=CARTESIAN_POINT('Ctrl Pts',(-32.8751106149865,-57.9897244385961,
22.));
#46612=CARTESIAN_POINT('Ctrl Pts',(-32.941684568455,-57.9823693038107,22.));
#46613=CARTESIAN_POINT('Ctrl Pts',(-33.0077191568455,-57.9713290351914,
22.));
#46614=CARTESIAN_POINT('Ctrl Pts',(-33.0728927905865,-57.9567622281368,
22.));
#46615=CARTESIAN_POINT('Ctrl Pts',(-33.1392231872252,-57.9419368757016,
22.));
#46616=CARTESIAN_POINT('Ctrl Pts',(-33.2046628033255,-57.9234587511961,
22.));
#46617=CARTESIAN_POINT('Ctrl Pts',(-33.268884582548,-57.9014427391759,22.));
#46618=CARTESIAN_POINT('Ctrl Pts',(-33.3226052862378,-57.8830266243862,
22.));
#46619=CARTESIAN_POINT('Ctrl Pts',(-33.3754743938389,-57.8621340596335,
22.));
#46620=CARTESIAN_POINT('Ctrl Pts',(-33.4272987060576,-57.8388046347892,
22.));
#46621=CARTESIAN_POINT('Ctrl Pts',(-33.4511753909088,-57.8280562176677,
22.));
#46622=CARTESIAN_POINT('Ctrl Pts',(-33.4748302312922,-57.8167901903543,
22.));
#46623=CARTESIAN_POINT('Ctrl Pts',(-33.4982437788218,-57.805008661511,22.));
#46624=CARTESIAN_POINT('Ctrl Pts',(-33.5084650463385,-57.7998653931571,
22.));
#46625=CARTESIAN_POINT('Ctrl Pts',(-33.5186400680679,-57.7946238947902,
22.));
#46626=CARTESIAN_POINT('Ctrl Pts',(-33.5287548615985,-57.7892910972224,
22.));
#46627=CARTESIAN_POINT('Ctrl Pts',(-33.5908341911573,-57.7565611658915,
22.));
#46628=CARTESIAN_POINT('Ctrl Pts',(-33.6507646084003,-57.7203369576369,
22.));
#46629=CARTESIAN_POINT('Ctrl Pts',(-33.7082063151154,-57.6807516371536,
22.));
#46630=CARTESIAN_POINT('Ctrl Pts',(-33.759565116122,-57.6453582842443,22.));
#46631=CARTESIAN_POINT('Ctrl Pts',(-33.8089350520295,-57.6072772063265,
22.));
#46632=CARTESIAN_POINT('Ctrl Pts',(-33.8560671885274,-57.566568812704,22.));
#46633=CARTESIAN_POINT('Ctrl Pts',(-33.90741383547,-57.5222203135642,22.));
#46634=CARTESIAN_POINT('Ctrl Pts',(-33.9561058514875,-57.4747541508591,
22.));
#46635=CARTESIAN_POINT('Ctrl Pts',(-34.002080913029,-57.4244894418756,22.));
#46636=CARTESIAN_POINT('Ctrl Pts',(-34.0198184128286,-57.4050969661371,
22.));
#46637=CARTESIAN_POINT('Ctrl Pts',(-34.0371511842958,-57.3852874792597,
22.));
#46638=CARTESIAN_POINT('Ctrl Pts',(-34.0540743682384,-57.365077729866,22.));
#46639=CARTESIAN_POINT('Ctrl Pts',(-34.0614983915393,-57.3562119247721,
22.));
#46640=CARTESIAN_POINT('Ctrl Pts',(-34.0688431367454,-57.3472694773831,
22.));
#46641=CARTESIAN_POINT('Ctrl Pts',(-34.0760999004284,-57.3382624488758,
22.));
#46642=CARTESIAN_POINT('Ctrl Pts',(-34.1199740932065,-57.2838062033164,
22.));
#46643=CARTESIAN_POINT('Ctrl Pts',(-34.160716274024,-57.2268964747641,22.));
#46644=CARTESIAN_POINT('Ctrl Pts',(-34.1982933189855,-57.1679133931134,
22.));
#46645=CARTESIAN_POINT('Ctrl Pts',(-34.2367405668874,-57.1075643910945,
22.));
#46646=CARTESIAN_POINT('Ctrl Pts',(-34.2718749445117,-57.0450442239734,
22.));
#46647=CARTESIAN_POINT('Ctrl Pts',(-34.303629683885,-56.9807132904548,22.));
#46648=CARTESIAN_POINT('Ctrl Pts',(-34.327924112439,-56.9314959673392,22.));
#46649=CARTESIAN_POINT('Ctrl Pts',(-34.3502397773156,-56.8812176908655,
22.));
#46650=CARTESIAN_POINT('Ctrl Pts',(-34.370531746488,-56.830026000176,22.));
#46651=CARTESIAN_POINT('Ctrl Pts',(-34.3831626883497,-56.7981612135006,
22.));
#46652=CARTESIAN_POINT('Ctrl Pts',(-34.3950092682771,-56.7659423000698,
22.));
#46653=CARTESIAN_POINT('Ctrl Pts',(-34.4060577406816,-56.7334031737991,
22.));
#46654=CARTESIAN_POINT('Ctrl Pts',(-34.4122566000728,-56.715146761412,22.));
#46655=CARTESIAN_POINT('Ctrl Pts',(-34.4182059308347,-56.6967833655941,
22.));
#46656=CARTESIAN_POINT('Ctrl Pts',(-34.423893091666,-56.6783523612847,22.));
#46657=CARTESIAN_POINT('Ctrl Pts',(-34.4459473654228,-56.6068786634752,
22.));
#46658=CARTESIAN_POINT('Ctrl Pts',(-34.4640895874025,-56.5343189897119,
22.));
#46659=CARTESIAN_POINT('Ctrl Pts',(-34.4782337109683,-56.4610520163338,
22.));
#46660=CARTESIAN_POINT('Ctrl Pts',(-34.4888128880671,-56.4062515698269,
22.));
#46661=CARTESIAN_POINT('Ctrl Pts',(-34.4971546283959,-56.3510545308008,
22.));
#46662=CARTESIAN_POINT('Ctrl Pts',(-34.5032062803068,-56.2956100237224,
22.));
#46663=CARTESIAN_POINT('Ctrl Pts',(-34.5050941235358,-56.2783138310772,
22.));
#46664=CARTESIAN_POINT('Ctrl Pts',(-34.5067589921147,-56.2609935142719,
22.));
#46665=CARTESIAN_POINT('Ctrl Pts',(-34.5081989725185,-56.2436535054264,
22.));
#46666=CARTESIAN_POINT('Ctrl Pts',(-34.509588864495,-56.2269166532411,22.));
#46667=CARTESIAN_POINT('Ctrl Pts',(-34.5107684790914,-56.2101700014401,
22.));
#46668=CARTESIAN_POINT('Ctrl Pts',(-34.5117364052776,-56.1934236229725,
22.));
#46669=CARTESIAN_POINT('Ctrl Pts',(-34.5160829441432,-56.1182228629321,
22.));
#46670=CARTESIAN_POINT('Ctrl Pts',(-34.5161676811367,-56.0429913941852,
22.));
#46671=CARTESIAN_POINT('Ctrl Pts',(-34.5118795397106,-55.9680950253044,
22.));
#46672=CARTESIAN_POINT('Ctrl Pts',(-34.5085977311867,-55.9107751943145,
22.));
#46673=CARTESIAN_POINT('Ctrl Pts',(-34.5027538123411,-55.8536509963143,
22.));
#46674=CARTESIAN_POINT('Ctrl Pts',(-34.4942777735197,-55.7968820122819,
22.));
#46675=CARTESIAN_POINT('Ctrl Pts',(-34.4923107028765,-55.783707390942,22.));
#46676=CARTESIAN_POINT('Ctrl Pts',(-34.4902017904221,-55.7705518962168,
22.));
#46677=CARTESIAN_POINT('Ctrl Pts',(-34.4879524958972,-55.7574168944054,
22.));
#46678=CARTESIAN_POINT('Ctrl Pts',(-31.6674621971265,-54.8470528177236,
20.8714803633902));
#46679=CARTESIAN_POINT('Ctrl Pts',(-31.7409214521311,-54.8037964055072,
20.8771939403667));
#46680=CARTESIAN_POINT('Ctrl Pts',(-31.8176439327865,-54.7663977740573,
20.8829075173431));
#46681=CARTESIAN_POINT('Ctrl Pts',(-31.896948563991,-54.7356618022518,20.8886210943196));
#46682=CARTESIAN_POINT('Ctrl Pts',(-32.4111477227468,-54.5363744390058,
20.9256670578423));
#46683=CARTESIAN_POINT('Ctrl Pts',(-33.0339012195891,-54.617187168241,20.962713021365));
#46684=CARTESIAN_POINT('Ctrl Pts',(-33.4802097929969,-54.9411120943331,
20.9997589848876));
#46685=CARTESIAN_POINT('Ctrl Pts',(-33.9265183664048,-55.2650370204253,
21.0368049484103));
#46686=CARTESIAN_POINT('Ctrl Pts',(-34.1963820163781,-55.8320741433745,
21.073850911933));
#46687=CARTESIAN_POINT('Ctrl Pts',(-34.1662812854629,-56.3827226982285,
21.1108968754557));
#46688=CARTESIAN_POINT('Ctrl Pts',(-34.1361805545477,-56.9333712530824,
21.1479428389784));
#46689=CARTESIAN_POINT('Ctrl Pts',(-33.806115442744,-57.4676312398412,21.184988802501));
#46690=CARTESIAN_POINT('Ctrl Pts',(-33.3271718011211,-57.740981554722,21.2220347660237));
#46691=CARTESIAN_POINT('Ctrl Pts',(-32.8482281594982,-58.0143318696029,
21.2590807295464));
#46692=CARTESIAN_POINT('Ctrl Pts',(-32.2204059880561,-58.0267725126059,
21.2961266930691));
#46693=CARTESIAN_POINT('Ctrl Pts',(-31.7309722501511,-57.772637960197,21.3331726565918));
#46694=CARTESIAN_POINT('Ctrl Pts',(-31.2415385122461,-57.5185034077881,
21.3702186201144));
#46695=CARTESIAN_POINT('Ctrl Pts',(-30.8904932078782,-56.9977936599673,
21.4072645836371));
#46696=CARTESIAN_POINT('Ctrl Pts',(-30.8386131457201,-56.4487584155402,
21.4443105471598));
#46697=CARTESIAN_POINT('Ctrl Pts',(-30.786733083562,-55.8997231711131,21.4813565106825));
#46698=CARTESIAN_POINT('Ctrl Pts',(-31.0340182636138,-55.3223624300798,
21.5184024742052));
#46699=CARTESIAN_POINT('Ctrl Pts',(-31.4670590682002,-54.9810209428387,
21.5554484377278));
#46700=CARTESIAN_POINT('Ctrl Pts',(-31.5295263145409,-54.9317815581341,
21.5607924129486));
#46701=CARTESIAN_POINT('Ctrl Pts',(-31.5958589129293,-54.8874534513961,
21.5661363881694));
#46702=CARTESIAN_POINT('Ctrl Pts',(-31.6652082225275,-54.8481806306043,
21.5714803633902));
#46703=CARTESIAN_POINT('Ctrl Pts',(-33.9541262883781,-54.8399232067375,
22.));
#46704=CARTESIAN_POINT('Ctrl Pts',(-33.4713921772736,-54.3563916207415,
21.9629540364773));
#46705=CARTESIAN_POINT('Ctrl Pts',(-31.9935412717563,-53.9174716604954,
21.888862109432));
#46706=CARTESIAN_POINT('Ctrl Pts',(-30.2271943832587,-55.4316007569426,
21.7777242188639));
#46707=CARTESIAN_POINT('Ctrl Pts',(-30.5464763025826,-57.7337498950934,
21.6665863282958));
#46708=CARTESIAN_POINT('Ctrl Pts',(-32.6512600365403,-58.7155097146097,
21.5554484377279));
#46709=CARTESIAN_POINT('Ctrl Pts',(-34.6188774786828,-57.4788960204646,
21.4443105471598));
#46710=CARTESIAN_POINT('Ctrl Pts',(-34.6464212862449,-55.1554778495401,
21.3331726565917));
#46711=CARTESIAN_POINT('Ctrl Pts',(-32.7096416422032,-53.872064985086,21.2220347660237));
#46712=CARTESIAN_POINT('Ctrl Pts',(-30.5808145803544,-54.8033004251176,
21.1108968754557));
#46713=CARTESIAN_POINT('Ctrl Pts',(-30.2087196709518,-57.0968534624393,
20.9997589848876));
#46714=CARTESIAN_POINT('Ctrl Pts',(-31.9338196700205,-58.6533891775714,
20.8886210943196));
#46715=CARTESIAN_POINT('Ctrl Pts',(-34.1771709144469,-58.0482026788782,
20.7774832037515));
#46716=CARTESIAN_POINT('Ctrl Pts',(-34.8853786224564,-55.8352230845946,
20.6663453131835));
#46717=CARTESIAN_POINT('Ctrl Pts',(-33.4102272112105,-54.0400181863803,
20.5552074226154));
#46718=CARTESIAN_POINT('Ctrl Pts',(-31.1019320194545,-54.3057581512874,
20.4440695320474));
#46719=CARTESIAN_POINT('Ctrl Pts',(-30.073305550394,-56.3892087930031,20.3329316414794));
#46720=CARTESIAN_POINT('Ctrl Pts',(-31.2658594095642,-58.3833638027876,
20.2217937509113));
#46721=CARTESIAN_POINT('Ctrl Pts',(-33.588036458114,-58.4629506390538,20.1106558603433));
#46722=CARTESIAN_POINT('Ctrl Pts',(-34.914321242052,-56.5551224909764,19.9995179697752));
#46723=CARTESIAN_POINT('Ctrl Pts',(-34.0307504904903,-54.406136137217,19.8883800792072));
#46724=CARTESIAN_POINT('Ctrl Pts',(-31.7460664163079,-53.9829831393046,
19.7772421886392));
#46725=CARTESIAN_POINT('Ctrl Pts',(-30.151466320847,-55.6729802447186,19.6661042980711));
#46726=CARTESIAN_POINT('Ctrl Pts',(-30.7065057264145,-57.9292539322017,
19.5549664075031));
#46727=CARTESIAN_POINT('Ctrl Pts',(-32.9031507850421,-58.6866113101154,
19.443828516935));
#46728=CARTESIAN_POINT('Ctrl Pts',(-34.730787355662,-57.2518345802401,19.332690626367));
#46729=CARTESIAN_POINT('Ctrl Pts',(-34.5165589620033,-54.9381911555042,
19.2215527357989));
#46730=CARTESIAN_POINT('Ctrl Pts',(-32.4565512804853,-53.8633851007702,
19.1104148452309));
#46731=CARTESIAN_POINT('Ctrl Pts',(-30.4363127049828,-55.0111985872155,
18.9992769546629));
#46732=CARTESIAN_POINT('Ctrl Pts',(-30.3049905142645,-57.3310249135316,
18.8881390640948));
#46733=CARTESIAN_POINT('Ctrl Pts',(-32.182785399016,-58.6995007346588,18.7770011735268));
#46734=CARTESIAN_POINT('Ctrl Pts',(-34.3509304054687,-57.8640446119295,
18.6658632829587));
#46735=CARTESIAN_POINT('Ctrl Pts',(-34.8248978208363,-55.5893590092039,
18.5547253923907));
#46736=CARTESIAN_POINT('Ctrl Pts',(-33.1708598946485,-53.9574894553413,
18.4435875018226));
#46737=CARTESIAN_POINT('Ctrl Pts',(-30.902776298825,-54.462104659654,18.3324496112546));
#46738=CARTESIAN_POINT('Ctrl Pts',(-30.0966496704334,-56.6413246029078,
18.2213117206866));
#46739=CARTESIAN_POINT('Ctrl Pts',(-31.4903368545418,-58.5004845570078,
18.1101738301185));
#46740=CARTESIAN_POINT('Ctrl Pts',(-33.8081801660464,-58.3378743316584,
17.9990359395505));
#46741=CARTESIAN_POINT('Ctrl Pts',(-34.928631335797,-56.3023329102471,17.8878980489824));
#46742=CARTESIAN_POINT('Ctrl Pts',(-33.8261287013397,-54.2570144404017,
17.7767601584144));
#46743=CARTESIAN_POINT('Ctrl Pts',(-31.5098054272241,-54.0740221130605,
17.6656222678464));
#46744=CARTESIAN_POINT('Ctrl Pts',(-30.0998184751404,-55.9208508807133,
17.5544843772783));
#46745=CARTESIAN_POINT('Ctrl Pts',(-30.8867448926705,-58.1070774278645,
17.4433464867103));
#46746=CARTESIAN_POINT('Ctrl Pts',(-33.1503020054966,-58.6316238024116,
17.3322085961423));
#46747=CARTESIAN_POINT('Ctrl Pts',(-34.8186303177654,-57.0143667589707,
17.2210707055742));
#46748=CARTESIAN_POINT('Ctrl Pts',(-34.3646900051272,-54.7356000103461,
17.1099328150062));
#46749=CARTESIAN_POINT('Ctrl Pts',(-32.2039777837733,-53.881104604526,16.9987949244381));
#46750=CARTESIAN_POINT('Ctrl Pts',(-30.3142180540518,-55.2330098770949,
16.8876570338701));
#46751=CARTESIAN_POINT('Ctrl Pts',(-30.4251293279102,-57.5539016004218,
16.776519143302));
#46752=CARTESIAN_POINT('Ctrl Pts',(-32.4351932585659,-58.7194412594432,
16.665381252734));
#46753=CARTESIAN_POINT('Ctrl Pts',(-34.5045755346153,-57.6627971861383,
16.554243362166));
#46754=CARTESIAN_POINT('Ctrl Pts',(-34.7391470903974,-55.3511276839614,
16.4431054715979));
#46755=CARTESIAN_POINT('Ctrl Pts',(-32.924201920686,-53.9003300643712,16.3319675810299));
#46756=CARTESIAN_POINT('Ctrl Pts',(-30.7209799221891,-54.6383358417407,
16.2208296904618));
#46757=CARTESIAN_POINT('Ctrl Pts',(-30.1461151763816,-56.8896399584928,
16.1096917998938));
#46758=CARTESIAN_POINT('Ctrl Pts',(-31.7257879044833,-58.5935982250311,
15.9985539093258));
#46759=CARTESIAN_POINT('Ctrl Pts',(-34.0141057438103,-58.1905583158083,
15.8874160187577));
#46760=CARTESIAN_POINT('Ctrl Pts',(-34.9165454246277,-56.0494272304867,
15.7762781281897));
#46761=CARTESIAN_POINT('Ctrl Pts',(-33.6070936729406,-54.130006533605,15.6651402376216));
#46762=CARTESIAN_POINT('Ctrl Pts',(-31.284306526822,-54.1891637565984,15.5540023470536));
#46763=CARTESIAN_POINT('Ctrl Pts',(-30.074257404191,-56.1727516226364,15.4428644564856));
#46764=CARTESIAN_POINT('Ctrl Pts',(-31.0845179881232,-58.2651696619898,
15.3317265659175));
#46765=CARTESIAN_POINT('Ctrl Pts',(-33.3903853125313,-58.551203914661,15.2205886753495));
#46766=CARTESIAN_POINT('Ctrl Pts',(-34.8812728580259,-56.7690439832156,
15.1094507847814));
#46767=CARTESIAN_POINT('Ctrl Pts',(-34.192554360499,-54.5499210682071,14.9983128942134));
#46768=CARTESIAN_POINT('Ctrl Pts',(-31.9546216431227,-53.9250235318367,
14.8871750036453));
#46769=CARTESIAN_POINT('Ctrl Pts',(-30.2158799584562,-55.4663271929179,
14.7760371130773));
#46770=CARTESIAN_POINT('Ctrl Pts',(-30.5678191761536,-57.7630592969624,
14.6648992225092));
#46771=CARTESIAN_POINT('Ctrl Pts',(-32.6883055651204,-58.7129949703236,
14.5537613319412));
#46772=CARTESIAN_POINT('Ctrl Pts',(-34.6364334330514,-57.4466471822883,
14.4426234413732));
#46773=CARTESIAN_POINT('Ctrl Pts',(-34.6290601547835,-55.1231186965397,
14.3314855508051));
#46774=CARTESIAN_POINT('Ctrl Pts',(-32.6729327631563,-53.8691609424836,
14.2203476602371));
#46775=CARTESIAN_POINT('Ctrl Pts',(-30.5585204707244,-54.8325367623412,
14.109209769669));
#46776=CARTESIAN_POINT('Ctrl Pts',(-30.2211615693062,-57.1314551632494,
13.998071879101));
#46777=CARTESIAN_POINT('Ctrl Pts',(-31.9696590133091,-58.6616944230991,
13.886933988533));
#46778=CARTESIAN_POINT('Ctrl Pts',(-34.2035641928434,-58.0226004643432,
13.7757960979649));
#46779=CARTESIAN_POINT('Ctrl Pts',(-34.8782165391171,-55.7991607039093,
13.6646582073969));
#46780=CARTESIAN_POINT('Ctrl Pts',(-33.3759826838065,-54.0264798110273,
13.5535203168288));
#46781=CARTESIAN_POINT('Ctrl Pts',(-31.072107305341,-54.3271826722053,13.4423824262608));
#46782=CARTESIAN_POINT('Ctrl Pts',(-30.074887383932,-56.4258925346357,13.3312445356927));
#46783=CARTESIAN_POINT('Ctrl Pts',(-31.2980228170538,-58.4019167094403,
13.2201066451247));
#46784=CARTESIAN_POINT('Ctrl Pts',(-33.6200956257376,-58.4460163820148,
13.1089687545567));
#46785=CARTESIAN_POINT('Ctrl Pts',(-34.9194345180072,-56.5189590291237,
12.9978308639886));
#46786=CARTESIAN_POINT('Ctrl Pts',(-33.9991195898381,-54.3822352088321,
12.8866929734206));
#46787=CARTESIAN_POINT('Ctrl Pts',(-32.4788453194858,-54.1263833506296,
12.8126010463752));
#46788=CARTESIAN_POINT('Ctrl Pts',(-31.8326342444893,-54.3482983416318,
12.7755550828525));
#46789=CARTESIAN_POINT('Ctrl Pts',(-33.8624214427591,-54.931476806163,22.0748149723825));
#46790=CARTESIAN_POINT('Ctrl Pts',(-33.4101310816148,-54.4784392630848,
22.0377690088598));
#46791=CARTESIAN_POINT('Ctrl Pts',(-32.0254812207533,-54.0671999021891,
21.9636770818144));
#46792=CARTESIAN_POINT('Ctrl Pts',(-30.3705294497321,-55.4858400606076,
21.8525391912464));
#46793=CARTESIAN_POINT('Ctrl Pts',(-30.6696757733002,-57.6428035756158,
21.7414013006784));
#46794=CARTESIAN_POINT('Ctrl Pts',(-32.6417207837188,-58.5626484614684,
21.6302634101103));
#46795=CARTESIAN_POINT('Ctrl Pts',(-34.4852499295344,-57.4040221256554,
21.5191255195423));
#46796=CARTESIAN_POINT('Ctrl Pts',(-34.5110566798406,-55.2271309148553,
21.4079876289742));
#46797=CARTESIAN_POINT('Ctrl Pts',(-32.6964205385156,-54.0246568103569,
21.2968497384062));
#46798=CARTESIAN_POINT('Ctrl Pts',(-30.7018484988176,-54.8971636496159,
21.1857118478381));
#46799=CARTESIAN_POINT('Ctrl Pts',(-30.3532198498734,-57.0460731790885,
21.0745739572701));
#46800=CARTESIAN_POINT('Ctrl Pts',(-31.969525977078,-58.5044455719578,20.9634360667021));
#46801=CARTESIAN_POINT('Ctrl Pts',(-34.071399702541,-57.9374253143107,20.852298176134));
#46802=CARTESIAN_POINT('Ctrl Pts',(-34.7349441106375,-55.8640078431203,
20.741160285566));
#46803=CARTESIAN_POINT('Ctrl Pts',(-33.352823499752,-54.1820180001326,20.6300223949979));
#46804=CARTESIAN_POINT('Ctrl Pts',(-31.1901015335783,-54.4309990063087,
20.5188845044299));
#46805=CARTESIAN_POINT('Ctrl Pts',(-30.2263456554001,-56.3830563013939,
20.4077466138619));
#46806=CARTESIAN_POINT('Ctrl Pts',(-31.3436908009795,-58.2514494163732,
20.2966087232938));
#46807=CARTESIAN_POINT('Ctrl Pts',(-33.5194191611043,-58.3260170884913,
20.1854708327258));
#46808=CARTESIAN_POINT('Ctrl Pts',(-34.7620614565392,-56.5385066096463,
20.0743329421577));
#46809=CARTESIAN_POINT('Ctrl Pts',(-33.9342133200027,-54.5250466289289,
19.9631950515897));
#46810=CARTESIAN_POINT('Ctrl Pts',(-31.7936134302447,-54.1285798828619,
19.8520571610216));
#46811=CARTESIAN_POINT('Ctrl Pts',(-30.2995771969099,-55.7119968893621,
19.7409192704536));
#46812=CARTESIAN_POINT('Ctrl Pts',(-30.8196129006622,-57.8259781007111,
19.6297813798856));
#46813=CARTESIAN_POINT('Ctrl Pts',(-32.8777259778579,-58.5355725422314,
19.5186434893175));
#46814=CARTESIAN_POINT('Ctrl Pts',(-34.590102181551,-57.1912803731281,19.4075055987495));
#46815=CARTESIAN_POINT('Ctrl Pts',(-34.3893841562315,-55.0235474616527,
19.2963677081814));
#46816=CARTESIAN_POINT('Ctrl Pts',(-32.4592913850741,-54.0165243251615,
19.1852298176134));
#46817=CARTESIAN_POINT('Ctrl Pts',(-30.5664596711081,-55.0919506610441,
19.0740919270453));
#46818=CARTESIAN_POINT('Ctrl Pts',(-30.4434193478744,-57.265476547833,18.9629540364773));
#46819=CARTESIAN_POINT('Ctrl Pts',(-32.2027906188128,-58.5476490919252,
18.8518161459092));
#46820=CARTESIAN_POINT('Ctrl Pts',(-34.2342010069002,-57.76488122287,18.7406782553412));
#46821=CARTESIAN_POINT('Ctrl Pts',(-34.6782775462125,-55.6336492484138,
18.6295403647732));
#46822=CARTESIAN_POINT('Ctrl Pts',(-33.1285519441201,-54.1046939645864,
18.5184024742052));
#46823=CARTESIAN_POINT('Ctrl Pts',(-31.0035056193152,-54.5774854822095,
18.4072645836371));
#46824=CARTESIAN_POINT('Ctrl Pts',(-30.2482175725494,-56.6192723633811,
18.2961266930691));
#46825=CARTESIAN_POINT('Ctrl Pts',(-31.5540115185799,-58.3611839203272,
18.184988802501));
#46826=CARTESIAN_POINT('Ctrl Pts',(-33.7256794498927,-58.2088287503542,
18.073850911933));
#46827=CARTESIAN_POINT('Ctrl Pts',(-34.7754690805687,-56.3016592683636,
17.9627130213649));
#46828=CARTESIAN_POINT('Ctrl Pts',(-33.7424960562255,-54.3853293299944,
17.8515751307969));
#46829=CARTESIAN_POINT('Ctrl Pts',(-31.5722523007556,-54.2138774604954,
17.7404372402288));
#46830=CARTESIAN_POINT('Ctrl Pts',(-30.2511865357786,-55.9442355004157,
17.6292993496608));
#46831=CARTESIAN_POINT('Ctrl Pts',(-30.9884852378828,-57.9925871122213,
17.5181614590928));
#46832=CARTESIAN_POINT('Ctrl Pts',(-33.1092905434961,-58.4840528357392,
17.4070235685247));
#46833=CARTESIAN_POINT('Ctrl Pts',(-34.6724053048228,-56.9687885206333,
17.2958856779567));
#46834=CARTESIAN_POINT('Ctrl Pts',(-34.2470928538933,-54.833732778786,17.1847477873887));
#46835=CARTESIAN_POINT('Ctrl Pts',(-32.2226465004149,-54.0331263438891,
17.0736098968206));
#46836=CARTESIAN_POINT('Ctrl Pts',(-30.4520649505092,-55.2997733652982,
16.9624720062526));
#46837=CARTESIAN_POINT('Ctrl Pts',(-30.5559815765657,-57.4742974595634,
16.8513341156845));
#46838=CARTESIAN_POINT('Ctrl Pts',(-32.4392803122598,-58.5663320624232,
16.7401962251165));
#46839=CARTESIAN_POINT('Ctrl Pts',(-34.3781564667511,-57.5763255173654,
16.6290583345484));
#46840=CARTESIAN_POINT('Ctrl Pts',(-34.5979347074811,-55.4104420425189,
16.5179204439804));
#46841=CARTESIAN_POINT('Ctrl Pts',(-32.897449518258,-54.0511393452008,16.4067825534124));
#46842=CARTESIAN_POINT('Ctrl Pts',(-30.833174277585,-54.7426025998055,16.2956446628443));
#46843=CARTESIAN_POINT('Ctrl Pts',(-30.2945635237364,-56.8519276476706,
16.1845067722763));
#46844=CARTESIAN_POINT('Ctrl Pts',(-31.7746137879455,-58.4484253511043,
16.0733688817082));
#46845=CARTESIAN_POINT('Ctrl Pts',(-33.9186182785215,-58.0708032566539,
15.9622309911402));
#46846=CARTESIAN_POINT('Ctrl Pts',(-34.7641453704728,-56.0647031498647,
15.8510931005721));
#46847=CARTESIAN_POINT('Ctrl Pts',(-33.5372745278125,-54.2663312092653,
15.7399552100041));
#46848=CARTESIAN_POINT('Ctrl Pts',(-31.3609745460779,-54.3217576668876,
15.6288173194361));
#46849=CARTESIAN_POINT('Ctrl Pts',(-30.2272374802945,-56.1802500577385,
15.517679428868));
#46850=CARTESIAN_POINT('Ctrl Pts',(-31.1737857225787,-58.14070921924,15.4065415383));
#46851=CARTESIAN_POINT('Ctrl Pts',(-33.3342329354787,-58.4087046487411,
15.2954036477319));
#46852=CARTESIAN_POINT('Ctrl Pts',(-34.731097277289,-56.7389370883627,15.1842657571639));
#46853=CARTESIAN_POINT('Ctrl Pts',(-34.0858129876404,-54.6597637265374,
15.0731278665959));
#46854=CARTESIAN_POINT('Ctrl Pts',(-31.9890160684358,-54.0742755128362,
14.9619899760278));
#46855=CARTESIAN_POINT('Ctrl Pts',(-30.3599285720183,-55.5183764650323,
14.8508520854598));
#46856=CARTESIAN_POINT('Ctrl Pts',(-30.6896726531006,-57.6702645725732,
14.7397141948917));
#46857=CARTESIAN_POINT('Ctrl Pts',(-32.6764300265812,-58.5602923101727,
14.6285763043237));
#46858=CARTESIAN_POINT('Ctrl Pts',(-34.5016987131586,-57.373807068692,14.5174384137556));
#46859=CARTESIAN_POINT('Ctrl Pts',(-34.4947904325672,-55.1968125001003,
14.4063005231876));
#46860=CARTESIAN_POINT('Ctrl Pts',(-32.6620267142976,-54.0219359119425,
14.2951626326196));
#46861=CARTESIAN_POINT('Ctrl Pts',(-30.6809603729033,-54.9245561897684,
14.1840247420515));
#46862=CARTESIAN_POINT('Ctrl Pts',(-30.3648770967317,-57.0784927148031,
14.0728868514835));
#46863=CARTESIAN_POINT('Ctrl Pts',(-32.0031051030323,-58.5122270450561,
13.9617489609154));
#46864=CARTESIAN_POINT('Ctrl Pts',(-34.0961284820971,-57.9134377099716,
13.8506110703474));
#46865=CARTESIAN_POINT('Ctrl Pts',(-34.7282337059125,-55.8302197456797,
13.7394731797794));
#46866=CARTESIAN_POINT('Ctrl Pts',(-33.3207386122115,-54.1693334258776,
13.6283352892113));
#46867=CARTESIAN_POINT('Ctrl Pts',(-31.1621577226746,-54.4510723843451,
13.5171973986433));
#46868=CARTESIAN_POINT('Ctrl Pts',(-30.2278277302023,-56.417426573495,13.4060595080752));
#46869=CARTESIAN_POINT('Ctrl Pts',(-31.3738258149644,-58.2688322792311,
13.2949216175072));
#46870=CARTESIAN_POINT('Ctrl Pts',(-33.549456509137,-58.3101507946959,13.1837837269392));
#46871=CARTESIAN_POINT('Ctrl Pts',(-34.7668522624408,-56.5046238057481,
13.0726458363711));
#46872=CARTESIAN_POINT('Ctrl Pts',(-33.9045772301756,-54.5026530186945,
12.9615079458031));
#46873=CARTESIAN_POINT('Ctrl Pts',(-32.4801794448133,-54.2629365232493,
12.8874160187577));
#46874=CARTESIAN_POINT('Ctrl Pts',(-31.8747218362409,-54.4708563886884,
12.850370055235));
#46875=CARTESIAN_POINT('Ctrl Pts',(-33.7707165971401,-55.0230304055885,
22.149629944765));
#46876=CARTESIAN_POINT('Ctrl Pts',(-33.3488699859559,-54.6004869054281,
22.1125839812423));
#46877=CARTESIAN_POINT('Ctrl Pts',(-32.0574211697503,-54.2169281438828,
22.0384920541969));
#46878=CARTESIAN_POINT('Ctrl Pts',(-30.5138645162054,-55.5400793642724,
21.9273541636289));
#46879=CARTESIAN_POINT('Ctrl Pts',(-30.7928752440178,-57.5518572561383,
21.8162162730608));
#46880=CARTESIAN_POINT('Ctrl Pts',(-32.6321815308973,-58.409787208327,21.7050783824928));
#46881=CARTESIAN_POINT('Ctrl Pts',(-34.351622380386,-57.3291482308462,21.5939404919248));
#46882=CARTESIAN_POINT('Ctrl Pts',(-34.3756920734364,-55.2987839801705,
21.4828026013567));
#46883=CARTESIAN_POINT('Ctrl Pts',(-32.6831994348279,-54.1772486356277,
21.3716647107887));
#46884=CARTESIAN_POINT('Ctrl Pts',(-30.822882417281,-54.9910268741142,21.2605268202207));
#46885=CARTESIAN_POINT('Ctrl Pts',(-30.497720028795,-56.9952928957376,21.1493889296526));
#46886=CARTESIAN_POINT('Ctrl Pts',(-32.0052322841356,-58.3555019663444,
21.0382510390845));
#46887=CARTESIAN_POINT('Ctrl Pts',(-33.965628490635,-57.8266479497429,20.9271131485165));
#46888=CARTESIAN_POINT('Ctrl Pts',(-34.5845095988185,-55.8927926016459,
20.8159752579485));
#46889=CARTESIAN_POINT('Ctrl Pts',(-33.2954197882935,-54.3240178138849,
20.7048373673804));
#46890=CARTESIAN_POINT('Ctrl Pts',(-31.278271047702,-54.55623986133,20.5936994768124));
#46891=CARTESIAN_POINT('Ctrl Pts',(-30.3793857604063,-56.3769038097847,
20.4825615862443));
#46892=CARTESIAN_POINT('Ctrl Pts',(-31.4215221923948,-58.1195350299587,
20.3714236956763));
#46893=CARTESIAN_POINT('Ctrl Pts',(-33.4508018640946,-58.1890835379289,
20.2602858051083));
#46894=CARTESIAN_POINT('Ctrl Pts',(-34.6098016710263,-56.5218907283162,
20.1491479145402));
#46895=CARTESIAN_POINT('Ctrl Pts',(-33.8376761495152,-54.6439571206407,
20.0380100239722));
#46896=CARTESIAN_POINT('Ctrl Pts',(-31.8411604441816,-54.2741766264193,
19.9268721334041));
#46897=CARTESIAN_POINT('Ctrl Pts',(-30.4476880729728,-55.7510135340056,
19.8157342428361));
#46898=CARTESIAN_POINT('Ctrl Pts',(-30.9327200749099,-57.7227022692206,
19.7045963522681));
#46899=CARTESIAN_POINT('Ctrl Pts',(-32.8523011706738,-58.3845337743473,
19.5934584617));
#46900=CARTESIAN_POINT('Ctrl Pts',(-34.44941700744,-57.1307261660161,19.482320571132));
#46901=CARTESIAN_POINT('Ctrl Pts',(-34.2622093504597,-55.1089037678011,
19.3711826805639));
#46902=CARTESIAN_POINT('Ctrl Pts',(-32.4620314896628,-54.1696635495527,
19.2600447899959));
#46903=CARTESIAN_POINT('Ctrl Pts',(-30.6966066372334,-55.1727027348726,
19.1489068994278));
#46904=CARTESIAN_POINT('Ctrl Pts',(-30.5818481814842,-57.1999281821345,
19.0377690088598));
#46905=CARTESIAN_POINT('Ctrl Pts',(-32.2227958386096,-58.3957974491916,
18.9266311182917));
#46906=CARTESIAN_POINT('Ctrl Pts',(-34.1174716083317,-57.6657178338107,
18.8154932277237));
#46907=CARTESIAN_POINT('Ctrl Pts',(-34.5316572715886,-55.6779394876238,
18.7043553371557));
#46908=CARTESIAN_POINT('Ctrl Pts',(-33.0862439935917,-54.2518984738315,
18.5932174465876));
#46909=CARTESIAN_POINT('Ctrl Pts',(-31.1042349398055,-54.692866304765,18.4820795560196));
#46910=CARTESIAN_POINT('Ctrl Pts',(-30.3997854746655,-56.5972201238544,
18.3709416654515));
#46911=CARTESIAN_POINT('Ctrl Pts',(-31.617686182618,-58.2218832836465,18.2598037748835));
#46912=CARTESIAN_POINT('Ctrl Pts',(-33.643178733739,-58.0797831690501,18.1486658843155));
#46913=CARTESIAN_POINT('Ctrl Pts',(-34.6223068253403,-56.3009856264801,
18.0375279937474));
#46914=CARTESIAN_POINT('Ctrl Pts',(-33.6588634111112,-54.5136442195871,
17.9263901031794));
#46915=CARTESIAN_POINT('Ctrl Pts',(-31.6346991742871,-54.3537328079304,
17.8152522126114));
#46916=CARTESIAN_POINT('Ctrl Pts',(-30.4025545964168,-55.9676201201181,
17.7041143220433));
#46917=CARTESIAN_POINT('Ctrl Pts',(-31.090225583095,-57.878096796578,17.5929764314753));
#46918=CARTESIAN_POINT('Ctrl Pts',(-33.0682790814956,-58.336481869067,17.4818385409072));
#46919=CARTESIAN_POINT('Ctrl Pts',(-34.5261802918802,-56.9232102822958,
17.3707006503392));
#46920=CARTESIAN_POINT('Ctrl Pts',(-34.1294957026595,-54.9318655472259,
17.2595627597711));
#46921=CARTESIAN_POINT('Ctrl Pts',(-32.2413152170565,-54.1851480832521,
17.1484248692031));
#46922=CARTESIAN_POINT('Ctrl Pts',(-30.5899118469666,-55.3665368535016,
17.037286978635));
#46923=CARTESIAN_POINT('Ctrl Pts',(-30.6868338252212,-57.3946933187052,
16.926149088067));
#46924=CARTESIAN_POINT('Ctrl Pts',(-32.4433673659537,-58.4132228654032,
16.815011197499));
#46925=CARTESIAN_POINT('Ctrl Pts',(-34.251737398887,-57.4898538485925,16.7038733069309));
#46926=CARTESIAN_POINT('Ctrl Pts',(-34.4567223245648,-55.4697564010764,
16.5927354163629));
#46927=CARTESIAN_POINT('Ctrl Pts',(-32.87069711583,-54.2019486260304,16.4815975257949));
#46928=CARTESIAN_POINT('Ctrl Pts',(-30.9453686329809,-54.8468693578704,
16.3704596352268));
#46929=CARTESIAN_POINT('Ctrl Pts',(-30.4430118710911,-56.8142153368483,
16.2593217446588));
#46930=CARTESIAN_POINT('Ctrl Pts',(-31.8234396714078,-58.3032524771776,
16.1481838540907));
#46931=CARTESIAN_POINT('Ctrl Pts',(-33.8231308132328,-57.9510481974995,
16.0370459635227));
#46932=CARTESIAN_POINT('Ctrl Pts',(-34.611745316318,-56.0799790692429,15.9259080729546));
#46933=CARTESIAN_POINT('Ctrl Pts',(-33.4674553826844,-54.4026558849256,
15.8147701823866));
#46934=CARTESIAN_POINT('Ctrl Pts',(-31.4376425653338,-54.4543515771769,
15.7036322918186));
#46935=CARTESIAN_POINT('Ctrl Pts',(-30.3802175563979,-56.1877484928405,
15.5924944012505));
#46936=CARTESIAN_POINT('Ctrl Pts',(-31.2630534570342,-58.0162487764902,
15.4813565106825));
#46937=CARTESIAN_POINT('Ctrl Pts',(-33.278080558426,-58.2662053828213,15.3702186201144));
#46938=CARTESIAN_POINT('Ctrl Pts',(-34.5809216965521,-56.7088301935098,
15.2590807295464));
#46939=CARTESIAN_POINT('Ctrl Pts',(-33.9790716147817,-54.7696063848677,
15.1479428389783));
#46940=CARTESIAN_POINT('Ctrl Pts',(-32.0234104937488,-54.2235274938358,
15.0368049484103));
#46941=CARTESIAN_POINT('Ctrl Pts',(-30.5039771855804,-55.5704257371467,
14.9256670578423));
#46942=CARTESIAN_POINT('Ctrl Pts',(-30.8115261300475,-57.577469848184,14.8145291672742));
#46943=CARTESIAN_POINT('Ctrl Pts',(-32.664554488042,-58.4075896500218,14.7033912767062));
#46944=CARTESIAN_POINT('Ctrl Pts',(-34.3669639932659,-57.3009669550956,
14.5922533861381));
#46945=CARTESIAN_POINT('Ctrl Pts',(-34.3605207103509,-55.2705063036608,
14.4811154955701));
#46946=CARTESIAN_POINT('Ctrl Pts',(-32.6511206654389,-54.1747108814015,
14.3699776050021));
#46947=CARTESIAN_POINT('Ctrl Pts',(-30.8034002750821,-55.0165756171955,
14.258839714434));
#46948=CARTESIAN_POINT('Ctrl Pts',(-30.5085926241571,-57.0255302663568,
14.147701823866));
#46949=CARTESIAN_POINT('Ctrl Pts',(-32.0365511927555,-58.3627596670131,
14.0365639332979));
#46950=CARTESIAN_POINT('Ctrl Pts',(-33.9886927713508,-57.8042749555999,
13.9254260427299));
#46951=CARTESIAN_POINT('Ctrl Pts',(-34.5782508727078,-55.8612787874501,
13.8142881521619));
#46952=CARTESIAN_POINT('Ctrl Pts',(-33.2654945406164,-54.3121870407279,
13.7031502615938));
#46953=CARTESIAN_POINT('Ctrl Pts',(-31.2522081400082,-54.574962096485,13.5920123710258));
#46954=CARTESIAN_POINT('Ctrl Pts',(-30.3807680764726,-56.4089606123543,
13.4808744804577));
#46955=CARTESIAN_POINT('Ctrl Pts',(-31.449628812875,-58.135747849022,13.3697365898897));
#46956=CARTESIAN_POINT('Ctrl Pts',(-33.4788173925363,-58.174285207377,13.2585986993216));
#46957=CARTESIAN_POINT('Ctrl Pts',(-34.6142700068744,-56.4902885823724,
13.1474608087536));
#46958=CARTESIAN_POINT('Ctrl Pts',(-33.8100348705132,-54.6230708285569,
13.0363229181856));
#46959=CARTESIAN_POINT('Ctrl Pts',(-32.4815135701408,-54.3994896958689,
12.9622309911402));
#46960=CARTESIAN_POINT('Ctrl Pts',(-31.9168094279925,-54.593414435745,12.9251850276175));
#46961=CARTESIAN_POINT('Ctrl Pts',(-33.6790117515211,-55.1145840050141,
22.2244449171475));
#46962=CARTESIAN_POINT('Ctrl Pts',(-33.2876088902971,-54.7225345477714,
22.1873989536248));
#46963=CARTESIAN_POINT('Ctrl Pts',(-32.0893611187473,-54.3666563855765,
22.1133070265794));
#46964=CARTESIAN_POINT('Ctrl Pts',(-30.6571995826787,-55.5943186679374,
22.0021691360114));
#46965=CARTESIAN_POINT('Ctrl Pts',(-30.9160747147354,-57.4609109366607,
21.8910312454433));
#46966=CARTESIAN_POINT('Ctrl Pts',(-32.6226422780758,-58.2569259551857,
21.7798933548753));
#46967=CARTESIAN_POINT('Ctrl Pts',(-34.2179948312376,-57.254274336037,21.6687554643072));
#46968=CARTESIAN_POINT('Ctrl Pts',(-34.2403274670321,-55.3704370454857,
21.5576175737392));
#46969=CARTESIAN_POINT('Ctrl Pts',(-32.6699783311403,-54.3298404608986,
21.4464796831712));
#46970=CARTESIAN_POINT('Ctrl Pts',(-30.9439163357442,-55.0848900986124,
21.3353417926032));
#46971=CARTESIAN_POINT('Ctrl Pts',(-30.6422202077166,-56.9445126123869,
21.2242039020351));
#46972=CARTESIAN_POINT('Ctrl Pts',(-32.0409385911932,-58.206558360731,21.1130660114671));
#46973=CARTESIAN_POINT('Ctrl Pts',(-33.8598572787291,-57.7158705851754,
21.001928120899));
#46974=CARTESIAN_POINT('Ctrl Pts',(-34.4340750869996,-55.9215773601716,
20.890790230331));
#46975=CARTESIAN_POINT('Ctrl Pts',(-33.238016076835,-54.4660176276372,20.7796523397629));
#46976=CARTESIAN_POINT('Ctrl Pts',(-31.3664405618257,-54.6814807163513,
20.6685144491949));
#46977=CARTESIAN_POINT('Ctrl Pts',(-30.5324258654125,-56.3707513181756,
20.5573765586268));
#46978=CARTESIAN_POINT('Ctrl Pts',(-31.4993535838102,-57.9876206435441,
20.4462386680588));
#46979=CARTESIAN_POINT('Ctrl Pts',(-33.3821845670849,-58.0521499873666,
20.3351007774907));
#46980=CARTESIAN_POINT('Ctrl Pts',(-34.4575418855134,-56.5052748469861,
20.2239628869227));
#46981=CARTESIAN_POINT('Ctrl Pts',(-33.7411389790275,-54.7628676123527,
20.1128249963547));
#46982=CARTESIAN_POINT('Ctrl Pts',(-31.8887074581185,-54.4197733699765,
20.0016871057866));
#46983=CARTESIAN_POINT('Ctrl Pts',(-30.5957989490357,-55.7900301786492,
19.8905492152186));
#46984=CARTESIAN_POINT('Ctrl Pts',(-31.0458272491576,-57.61942643773,19.7794113246506));
#46985=CARTESIAN_POINT('Ctrl Pts',(-32.8268763634896,-58.2334950064633,
19.6682734340825));
#46986=CARTESIAN_POINT('Ctrl Pts',(-34.308731833329,-57.070171958904,19.5571355435145));
#46987=CARTESIAN_POINT('Ctrl Pts',(-34.1350345446879,-55.1942600739497,
19.4459976529464));
#46988=CARTESIAN_POINT('Ctrl Pts',(-32.4647715942516,-54.3228027739439,
19.3348597623784));
#46989=CARTESIAN_POINT('Ctrl Pts',(-30.8267536033587,-55.2534548087013,
19.2237218718103));
#46990=CARTESIAN_POINT('Ctrl Pts',(-30.7202770150941,-57.1343798164359,
19.1125839812423));
#46991=CARTESIAN_POINT('Ctrl Pts',(-32.2428010584064,-58.243945806458,19.0014460906742));
#46992=CARTESIAN_POINT('Ctrl Pts',(-34.0007422097632,-57.5665544447512,
18.8903082001062));
#46993=CARTESIAN_POINT('Ctrl Pts',(-34.3850369969647,-55.7222297268337,
18.7791703095382));
#46994=CARTESIAN_POINT('Ctrl Pts',(-33.0439360430634,-54.3991029830766,
18.6680324189701));
#46995=CARTESIAN_POINT('Ctrl Pts',(-31.2049642602956,-54.8082471273205,
18.5568945284021));
#46996=CARTESIAN_POINT('Ctrl Pts',(-30.5513533767816,-56.5751678843276,
18.4457566378341));
#46997=CARTESIAN_POINT('Ctrl Pts',(-31.6813608466561,-58.082582646966,18.334618747266));
#46998=CARTESIAN_POINT('Ctrl Pts',(-33.5606780175853,-57.9507375877458,
18.223480856698));
#46999=CARTESIAN_POINT('Ctrl Pts',(-34.469144570112,-56.3003119845966,18.1123429661299));
#47000=CARTESIAN_POINT('Ctrl Pts',(-33.5752307659969,-54.6419591091798,
18.0012050755619));
#47001=CARTESIAN_POINT('Ctrl Pts',(-31.6971460478186,-54.4935881553653,
17.8900671849938));
#47002=CARTESIAN_POINT('Ctrl Pts',(-30.5539226570551,-55.9910047398205,
17.7789292944258));
#47003=CARTESIAN_POINT('Ctrl Pts',(-31.1919659283072,-57.7636064809347,
17.6677914038578));
#47004=CARTESIAN_POINT('Ctrl Pts',(-33.027267619495,-58.1889109023947,17.5566535132897));
#47005=CARTESIAN_POINT('Ctrl Pts',(-34.3799552789376,-56.8776320439583,
17.4455156227217));
#47006=CARTESIAN_POINT('Ctrl Pts',(-34.0118985514257,-55.0299983156659,
17.3343777321536));
#47007=CARTESIAN_POINT('Ctrl Pts',(-32.2599839336981,-54.3371698226151,
17.2232398415856));
#47008=CARTESIAN_POINT('Ctrl Pts',(-30.727758743424,-55.4333003417049,17.1121019510175));
#47009=CARTESIAN_POINT('Ctrl Pts',(-30.8176860738768,-57.3150891778468,
17.0009640604495));
#47010=CARTESIAN_POINT('Ctrl Pts',(-32.4474544196476,-58.2601136683832,
16.8898261698815));
#47011=CARTESIAN_POINT('Ctrl Pts',(-34.1253183310228,-57.4033821798196,
16.7786882793134));
#47012=CARTESIAN_POINT('Ctrl Pts',(-34.3155099416485,-55.5290707596339,
16.6675503887454));
#47013=CARTESIAN_POINT('Ctrl Pts',(-32.8439447134021,-54.3527579068599,
16.5564124981773));
#47014=CARTESIAN_POINT('Ctrl Pts',(-31.0575629883768,-54.9511361159353,
16.4452746076093));
#47015=CARTESIAN_POINT('Ctrl Pts',(-30.5914602184459,-56.776503026026,16.3341367170413));
#47016=CARTESIAN_POINT('Ctrl Pts',(-31.87226555487,-58.1580796032509,16.2229988264732));
#47017=CARTESIAN_POINT('Ctrl Pts',(-33.727643347944,-57.8312931383451,16.1118609359052));
#47018=CARTESIAN_POINT('Ctrl Pts',(-34.4593452621631,-56.0952549886209,
16.0007230453371));
#47019=CARTESIAN_POINT('Ctrl Pts',(-33.3976362375564,-54.5389805605859,
15.8895851547691));
#47020=CARTESIAN_POINT('Ctrl Pts',(-31.5143105845896,-54.5869454874661,
15.7784472642011));
#47021=CARTESIAN_POINT('Ctrl Pts',(-30.5331976325014,-56.1952469279427,
15.667309373633));
#47022=CARTESIAN_POINT('Ctrl Pts',(-31.3523211914896,-57.8917883337404,
15.556171483065));
#47023=CARTESIAN_POINT('Ctrl Pts',(-33.2219281813735,-58.1237061169015,
15.4450335924969));
#47024=CARTESIAN_POINT('Ctrl Pts',(-34.4307461158152,-56.6787232986569,
15.3338957019289));
#47025=CARTESIAN_POINT('Ctrl Pts',(-33.872330241923,-54.879449043198,15.2227578113608));
#47026=CARTESIAN_POINT('Ctrl Pts',(-32.057804919062,-54.3727794748353,15.1116199207928));
#47027=CARTESIAN_POINT('Ctrl Pts',(-30.6480257991425,-55.6224750092611,
15.0004820302248));
#47028=CARTESIAN_POINT('Ctrl Pts',(-30.9333796069945,-57.4846751237948,
14.8893441396567));
#47029=CARTESIAN_POINT('Ctrl Pts',(-32.6526789495027,-58.2548869898709,
14.7782062490887));
#47030=CARTESIAN_POINT('Ctrl Pts',(-34.2322292733731,-57.2281268414992,
14.6670683585206));
#47031=CARTESIAN_POINT('Ctrl Pts',(-34.2262509881345,-55.3442001072214,
14.5559304679526));
#47032=CARTESIAN_POINT('Ctrl Pts',(-32.6402146165803,-54.3274858508605,
14.4447925773845));
#47033=CARTESIAN_POINT('Ctrl Pts',(-30.9258401772609,-55.1085950446227,
14.3336546868165));
#47034=CARTESIAN_POINT('Ctrl Pts',(-30.6523081515825,-56.9725678179105,
14.2225167962485));
#47035=CARTESIAN_POINT('Ctrl Pts',(-32.0699972824786,-58.2132922889699,
14.1113789056804));
#47036=CARTESIAN_POINT('Ctrl Pts',(-33.8812570606045,-57.6951122012284,
14.0002410151124));
#47037=CARTESIAN_POINT('Ctrl Pts',(-34.4282680395032,-55.8923378292204,
13.8891031245443));
#47038=CARTESIAN_POINT('Ctrl Pts',(-33.2102504690214,-54.4550406555783,
13.7779652339763));
#47039=CARTESIAN_POINT('Ctrl Pts',(-31.3422585573418,-54.6988518086249,
13.6668273434082));
#47040=CARTESIAN_POINT('Ctrl Pts',(-30.5337084227428,-56.4004946512136,
13.5556894528402));
#47041=CARTESIAN_POINT('Ctrl Pts',(-31.5254318107855,-58.0026634188128,
13.4445515622722));
#47042=CARTESIAN_POINT('Ctrl Pts',(-33.4081782759357,-58.0384196200582,
13.3334136717041));
#47043=CARTESIAN_POINT('Ctrl Pts',(-34.4616877513079,-56.4759533589966,
13.2222757811361));
#47044=CARTESIAN_POINT('Ctrl Pts',(-33.7154925108507,-54.7434886384194,
13.111137890568));
#47045=CARTESIAN_POINT('Ctrl Pts',(-32.4828476954683,-54.5360428684886,
13.0370459635227));
#47046=CARTESIAN_POINT('Ctrl Pts',(-31.9588970197441,-54.7159724828016,
13.));
#47047=CARTESIAN_POINT('Ctrl Pts',(-31.667262219952,-54.851191363199,21.3785196366098));
#47048=CARTESIAN_POINT('Ctrl Pts',(-31.479741769716,-54.9581664087852,21.3641270219409));
#47049=CARTESIAN_POINT('Ctrl Pts',(-31.3126103376672,-55.0996825231223,
21.349734407272));
#47050=CARTESIAN_POINT('Ctrl Pts',(-31.1813106469723,-55.2689855779558,
21.3353417926031));
#47051=CARTESIAN_POINT('Ctrl Pts',(-30.843350959735,-55.7047642698706,21.2982958290804));
#47052=CARTESIAN_POINT('Ctrl Pts',(-30.7427855837258,-56.3246384411287,
21.2612498655577));
#47053=CARTESIAN_POINT('Ctrl Pts',(-30.9256226263006,-56.8449164848151,
21.2242039020351));
#47054=CARTESIAN_POINT('Ctrl Pts',(-31.1084596688754,-57.3651945285016,
21.1871579385124));
#47055=CARTESIAN_POINT('Ctrl Pts',(-31.5746991300343,-57.7858764446163,
21.1501119749897));
#47056=CARTESIAN_POINT('Ctrl Pts',(-32.1109719752031,-57.9144361067477,
21.113066011467));
#47057=CARTESIAN_POINT('Ctrl Pts',(-32.6472448203718,-58.0429957688791,
21.0760200479444));
#47058=CARTESIAN_POINT('Ctrl Pts',(-33.2535510495505,-57.8794331770273,
21.0389740844217));
#47059=CARTESIAN_POINT('Ctrl Pts',(-33.6524071321849,-57.4986030102674,
21.001928120899));
#47060=CARTESIAN_POINT('Ctrl Pts',(-34.0512632148193,-57.1177728435075,
20.9648821573763));
#47061=CARTESIAN_POINT('Ctrl Pts',(-34.2426691509094,-56.5196751018395,
20.9278361938536));
#47062=CARTESIAN_POINT('Ctrl Pts',(-34.1390289505938,-55.9780329422498,
20.890790230331));
#47063=CARTESIAN_POINT('Ctrl Pts',(-34.0353887502781,-55.4363907826601,
20.8537442668083));
#47064=CARTESIAN_POINT('Ctrl Pts',(-33.6367024135565,-54.9512042051487,
20.8166983032856));
#47065=CARTESIAN_POINT('Ctrl Pts',(-33.1254299926942,-54.7445214311786,
20.7796523397629));
#47066=CARTESIAN_POINT('Ctrl Pts',(-32.6601848660756,-54.5564452717343,
20.7459414387119));
#47067=CARTESIAN_POINT('Ctrl Pts',(-32.1017123235945,-54.5989854456511,
20.7122305376608));
#47068=CARTESIAN_POINT('Ctrl Pts',(-31.6651488727497,-54.8473747039335,
20.6785196366098));
#47069=CARTESIAN_POINT('Ctrl Pts',(-33.9541262883781,-54.8399232067375,
22.));
#47070=CARTESIAN_POINT('Ctrl Pts',(-33.8977770566593,-54.7931706099728,
22.));
#47071=CARTESIAN_POINT('Ctrl Pts',(-33.8389107618331,-54.7498380989966,
22.));
#47072=CARTESIAN_POINT('Ctrl Pts',(-33.777876546057,-54.7099422292584,22.));
#47073=CARTESIAN_POINT('Ctrl Pts',(-33.7151426127656,-54.668935315367,22.));
#47074=CARTESIAN_POINT('Ctrl Pts',(-33.6501173479606,-54.6315587953762,
22.));
#47075=CARTESIAN_POINT('Ctrl Pts',(-33.583156824249,-54.5978800039319,22.));
#47076=CARTESIAN_POINT('Ctrl Pts',(-33.5265763653144,-54.5694220204714,
22.));
#47077=CARTESIAN_POINT('Ctrl Pts',(-33.4686133977519,-54.5436050119993,
22.));
#47078=CARTESIAN_POINT('Ctrl Pts',(-33.4094785141786,-54.5204983074657,
22.));
#47079=CARTESIAN_POINT('Ctrl Pts',(-33.3832054797332,-54.5102322308718,
22.));
#47080=CARTESIAN_POINT('Ctrl Pts',(-33.3567011132793,-54.5005015028802,
22.));
#47081=CARTESIAN_POINT('Ctrl Pts',(-33.3299840335547,-54.4913139103878,
22.));
#47082=CARTESIAN_POINT('Ctrl Pts',(-33.3153052179459,-54.4862660916338,
22.));
#47083=CARTESIAN_POINT('Ctrl Pts',(-33.3005621960494,-54.4813822417943,
22.));
#47084=CARTESIAN_POINT('Ctrl Pts',(-33.2857580867463,-54.4766637893077,
22.));
#47085=CARTESIAN_POINT('Ctrl Pts',(-33.2721048859179,-54.4723121611158,
22.));
#47086=CARTESIAN_POINT('Ctrl Pts',(-33.2583976935737,-54.4681007280233,
22.));
#47087=CARTESIAN_POINT('Ctrl Pts',(-33.2446602943265,-54.4640366443481,
22.));
#47088=CARTESIAN_POINT('Ctrl Pts',(-33.1744615987436,-54.4432690035735,
22.));
#47089=CARTESIAN_POINT('Ctrl Pts',(-33.1033546243453,-54.426305105702,22.));
#47090=CARTESIAN_POINT('Ctrl Pts',(-33.0316734669904,-54.4132045353859,
22.));
#47091=CARTESIAN_POINT('Ctrl Pts',(-32.9605481884919,-54.4002055584357,
22.));
#47092=CARTESIAN_POINT('Ctrl Pts',(-32.8888565785783,-54.3910102235869,
22.));
#47093=CARTESIAN_POINT('Ctrl Pts',(-32.8169264247812,-54.3857276509517,
22.));
#47094=CARTESIAN_POINT('Ctrl Pts',(-32.7571464346349,-54.3813373900748,
22.));
#47095=CARTESIAN_POINT('Ctrl Pts',(-32.6972014393858,-54.3796505588111,
22.));
#47096=CARTESIAN_POINT('Ctrl Pts',(-32.6372877974345,-54.3807569468889,
22.));
#47097=CARTESIAN_POINT('Ctrl Pts',(-32.6122799917819,-54.3812187505304,
22.));
#47098=CARTESIAN_POINT('Ctrl Pts',(-32.58727777557,-54.3821674889407,22.));
#47099=CARTESIAN_POINT('Ctrl Pts',(-32.5622960765744,-54.3836109807411,
22.));
#47100=CARTESIAN_POINT('Ctrl Pts',(-32.5507331511287,-54.3842791093608,
22.));
#47101=CARTESIAN_POINT('Ctrl Pts',(-32.5391746274407,-54.3850532424534,
22.));
#47102=CARTESIAN_POINT('Ctrl Pts',(-32.5276220201243,-54.3859342108708,
22.));
#47103=CARTESIAN_POINT('Ctrl Pts',(-32.5155719563499,-54.3868531138787,
22.));
#47104=CARTESIAN_POINT('Ctrl Pts',(-32.5035366028335,-54.387887649022,22.));
#47105=CARTESIAN_POINT('Ctrl Pts',(-32.4915220458793,-54.3890378132804,
22.));
#47106=CARTESIAN_POINT('Ctrl Pts',(-32.4230954842274,-54.3955883490877,
22.));
#47107=CARTESIAN_POINT('Ctrl Pts',(-32.3552950943445,-54.4058891778527,
22.));
#47108=CARTESIAN_POINT('Ctrl Pts',(-32.2884097214115,-54.4200315485695,
22.));
#47109=CARTESIAN_POINT('Ctrl Pts',(-32.2277876728223,-54.4328495900511,
22.));
#47110=CARTESIAN_POINT('Ctrl Pts',(-32.1679169373206,-54.4488239715848,
22.));
#47111=CARTESIAN_POINT('Ctrl Pts',(-32.1090267714104,-54.4680568733301,
22.));
#47112=CARTESIAN_POINT('Ctrl Pts',(-32.0393564154629,-54.4908104704681,
22.));
#47113=CARTESIAN_POINT('Ctrl Pts',(-31.9710568700512,-54.5181250014914,
22.));
#47114=CARTESIAN_POINT('Ctrl Pts',(-31.904456962017,-54.5497238479896,22.));
#47115=CARTESIAN_POINT('Ctrl Pts',(-31.8897939177247,-54.5566808438693,
22.));
#47116=CARTESIAN_POINT('Ctrl Pts',(-31.8752134430768,-54.5638456669609,
22.));
#47117=CARTESIAN_POINT('Ctrl Pts',(-31.8607193748279,-54.5712156030182,
22.));
#47118=CARTESIAN_POINT('Ctrl Pts',(-31.8457643400408,-54.5788199310938,
22.));
#47119=CARTESIAN_POINT('Ctrl Pts',(-31.8308959671029,-54.5866456915096,
22.));
#47120=CARTESIAN_POINT('Ctrl Pts',(-31.816148277589,-54.5946733379087,22.));
#47121=CARTESIAN_POINT('Ctrl Pts',(-31.7559125281882,-54.6274616127308,
22.));
#47122=CARTESIAN_POINT('Ctrl Pts',(-31.6976088413262,-54.6636511833659,
22.));
#47123=CARTESIAN_POINT('Ctrl Pts',(-31.6414698544792,-54.7029684704927,
22.));
#47124=CARTESIAN_POINT('Ctrl Pts',(-31.5853421057777,-54.7422778869148,
22.));
#47125=CARTESIAN_POINT('Ctrl Pts',(-31.5313774894047,-54.7847146963307,
22.));
#47126=CARTESIAN_POINT('Ctrl Pts',(-31.4798463246137,-54.8300409282788,
22.));
#47127=CARTESIAN_POINT('Ctrl Pts',(-31.4425466815154,-54.8628492740926,
22.));
#47128=CARTESIAN_POINT('Ctrl Pts',(-31.4065227400659,-54.897172238623,22.));
#47129=CARTESIAN_POINT('Ctrl Pts',(-31.3718924922097,-54.9329270615862,
22.));
#47130=CARTESIAN_POINT('Ctrl Pts',(-31.3459157226426,-54.959747395096,22.));
#47131=CARTESIAN_POINT('Ctrl Pts',(-31.3207234114472,-54.9873735408281,
22.));
#47132=CARTESIAN_POINT('Ctrl Pts',(-31.296370938734,-55.0157718710984,22.));
#47133=CARTESIAN_POINT('Ctrl Pts',(-31.2882802397597,-55.0252067381156,
22.));
#47134=CARTESIAN_POINT('Ctrl Pts',(-31.2802886268347,-55.0347194488924,
22.));
#47135=CARTESIAN_POINT('Ctrl Pts',(-31.2723979365151,-55.0443082314672,
22.));
#47136=CARTESIAN_POINT('Ctrl Pts',(-31.2305359635119,-55.0951789843448,
22.));
#47137=CARTESIAN_POINT('Ctrl Pts',(-31.1915084683768,-55.1481921234089,
22.));
#47138=CARTESIAN_POINT('Ctrl Pts',(-31.1555797357512,-55.2031373177153,
22.));
#47139=CARTESIAN_POINT('Ctrl Pts',(-31.1302981918184,-55.2417999490479,
22.));
#47140=CARTESIAN_POINT('Ctrl Pts',(-31.1065518383412,-55.2814196841498,
22.));
#47141=CARTESIAN_POINT('Ctrl Pts',(-31.0844478042135,-55.3219265814321,
22.));
#47142=CARTESIAN_POINT('Ctrl Pts',(-31.0773529644147,-55.3349282781045,
22.));
#47143=CARTESIAN_POINT('Ctrl Pts',(-31.0704265008799,-55.3480232016838,
22.));
#47144=CARTESIAN_POINT('Ctrl Pts',(-31.0636752116797,-55.3612032674949,
22.));
#47145=CARTESIAN_POINT('Ctrl Pts',(-31.0349131818561,-55.4173533500487,
22.));
#47146=CARTESIAN_POINT('Ctrl Pts',(-31.0093835904652,-55.474934657336,22.));
#47147=CARTESIAN_POINT('Ctrl Pts',(-30.9873422739933,-55.5337599436784,
22.));
#47148=CARTESIAN_POINT('Ctrl Pts',(-30.967023266383,-55.5879886210984,22.));
#47149=CARTESIAN_POINT('Ctrl Pts',(-30.9496688942467,-55.6432750194878,
22.));
#47150=CARTESIAN_POINT('Ctrl Pts',(-30.9355188507018,-55.6994745658575,
22.));
#47151=CARTESIAN_POINT('Ctrl Pts',(-30.9328706183904,-55.7099925161458,
22.));
#47152=CARTESIAN_POINT('Ctrl Pts',(-30.9303347375364,-55.7205424451195,
22.));
#47153=CARTESIAN_POINT('Ctrl Pts',(-30.9279109916838,-55.7311226632894,
22.));
#47154=CARTESIAN_POINT('Origin',(-32.5,-56.2916512459885,17.));
#47155=CARTESIAN_POINT('Origin',(-65.,8.89946740503873E-15,13.));
#47156=CARTESIAN_POINT('Ctrl Pts',(-63.3648706727485,0.319230454628309,
13.));
#47157=CARTESIAN_POINT('Ctrl Pts',(-63.3697100624564,0.381552584091251,
13.));
#47158=CARTESIAN_POINT('Ctrl Pts',(-63.378326567255,0.443390469645943,13.));
#47159=CARTESIAN_POINT('Ctrl Pts',(-63.3904636088592,0.504524999022397,
13.));
#47160=CARTESIAN_POINT('Ctrl Pts',(-63.3981627172652,0.543305567168445,
13.));
#47161=CARTESIAN_POINT('Ctrl Pts',(-63.407279543875,0.581803401425318,13.));
#47162=CARTESIAN_POINT('Ctrl Pts',(-63.4177589835186,0.619964019244192,
13.));
#47163=CARTESIAN_POINT('Ctrl Pts',(-63.4249317270596,0.646083385764472,
13.));
#47164=CARTESIAN_POINT('Ctrl Pts',(-63.4327429983568,0.672044791355041,
13.));
#47165=CARTESIAN_POINT('Ctrl Pts',(-63.44117717048,0.697830748236588,13.));
#47166=CARTESIAN_POINT('Ctrl Pts',(-63.445633981288,0.711456641761924,13.));
#47167=CARTESIAN_POINT('Ctrl Pts',(-63.4502647769169,0.725033238553723,
13.));
#47168=CARTESIAN_POINT('Ctrl Pts',(-63.4550623359166,0.738544708502568,
13.));
#47169=CARTESIAN_POINT('Ctrl Pts',(-63.4771367982024,0.800713497636903,
13.));
#47170=CARTESIAN_POINT('Ctrl Pts',(-63.5027603464941,0.861575211953918,
13.));
#47171=CARTESIAN_POINT('Ctrl Pts',(-63.5316785435678,0.920885280715688,
13.));
#47172=CARTESIAN_POINT('Ctrl Pts',(-63.5525352082166,0.963661468017855,
13.));
#47173=CARTESIAN_POINT('Ctrl Pts',(-63.5751068651926,1.00563071995468,13.));
#47174=CARTESIAN_POINT('Ctrl Pts',(-63.5993147001603,1.04669965511365,13.));
#47175=CARTESIAN_POINT('Ctrl Pts',(-63.605972789105,1.05799519738412,13.));
#47176=CARTESIAN_POINT('Ctrl Pts',(-63.6127547253029,1.06922261593755,13.));
#47177=CARTESIAN_POINT('Ctrl Pts',(-63.6196590396186,1.08037991874502,13.));
#47178=CARTESIAN_POINT('Ctrl Pts',(-63.626655937187,1.09168683516212,13.));
#47179=CARTESIAN_POINT('Ctrl Pts',(-63.6337742037898,1.10291470667948,13.));
#47180=CARTESIAN_POINT('Ctrl Pts',(-63.6410091868788,1.11405768733435,13.));
#47181=CARTESIAN_POINT('Ctrl Pts',(-63.677959727572,1.17096717213473,13.));
#47182=CARTESIAN_POINT('Ctrl Pts',(-63.7179710364896,1.22569615332497,13.));
#47183=CARTESIAN_POINT('Ctrl Pts',(-63.7607845670049,1.27799720806722,13.));
#47184=CARTESIAN_POINT('Ctrl Pts',(-63.8042168530072,1.3310541351752,13.));
#47185=CARTESIAN_POINT('Ctrl Pts',(-63.8505333120092,1.38161344795932,13.));
#47186=CARTESIAN_POINT('Ctrl Pts',(-63.8995151782878,1.42940352748706,13.));
#47187=CARTESIAN_POINT('Ctrl Pts',(-63.9298610020025,1.4590110014124,13.));
#47188=CARTESIAN_POINT('Ctrl Pts',(-63.9612308491613,1.48755527123026,13.));
#47189=CARTESIAN_POINT('Ctrl Pts',(-63.9935813334301,1.51496662398692,13.));
#47190=CARTESIAN_POINT('Ctrl Pts',(-64.0200865946909,1.53742517701162,13.));
#47191=CARTESIAN_POINT('Ctrl Pts',(-64.047250267223,1.55912317435164,13.));
#47192=CARTESIAN_POINT('Ctrl Pts',(-64.075051394616,1.58001951663649,13.));
#47193=CARTESIAN_POINT('Ctrl Pts',(-64.0864069560373,1.58855477115841,13.));
#47194=CARTESIAN_POINT('Ctrl Pts',(-64.0978710427711,1.59695761719764,13.));
#47195=CARTESIAN_POINT('Ctrl Pts',(-64.1094224885555,1.60521141799748,13.));
#47196=CARTESIAN_POINT('Ctrl Pts',(-64.1667717340698,1.64618890751108,13.));
#47197=CARTESIAN_POINT('Ctrl Pts',(-64.226369023308,1.68357081331289,13.));
#47198=CARTESIAN_POINT('Ctrl Pts',(-64.2879736623947,1.71708519907432,13.));
#47199=CARTESIAN_POINT('Ctrl Pts',(-64.2948173902461,1.7208083494516,13.));
#47200=CARTESIAN_POINT('Ctrl Pts',(-64.3016859371774,1.72448374345449,13.));
#47201=CARTESIAN_POINT('Ctrl Pts',(-64.3085790067212,1.7281109868477,13.));
#47202=CARTESIAN_POINT('Ctrl Pts',(-64.3682468605388,1.75950916543472,13.));
#47203=CARTESIAN_POINT('Ctrl Pts',(-64.4297493247303,1.78730275834661,13.));
#47204=CARTESIAN_POINT('Ctrl Pts',(-64.492755333163,1.81157421873888,13.));
#47205=CARTESIAN_POINT('Ctrl Pts',(-64.56053950575,1.83768634520258,13.));
#47206=CARTESIAN_POINT('Ctrl Pts',(-64.6300645515071,1.85972265026168,13.));
#47207=CARTESIAN_POINT('Ctrl Pts',(-64.7009535899316,1.87773216280558,13.));
#47208=CARTESIAN_POINT('Ctrl Pts',(-64.7139243241626,1.88102740570952,13.));
#47209=CARTESIAN_POINT('Ctrl Pts',(-64.7269407953937,1.88418768229335,13.));
#47210=CARTESIAN_POINT('Ctrl Pts',(-64.7400007805811,1.88721308456642,13.));
#47211=CARTESIAN_POINT('Ctrl Pts',(-64.7512396222652,1.88981661103981,13.));
#47212=CARTESIAN_POINT('Ctrl Pts',(-64.7625015968045,1.89231813883989,13.));
#47213=CARTESIAN_POINT('Ctrl Pts',(-64.7737835811084,1.89471786797902,13.));
#47214=CARTESIAN_POINT('Ctrl Pts',(-64.8432969406401,1.90950367426388,13.));
#47215=CARTESIAN_POINT('Ctrl Pts',(-64.9135854863648,1.92043263341767,13.));
#47216=CARTESIAN_POINT('Ctrl Pts',(-64.9842819829643,1.92760569488594,13.));
#47217=CARTESIAN_POINT('Ctrl Pts',(-65.0564694634963,1.93493003569491,13.));
#47218=CARTESIAN_POINT('Ctrl Pts',(-65.1290831836877,1.93833864552109,13.));
#47219=CARTESIAN_POINT('Ctrl Pts',(-65.2017596774405,1.93789121633711,13.));
#47220=CARTESIAN_POINT('Ctrl Pts',(-65.2748769213569,1.93744107369689,13.));
#47221=CARTESIAN_POINT('Ctrl Pts',(-65.3480587637033,1.93308814118439,13.));
#47222=CARTESIAN_POINT('Ctrl Pts',(-65.4209476364575,1.92484231982115,13.));
#47223=CARTESIAN_POINT('Ctrl Pts',(-65.4389597304286,1.92280463555397,13.));
#47224=CARTESIAN_POINT('Ctrl Pts',(-65.456953949584,1.9205289761305,13.));
#47225=CARTESIAN_POINT('Ctrl Pts',(-65.4749248968271,1.91801499809801,13.));
#47226=CARTESIAN_POINT('Ctrl Pts',(-65.488986293,1.91604793199924,13.));
#47227=CARTESIAN_POINT('Ctrl Pts',(-65.5030350337315,1.91393458318872,13.));
#47228=CARTESIAN_POINT('Ctrl Pts',(-65.517047263033,1.91167847476885,13.));
#47229=CARTESIAN_POINT('Ctrl Pts',(-65.591432040293,1.89970178507336,13.));
#47230=CARTESIAN_POINT('Ctrl Pts',(-65.6649215571519,1.8836885467828,13.));
#47231=CARTESIAN_POINT('Ctrl Pts',(-65.7371322841359,1.86371341413835,13.));
#47232=CARTESIAN_POINT('Ctrl Pts',(-65.8094217303428,1.84371650596295,13.));
#47233=CARTESIAN_POINT('Ctrl Pts',(-65.8804307225326,1.81974914171634,13.));
#47234=CARTESIAN_POINT('Ctrl Pts',(-65.9497816751238,1.7918347665136,13.));
#47235=CARTESIAN_POINT('Ctrl Pts',(-66.0175539936567,1.76455580555915,13.));
#47236=CARTESIAN_POINT('Ctrl Pts',(-66.0837439306865,1.7335073683895,13.));
#47237=CARTESIAN_POINT('Ctrl Pts',(-66.1479900588654,1.69866277532066,13.));
#47238=CARTESIAN_POINT('Ctrl Pts',(-66.1618069173365,1.69116905041364,13.));
#47239=CARTESIAN_POINT('Ctrl Pts',(-66.1755338056604,1.68349956912868,13.));
#47240=CARTESIAN_POINT('Ctrl Pts',(-66.1891670016328,1.67565377050186,13.));
#47241=CARTESIAN_POINT('Ctrl Pts',(-66.2007100870974,1.66901081427424,13.));
#47242=CARTESIAN_POINT('Ctrl Pts',(-66.2121860050345,1.6622414568886,13.));
#47243=CARTESIAN_POINT('Ctrl Pts',(-66.2235939546713,1.65534738192939,13.));
#47244=CARTESIAN_POINT('Ctrl Pts',(-66.8826275096638,0.823232180103066,
13.));
#47245=CARTESIAN_POINT('Ctrl Pts',(-66.9060091418342,0.752340565238968,
13.));
#47246=CARTESIAN_POINT('Ctrl Pts',(-66.9251542481801,0.68022746278438,13.));
#47247=CARTESIAN_POINT('Ctrl Pts',(-66.9401506980285,0.607243329609344,
13.));
#47248=CARTESIAN_POINT('Ctrl Pts',(-66.9547542267029,0.536171449772777,
13.));
#47249=CARTESIAN_POINT('Ctrl Pts',(-66.9654231894066,0.464272677051844,
13.));
#47250=CARTESIAN_POINT('Ctrl Pts',(-66.9721930205228,0.391873748623409,
13.));
#47251=CARTESIAN_POINT('Ctrl Pts',(-66.9737040257789,0.375714532903923,
13.));
#47252=CARTESIAN_POINT('Ctrl Pts',(-66.9750207650679,0.359528284463992,
13.));
#47253=CARTESIAN_POINT('Ctrl Pts',(-66.9761428768271,0.343325629877727,
13.));
#47254=CARTESIAN_POINT('Ctrl Pts',(-66.9812921188236,0.268973508740579,
13.));
#47255=CARTESIAN_POINT('Ctrl Pts',(-66.9823380095277,0.194422974417003,
13.));
#47256=CARTESIAN_POINT('Ctrl Pts',(-66.9793427332487,0.120028700639496,
13.));
#47257=CARTESIAN_POINT('Ctrl Pts',(-66.977239855127,0.0677990977152428,
13.));
#47258=CARTESIAN_POINT('Ctrl Pts',(-66.9731439810344,0.0156465389589379,
13.));
#47259=CARTESIAN_POINT('Ctrl Pts',(-66.9670620462898,-0.0363014254759868,
13.));
#47260=CARTESIAN_POINT('Ctrl Pts',(-66.9647496285849,-0.0560526062653882,
13.));
#47261=CARTESIAN_POINT('Ctrl Pts',(-66.9621499864736,-0.0757741525187293,
13.));
#47262=CARTESIAN_POINT('Ctrl Pts',(-66.9592630725001,-0.0954588083553777,
13.));
#47263=CARTESIAN_POINT('Ctrl Pts',(-66.9565142387798,-0.114201952846506,
13.));
#47264=CARTESIAN_POINT('Ctrl Pts',(-66.9535037847693,-0.132917493441565,
13.));
#47265=CARTESIAN_POINT('Ctrl Pts',(-66.9502376703059,-0.151566178101122,
13.));
#47266=CARTESIAN_POINT('Ctrl Pts',(-66.9377139254706,-0.223073582635083,
13.));
#47267=CARTESIAN_POINT('Ctrl Pts',(-66.9214263256518,-0.293675712348754,
13.));
#47268=CARTESIAN_POINT('Ctrl Pts',(-66.901430305801,-0.363043772410292,
13.));
#47269=CARTESIAN_POINT('Ctrl Pts',(-66.8818637674749,-0.430921920958888,
13.));
#47270=CARTESIAN_POINT('Ctrl Pts',(-66.858745943864,-0.497619260724826,
13.));
#47271=CARTESIAN_POINT('Ctrl Pts',(-66.8320856793692,-0.562804370280902,
13.));
#47272=CARTESIAN_POINT('Ctrl Pts',(-66.8060100727734,-0.626559974544455,
13.));
#47273=CARTESIAN_POINT('Ctrl Pts',(-66.776545304655,-0.688869612388516,
13.));
#47274=CARTESIAN_POINT('Ctrl Pts',(-66.743664114667,-0.749389827227639,
13.));
#47275=CARTESIAN_POINT('Ctrl Pts',(-66.7329788263415,-0.769056875327405,
13.));
#47276=CARTESIAN_POINT('Ctrl Pts',(-66.7219324918179,-0.788534645854941,
13.));
#47277=CARTESIAN_POINT('Ctrl Pts',(-66.7105234437577,-0.807810393773745,
13.));
#47278=CARTESIAN_POINT('Ctrl Pts',(-66.7040881270254,-0.818682952330261,
13.));
#47279=CARTESIAN_POINT('Ctrl Pts',(-66.6975366287906,-0.829492290648959,
13.));
#47280=CARTESIAN_POINT('Ctrl Pts',(-66.6908782710633,-0.840221024848607,
13.));
#47281=CARTESIAN_POINT('Ctrl Pts',(-66.6548614907131,-0.898255525086147,
13.));
#47282=CARTESIAN_POINT('Ctrl Pts',(-66.615661353053,-0.954037570632601,
13.));
#47283=CARTESIAN_POINT('Ctrl Pts',(-66.5732918036362,-1.00726408538098,
13.));
#47284=CARTESIAN_POINT('Ctrl Pts',(-66.567176292694,-1.01494666255824,13.));
#47285=CARTESIAN_POINT('Ctrl Pts',(-66.5609946871419,-1.0225759395538,13.));
#47286=CARTESIAN_POINT('Ctrl Pts',(-66.5547469639699,-1.03015094108865,
13.));
#47287=CARTESIAN_POINT('Ctrl Pts',(-66.5106056086058,-1.08366977113728,
13.));
#47288=CARTESIAN_POINT('Ctrl Pts',(-66.4631661110425,-1.13448299231823,
13.));
#47289=CARTESIAN_POINT('Ctrl Pts',(-66.4127666235244,-1.18244447912767,
13.));
#47290=CARTESIAN_POINT('Ctrl Pts',(-66.3657479708622,-1.22718867396982,
13.));
#47291=CARTESIAN_POINT('Ctrl Pts',(-66.3161520834424,-1.26945072111176,
13.));
#47292=CARTESIAN_POINT('Ctrl Pts',(-66.2642393874467,-1.30907445581882,
13.));
#47293=CARTESIAN_POINT('Ctrl Pts',(-66.2527825898775,-1.31781915880077,
13.));
#47294=CARTESIAN_POINT('Ctrl Pts',(-66.2412129249561,-1.32643521268399,
13.));
#47295=CARTESIAN_POINT('Ctrl Pts',(-66.2295331629306,-1.33492068207895,
13.));
#47296=CARTESIAN_POINT('Ctrl Pts',(-66.2204025954476,-1.34155413494954,
13.));
#47297=CARTESIAN_POINT('Ctrl Pts',(-66.211205267767,-1.3481073045967,13.));
#47298=CARTESIAN_POINT('Ctrl Pts',(-66.20195334148,-1.35457199230889,13.));
#47299=CARTESIAN_POINT('Ctrl Pts',(-66.1459049971557,-1.39373519266308,
13.));
#47300=CARTESIAN_POINT('Ctrl Pts',(-66.0877532412386,-1.42972959266972,
13.));
#47301=CARTESIAN_POINT('Ctrl Pts',(-66.0278290563933,-1.46243222383127,
13.));
#47302=CARTESIAN_POINT('Ctrl Pts',(-65.9681817046083,-1.4949837779363,13.));
#47303=CARTESIAN_POINT('Ctrl Pts',(-65.906777156648,-1.52427416697934,13.));
#47304=CARTESIAN_POINT('Ctrl Pts',(-65.8439279088097,-1.55013292110232,
13.));
#47305=CARTESIAN_POINT('Ctrl Pts',(-65.7824252697681,-1.57543762522515,
13.));
#47306=CARTESIAN_POINT('Ctrl Pts',(-65.7195382072492,-1.59745625930267,
13.));
#47307=CARTESIAN_POINT('Ctrl Pts',(-65.6555614671547,-1.61597952395889,
13.));
#47308=CARTESIAN_POINT('Ctrl Pts',(-65.6420830167795,-1.6198819563599,13.));
#47309=CARTESIAN_POINT('Ctrl Pts',(-65.6285562369111,-1.6236290657015,13.));
#47310=CARTESIAN_POINT('Ctrl Pts',(-65.6149839556941,-1.62721860052123,
13.));
#47311=CARTESIAN_POINT('Ctrl Pts',(-65.6021159150352,-1.63062188102127,
13.));
#47312=CARTESIAN_POINT('Ctrl Pts',(-65.5892052056162,-1.63388381680147,
13.));
#47313=CARTESIAN_POINT('Ctrl Pts',(-65.5762752297125,-1.63699772297707,
13.));
#47314=CARTESIAN_POINT('Ctrl Pts',(-65.5127465220931,-1.65229724375406,
13.));
#47315=CARTESIAN_POINT('Ctrl Pts',(-65.4486405343066,-1.66405837362243,
13.));
#47316=CARTESIAN_POINT('Ctrl Pts',(-65.3842420394353,-1.67213585463769,
13.));
#47317=CARTESIAN_POINT('Ctrl Pts',(-65.3210685725296,-1.68005968081747,
13.));
#47318=CARTESIAN_POINT('Ctrl Pts',(-65.2576127400953,-1.68443871292178,
13.));
#47319=CARTESIAN_POINT('Ctrl Pts',(-65.1941497363329,-1.68508652435015,
13.));
#47320=CARTESIAN_POINT('Ctrl Pts',(-65.1327484539533,-1.6857132903411,13.));
#47321=CARTESIAN_POINT('Ctrl Pts',(-65.0713397980825,-1.68284723930874,
13.));
#47322=CARTESIAN_POINT('Ctrl Pts',(-65.0101900872574,-1.67627347092458,
13.));
#47323=CARTESIAN_POINT('Ctrl Pts',(-65.000007166314,-1.67517877786957,13.));
#47324=CARTESIAN_POINT('Ctrl Pts',(-64.989831478164,-1.67398116343886,13.));
#47325=CARTESIAN_POINT('Ctrl Pts',(-64.9796643197989,-1.67267950846502,
13.));
#47326=CARTESIAN_POINT('Ctrl Pts',(-64.9689074729785,-1.67130235836429,
13.));
#47327=CARTESIAN_POINT('Ctrl Pts',(-64.9581601737451,-1.66980874798798,
13.));
#47328=CARTESIAN_POINT('Ctrl Pts',(-64.9474239513002,-1.66819938802346,
13.));
#47329=CARTESIAN_POINT('Origin',(-65.,8.88178419700125E-15,23.5459252805377));
#47330=CARTESIAN_POINT('Ctrl Pts',(-62.9434348764936,-0.00149614206265766,
21.7959252805377));
#47331=CARTESIAN_POINT('Ctrl Pts',(-62.9426160796481,-0.0997858054225679,
21.7905813053169));
#47332=CARTESIAN_POINT('Ctrl Pts',(-62.9937092272654,-0.878618068249771,
21.7481913665734));
#47333=CARTESIAN_POINT('Ctrl Pts',(-63.9890540527047,-2.20843040890227,
21.6687554643073));
#47334=CARTESIAN_POINT('Ctrl Pts',(-66.3069967286646,-2.04687460564973,
21.5576175737392));
#47335=CARTESIAN_POINT('Ctrl Pts',(-67.428612079538,-0.0121339679509515,
21.4464796831712));
#47336=CARTESIAN_POINT('Ctrl Pts',(-66.3273005244664,2.03388573489001,21.3353417926031));
#47337=CARTESIAN_POINT('Ctrl Pts',(-64.0110910734901,2.21817972145312,21.2242039020351));
#47338=CARTESIAN_POINT('Ctrl Pts',(-62.9978510382059,0.892619747709234,
21.1443983980133));
#47339=CARTESIAN_POINT('Ctrl Pts',(-62.942718846502,0.106740802471778,21.1016388575141));
#47340=CARTESIAN_POINT('Ctrl Pts',(-62.9436210622307,0.00160392935066219,
21.0959252805377));
#47341=CARTESIAN_POINT('Ctrl Pts',(-62.9473239618077,0.00235074752841319,
21.8540747194623));
#47342=CARTESIAN_POINT('Ctrl Pts',(-62.9508762982105,-0.467866578479425,
21.8286245525962));
#47343=CARTESIAN_POINT('Ctrl Pts',(-63.3434621334709,-1.62957520615004,
21.7661284222074));
#47344=CARTESIAN_POINT('Ctrl Pts',(-65.2721300366129,-2.41280623887488,
21.6665863282959));
#47345=CARTESIAN_POINT('Ctrl Pts',(-67.1747422685441,-1.08094901338604,
21.5554484377278));
#47346=CARTESIAN_POINT('Ctrl Pts',(-67.0876157148515,1.24138505016238,21.4443105471598));
#47347=CARTESIAN_POINT('Ctrl Pts',(-65.0892538486774,2.42692553227055,21.3331726565917));
#47348=CARTESIAN_POINT('Ctrl Pts',(-63.2787520820962,1.52545559952442,21.2364273806926));
#47349=CARTESIAN_POINT('Ctrl Pts',(-62.9500869585733,0.417919283968027,
21.1767280683161));
#47350=CARTESIAN_POINT('Ctrl Pts',(-62.9479182248742,-0.00116161895480603,
21.1540747194623));
#47351=CARTESIAN_POINT('Ctrl Pts',(-66.2690708798524,-1.07935865304854,
22.));
#47352=CARTESIAN_POINT('Ctrl Pts',(-66.6279833110066,-0.657362393039546,
21.9629540364773));
#47353=CARTESIAN_POINT('Ctrl Pts',(-66.8852826717605,0.565789777391224,
21.8888621094319));
#47354=CARTESIAN_POINT('Ctrl Pts',(-65.5450879211412,1.89344353213328,21.7777242188639));
#47355=CARTESIAN_POINT('Ctrl Pts',(-63.7057951684468,1.4835378033008,21.6665863282959));
#47356=CARTESIAN_POINT('Ctrl Pts',(-63.0512142972679,-0.282082603662771,
21.5554484377278));
#47357=CARTESIAN_POINT('Ctrl Pts',(-64.180320745495,-1.79060472623491,21.4443105471598));
#47358=CARTESIAN_POINT('Ctrl Pts',(-66.0597184815454,-1.65961459691566,
21.3331726565917));
#47359=CARTESIAN_POINT('Ctrl Pts',(-66.9691289570557,-0.00983827259096255,
21.2220347660237));
#47360=CARTESIAN_POINT('Ctrl Pts',(-66.0761808851497,1.64908316550761,21.1108968754557));
#47361=CARTESIAN_POINT('Ctrl Pts',(-64.1981884552545,1.79850951013062,20.9997589848876));
#47362=CARTESIAN_POINT('Ctrl Pts',(-63.0541051349916,0.30177526833428,20.8886210943196));
#47363=CARTESIAN_POINT('Ctrl Pts',(-63.6911204902705,-1.47119522218438,
20.7774832037516));
#47364=CARTESIAN_POINT('Ctrl Pts',(-65.5261685894954,-1.89755500871052,
20.6663453131835));
#47365=CARTESIAN_POINT('Ctrl Pts',(-66.8796083671824,-0.587065728133525,
20.5552074226155));
#47366=CARTESIAN_POINT('Ctrl Pts',(-66.5126214133544,1.26077376527148,20.4440695320474));
#47367=CARTESIAN_POINT('Ctrl Pts',(-64.7611148635138,1.95461157704263,20.3329316414794));
#47368=CARTESIAN_POINT('Ctrl Pts',(-63.2282626195245,0.859371828191353,
20.2217937509113));
#47369=CARTESIAN_POINT('Ctrl Pts',(-63.3171016769871,-1.02246099457514,
20.1106558603433));
#47370=CARTESIAN_POINT('Ctrl Pts',(-64.9463166628138,-1.96842352553114,
19.9995179697752));
#47371=CARTESIAN_POINT('Ctrl Pts',(-66.6246686119733,-1.11266575470346,
19.8883800792072));
#47372=CARTESIAN_POINT('Ctrl Pts',(-66.8159429576165,0.761527637475698,
19.7772421886392));
#47373=CARTESIAN_POINT('Ctrl Pts',(-65.3450641189423,1.9386861278219,19.6661042980711));
#47374=CARTESIAN_POINT('Ctrl Pts',(-63.5583441794198,1.34134322872205,19.5549664075031));
#47375=CARTESIAN_POINT('Ctrl Pts',(-63.0911881617047,-0.483746344304426,
19.443828516935));
#47376=CARTESIAN_POINT('Ctrl Pts',(-64.3711892671104,-1.86605739990807,
19.332690626367));
#47377=CARTESIAN_POINT('Ctrl Pts',(-66.2267479674628,-1.54034495606734,
19.221552735799));
#47378=CARTESIAN_POINT('Ctrl Pts',(-66.9594503409616,0.195262695377469,
19.1104148452309));
#47379=CARTESIAN_POINT('Ctrl Pts',(-65.8986455956832,1.75214418700341,18.9992769546629));
#47380=CARTESIAN_POINT('Ctrl Pts',(-64.0153003453502,1.70526823375496,18.8881390640948));
#47381=CARTESIAN_POINT('Ctrl Pts',(-63.0332618561676,0.0975409270146975,
18.7770011735268));
#47382=CARTESIAN_POINT('Ctrl Pts',(-63.8514010943644,-1.59946669637174,
18.6658632829587));
#47383=CARTESIAN_POINT('Ctrl Pts',(-65.720865936886,-1.83246431340308,18.5547253923907));
#47384=CARTESIAN_POINT('Ctrl Pts',(-66.9305140122006,-0.388186562807738,
18.4435875018227));
#47385=CARTESIAN_POINT('Ctrl Pts',(-66.3731407186298,1.41140275105549,18.3324496112546));
#47386=CARTESIAN_POINT('Ctrl Pts',(-64.5589161528223,1.91911912048435,18.2213117206866));
#47387=CARTESIAN_POINT('Ctrl Pts',(-63.1484206345677,0.670243994641496,
18.1101738301185));
#47388=CARTESIAN_POINT('Ctrl Pts',(-63.4326967078313,-1.19211306057993,
17.9990359395505));
#47389=CARTESIAN_POINT('Ctrl Pts',(-65.1515432588453,-1.96331551197125,
17.8878980489824));
#47390=CARTESIAN_POINT('Ctrl Pts',(-66.7316805464207,-0.937473009742842,
17.7767601584144));
#47391=CARTESIAN_POINT('Ctrl Pts',(-66.7267909912641,0.946449169970149,
17.6656222678463));
#47392=CARTESIAN_POINT('Ctrl Pts',(-65.1413500586618,1.9640756909459,17.5544843772784));
#47393=CARTESIAN_POINT('Ctrl Pts',(-63.4265298143476,1.18396145786557,17.4433464867103));
#47394=CARTESIAN_POINT('Ctrl Pts',(-63.1519246753265,-0.679846124635249,
17.3322085961423));
#47395=CARTESIAN_POINT('Ctrl Pts',(-64.5688838395789,-1.92138283927799,
17.2210707055742));
#47396=CARTESIAN_POINT('Ctrl Pts',(-66.3804485146544,-1.40425605116614,
17.1099328150062));
#47397=CARTESIAN_POINT('Ctrl Pts',(-66.9284730089157,0.398202225924807,
16.9987949244381));
#47398=CARTESIAN_POINT('Ctrl Pts',(-65.7113442877452,1.83618148970649,16.8876570338701));
#47399=CARTESIAN_POINT('Ctrl Pts',(-63.8431140728085,1.59348301224527,16.776519143302));
#47400=CARTESIAN_POINT('Ctrl Pts',(-63.033794667009,-0.107748537650181,
16.665381252734));
#47401=CARTESIAN_POINT('Ctrl Pts',(-64.024165300781,-1.71035662908352,16.5542433621659));
#47402=CARTESIAN_POINT('Ctrl Pts',(-65.9077285014668,-1.74745590115202,
16.4431054715979));
#47403=CARTESIAN_POINT('Ctrl Pts',(-66.9604375104179,-0.18508896940078,
16.3319675810299));
#47404=CARTESIAN_POINT('Ctrl Pts',(-66.2187358332113,1.54669199509962,16.2208296904618));
#47405=CARTESIAN_POINT('Ctrl Pts',(-64.3615114264595,1.86276823579531,16.1096917998938));
#47406=CARTESIAN_POINT('Ctrl Pts',(-63.0887028520271,0.473831585058423,
15.9985539093257));
#47407=CARTESIAN_POINT('Ctrl Pts',(-63.5653262327086,-1.34880848913672,
15.8874160187577));
#47408=CARTESIAN_POINT('Ctrl Pts',(-65.3551227829179,-1.9368688566197,15.7762781281897));
#47409=CARTESIAN_POINT('Ctrl Pts',(-66.819871422519,-0.75209119420401,15.6651402376216));
#47410=CARTESIAN_POINT('Ctrl Pts',(-66.6188711104164,1.12108406786279,15.5540023470536));
#47411=CARTESIAN_POINT('Ctrl Pts',(-64.9360997115566,1.96811836805764,15.4428644564855));
#47412=CARTESIAN_POINT('Ctrl Pts',(-63.3118169716773,1.01371160717774,15.3317265659175));
#47413=CARTESIAN_POINT('Ctrl Pts',(-63.2327473023447,-0.868556886382297,
15.2205886753495));
#47414=CARTESIAN_POINT('Ctrl Pts',(-64.771264070325,-1.95582540705099,15.1094507847814));
#47415=CARTESIAN_POINT('Ctrl Pts',(-66.5191454265163,-1.25290476136478,
14.9983128942134));
#47416=CARTESIAN_POINT('Ctrl Pts',(-66.8765357500253,0.596813839734138,
14.8871750036453));
#47417=CARTESIAN_POINT('Ctrl Pts',(-65.516311611266,1.90026192842666,14.7760371130773));
#47418=CARTESIAN_POINT('Ctrl Pts',(-63.6835016170176,1.46437879615622,14.6648992225092));
#47419=CARTESIAN_POINT('Ctrl Pts',(-63.0556974877489,-0.311866999404029,
14.5537613319412));
#47420=CARTESIAN_POINT('Ctrl Pts',(-64.2075355674246,-1.80265710789544,
14.4426234413732));
#47421=CARTESIAN_POINT('Ctrl Pts',(-66.0847251913073,-1.64345528891983,
14.3314855508051));
#47422=CARTESIAN_POINT('Ctrl Pts',(-66.969053819969,0.0200209189642882,
14.2203476602371));
#47423=CARTESIAN_POINT('Ctrl Pts',(-66.0510846129266,1.66516952053626,14.109209769669));
#47424=CARTESIAN_POINT('Ctrl Pts',(-64.1710468184079,1.78617400482043,13.998071879101));
#47425=CARTESIAN_POINT('Ctrl Pts',(-63.049757131241,0.272264377212432,13.8869339885329));
#47426=CARTESIAN_POINT('Ctrl Pts',(-63.7135511069036,-1.49083448335768,
13.7757960979649));
#47427=CARTESIAN_POINT('Ctrl Pts',(-65.5548379149366,-1.88939023827018,
13.6646582073969));
#47428=CARTESIAN_POINT('Ctrl Pts',(-66.8882920122399,-0.558497016674497,
13.5535203168288));
#47429=CARTESIAN_POINT('Ctrl Pts',(-66.4933378285089,1.28345860874756,13.4423824262608));
#47430=CARTESIAN_POINT('Ctrl Pts',(-64.7315804519141,1.95092037563963,13.3312445356927));
#47431=CARTESIAN_POINT('Ctrl Pts',(-63.2153798048402,0.832146062593817,
13.2201066451247));
#47432=CARTESIAN_POINT('Ctrl Pts',(-63.3329222496525,-1.04723556764185,
13.1089687545567));
#47433=CARTESIAN_POINT('Ctrl Pts',(-64.9758366741791,-1.97019425053384,
12.9978308639886));
#47434=CARTESIAN_POINT('Ctrl Pts',(-66.6419915114447,-1.08548270413876,
12.8866929734206));
#47435=CARTESIAN_POINT('Ctrl Pts',(-66.7483953817108,0.159901738299123,
12.8126010463752));
#47436=CARTESIAN_POINT('Ctrl Pts',(-66.526442356053,0.66748013726814,12.7755550828525));
#47437=CARTESIAN_POINT('Ctrl Pts',(-66.3677806246588,-1.16331236980977,
22.0748149723825));
#47438=CARTESIAN_POINT('Ctrl Pts',(-66.7546096639785,-0.708492771249656,
22.0377690088598));
#47439=CARTESIAN_POINT('Ctrl Pts',(-67.0319220552433,0.60979753568671,21.9636770818144));
#47440=CARTESIAN_POINT('Ctrl Pts',(-65.5874854660279,2.04071767641436,21.8525391912464));
#47441=CARTESIAN_POINT('Ctrl Pts',(-63.605130476917,1.59892902399572,21.7414013006783));
#47442=CARTESIAN_POINT('Ctrl Pts',(-62.8996355773925,-0.304023302377036,
21.6302634101103));
#47443=CARTESIAN_POINT('Ctrl Pts',(-64.1165651812316,-1.9298799537907,21.5191255195423));
#47444=CARTESIAN_POINT('Ctrl Pts',(-66.1421445639184,-1.78870126649369,
21.4079876289742));
#47445=CARTESIAN_POINT('Ctrl Pts',(-67.1222899978831,-0.0106035043776257,
21.2968497384062));
#47446=CARTESIAN_POINT('Ctrl Pts',(-66.1598874315886,1.77735068863507,21.1857118478382));
#47447=CARTESIAN_POINT('Ctrl Pts',(-64.135822661333,1.93839958057146,21.0745739572701));
#47448=CARTESIAN_POINT('Ctrl Pts',(-62.9027512676903,0.325247684413701,
20.9634360667021));
#47449=CARTESIAN_POINT('Ctrl Pts',(-63.5893143859473,-1.58562642318961,
20.852298176134));
#47450=CARTESIAN_POINT('Ctrl Pts',(-65.5670945677199,-2.04514894821357,
20.741160285566));
#47451=CARTESIAN_POINT('Ctrl Pts',(-67.0258063969427,-0.632728353546071,
20.630022394998));
#47452=CARTESIAN_POINT('Ctrl Pts',(-66.6302747895932,1.35883815127574,20.5188845044299));
#47453=CARTESIAN_POINT('Ctrl Pts',(-64.7425341118513,2.10664343990284,20.4077466138619));
#47454=CARTESIAN_POINT('Ctrl Pts',(-63.0904549151108,0.92621472499195,20.2966087232938));
#47455=CARTESIAN_POINT('Ctrl Pts',(-63.1862039732914,-1.10198914816479,
20.1854708327258));
#47456=CARTESIAN_POINT('Ctrl Pts',(-64.9421411131276,-2.12152969710982,
20.0743329421577));
#47457=CARTESIAN_POINT('Ctrl Pts',(-66.7510371439672,-1.19921013488373,
19.9631950515897));
#47458=CARTESIAN_POINT('Ctrl Pts',(-66.9571890209963,0.820760104276152,
19.8520571610216));
#47459=CARTESIAN_POINT('Ctrl Pts',(-65.3719035899786,2.08947929152553,19.7409192704536));
#47460=CARTESIAN_POINT('Ctrl Pts',(-63.4462105859322,1.44567439722259,19.6297813798856));
#47461=CARTESIAN_POINT('Ctrl Pts',(-62.9427186534739,-0.521372673105617,
19.5186434893175));
#47462=CARTESIAN_POINT('Ctrl Pts',(-64.3222796687889,-2.0112014203591,19.4075055987495));
#47463=CARTESIAN_POINT('Ctrl Pts',(-66.3221657890617,-1.66015470029927,
19.2963677081814));
#47464=CARTESIAN_POINT('Ctrl Pts',(-67.1118585682623,0.210450445042934,
19.1852298176134));
#47465=CARTESIAN_POINT('Ctrl Pts',(-65.9685432498092,1.88842791103254,19.0740919270454));
#47466=CARTESIAN_POINT('Ctrl Pts',(-63.9387093107874,1.8379058939935,18.9629540364773));
#47467=CARTESIAN_POINT('Ctrl Pts',(-62.8802867754522,0.105127768826814,
18.8518161459093));
#47468=CARTESIAN_POINT('Ctrl Pts',(-63.762061793731,-1.72387499533423,18.7406782553413));
#47469=CARTESIAN_POINT('Ctrl Pts',(-65.7769356913806,-1.97499542621529,
18.6295403647732));
#47470=CARTESIAN_POINT('Ctrl Pts',(-67.0806715396602,-0.418380145499115,
18.5184024742052));
#47471=CARTESIAN_POINT('Ctrl Pts',(-66.4799451312683,1.52118322714049,18.4072645836371));
#47472=CARTESIAN_POINT('Ctrl Pts',(-64.5246081605074,2.06839034059005,18.296126693069));
#47473=CARTESIAN_POINT('Ctrl Pts',(-63.0044027317441,0.722376318154277,
18.184988802501));
#47474=CARTESIAN_POINT('Ctrl Pts',(-63.3107901142278,-1.28483694059203,
18.073850911933));
#47475=CARTESIAN_POINT('Ctrl Pts',(-65.1633304621018,-2.11602437657286,
17.962713021365));
#47476=CARTESIAN_POINT('Ctrl Pts',(-66.8663725857206,-1.01039070332778,
17.8515751307969));
#47477=CARTESIAN_POINT('Ctrl Pts',(-66.8611027155246,1.02006503928305,17.7404372402289));
#47478=CARTESIAN_POINT('Ctrl Pts',(-65.1523444234686,2.11684368311381,17.6292993496608));
#47479=CARTESIAN_POINT('Ctrl Pts',(-63.3041435529085,1.27605129715033,17.5181614590928));
#47480=CARTESIAN_POINT('Ctrl Pts',(-63.0081793206914,-0.732725312500785,
17.4070235685247));
#47481=CARTESIAN_POINT('Ctrl Pts',(-64.5353511450282,-2.07083013394973,
17.2958856779567));
#47482=CARTESIAN_POINT('Ctrl Pts',(-66.4878213357972,-1.51348064898344,
17.1847477873886));
#47483=CARTESIAN_POINT('Ctrl Pts',(-67.0784717848694,0.429174838035305,
17.0736098968206));
#47484=CARTESIAN_POINT('Ctrl Pts',(-65.7666734377774,1.97900172862673,16.9624720062526));
#47485=CARTESIAN_POINT('Ctrl Pts',(-63.7531301984196,1.71742589359988,16.8513341156845));
#47486=CARTESIAN_POINT('Ctrl Pts',(-62.8808610289137,-0.116129338772932,
16.7401962251165));
#47487=CARTESIAN_POINT('Ctrl Pts',(-63.9482637923134,-1.84339007037128,
16.6290583345485));
#47488=CARTESIAN_POINT('Ctrl Pts',(-65.9783326341088,-1.88337496509217,
16.5179204439804));
#47489=CARTESIAN_POINT('Ctrl Pts',(-67.1129225208572,-0.199485395342068,
16.4067825534124));
#47490=CARTESIAN_POINT('Ctrl Pts',(-66.3135304620949,1.66699541908822,16.2956446628443));
#47491=CARTESIAN_POINT('Ctrl Pts',(-64.3118490749262,2.00765642140263,16.1845067722763));
#47492=CARTESIAN_POINT('Ctrl Pts',(-62.9400400336448,0.510686732855833,
16.0733688817082));
#47493=CARTESIAN_POINT('Ctrl Pts',(-63.4537357110932,-1.45372031389701,
15.9622309911402));
#47494=CARTESIAN_POINT('Ctrl Pts',(-65.3827446280278,-2.08752067094761,
15.8510931005722));
#47495=CARTESIAN_POINT('Ctrl Pts',(-66.9614230462693,-0.810589683949272,
15.7399552100041));
#47496=CARTESIAN_POINT('Ctrl Pts',(-66.7447887062896,1.20828323380549,15.6288173194361));
#47497=CARTESIAN_POINT('Ctrl Pts',(-64.931129476036,2.12120080414855,15.517679428868));
#47498=CARTESIAN_POINT('Ctrl Pts',(-63.1805082177236,1.09255922368242,15.4065415383));
#47499=CARTESIAN_POINT('Ctrl Pts',(-63.0952884215498,-0.93611420722686,
15.2954036477319));
#47500=CARTESIAN_POINT('Ctrl Pts',(-64.7534727352587,-2.10795168295957,
15.1842657571639));
#47501=CARTESIAN_POINT('Ctrl Pts',(-66.6373062477565,-1.35035708749135,
15.0731278665959));
#47502=CARTESIAN_POINT('Ctrl Pts',(-67.022494788205,0.643234684111219,14.9619899760278));
#47503=CARTESIAN_POINT('Ctrl Pts',(-65.5564709027586,2.04806641515652,14.8508520854598));
#47504=CARTESIAN_POINT('Ctrl Pts',(-63.5811029082571,1.57827980796209,14.7397141948917));
#47505=CARTESIAN_POINT('Ctrl Pts',(-62.9044674754165,-0.336124361552553,
14.6285763043237));
#47506=CARTESIAN_POINT('Ctrl Pts',(-64.1458968022858,-1.94286978310439,
14.5174384137556));
#47507=CARTESIAN_POINT('Ctrl Pts',(-66.1690963233843,-1.7712850695456,14.4063005231876));
#47508=CARTESIAN_POINT('Ctrl Pts',(-67.1222090165502,0.0215781683135005,
14.2951626326196));
#47509=CARTESIAN_POINT('Ctrl Pts',(-66.1328391433939,1.79468825825304,14.1840247420515));
#47510=CARTESIAN_POINT('Ctrl Pts',(-64.1065699177788,1.92510460593566,14.0728868514835));
#47511=CARTESIAN_POINT('Ctrl Pts',(-62.8980650713711,0.293441403351154,
13.9617489609155));
#47512=CARTESIAN_POINT('Ctrl Pts',(-63.613489680895,-1.60679324794458,13.8506110703474));
#47513=CARTESIAN_POINT('Ctrl Pts',(-65.5979938251871,-2.03634911284551,
13.7394731797794));
#47514=CARTESIAN_POINT('Ctrl Pts',(-67.0351654655728,-0.601937535928643,
13.6283352892113));
#47515=CARTESIAN_POINT('Ctrl Pts',(-66.6094913060666,1.38328744711303,13.5171973986433));
#47516=CARTESIAN_POINT('Ctrl Pts',(-64.7107024808619,2.10266513274846,13.4060595080752));
#47517=CARTESIAN_POINT('Ctrl Pts',(-63.0765700607689,0.89687130905907,13.2949216175072));
#47518=CARTESIAN_POINT('Ctrl Pts',(-63.2032550876981,-1.12869071508498,
13.1837837269391));
#47519=CARTESIAN_POINT('Ctrl Pts',(-64.9739572238164,-2.12343815107306,
13.0726458363711));
#47520=CARTESIAN_POINT('Ctrl Pts',(-66.7697074378301,-1.16991275640645,
12.9615079458031));
#47521=CARTESIAN_POINT('Ctrl Pts',(-66.8843875194939,0.172339073385913,
12.8874160187577));
#47522=CARTESIAN_POINT('Ctrl Pts',(-66.6451707405899,0.719397484879782,
12.850370055235));
#47523=CARTESIAN_POINT('Ctrl Pts',(-66.4664903694652,-1.24726608657099,
22.149629944765));
#47524=CARTESIAN_POINT('Ctrl Pts',(-66.8812360169505,-0.759623149459765,
22.1125839812423));
#47525=CARTESIAN_POINT('Ctrl Pts',(-67.1785614387261,0.653805293982196,
22.0384920541969));
#47526=CARTESIAN_POINT('Ctrl Pts',(-65.6298830109146,2.18799182069543,21.9273541636289));
#47527=CARTESIAN_POINT('Ctrl Pts',(-63.5044657853871,1.71432024469064,21.8162162730608));
#47528=CARTESIAN_POINT('Ctrl Pts',(-62.7480568575172,-0.325964001091306,
21.7050783824928));
#47529=CARTESIAN_POINT('Ctrl Pts',(-64.0528096169681,-2.06915518134648,
21.5939404919247));
#47530=CARTESIAN_POINT('Ctrl Pts',(-66.2245706462915,-1.91778793607171,
21.4828026013567));
#47531=CARTESIAN_POINT('Ctrl Pts',(-67.2754510387106,-0.0113687361642878,
21.3716647107886));
#47532=CARTESIAN_POINT('Ctrl Pts',(-66.2435939780275,1.90561821176254,21.2605268202207));
#47533=CARTESIAN_POINT('Ctrl Pts',(-64.0734568674116,2.07828965101229,21.1493889296526));
#47534=CARTESIAN_POINT('Ctrl Pts',(-62.751397400389,0.348720100493122,21.0382510390846));
#47535=CARTESIAN_POINT('Ctrl Pts',(-63.4875082816241,-1.70005762419485,
20.9271131485165));
#47536=CARTESIAN_POINT('Ctrl Pts',(-65.6080205459445,-2.19274288771661,
20.8159752579485));
#47537=CARTESIAN_POINT('Ctrl Pts',(-67.172004426703,-0.678390978958618,
20.7048373673804));
#47538=CARTESIAN_POINT('Ctrl Pts',(-66.7479281658321,1.45690253728,20.5936994768124));
#47539=CARTESIAN_POINT('Ctrl Pts',(-64.7239533601888,2.25867530276305,20.4825615862443));
#47540=CARTESIAN_POINT('Ctrl Pts',(-62.9526472106971,0.993057621792547,
20.3714236956763));
#47541=CARTESIAN_POINT('Ctrl Pts',(-63.0553062695956,-1.18151730175445,
20.2602858051083));
#47542=CARTESIAN_POINT('Ctrl Pts',(-64.9379655634416,-2.27463586868849,
20.1491479145402));
#47543=CARTESIAN_POINT('Ctrl Pts',(-66.8774056759608,-1.285754515064,20.0380100239722));
#47544=CARTESIAN_POINT('Ctrl Pts',(-67.0984350843764,0.879992571076608,
19.9268721334041));
#47545=CARTESIAN_POINT('Ctrl Pts',(-65.3987430610147,2.24027245522917,19.8157342428361));
#47546=CARTESIAN_POINT('Ctrl Pts',(-63.3340769924447,1.55000556572313,19.7045963522681));
#47547=CARTESIAN_POINT('Ctrl Pts',(-62.7942491452433,-0.558999001906807,
19.5934584617));
#47548=CARTESIAN_POINT('Ctrl Pts',(-64.2733700704672,-2.15634544081014,
19.482320571132));
#47549=CARTESIAN_POINT('Ctrl Pts',(-66.4175836106607,-1.7799644445312,19.3711826805639));
#47550=CARTESIAN_POINT('Ctrl Pts',(-67.2642667955629,0.225638194708396,
19.2600447899959));
#47551=CARTESIAN_POINT('Ctrl Pts',(-66.0384409039352,2.02471163506166,19.1489068994278));
#47552=CARTESIAN_POINT('Ctrl Pts',(-63.8621182762245,1.97054355423204,19.0377690088598));
#47553=CARTESIAN_POINT('Ctrl Pts',(-62.727311694737,0.112714610638931,18.9266311182918));
#47554=CARTESIAN_POINT('Ctrl Pts',(-63.6727224930976,-1.84828329429672,
18.8154932277237));
#47555=CARTESIAN_POINT('Ctrl Pts',(-65.8330054458753,-2.11752653902751,
18.7043553371557));
#47556=CARTESIAN_POINT('Ctrl Pts',(-67.2308290671198,-0.448573728190495,
18.5932174465877));
#47557=CARTESIAN_POINT('Ctrl Pts',(-66.5867495439068,1.63096370322549,18.4820795560196));
#47558=CARTESIAN_POINT('Ctrl Pts',(-64.4903001681923,2.21766156069575,18.3709416654516));
#47559=CARTESIAN_POINT('Ctrl Pts',(-62.8603848289206,0.774508641667059,
18.2598037748835));
#47560=CARTESIAN_POINT('Ctrl Pts',(-63.1888835206242,-1.37756082060413,
18.1486658843155));
#47561=CARTESIAN_POINT('Ctrl Pts',(-65.1751176653583,-2.26873324117447,
18.0375279937474));
#47562=CARTESIAN_POINT('Ctrl Pts',(-67.0010646250206,-1.08330839691272,
17.9263901031794));
#47563=CARTESIAN_POINT('Ctrl Pts',(-66.9954144397851,1.09368090859596,17.8152522126113));
#47564=CARTESIAN_POINT('Ctrl Pts',(-65.1633387882755,2.26961167528172,17.7041143220433));
#47565=CARTESIAN_POINT('Ctrl Pts',(-63.1817572914694,1.36814113643509,17.5929764314753));
#47566=CARTESIAN_POINT('Ctrl Pts',(-62.8644339660562,-0.785604500366324,
17.4818385409072));
#47567=CARTESIAN_POINT('Ctrl Pts',(-64.5018184504777,-2.22027742862146,
17.3707006503392));
#47568=CARTESIAN_POINT('Ctrl Pts',(-66.5951941569401,-1.62270524680074,
17.2595627597711));
#47569=CARTESIAN_POINT('Ctrl Pts',(-67.2284705608229,0.460147450145801,
17.1484248692031));
#47570=CARTESIAN_POINT('Ctrl Pts',(-65.8220025878096,2.12182196754698,17.0372869786351));
#47571=CARTESIAN_POINT('Ctrl Pts',(-63.6631463240307,1.84136877495449,16.926149088067));
#47572=CARTESIAN_POINT('Ctrl Pts',(-62.7279273908184,-0.124510139895683,
16.815011197499));
#47573=CARTESIAN_POINT('Ctrl Pts',(-63.8723622838458,-1.97642351165904,
16.7038733069309));
#47574=CARTESIAN_POINT('Ctrl Pts',(-66.0489367667509,-2.01929402903231,
16.5927354163629));
#47575=CARTESIAN_POINT('Ctrl Pts',(-67.2654075312964,-0.213881821283357,
16.4815975257949));
#47576=CARTESIAN_POINT('Ctrl Pts',(-66.4083250909786,1.78729884307681,16.3704596352268));
#47577=CARTESIAN_POINT('Ctrl Pts',(-64.2621867233928,2.15254460700996,16.2593217446588));
#47578=CARTESIAN_POINT('Ctrl Pts',(-62.7913772152625,0.547541880653244,
16.1481838540907));
#47579=CARTESIAN_POINT('Ctrl Pts',(-63.3421451894777,-1.55863213865729,
16.0370459635227));
#47580=CARTESIAN_POINT('Ctrl Pts',(-65.4103664731376,-2.23817248527552,
15.9259080729546));
#47581=CARTESIAN_POINT('Ctrl Pts',(-67.1029746700197,-0.869088173694531,
15.8147701823866));
#47582=CARTESIAN_POINT('Ctrl Pts',(-66.8707063021627,1.2954823997482,15.7036322918186));
#47583=CARTESIAN_POINT('Ctrl Pts',(-64.9261592405154,2.27428324023947,15.5924944012505));
#47584=CARTESIAN_POINT('Ctrl Pts',(-63.0491994637699,1.17140684018709,15.4813565106825));
#47585=CARTESIAN_POINT('Ctrl Pts',(-62.9578295407548,-1.00367152807142,
15.3702186201144));
#47586=CARTESIAN_POINT('Ctrl Pts',(-64.7356814001924,-2.26007795886815,
15.2590807295464));
#47587=CARTESIAN_POINT('Ctrl Pts',(-66.7554670689966,-1.44780941361791,
15.1479428389783));
#47588=CARTESIAN_POINT('Ctrl Pts',(-67.1684538263848,0.689655528488298,
15.0368049484103));
#47589=CARTESIAN_POINT('Ctrl Pts',(-65.5966301942511,2.19587090188638,14.9256670578423));
#47590=CARTESIAN_POINT('Ctrl Pts',(-63.4787041994968,1.69218081976796,14.8145291672742));
#47591=CARTESIAN_POINT('Ctrl Pts',(-62.753237463084,-0.360381723701076,
14.7033912767062));
#47592=CARTESIAN_POINT('Ctrl Pts',(-64.084258037147,-2.08308245831335,14.5922533861381));
#47593=CARTESIAN_POINT('Ctrl Pts',(-66.2534674554613,-1.89911485017137,
14.4811154955701));
#47594=CARTESIAN_POINT('Ctrl Pts',(-67.2753642131315,0.0231354176627139,
14.3699776050021));
#47595=CARTESIAN_POINT('Ctrl Pts',(-66.214593673861,1.92420699596982,14.258839714434));
#47596=CARTESIAN_POINT('Ctrl Pts',(-64.0420930171499,2.06403520705089,14.147701823866));
#47597=CARTESIAN_POINT('Ctrl Pts',(-62.746373011501,0.314618429489875,14.0365639332979));
#47598=CARTESIAN_POINT('Ctrl Pts',(-63.5134282548864,-1.72275201253147,
13.9254260427299));
#47599=CARTESIAN_POINT('Ctrl Pts',(-65.6411497354375,-2.18330798742085,
13.8142881521618));
#47600=CARTESIAN_POINT('Ctrl Pts',(-67.1820389189058,-0.645378055182786,
13.7031502615938));
#47601=CARTESIAN_POINT('Ctrl Pts',(-66.7256447836243,1.4831162854785,13.5920123710258));
#47602=CARTESIAN_POINT('Ctrl Pts',(-64.6898245098097,2.25440988985728,13.4808744804577));
#47603=CARTESIAN_POINT('Ctrl Pts',(-62.9377603166977,0.961596555524325,
13.3697365898897));
#47604=CARTESIAN_POINT('Ctrl Pts',(-63.0735879257438,-1.21014586252811,
13.2585986993216));
#47605=CARTESIAN_POINT('Ctrl Pts',(-64.9720777734537,-2.27668205161229,
13.1474608087536));
#47606=CARTESIAN_POINT('Ctrl Pts',(-66.8974233642155,-1.25434280867415,
13.0363229181856));
#47607=CARTESIAN_POINT('Ctrl Pts',(-67.020379657277,0.184776408472704,12.9622309911402));
#47608=CARTESIAN_POINT('Ctrl Pts',(-66.7638991251268,0.771314832491424,
12.9251850276175));
#47609=CARTESIAN_POINT('Ctrl Pts',(-66.5652001142717,-1.33121980333222,
22.2244449171475));
#47610=CARTESIAN_POINT('Ctrl Pts',(-67.0078623699224,-0.810753527669875,
22.1873989536248));
#47611=CARTESIAN_POINT('Ctrl Pts',(-67.3252008222088,0.697813052277679,
22.1133070265794));
#47612=CARTESIAN_POINT('Ctrl Pts',(-65.6722805558013,2.33526596497651,22.0021691360114));
#47613=CARTESIAN_POINT('Ctrl Pts',(-63.4038010938572,1.82971146538555,21.8910312454434));
#47614=CARTESIAN_POINT('Ctrl Pts',(-62.5964781376417,-0.34790469980557,
21.7798933548753));
#47615=CARTESIAN_POINT('Ctrl Pts',(-63.9890540527047,-2.20843040890227,
21.6687554643073));
#47616=CARTESIAN_POINT('Ctrl Pts',(-66.3069967286646,-2.04687460564973,
21.5576175737392));
#47617=CARTESIAN_POINT('Ctrl Pts',(-67.428612079538,-0.0121339679509515,
21.4464796831712));
#47618=CARTESIAN_POINT('Ctrl Pts',(-66.3273005244664,2.03388573489001,21.3353417926031));
#47619=CARTESIAN_POINT('Ctrl Pts',(-64.0110910734901,2.21817972145312,21.2242039020351));
#47620=CARTESIAN_POINT('Ctrl Pts',(-62.6000435330876,0.372192516572544,
21.1130660114671));
#47621=CARTESIAN_POINT('Ctrl Pts',(-63.385702177301,-1.81448882520009,21.001928120899));
#47622=CARTESIAN_POINT('Ctrl Pts',(-65.648946524169,-2.34033682721966,20.8907902303309));
#47623=CARTESIAN_POINT('Ctrl Pts',(-67.3182024564633,-0.724053604371166,
20.7796523397629));
#47624=CARTESIAN_POINT('Ctrl Pts',(-66.865581542071,1.55496692328426,20.6685144491949));
#47625=CARTESIAN_POINT('Ctrl Pts',(-64.7053726085262,2.41070716562326,20.5573765586268));
#47626=CARTESIAN_POINT('Ctrl Pts',(-62.8148395062834,1.05990051859314,20.4462386680588));
#47627=CARTESIAN_POINT('Ctrl Pts',(-62.9244085658998,-1.2610454553441,20.3351007774907));
#47628=CARTESIAN_POINT('Ctrl Pts',(-64.9337900137556,-2.42774204026717,
20.2239628869227));
#47629=CARTESIAN_POINT('Ctrl Pts',(-67.0037742079544,-1.37229889524426,
20.1128249963547));
#47630=CARTESIAN_POINT('Ctrl Pts',(-67.2396811477566,0.939225037877063,
20.0016871057866));
#47631=CARTESIAN_POINT('Ctrl Pts',(-65.4255825320509,2.3910656189328,19.8905492152186));
#47632=CARTESIAN_POINT('Ctrl Pts',(-63.2219433989572,1.65433673422367,19.7794113246505));
#47633=CARTESIAN_POINT('Ctrl Pts',(-62.6457796370125,-0.596625330707996,
19.6682734340825));
#47634=CARTESIAN_POINT('Ctrl Pts',(-64.2244604721458,-2.30148946126117,
19.5571355435145));
#47635=CARTESIAN_POINT('Ctrl Pts',(-66.5130014322595,-1.89977418876313,
19.4459976529464));
#47636=CARTESIAN_POINT('Ctrl Pts',(-67.4166750228636,0.24082594437386,19.3348597623784));
#47637=CARTESIAN_POINT('Ctrl Pts',(-66.1083385580613,2.16099535909079,19.2237218718103));
#47638=CARTESIAN_POINT('Ctrl Pts',(-63.7855272416617,2.10318121447059,19.1125839812423));
#47639=CARTESIAN_POINT('Ctrl Pts',(-62.5743366140217,0.120301452451048,
19.0014460906743));
#47640=CARTESIAN_POINT('Ctrl Pts',(-63.5833831924642,-1.97269159325921,
18.8903082001062));
#47641=CARTESIAN_POINT('Ctrl Pts',(-65.88907520037,-2.26005765183972,18.7791703095382));
#47642=CARTESIAN_POINT('Ctrl Pts',(-67.3809865945794,-0.478767310881874,
18.6680324189701));
#47643=CARTESIAN_POINT('Ctrl Pts',(-66.6935539565454,1.74074417931049,18.5568945284021));
#47644=CARTESIAN_POINT('Ctrl Pts',(-64.4559921758773,2.36693278080145,18.445756637834));
#47645=CARTESIAN_POINT('Ctrl Pts',(-62.7163669260972,0.826640965179838,
18.334618747266));
#47646=CARTESIAN_POINT('Ctrl Pts',(-63.0669769270206,-1.47028470061622,
18.2234808566979));
#47647=CARTESIAN_POINT('Ctrl Pts',(-65.1869048686148,-2.42144210577607,
18.1123429661299));
#47648=CARTESIAN_POINT('Ctrl Pts',(-67.1357566643205,-1.15622609049766,
18.0012050755618));
#47649=CARTESIAN_POINT('Ctrl Pts',(-67.1297261640456,1.16729677790886,17.8900671849939));
#47650=CARTESIAN_POINT('Ctrl Pts',(-65.1743331530824,2.42237966744963,17.7789292944258));
#47651=CARTESIAN_POINT('Ctrl Pts',(-63.0593710300304,1.46023097571985,17.6677914038578));
#47652=CARTESIAN_POINT('Ctrl Pts',(-62.720688611421,-0.83848368823186,17.5566535132897));
#47653=CARTESIAN_POINT('Ctrl Pts',(-64.4682857559272,-2.36972472329319,
17.4455156227217));
#47654=CARTESIAN_POINT('Ctrl Pts',(-66.7025669780829,-1.73192984461803,
17.3343777321536));
#47655=CARTESIAN_POINT('Ctrl Pts',(-67.3784693367765,0.491120062256299,
17.2232398415856));
#47656=CARTESIAN_POINT('Ctrl Pts',(-65.8773317378418,2.26464220646723,17.1121019510175));
#47657=CARTESIAN_POINT('Ctrl Pts',(-63.5731624496418,1.9653116563091,17.0009640604495));
#47658=CARTESIAN_POINT('Ctrl Pts',(-62.5749937527231,-0.132890941018434,
16.8898261698815));
#47659=CARTESIAN_POINT('Ctrl Pts',(-63.7964607753782,-2.1094569529468,16.7786882793134));
#47660=CARTESIAN_POINT('Ctrl Pts',(-66.119540899393,-2.15521309297246,16.6675503887454));
#47661=CARTESIAN_POINT('Ctrl Pts',(-67.4178925417354,-0.228278247224643,
16.5564124981773));
#47662=CARTESIAN_POINT('Ctrl Pts',(-66.5031197198625,1.9076022670654,16.4452746076093));
#47663=CARTESIAN_POINT('Ctrl Pts',(-64.2125243718594,2.29743279261729,16.3341367170413));
#47664=CARTESIAN_POINT('Ctrl Pts',(-62.6427143968803,0.584397028450654,
16.2229988264732));
#47665=CARTESIAN_POINT('Ctrl Pts',(-63.2305546678621,-1.66354396341758,
16.1118609359052));
#47666=CARTESIAN_POINT('Ctrl Pts',(-65.4379883182475,-2.38882429960344,
16.0007230453371));
#47667=CARTESIAN_POINT('Ctrl Pts',(-67.24452629377,-0.927586663439792,15.8895851547691));
#47668=CARTESIAN_POINT('Ctrl Pts',(-66.996623898036,1.38268156569091,15.7784472642011));
#47669=CARTESIAN_POINT('Ctrl Pts',(-64.9211890049946,2.42736567633039,15.667309373633));
#47670=CARTESIAN_POINT('Ctrl Pts',(-62.9178907098163,1.25025445669176,15.556171483065));
#47671=CARTESIAN_POINT('Ctrl Pts',(-62.8203706599597,-1.07122884891598,
15.4450335924969));
#47672=CARTESIAN_POINT('Ctrl Pts',(-64.7178900651262,-2.41220423477673,
15.3338957019289));
#47673=CARTESIAN_POINT('Ctrl Pts',(-66.8736278902366,-1.54526173974447,
15.2227578113608));
#47674=CARTESIAN_POINT('Ctrl Pts',(-67.3144128645646,0.736076372865376,
15.1116199207928));
#47675=CARTESIAN_POINT('Ctrl Pts',(-65.6367894857436,2.34367538861625,15.0004820302248));
#47676=CARTESIAN_POINT('Ctrl Pts',(-63.3763054907363,1.80608183157382,14.8893441396567));
#47677=CARTESIAN_POINT('Ctrl Pts',(-62.6020074507516,-0.384639085849599,
14.7782062490887));
#47678=CARTESIAN_POINT('Ctrl Pts',(-64.0226192720082,-2.2232951335223,14.6670683585206));
#47679=CARTESIAN_POINT('Ctrl Pts',(-66.3378385875382,-2.02694463079713,
14.5559304679526));
#47680=CARTESIAN_POINT('Ctrl Pts',(-67.4285194097127,0.0246926670119235,
14.4447925773845));
#47681=CARTESIAN_POINT('Ctrl Pts',(-66.2963482043283,2.05372573368661,14.3336546868165));
#47682=CARTESIAN_POINT('Ctrl Pts',(-63.9776161165208,2.20296580816612,14.2225167962485));
#47683=CARTESIAN_POINT('Ctrl Pts',(-62.5946809516312,0.335795455628598,
14.1113789056804));
#47684=CARTESIAN_POINT('Ctrl Pts',(-63.4133668288776,-1.83871077711837,
14.0002410151124));
#47685=CARTESIAN_POINT('Ctrl Pts',(-65.684305645688,-2.33026686199619,13.8891031245443));
#47686=CARTESIAN_POINT('Ctrl Pts',(-67.3289123722387,-0.688818574436933,
13.7779652339763));
#47687=CARTESIAN_POINT('Ctrl Pts',(-66.8417982611818,1.58294512384397,13.6668273434083));
#47688=CARTESIAN_POINT('Ctrl Pts',(-64.6689465387577,2.4061546469661,13.5556894528402));
#47689=CARTESIAN_POINT('Ctrl Pts',(-62.7989505726263,1.02632180198958,13.4445515622722));
#47690=CARTESIAN_POINT('Ctrl Pts',(-62.9439207637896,-1.29160100997124,
13.3334136717041));
#47691=CARTESIAN_POINT('Ctrl Pts',(-64.970198323091,-2.42992595215151,13.2222757811361));
#47692=CARTESIAN_POINT('Ctrl Pts',(-67.0251392906009,-1.33877286094185,
13.111137890568));
#47693=CARTESIAN_POINT('Ctrl Pts',(-67.1563717950601,0.197213743559495,
13.0370459635227));
#47694=CARTESIAN_POINT('Ctrl Pts',(-66.8826275096638,0.823232180103066,
13.));
#47695=CARTESIAN_POINT('Ctrl Pts',(-66.2690708798524,-1.07935865304854,
22.));
#47696=CARTESIAN_POINT('Ctrl Pts',(-66.3144013959117,-1.03707009263694,
22.));
#47697=CARTESIAN_POINT('Ctrl Pts',(-66.3570019677261,-0.992212513379911,
22.));
#47698=CARTESIAN_POINT('Ctrl Pts',(-66.3968740280373,-0.945130914767996,
22.));
#47699=CARTESIAN_POINT('Ctrl Pts',(-66.4393785568392,-0.894940853140404,
22.));
#47700=CARTESIAN_POINT('Ctrl Pts',(-66.4787831170347,-0.842223171995407,
22.));
#47701=CARTESIAN_POINT('Ctrl Pts',(-66.5150606107891,-0.787341095408292,
22.));
#47702=CARTESIAN_POINT('Ctrl Pts',(-66.5468034178243,-0.739319278394567,
22.));
#47703=CARTESIAN_POINT('Ctrl Pts',(-66.5761518212759,-0.689639120404083,
22.));
#47704=CARTESIAN_POINT('Ctrl Pts',(-66.6030647719515,-0.638516396530674,
22.));
#47705=CARTESIAN_POINT('Ctrl Pts',(-66.6165687845846,-0.612864734721154,
22.));
#47706=CARTESIAN_POINT('Ctrl Pts',(-66.6294592637971,-0.586849522995566,
22.));
#47707=CARTESIAN_POINT('Ctrl Pts',(-66.6417286804056,-0.560496177528319,
22.));
#47708=CARTESIAN_POINT('Ctrl Pts',(-66.6473326302021,-0.548459515176508,
22.));
#47709=CARTESIAN_POINT('Ctrl Pts',(-66.6528075873815,-0.536350650682513,
22.));
#47710=CARTESIAN_POINT('Ctrl Pts',(-66.6581443434041,-0.524191916018695,
22.));
#47711=CARTESIAN_POINT('Ctrl Pts',(-66.6850645452328,-0.462859602953103,
22.));
#47712=CARTESIAN_POINT('Ctrl Pts',(-66.708523501665,-0.40015185577214,22.));
#47713=CARTESIAN_POINT('Ctrl Pts',(-66.7284976532658,-0.336426402788346,
22.));
#47714=CARTESIAN_POINT('Ctrl Pts',(-66.7488259022754,-0.271571238854653,
22.));
#47715=CARTESIAN_POINT('Ctrl Pts',(-66.7655452530591,-0.205661124512927,
22.));
#47716=CARTESIAN_POINT('Ctrl Pts',(-66.7785915546302,-0.139036642022517,
22.));
#47717=CARTESIAN_POINT('Ctrl Pts',(-66.7895042319157,-0.0833080914624547,
22.));
#47718=CARTESIAN_POINT('Ctrl Pts',(-66.7978464644169,-0.0270787840751074,
22.));
#47719=CARTESIAN_POINT('Ctrl Pts',(-66.803555876155,0.0294642474108197,
22.));
#47720=CARTESIAN_POINT('Ctrl Pts',(-66.8061865906771,0.055517469857954,
22.));
#47721=CARTESIAN_POINT('Ctrl Pts',(-66.8082580030099,0.0816374113820257,
22.));
#47722=CARTESIAN_POINT('Ctrl Pts',(-66.8097622067333,0.107806177309204,
22.));
#47723=CARTESIAN_POINT('Ctrl Pts',(-66.8104186759519,0.119226830677735,
22.));
#47724=CARTESIAN_POINT('Ctrl Pts',(-66.8109669930214,0.130656542103401,
22.));
#47725=CARTESIAN_POINT('Ctrl Pts',(-66.8114061694303,0.142079754470107,
22.));
#47726=CARTESIAN_POINT('Ctrl Pts',(-66.8141021938362,0.212204785583915,
22.));
#47727=CARTESIAN_POINT('Ctrl Pts',(-66.8126973724676,0.282216215101275,
22.));
#47728=CARTESIAN_POINT('Ctrl Pts',(-66.8071370154229,0.351753309284076,
22.));
#47729=CARTESIAN_POINT('Ctrl Pts',(-66.8021656669832,0.413924339289,22.));
#47730=CARTESIAN_POINT('Ctrl Pts',(-66.7938721956328,0.475717167657645,
22.));
#47731=CARTESIAN_POINT('Ctrl Pts',(-66.7821843766151,0.536886120776816,
22.));
#47732=CARTESIAN_POINT('Ctrl Pts',(-66.7694512323358,0.603525850935252,
22.));
#47733=CARTESIAN_POINT('Ctrl Pts',(-66.7526905137875,0.669425953598385,
22.));
#47734=CARTESIAN_POINT('Ctrl Pts',(-66.7321474941547,0.734372824653822,
22.));
#47735=CARTESIAN_POINT('Ctrl Pts',(-66.7242214209375,0.759431149301981,
22.));
#47736=CARTESIAN_POINT('Ctrl Pts',(-66.71573174826,0.7843475255859,22.));
#47737=CARTESIAN_POINT('Ctrl Pts',(-66.7066905572877,0.809109365072399,
22.));
#47738=CARTESIAN_POINT('Ctrl Pts',(-66.7027243122882,0.819972040392798,
22.));
#47739=CARTESIAN_POINT('Ctrl Pts',(-66.698652038392,0.830804390665135,22.));
#47740=CARTESIAN_POINT('Ctrl Pts',(-66.6944798306887,0.841592845029703,
22.));
#47741=CARTESIAN_POINT('Ctrl Pts',(-66.6692560535916,0.906816244118129,
22.));
#47742=CARTESIAN_POINT('Ctrl Pts',(-66.6403413435161,0.970554427317731,
22.));
#47743=CARTESIAN_POINT('Ctrl Pts',(-66.6080484131291,1.03258856562458,22.));
#47744=CARTESIAN_POINT('Ctrl Pts',(-66.5750071922411,1.09606015652187,22.));
#47745=CARTESIAN_POINT('Ctrl Pts',(-66.5384290749239,1.15774863477848,22.));
#47746=CARTESIAN_POINT('Ctrl Pts',(-66.4985928798434,1.21741589242134,22.));
#47747=CARTESIAN_POINT('Ctrl Pts',(-66.468112635167,1.26306966554027,22.));
#47748=CARTESIAN_POINT('Ctrl Pts',(-66.4357237709971,1.30754017026325,22.));
#47749=CARTESIAN_POINT('Ctrl Pts',(-66.4015316630533,1.350714655026,22.));
#47750=CARTESIAN_POINT('Ctrl Pts',(-66.3802494925467,1.37758772023045,22.));
#47751=CARTESIAN_POINT('Ctrl Pts',(-66.3582683894257,1.40395856102689,22.));
#47752=CARTESIAN_POINT('Ctrl Pts',(-66.335610863513,1.4297983034856,22.));
#47753=CARTESIAN_POINT('Ctrl Pts',(-66.3229007386857,1.44429354685069,22.));
#47754=CARTESIAN_POINT('Ctrl Pts',(-66.3099732536082,1.45862623051551,22.));
#47755=CARTESIAN_POINT('Ctrl Pts',(-66.296856182647,1.47276572504358,22.));
#47756=CARTESIAN_POINT('Ctrl Pts',(-66.2459827546405,1.52760453464138,22.));
#47757=CARTESIAN_POINT('Ctrl Pts',(-66.1922128067209,1.57959843571923,22.));
#47758=CARTESIAN_POINT('Ctrl Pts',(-66.1358313615937,1.62848347077225,22.));
#47759=CARTESIAN_POINT('Ctrl Pts',(-66.093660348142,1.66504747629138,22.));
#47760=CARTESIAN_POINT('Ctrl Pts',(-66.0500271947631,1.69987205103595,22.));
#47761=CARTESIAN_POINT('Ctrl Pts',(-66.0050347650922,1.73283699196269,22.));
#47762=CARTESIAN_POINT('Ctrl Pts',(-65.9909996372478,1.7431202143553,22.));
#47763=CARTESIAN_POINT('Ctrl Pts',(-65.9768321470569,1.75322240061157,22.));
#47764=CARTESIAN_POINT('Ctrl Pts',(-65.9625351771215,1.76313967659916,22.));
#47765=CARTESIAN_POINT('Ctrl Pts',(-65.9487346476095,1.77271259033996,22.));
#47766=CARTESIAN_POINT('Ctrl Pts',(-65.9348204929772,1.7821082799947,22.));
#47767=CARTESIAN_POINT('Ctrl Pts',(-65.9208007361055,1.79132048319868,22.));
#47768=CARTESIAN_POINT('Ctrl Pts',(-65.8578459989061,1.83268723706198,22.));
#47769=CARTESIAN_POINT('Ctrl Pts',(-65.7927339839887,1.87037831023573,22.));
#47770=CARTESIAN_POINT('Ctrl Pts',(-65.7257260556133,1.90411450231801,22.));
#47771=CARTESIAN_POINT('Ctrl Pts',(-65.6744429845673,1.92993376844555,22.));
#47772=CARTESIAN_POINT('Ctrl Pts',(-65.6220484504102,1.95343614609126,22.));
#47773=CARTESIAN_POINT('Ctrl Pts',(-65.5686456989049,1.97448116510365,22.));
#47774=CARTESIAN_POINT('Ctrl Pts',(-65.5562524015237,1.97936513028633,22.));
#47775=CARTESIAN_POINT('Ctrl Pts',(-65.54380476008,1.98411668136774,22.));
#47776=CARTESIAN_POINT('Ctrl Pts',(-65.531304687333,1.98873639975131,22.));
#47777=CARTESIAN_POINT('Ctrl Pts',(-63.3326792503596,0.00130047270867312,
20.8714803633902));
#47778=CARTESIAN_POINT('Ctrl Pts',(-63.3319477300267,0.0865458945944494,
20.8771939403667));
#47779=CARTESIAN_POINT('Ctrl Pts',(-63.3379207823453,0.171688456696982,
20.8829075173431));
#47780=CARTESIAN_POINT('Ctrl Pts',(-63.3509549142486,0.255735893547228,
20.8886210943196));
#47781=CARTESIAN_POINT('Ctrl Pts',(-63.4354662417459,0.800686682266395,
20.9256670578423));
#47782=CARTESIAN_POINT('Ctrl Pts',(-63.8168273485002,1.29959809619851,20.9627130213649));
#47783=CARTESIAN_POINT('Ctrl Pts',(-64.3205066401932,1.52414941239406,20.9997589848876));
#47784=CARTESIAN_POINT('Ctrl Pts',(-64.8241859318862,1.74870072858962,21.0368049484103));
#47785=CARTESIAN_POINT('Ctrl Pts',(-65.4501834085179,1.69889194704861,21.073850911933));
#47786=CARTESIAN_POINT('Ctrl Pts',(-65.9120068254848,1.39750064992835,21.1108968754557));
#47787=CARTESIAN_POINT('Ctrl Pts',(-66.3738302424517,1.09610935280808,21.1479428389783));
#47788=CARTESIAN_POINT('Ctrl Pts',(-66.6714795997537,0.543135540108559,
21.184988802501));
#47789=CARTESIAN_POINT('Ctrl Pts',(-66.6687358658196,-0.0083140869619841,
21.2220347660237));
#47790=CARTESIAN_POINT('Ctrl Pts',(-66.6659921318856,-0.55976371403253,
21.2590807295464));
#47791=CARTESIAN_POINT('Ctrl Pts',(-66.3628553067155,-1.1096891554741,21.2961266930691));
#47792=CARTESIAN_POINT('Ctrl Pts',(-65.898053938122,-1.40648356441475,21.3331726565917));
#47793=CARTESIAN_POINT('Ctrl Pts',(-65.4332525695286,-1.70327797335541,
21.3702186201144));
#47794=CARTESIAN_POINT('Ctrl Pts',(-64.8067866575118,-1.74694134979516,
21.4072645836371));
#47795=CARTESIAN_POINT('Ctrl Pts',(-64.3053692934656,-1.51735268425301,
21.4443105471598));
#47796=CARTESIAN_POINT('Ctrl Pts',(-63.8039519294193,-1.28776401871086,
21.4813565106825));
#47797=CARTESIAN_POINT('Ctrl Pts',(-63.4275831133436,-0.784923311186817,
21.5184024742051));
#47798=CARTESIAN_POINT('Ctrl Pts',(-63.3484955171689,-0.239232889597532,
21.5554484377278));
#47799=CARTESIAN_POINT('Ctrl Pts',(-63.337086928647,-0.160515647180253,
21.5607924129486));
#47800=CARTESIAN_POINT('Ctrl Pts',(-63.3318644062264,-0.0809067535388516,
21.5661363881694));
#47801=CARTESIAN_POINT('Ctrl Pts',(-63.3325282901756,-0.00121307831917494,
21.5714803633902));
#47802=CARTESIAN_POINT('Ctrl Pts',(-64.4698297828114,1.98517432567173,22.));
#47803=CARTESIAN_POINT('Ctrl Pts',(-63.8097120902545,1.8088801151799,21.9629540364773));
#47804=CARTESIAN_POINT('Ctrl Pts',(-62.6906509614045,0.748610048502907,
21.888862109432));
#47805=CARTESIAN_POINT('Ctrl Pts',(-63.1187889329782,-1.53833553624065,
21.7777242188639));
#47806=CARTESIAN_POINT('Ctrl Pts',(-65.2721300366129,-2.41280623887488,
21.6665863282959));
#47807=CARTESIAN_POINT('Ctrl Pts',(-67.1747422685441,-1.08094901338604,
21.5554484377278));
#47808=CARTESIAN_POINT('Ctrl Pts',(-67.0876157148515,1.24138505016238,21.4443105471598));
#47809=CARTESIAN_POINT('Ctrl Pts',(-65.0892538486774,2.42692553227055,21.3331726565917));
#47810=CARTESIAN_POINT('Ctrl Pts',(-63.0094071033202,1.39134559511319,21.2220347660237));
#47811=CARTESIAN_POINT('Ctrl Pts',(-62.7514666617416,-0.917885875238364,
21.1108968754557));
#47812=CARTESIAN_POINT('Ctrl Pts',(-64.5516876929394,-2.38689686810909,
20.9997589848876));
#47813=CARTESIAN_POINT('Ctrl Pts',(-66.7622271403759,-1.67118893435551,
20.8886210943196));
#47814=CARTESIAN_POINT('Ctrl Pts',(-67.3597936726881,0.574194749175807,
20.7774832037516));
#47815=CARTESIAN_POINT('Ctrl Pts',(-65.7974074532359,2.29400261230211,20.6663453131835));
#47816=CARTESIAN_POINT('Ctrl Pts',(-63.5051485972519,1.91408833219885,20.5552074226155));
#47817=CARTESIAN_POINT('Ctrl Pts',(-62.5811424445442,-0.217814955653705,
20.4440695320474));
#47818=CARTESIAN_POINT('Ctrl Pts',(-63.8711449203827,-2.15034861017486,
20.3329316414794));
#47819=CARTESIAN_POINT('Ctrl Pts',(-66.1944008109328,-2.11464436694831,
20.2217937509113));
#47820=CARTESIAN_POINT('Ctrl Pts',(-67.4244083164919,-0.143381864737536,
20.1106558603433));
#47821=CARTESIAN_POINT('Ctrl Pts',(-66.4353272830534,1.95911953903996,19.9995179697752));
#47822=CARTESIAN_POINT('Ctrl Pts',(-64.132474966303,2.26841668404626,19.8883800792072));
#47823=CARTESIAN_POINT('Ctrl Pts',(-62.6236781227743,0.50140627563106,19.7772421886392));
#47824=CARTESIAN_POINT('Ctrl Pts',(-63.2899556571721,-1.72454696459255,
19.6661042980711));
#47825=CARTESIAN_POINT('Ctrl Pts',(-65.5214561645339,-2.37200281981328,
19.5549664075031));
#47826=CARTESIAN_POINT('Ctrl Pts',(-67.2756619344365,-0.848337588988209,
19.443828516935));
#47827=CARTESIAN_POINT('Ctrl Pts',(-66.9469285261459,1.45182065545647,19.332690626367));
#47828=CARTESIAN_POINT('Ctrl Pts',(-64.8361493591312,2.42311099039749,19.221552735799));
#47829=CARTESIAN_POINT('Ctrl Pts',(-62.8753445414284,1.17650035527427,19.1104148452309));
#47830=CARTESIAN_POINT('Ctrl Pts',(-62.8592609604237,-1.14697439714762,
18.9992769546629));
#47831=CARTESIAN_POINT('Ctrl Pts',(-64.8026200998564,-2.42061047643985,
18.8881390640948));
#47832=CARTESIAN_POINT('Ctrl Pts',(-66.9266433003906,-1.4786343349792,18.7770011735268));
#47833=CARTESIAN_POINT('Ctrl Pts',(-67.2871880384261,0.816752582102682,
18.6658632829587));
#47834=CARTESIAN_POINT('Ctrl Pts',(-65.5542436264288,2.36455659820144,18.5547253923907));
#47835=CARTESIAN_POINT('Ctrl Pts',(-63.3139937376034,1.74805514406081,18.4435875018227));
#47836=CARTESIAN_POINT('Ctrl Pts',(-62.6169645013648,-0.468461007727317,
18.3324496112546));
#47837=CARTESIAN_POINT('Ctrl Pts',(-64.1011546824859,-2.25618948643599,
18.2213117206866));
#47838=CARTESIAN_POINT('Ctrl Pts',(-66.4080681763277,-1.97880214127948,
18.1101738301185));
#47839=CARTESIAN_POINT('Ctrl Pts',(-67.4261608997972,0.109805244932097,
17.9990359395505));
#47840=CARTESIAN_POINT('Ctrl Pts',(-66.2235610371465,2.09790664518148,17.8878980489825));
#47841=CARTESIAN_POINT('Ctrl Pts',(-63.9010218810697,2.16577030121657,17.7767601584144));
#47842=CARTESIAN_POINT('Ctrl Pts',(-62.5843898605093,0.251279839042483,
17.6656222678464));
#47843=CARTESIAN_POINT('Ctrl Pts',(-63.478793195507,-1.89320990951441,17.5544843772783));
#47844=CARTESIAN_POINT('Ctrl Pts',(-65.7655743703156,-2.30482315743207,
17.4433464867103));
#47845=CARTESIAN_POINT('Ctrl Pts',(-67.3516166417705,-0.606805630879782,
17.3322085961422));
#47846=CARTESIAN_POINT('Ctrl Pts',(-66.7851975318663,1.6466279712607,17.2210707055742));
#47847=CARTESIAN_POINT('Ctrl Pts',(-64.5847668755277,2.39288431727496,17.1099328150062));
#47848=CARTESIAN_POINT('Ctrl Pts',(-62.7644038070828,0.948906510533639,
16.9987949244381));
#47849=CARTESIAN_POINT('Ctrl Pts',(-62.9903072873999,-1.36361618663093,
16.8876570338701));
#47850=CARTESIAN_POINT('Ctrl Pts',(-65.0557052990257,-2.42800552371271,
16.776519143302));
#47851=CARTESIAN_POINT('Ctrl Pts',(-67.0701156187118,-1.27001386948507,
16.665381252734));
#47852=CARTESIAN_POINT('Ctrl Pts',(-67.1897256358837,1.05043588241969,16.5542433621659));
#47853=CARTESIAN_POINT('Ctrl Pts',(-65.3050549453524,2.4094097583915,16.4431054715979));
#47854=CARTESIAN_POINT('Ctrl Pts',(-63.141164003784,1.56302355794459,16.3319675810298));
#47855=CARTESIAN_POINT('Ctrl Pts',(-62.6786867301813,-0.714015830985951,
16.2208296904619));
#47856=CARTESIAN_POINT('Ctrl Pts',(-64.3409338179361,-2.33750843231644,
16.1096917998938));
#47857=CARTESIAN_POINT('Ctrl Pts',(-66.6064316564341,-1.82145305641562,
15.9985539093258));
#47858=CARTESIAN_POINT('Ctrl Pts',(-67.401544381661,0.361798958737847,15.8874160187577));
#47859=CARTESIAN_POINT('Ctrl Pts',(-65.9984962989145,2.21389228381421,15.7762781281897));
#47860=CARTESIAN_POINT('Ctrl Pts',(-63.6815132301988,2.03958489439844,15.6651402376216));
#47861=CARTESIAN_POINT('Ctrl Pts',(-62.5713560542506,-0.00157767958229344,
15.5540023470536));
#47862=CARTESIAN_POINT('Ctrl Pts',(-63.6841642251148,-2.04129618504103,
15.4428644564855));
#47863=CARTESIAN_POINT('Ctrl Pts',(-66.0013718021885,-2.21259314346662,
15.3317265659175));
#47864=CARTESIAN_POINT('Ctrl Pts',(-67.4020124146433,-0.358678503164364,
15.2205886753494));
#47865=CARTESIAN_POINT('Ctrl Pts',(-66.6040638188323,1.82353863480769,15.1094507847814));
#47866=CARTESIAN_POINT('Ctrl Pts',(-64.3378974271891,2.33665018787606,14.9983128942134));
#47867=CARTESIAN_POINT('Ctrl Pts',(-62.6777610116056,0.710999308952895,
14.8871750036453));
#47868=CARTESIAN_POINT('Ctrl Pts',(-63.1431963129713,-1.56543726976266,
14.7760371130773));
#47869=CARTESIAN_POINT('Ctrl Pts',(-65.3081850174459,-2.40901142364103,
14.6648992225093));
#47870=CARTESIAN_POINT('Ctrl Pts',(-67.1910886177016,-1.04758997952521,
14.5537613319412));
#47871=CARTESIAN_POINT('Ctrl Pts',(-67.068463685159,1.27270221153157,14.4426234413732));
#47872=CARTESIAN_POINT('Ctrl Pts',(-65.0525510239567,2.42807611461694,14.3314855508051));
#47873=CARTESIAN_POINT('Ctrl Pts',(-62.9885367426501,1.36100346218852,14.2203476602371));
#47874=CARTESIAN_POINT('Ctrl Pts',(-62.7656397187534,-0.951809206360656,
14.109209769669));
#47875=CARTESIAN_POINT('Ctrl Pts',(-64.5878737813476,-2.39342385873017,
13.998071879101));
#47876=CARTESIAN_POINT('Ctrl Pts',(-66.7873400138256,-1.64430308142018,
13.8869339885329));
#47877=CARTESIAN_POINT('Ctrl Pts',(-67.3508170614469,0.60985221755875,13.7757960979649));
#47878=CARTESIAN_POINT('Ctrl Pts',(-65.7625975239189,2.30583209920717,13.6646582073969));
#47879=CARTESIAN_POINT('Ctrl Pts',(-63.4762984963492,1.89119971793715,13.5535203168288));
#47880=CARTESIAN_POINT('Ctrl Pts',(-62.5847903309572,-0.254354168931198,
13.4423824262608));
#47881=CARTESIAN_POINT('Ctrl Pts',(-63.9036938704104,-2.16732302296763,
13.3312445356927));
#47882=CARTESIAN_POINT('Ctrl Pts',(-66.2265689546786,-2.09606376419021,
13.2201066451247));
#47883=CARTESIAN_POINT('Ctrl Pts',(-67.4257384694328,-0.107152139943094,
13.1089687545567));
#47884=CARTESIAN_POINT('Ctrl Pts',(-66.4066260077932,1.98162422647334,12.9978308639886));
#47885=CARTESIAN_POINT('Ctrl Pts',(-64.0958295620755,2.25299485262721,12.8866929734206));
#47886=CARTESIAN_POINT('Ctrl Pts',(-63.1142456563632,1.06431345694515,12.8126010463752));
#47887=CARTESIAN_POINT('Ctrl Pts',(-62.9833241385535,0.393720754290225,
12.7755550828525));
#47888=CARTESIAN_POINT('Ctrl Pts',(-64.5032651029123,1.85997880000277,22.0748149723825));
#47889=CARTESIAN_POINT('Ctrl Pts',(-63.8847779011663,1.69480262890401,22.0377690088598));
#47890=CARTESIAN_POINT('Ctrl Pts',(-62.8362906481067,0.701398764671866,
21.9636770818144));
#47891=CARTESIAN_POINT('Ctrl Pts',(-63.2374279891983,-1.44132001290634,
21.8525391912464));
#47892=CARTESIAN_POINT('Ctrl Pts',(-65.2549680863783,-2.26064199742415,
21.7414013006783));
#47893=CARTESIAN_POINT('Ctrl Pts',(-67.0375915921608,-1.01277868788759,
21.6302634101104));
#47894=CARTESIAN_POINT('Ctrl Pts',(-66.9559596968202,1.16309678504487,21.5191255195423));
#47895=CARTESIAN_POINT('Ctrl Pts',(-65.0836250319239,2.27387085397713,21.4079876289743));
#47896=CARTESIAN_POINT('Ctrl Pts',(-63.1349443525531,1.30360002994302,21.2968497384062));
#47897=CARTESIAN_POINT('Ctrl Pts',(-62.8932709907757,-0.859999168177664,
21.1857118478382));
#47898=CARTESIAN_POINT('Ctrl Pts',(-64.5799606230396,-2.23636660774045,
21.0745739572701));
#47899=CARTESIAN_POINT('Ctrl Pts',(-66.6510918358667,-1.56579497755124,
20.9634360667021));
#47900=CARTESIAN_POINT('Ctrl Pts',(-67.2109726822582,0.537983010725535,
20.8522981761341));
#47901=CARTESIAN_POINT('Ctrl Pts',(-65.7471187486173,2.14933075189209,20.741160285566));
#47902=CARTESIAN_POINT('Ctrl Pts',(-63.5994217826059,1.79337586285671,20.630022394998));
#47903=CARTESIAN_POINT('Ctrl Pts',(-62.73368831382,-0.204078399866647,20.5188845044299));
#47904=CARTESIAN_POINT('Ctrl Pts',(-63.9423364541786,-2.01473632608426,
20.4077466138619));
#47905=CARTESIAN_POINT('Ctrl Pts',(-66.1190756188575,-1.98128378007219,
20.2966087232938));
#47906=CARTESIAN_POINT('Ctrl Pts',(-67.2715123870543,-0.134339450832078,
20.1854708327258));
#47907=CARTESIAN_POINT('Ctrl Pts',(-66.3448080015046,1.83556716514179,20.0743329421578));
#47908=CARTESIAN_POINT('Ctrl Pts',(-64.1871856540346,2.12535840673386,19.9631950515897));
#47909=CARTESIAN_POINT('Ctrl Pts',(-62.7735414686431,0.469784960847985,
19.8520571610217));
#47910=CARTESIAN_POINT('Ctrl Pts',(-63.3978000402315,-1.61578796998893,
19.7409192704536));
#47911=CARTESIAN_POINT('Ctrl Pts',(-65.4885703983884,-2.2224118564029,19.6297813798856));
#47912=CARTESIAN_POINT('Ctrl Pts',(-67.1321467335585,-0.794836962355745,
19.5186434893175));
#47913=CARTESIAN_POINT('Ctrl Pts',(-66.8241449815883,1.3602612151663,19.4075055987495));
#47914=CARTESIAN_POINT('Ctrl Pts',(-64.8464826416291,2.27029687716117,19.2963677081814));
#47915=CARTESIAN_POINT('Ctrl Pts',(-63.0093364803535,1.10230406000512,19.1852298176134));
#47916=CARTESIAN_POINT('Ctrl Pts',(-62.9942672144912,-1.07464016396578,
19.0740919270454));
#47917=CARTESIAN_POINT('Ctrl Pts',(-64.8150679136506,-2.26795405875465,
18.9629540364773));
#47918=CARTESIAN_POINT('Ctrl Pts',(-66.8051390487741,-1.38538388314432,
18.8518161459093));
#47919=CARTESIAN_POINT('Ctrl Pts',(-67.1429459408574,0.765243871993194,
18.7406782553413));
#47920=CARTESIAN_POINT('Ctrl Pts',(-65.5192901106281,2.21543523265805,18.6295403647732));
#47921=CARTESIAN_POINT('Ctrl Pts',(-63.4203221529835,1.63781360011733,18.5184024742052));
#47922=CARTESIAN_POINT('Ctrl Pts',(-62.7672512434818,-0.438917394675609,
18.4072645836371));
#47923=CARTESIAN_POINT('Ctrl Pts',(-64.1578405919126,-2.11390232046251,
18.2961266930691));
#47924=CARTESIAN_POINT('Ctrl Pts',(-66.3192679973039,-1.85400847904605,
18.184988802501));
#47925=CARTESIAN_POINT('Ctrl Pts',(-67.2731544432459,0.102880349126872,
18.073850911933));
#47926=CARTESIAN_POINT('Ctrl Pts',(-66.1463968479604,1.96560162700177,17.9627130213649));
#47927=CARTESIAN_POINT('Ctrl Pts',(-63.9703292167121,2.02918544424322,17.8515751307969));
#47928=CARTESIAN_POINT('Ctrl Pts',(-62.7367309306682,0.235432811840836,
17.7404372402289));
#47929=CARTESIAN_POINT('Ctrl Pts',(-63.5747284910006,-1.77381414322918,
17.6292993496608));
#47930=CARTESIAN_POINT('Ctrl Pts',(-65.7172932271985,-2.15946889658092,
17.5181614590928));
#47931=CARTESIAN_POINT('Ctrl Pts',(-67.2033113378831,-0.568537278849199,
17.4070235685247));
#47932=CARTESIAN_POINT('Ctrl Pts',(-66.6726135937532,1.54278295786449,17.2958856779567));
#47933=CARTESIAN_POINT('Ctrl Pts',(-64.6109536585329,2.24197645689606,17.1847477873887));
#47934=CARTESIAN_POINT('Ctrl Pts',(-62.9053922517429,0.889063479188389,
17.0736098968206));
#47935=CARTESIAN_POINT('Ctrl Pts',(-63.1170490714002,-1.27761938368608,
16.9624720062526));
#47936=CARTESIAN_POINT('Ctrl Pts',(-65.0521922301209,-2.27488273548328,
16.8513341156845));
#47937=CARTESIAN_POINT('Ctrl Pts',(-66.9395632487115,-1.18992012056796,
16.7401962251165));
#47938=CARTESIAN_POINT('Ctrl Pts',(-67.0516300296139,0.984189875315718,
16.6290583345485));
#47939=CARTESIAN_POINT('Ctrl Pts',(-65.2858165773424,2.2574597168496,16.5179204439804));
#47940=CARTESIAN_POINT('Ctrl Pts',(-63.2583919704513,1.4644510782186,16.4067825534124));
#47941=CARTESIAN_POINT('Ctrl Pts',(-62.8250809441801,-0.668986240314613,
16.2956446628443));
#47942=CARTESIAN_POINT('Ctrl Pts',(-64.3824979949693,-2.19009286626007,
16.1845067722763));
#47943=CARTESIAN_POINT('Ctrl Pts',(-66.5051216338947,-1.70658265439078,
16.0733688817082));
#47944=CARTESIAN_POINT('Ctrl Pts',(-67.2500903721106,0.338982015036773,
15.9622309911402));
#47945=CARTESIAN_POINT('Ctrl Pts',(-65.9355258749046,2.07427260172267,15.8510931005721));
#47946=CARTESIAN_POINT('Ctrl Pts',(-63.7646639349497,1.91095795232156,15.7399552100041));
#47947=CARTESIAN_POINT('Ctrl Pts',(-62.7245191047287,-0.00147818281664962,
15.6288173194361));
#47948=CARTESIAN_POINT('Ctrl Pts',(-63.7671477441945,-1.91256131998288,
15.517679428868));
#47949=CARTESIAN_POINT('Ctrl Pts',(-65.9382200338304,-2.07305539199277,
15.4065415383));
#47950=CARTESIAN_POINT('Ctrl Pts',(-67.2505288884734,-0.336058351790693,
15.2954036477319));
#47951=CARTESIAN_POINT('Ctrl Pts',(-66.5029031245757,1.70853670524911,15.1842657571639));
#47952=CARTESIAN_POINT('Ctrl Pts',(-64.3796530949801,2.18928874722443,15.0731278665959));
#47953=CARTESIAN_POINT('Ctrl Pts',(-62.8242136062828,0.666159956013699,
14.9619899760278));
#47954=CARTESIAN_POINT('Ctrl Pts',(-63.2602961115408,-1.46671256868463,
14.8508520854598));
#47955=CARTESIAN_POINT('Ctrl Pts',(-65.2887492506402,-2.25708650318186,
14.7397141948917));
#47956=CARTESIAN_POINT('Ctrl Pts',(-67.0529070546353,-0.981523450013844,
14.6285763043237));
#47957=CARTESIAN_POINT('Ctrl Pts',(-66.93801549477,1.19243892163695,14.5174384137556));
#47958=CARTESIAN_POINT('Ctrl Pts',(-65.0492368802144,2.2749488745541,14.4063005231876));
#47959=CARTESIAN_POINT('Ctrl Pts',(-63.115390186507,1.27517143137767,14.2951626326196));
#47960=CARTESIAN_POINT('Ctrl Pts',(-62.9065502203286,-0.89178311576201,
14.1840247420515));
#47961=CARTESIAN_POINT('Ctrl Pts',(-64.6138646265439,-2.24248197203165,
14.0728868514835));
#47962=CARTESIAN_POINT('Ctrl Pts',(-66.6746209595408,-1.54060468779531,
13.9617489609154));
#47963=CARTESIAN_POINT('Ctrl Pts',(-67.2025621832966,0.571391731761459,
13.8506110703474));
#47964=CARTESIAN_POINT('Ctrl Pts',(-65.7145041163797,2.16041420918538,13.7394731797794));
#47965=CARTESIAN_POINT('Ctrl Pts',(-63.5723911206821,1.77193072489695,13.6283352892113));
#47966=CARTESIAN_POINT('Ctrl Pts',(-62.7371061453451,-0.238313258330233,
13.5171973986433));
#47967=CARTESIAN_POINT('Ctrl Pts',(-63.9728326963629,-2.03064024320064,
13.4060595080752));
#47968=CARTESIAN_POINT('Ctrl Pts',(-66.1492150704054,-1.9638749677707,13.2949216175072));
#47969=CARTESIAN_POINT('Ctrl Pts',(-67.2727586535603,-0.100394562881346,
13.1837837269391));
#47970=CARTESIAN_POINT('Ctrl Pts',(-66.3179167794963,1.85665258871667,13.0726458363711));
#47971=CARTESIAN_POINT('Ctrl Pts',(-64.1528513015804,2.11090915705048,12.9615079458031));
#47972=CARTESIAN_POINT('Ctrl Pts',(-63.2331712354829,0.997192257060744,
12.8874160187577));
#47973=CARTESIAN_POINT('Ctrl Pts',(-63.1105063166185,0.368890654402919,
12.850370055235));
#47974=CARTESIAN_POINT('Ctrl Pts',(-64.5367004230132,1.73478327433381,22.149629944765));
#47975=CARTESIAN_POINT('Ctrl Pts',(-63.9598437120782,1.58072514262811,22.1125839812423));
#47976=CARTESIAN_POINT('Ctrl Pts',(-62.9819303348089,0.654187480840823,
22.0384920541969));
#47977=CARTESIAN_POINT('Ctrl Pts',(-63.3560670454183,-1.34430448957202,
21.9273541636289));
#47978=CARTESIAN_POINT('Ctrl Pts',(-65.2378061361438,-2.10847775597343,
21.8162162730608));
#47979=CARTESIAN_POINT('Ctrl Pts',(-66.9004409157773,-0.944608362389142,
21.7050783824928));
#47980=CARTESIAN_POINT('Ctrl Pts',(-66.8243036787891,1.08480851992736,21.5939404919248));
#47981=CARTESIAN_POINT('Ctrl Pts',(-65.0779962151703,2.12081617568372,21.4828026013567));
#47982=CARTESIAN_POINT('Ctrl Pts',(-63.260481601786,1.21585446477284,21.3716647107887));
#47983=CARTESIAN_POINT('Ctrl Pts',(-63.0350753198097,-0.802112461116964,
21.2605268202206));
#47984=CARTESIAN_POINT('Ctrl Pts',(-64.6082335531397,-2.08583634737181,
21.1493889296526));
#47985=CARTESIAN_POINT('Ctrl Pts',(-66.5399565313575,-1.46040102074697,
21.0382510390845));
#47986=CARTESIAN_POINT('Ctrl Pts',(-67.0621516918281,0.501771272275262,
20.9271131485165));
#47987=CARTESIAN_POINT('Ctrl Pts',(-65.6968300439987,2.00465889148208,20.8159752579485));
#47988=CARTESIAN_POINT('Ctrl Pts',(-63.6936949679598,1.67266339351457,20.7048373673804));
#47989=CARTESIAN_POINT('Ctrl Pts',(-62.8862341830959,-0.190341844079587,
20.5936994768124));
#47990=CARTESIAN_POINT('Ctrl Pts',(-64.0135279879744,-1.87912404199366,
20.4825615862443));
#47991=CARTESIAN_POINT('Ctrl Pts',(-66.0437504267822,-1.84792319319606,
20.3714236956763));
#47992=CARTESIAN_POINT('Ctrl Pts',(-67.1186164576166,-0.125297036926618,
20.2602858051083));
#47993=CARTESIAN_POINT('Ctrl Pts',(-66.2542887199558,1.71201479124362,20.1491479145402));
#47994=CARTESIAN_POINT('Ctrl Pts',(-64.2418963417663,1.98230012942146,20.0380100239722));
#47995=CARTESIAN_POINT('Ctrl Pts',(-62.9234048145118,0.438163646064908,
19.9268721334041));
#47996=CARTESIAN_POINT('Ctrl Pts',(-63.505644423291,-1.50702897538531,19.8157342428361));
#47997=CARTESIAN_POINT('Ctrl Pts',(-65.4556846322429,-2.07282089299252,
19.7045963522681));
#47998=CARTESIAN_POINT('Ctrl Pts',(-66.9886315326805,-0.741336335723279,
19.5934584617));
#47999=CARTESIAN_POINT('Ctrl Pts',(-66.7013614370307,1.26870177487613,19.482320571132));
#48000=CARTESIAN_POINT('Ctrl Pts',(-64.856815924127,2.11748276392484,19.3711826805639));
#48001=CARTESIAN_POINT('Ctrl Pts',(-63.1433284192787,1.02810776473597,19.2600447899959));
#48002=CARTESIAN_POINT('Ctrl Pts',(-63.1292734685587,-1.00230593078394,
19.1489068994279));
#48003=CARTESIAN_POINT('Ctrl Pts',(-64.8275157274446,-2.11529764106946,
19.0377690088598));
#48004=CARTESIAN_POINT('Ctrl Pts',(-66.6836347971578,-1.29213343130944,
18.9266311182918));
#48005=CARTESIAN_POINT('Ctrl Pts',(-66.9987038432886,0.713735161883704,
18.8154932277237));
#48006=CARTESIAN_POINT('Ctrl Pts',(-65.4843365948275,2.06631386711467,18.7043553371557));
#48007=CARTESIAN_POINT('Ctrl Pts',(-63.5266505683636,1.52757205617384,18.5932174465876));
#48008=CARTESIAN_POINT('Ctrl Pts',(-62.9175379855987,-0.409373781623898,
18.4820795560196));
#48009=CARTESIAN_POINT('Ctrl Pts',(-64.2145265013393,-1.97161515448904,
18.3709416654516));
#48010=CARTESIAN_POINT('Ctrl Pts',(-66.2304678182801,-1.72921481681262,
18.2598037748835));
#48011=CARTESIAN_POINT('Ctrl Pts',(-67.1201479866946,0.0959554533216485,
18.1486658843155));
#48012=CARTESIAN_POINT('Ctrl Pts',(-66.0692326587742,1.83329660882205,18.0375279937474));
#48013=CARTESIAN_POINT('Ctrl Pts',(-64.0396365523547,1.89260058726988,17.9263901031794));
#48014=CARTESIAN_POINT('Ctrl Pts',(-62.8890720008271,0.219585784639187,
17.8152522126113));
#48015=CARTESIAN_POINT('Ctrl Pts',(-63.6706637864943,-1.65441837694395,
17.7041143220433));
#48016=CARTESIAN_POINT('Ctrl Pts',(-65.6690120840812,-2.01411463572976,
17.5929764314753));
#48017=CARTESIAN_POINT('Ctrl Pts',(-67.0550060339956,-0.530268926818617,
17.4818385409072));
#48018=CARTESIAN_POINT('Ctrl Pts',(-66.5600296556403,1.43893794446827,17.3707006503392));
#48019=CARTESIAN_POINT('Ctrl Pts',(-64.6371404415378,2.09106859651716,17.2595627597711));
#48020=CARTESIAN_POINT('Ctrl Pts',(-63.0463806964032,0.82922044784314,17.1484248692031));
#48021=CARTESIAN_POINT('Ctrl Pts',(-63.2437908554003,-1.19162258074124,
17.0372869786351));
#48022=CARTESIAN_POINT('Ctrl Pts',(-65.0486791612162,-2.12175994725384,
16.926149088067));
#48023=CARTESIAN_POINT('Ctrl Pts',(-66.8090108787112,-1.10982637165084,
16.815011197499));
#48024=CARTESIAN_POINT('Ctrl Pts',(-66.9135344233438,0.917943868211746,
16.7038733069309));
#48025=CARTESIAN_POINT('Ctrl Pts',(-65.2665782093324,2.10550967530769,16.5927354163629));
#48026=CARTESIAN_POINT('Ctrl Pts',(-63.3756199371186,1.3658785984926,16.4815975257949));
#48027=CARTESIAN_POINT('Ctrl Pts',(-62.9714751581789,-0.623956649643275,
16.3704596352268));
#48028=CARTESIAN_POINT('Ctrl Pts',(-64.4240621720026,-2.04267730020369,
16.2593217446588));
#48029=CARTESIAN_POINT('Ctrl Pts',(-66.4038116113553,-1.59171225236595,
16.1481838540907));
#48030=CARTESIAN_POINT('Ctrl Pts',(-67.0986363625603,0.316165071335702,
16.0370459635227));
#48031=CARTESIAN_POINT('Ctrl Pts',(-65.8725554508947,1.93465291963113,15.9259080729547));
#48032=CARTESIAN_POINT('Ctrl Pts',(-63.8478146397005,1.78233101024468,15.8147701823866));
#48033=CARTESIAN_POINT('Ctrl Pts',(-62.8776821552069,-0.00137868605100532,
15.7036322918186));
#48034=CARTESIAN_POINT('Ctrl Pts',(-63.8501312632741,-1.78382645492473,
15.5924944012505));
#48035=CARTESIAN_POINT('Ctrl Pts',(-65.8750682654724,-1.93351764051893,
15.4813565106825));
#48036=CARTESIAN_POINT('Ctrl Pts',(-67.0990453623036,-0.313438200417021,
15.3702186201144));
#48037=CARTESIAN_POINT('Ctrl Pts',(-66.401742430319,1.59353477569053,15.2590807295464));
#48038=CARTESIAN_POINT('Ctrl Pts',(-64.4214087627711,2.0419273065728,15.1479428389783));
#48039=CARTESIAN_POINT('Ctrl Pts',(-62.9706662009597,0.621320603074505,
15.0368049484103));
#48040=CARTESIAN_POINT('Ctrl Pts',(-63.3773959101104,-1.3679878676066,14.9256670578422));
#48041=CARTESIAN_POINT('Ctrl Pts',(-65.2693134838344,-2.10516158272268,
14.8145291672742));
#48042=CARTESIAN_POINT('Ctrl Pts',(-66.914725491569,-0.915456920502479,
14.7033912767062));
#48043=CARTESIAN_POINT('Ctrl Pts',(-66.8075673043809,1.11217563174233,14.5922533861381));
#48044=CARTESIAN_POINT('Ctrl Pts',(-65.0459227364722,2.12182163449127,14.4811154955701));
#48045=CARTESIAN_POINT('Ctrl Pts',(-63.2422436303638,1.18933940056681,14.3699776050021));
#48046=CARTESIAN_POINT('Ctrl Pts',(-63.0474607219038,-0.831757025163361,
14.258839714434));
#48047=CARTESIAN_POINT('Ctrl Pts',(-64.6398554717402,-2.09154008533313,
14.147701823866));
#48048=CARTESIAN_POINT('Ctrl Pts',(-66.5619019052561,-1.43690629417044,
14.0365639332979));
#48049=CARTESIAN_POINT('Ctrl Pts',(-67.0543073051464,0.532931245964165,
13.9254260427299));
#48050=CARTESIAN_POINT('Ctrl Pts',(-65.6664107088406,2.0149963191636,13.8142881521618));
#48051=CARTESIAN_POINT('Ctrl Pts',(-63.668483745015,1.65266173185674,13.7031502615938));
#48052=CARTESIAN_POINT('Ctrl Pts',(-62.889421959733,-0.222272347729264,
13.5920123710258));
#48053=CARTESIAN_POINT('Ctrl Pts',(-64.0419715223154,-1.89395746343365,
13.4808744804577));
#48054=CARTESIAN_POINT('Ctrl Pts',(-66.0718611861322,-1.83168617135119,
13.3697365898897));
#48055=CARTESIAN_POINT('Ctrl Pts',(-67.1197788376878,-0.0936369858196002,
13.2585986993216));
#48056=CARTESIAN_POINT('Ctrl Pts',(-66.2292075511993,1.73168095096001,13.1474608087536));
#48057=CARTESIAN_POINT('Ctrl Pts',(-64.2098730410853,1.96882346147376,13.0363229181856));
#48058=CARTESIAN_POINT('Ctrl Pts',(-63.3520968146026,0.930071057176342,
12.9622309911402));
#48059=CARTESIAN_POINT('Ctrl Pts',(-63.2376884946835,0.344060554515614,
12.9251850276175));
#48060=CARTESIAN_POINT('Ctrl Pts',(-64.5701357431142,1.60958774866485,22.2244449171475));
#48061=CARTESIAN_POINT('Ctrl Pts',(-64.0349095229901,1.46664765635222,22.1873989536248));
#48062=CARTESIAN_POINT('Ctrl Pts',(-63.1275700215111,0.606976197009781,
22.1133070265794));
#48063=CARTESIAN_POINT('Ctrl Pts',(-63.4747061016385,-1.24728896623771,
22.0021691360114));
#48064=CARTESIAN_POINT('Ctrl Pts',(-65.2206441859093,-1.95631351452271,
21.8910312454434));
#48065=CARTESIAN_POINT('Ctrl Pts',(-66.7632902393938,-0.87643803689069,
21.7798933548753));
#48066=CARTESIAN_POINT('Ctrl Pts',(-66.692647660758,1.00652025480985,21.6687554643073));
#48067=CARTESIAN_POINT('Ctrl Pts',(-65.0723673984167,1.96776149739031,21.5576175737392));
#48068=CARTESIAN_POINT('Ctrl Pts',(-63.3860188510191,1.12810889960267,21.4464796831712));
#48069=CARTESIAN_POINT('Ctrl Pts',(-63.1768796488437,-0.744225754056264,
21.3353417926031));
#48070=CARTESIAN_POINT('Ctrl Pts',(-64.6365064832399,-1.93530608700316,
21.2242039020351));
#48071=CARTESIAN_POINT('Ctrl Pts',(-66.4288212268481,-1.35500706394271,
21.113066011467));
#48072=CARTESIAN_POINT('Ctrl Pts',(-66.9133307013985,0.465559533824989,
21.001928120899));
#48073=CARTESIAN_POINT('Ctrl Pts',(-65.6465413393799,1.85998703107206,20.890790230331));
#48074=CARTESIAN_POINT('Ctrl Pts',(-63.7879681533139,1.55195092417242,20.7796523397629));
#48075=CARTESIAN_POINT('Ctrl Pts',(-63.0387800523716,-0.176605288292527,
20.6685144491949));
#48076=CARTESIAN_POINT('Ctrl Pts',(-64.0847195217704,-1.74351175790306,
20.5573765586268));
#48077=CARTESIAN_POINT('Ctrl Pts',(-65.9684252347068,-1.71456260631994,
20.4462386680588));
#48078=CARTESIAN_POINT('Ctrl Pts',(-66.965720528179,-0.116254623021161,
20.3351007774908));
#48079=CARTESIAN_POINT('Ctrl Pts',(-66.163769438407,1.58846241734546,20.2239628869227));
#48080=CARTESIAN_POINT('Ctrl Pts',(-64.296607029498,1.83924185210905,20.1128249963547));
#48081=CARTESIAN_POINT('Ctrl Pts',(-63.0732681603805,0.406542331281834,
20.0016871057866));
#48082=CARTESIAN_POINT('Ctrl Pts',(-63.6134888063506,-1.39826998078169,
19.8905492152186));
#48083=CARTESIAN_POINT('Ctrl Pts',(-65.4227988660973,-1.92322992958215,
19.7794113246506));
#48084=CARTESIAN_POINT('Ctrl Pts',(-66.8451163318026,-0.687835709090815,
19.6682734340825));
#48085=CARTESIAN_POINT('Ctrl Pts',(-66.5785778924731,1.17714233458595,19.5571355435145));
#48086=CARTESIAN_POINT('Ctrl Pts',(-64.8671492066249,1.96466865068852,19.4459976529464));
#48087=CARTESIAN_POINT('Ctrl Pts',(-63.277320358204,0.953911469466815,19.3348597623784));
#48088=CARTESIAN_POINT('Ctrl Pts',(-63.2642797226261,-0.929971697602105,
19.2237218718103));
#48089=CARTESIAN_POINT('Ctrl Pts',(-64.8399635412389,-1.96264122338425,
19.1125839812423));
#48090=CARTESIAN_POINT('Ctrl Pts',(-66.5621305455413,-1.19888297947456,
19.0014460906742));
#48091=CARTESIAN_POINT('Ctrl Pts',(-66.8544617457199,0.662226451774217,
18.8903082001062));
#48092=CARTESIAN_POINT('Ctrl Pts',(-65.4493830790269,1.91719250157129,18.7791703095382));
#48093=CARTESIAN_POINT('Ctrl Pts',(-63.6329789837436,1.41733051223035,18.6680324189701));
#48094=CARTESIAN_POINT('Ctrl Pts',(-63.0678247277157,-0.379830168572191,
18.5568945284021));
#48095=CARTESIAN_POINT('Ctrl Pts',(-64.271212410766,-1.82932798851556,18.445756637834));
#48096=CARTESIAN_POINT('Ctrl Pts',(-66.1416676392564,-1.6044211545792,18.334618747266));
#48097=CARTESIAN_POINT('Ctrl Pts',(-66.9671415301433,0.0890305575164271,
18.223480856698));
#48098=CARTESIAN_POINT('Ctrl Pts',(-65.9920684695881,1.70099159064234,18.1123429661299));
#48099=CARTESIAN_POINT('Ctrl Pts',(-64.1089438879971,1.75601573029653,18.0012050755619));
#48100=CARTESIAN_POINT('Ctrl Pts',(-63.0414130709861,0.203738757437537,
17.8900671849938));
#48101=CARTESIAN_POINT('Ctrl Pts',(-63.7665990819878,-1.53502261065872,
17.7789292944258));
#48102=CARTESIAN_POINT('Ctrl Pts',(-65.6207309409642,-1.86876037487861,
17.6677914038578));
#48103=CARTESIAN_POINT('Ctrl Pts',(-66.906700730108,-0.492000574788033,
17.5566535132897));
#48104=CARTESIAN_POINT('Ctrl Pts',(-66.4474457175273,1.33509293107206,17.4455156227217));
#48105=CARTESIAN_POINT('Ctrl Pts',(-64.6633272245428,1.94016073613826,17.3343777321536));
#48106=CARTESIAN_POINT('Ctrl Pts',(-63.1873691410633,0.769377416497892,
17.2232398415856));
#48107=CARTESIAN_POINT('Ctrl Pts',(-63.3705326394006,-1.10562577779639,
17.1121019510176));
#48108=CARTESIAN_POINT('Ctrl Pts',(-65.0451660923113,-1.9686371590244,17.0009640604495));
#48109=CARTESIAN_POINT('Ctrl Pts',(-66.6784585087109,-1.02973262273373,
16.8898261698815));
#48110=CARTESIAN_POINT('Ctrl Pts',(-66.7754388170738,0.851697861107777,
16.7786882793134));
#48111=CARTESIAN_POINT('Ctrl Pts',(-65.2473398413224,1.95355963376579,16.6675503887454));
#48112=CARTESIAN_POINT('Ctrl Pts',(-63.4928479037859,1.26730611876661,16.5564124981773));
#48113=CARTESIAN_POINT('Ctrl Pts',(-63.1178693721777,-0.578927058971938,
16.4452746076093));
#48114=CARTESIAN_POINT('Ctrl Pts',(-64.4656263490359,-1.89526173414731,
16.3341367170413));
#48115=CARTESIAN_POINT('Ctrl Pts',(-66.3025015888158,-1.47684185034112,
16.2229988264732));
#48116=CARTESIAN_POINT('Ctrl Pts',(-66.9471823530099,0.29334812763463,16.1118609359052));
#48117=CARTESIAN_POINT('Ctrl Pts',(-65.8095850268848,1.79503323753959,16.0007230453371));
#48118=CARTESIAN_POINT('Ctrl Pts',(-63.9309653444513,1.65370406816781,15.8895851547691));
#48119=CARTESIAN_POINT('Ctrl Pts',(-63.0308452056851,-0.00127918928536197,
15.778447264201));
#48120=CARTESIAN_POINT('Ctrl Pts',(-63.9331147823537,-1.65509158986658,
15.667309373633));
#48121=CARTESIAN_POINT('Ctrl Pts',(-65.8119164971145,-1.79397988904508,
15.556171483065));
#48122=CARTESIAN_POINT('Ctrl Pts',(-66.9475618361337,-0.29081804904335,
15.4450335924969));
#48123=CARTESIAN_POINT('Ctrl Pts',(-66.3005817360626,1.47853284613195,15.3338957019289));
#48124=CARTESIAN_POINT('Ctrl Pts',(-64.4631644305619,1.89456586592117,15.2227578113608));
#48125=CARTESIAN_POINT('Ctrl Pts',(-63.1171187956369,0.576481250135308,
15.1116199207928));
#48126=CARTESIAN_POINT('Ctrl Pts',(-63.4944957086799,-1.26926316652857,
15.0004820302248));
#48127=CARTESIAN_POINT('Ctrl Pts',(-65.2498777170288,-1.95323666226351,
14.8893441396567));
#48128=CARTESIAN_POINT('Ctrl Pts',(-66.7765439285027,-0.849390390991115,
14.7782062490887));
#48129=CARTESIAN_POINT('Ctrl Pts',(-66.6771191139918,1.03191234184772,14.6670683585206));
#48130=CARTESIAN_POINT('Ctrl Pts',(-65.0426085927299,1.96869439442843,14.5559304679526));
#48131=CARTESIAN_POINT('Ctrl Pts',(-63.3690970742208,1.10350736975597,14.4447925773845));
#48132=CARTESIAN_POINT('Ctrl Pts',(-63.1883712234789,-0.771730934564716,
14.3336546868165));
#48133=CARTESIAN_POINT('Ctrl Pts',(-64.6658463169365,-1.94059819863461,
14.2225167962484));
#48134=CARTESIAN_POINT('Ctrl Pts',(-66.4491828509713,-1.33320790054558,
14.1113789056804));
#48135=CARTESIAN_POINT('Ctrl Pts',(-66.9060524269962,0.494470760166873,
14.0002410151124));
#48136=CARTESIAN_POINT('Ctrl Pts',(-65.6183173013013,1.86957842914181,13.8891031245443));
#48137=CARTESIAN_POINT('Ctrl Pts',(-63.764576369348,1.53339273881654,13.7779652339763));
#48138=CARTESIAN_POINT('Ctrl Pts',(-63.0417377741208,-0.206231437128299,
13.6668273434082));
#48139=CARTESIAN_POINT('Ctrl Pts',(-64.111110348268,-1.75727468366666,13.5556894528402));
#48140=CARTESIAN_POINT('Ctrl Pts',(-65.9945073018589,-1.69949737493168,
13.4445515622722));
#48141=CARTESIAN_POINT('Ctrl Pts',(-66.9667990218154,-0.0868794087578511,
13.3334136717041));
#48142=CARTESIAN_POINT('Ctrl Pts',(-66.1404983229023,1.60670931320335,13.2222757811361));
#48143=CARTESIAN_POINT('Ctrl Pts',(-64.2668947805903,1.82673776589703,13.111137890568));
#48144=CARTESIAN_POINT('Ctrl Pts',(-63.4710223937224,0.862949857291941,
13.0370459635227));
#48145=CARTESIAN_POINT('Ctrl Pts',(-63.3648706727485,0.319230454628309,
13.));
#48146=CARTESIAN_POINT('Ctrl Pts',(-63.3361634080255,-0.000941845566861395,
21.3785196366098));
#48147=CARTESIAN_POINT('Ctrl Pts',(-63.3350462116423,-0.216826197428599,
21.3641270219409));
#48148=CARTESIAN_POINT('Ctrl Pts',(-63.3740367968513,-0.432323693321025,
21.349734407272));
#48149=CARTESIAN_POINT('Ctrl Pts',(-63.4550073216056,-0.630683367270925,
21.3353417926031));
#48150=CARTESIAN_POINT('Ctrl Pts',(-63.6634219269757,-1.14125253170523,
21.2982958290804));
#48151=CARTESIAN_POINT('Ctrl Pts',(-64.1499642051078,-1.5382793093542,21.2612498655578));
#48152=CARTESIAN_POINT('Ctrl Pts',(-64.6919544681085,-1.64007619433527,
21.2242039020351));
#48153=CARTESIAN_POINT('Ctrl Pts',(-65.2339447311093,-1.74187307931634,
21.1871579385124));
#48154=CARTESIAN_POINT('Ctrl Pts',(-65.8313829789787,-1.54844007162952,
21.1501119749897));
#48155=CARTESIAN_POINT('Ctrl Pts',(-66.2108536820051,-1.1482958014915,21.113066011467));
#48156=CARTESIAN_POINT('Ctrl Pts',(-66.5903243850316,-0.748151531353475,
21.0760200479444));
#48157=CARTESIAN_POINT('Ctrl Pts',(-66.751827543215,-0.141295998764244,
21.0389740844217));
#48158=CARTESIAN_POINT('Ctrl Pts',(-66.6214475619703,0.394536350404884,
21.001928120899));
#48159=CARTESIAN_POINT('Ctrl Pts',(-66.4910675807256,0.930368699574014,
20.9648821573763));
#48160=CARTESIAN_POINT('Ctrl Pts',(-66.0688044600528,1.39517786532304,20.9278361938536));
#48161=CARTESIAN_POINT('Ctrl Pts',(-65.5479107020387,1.57624309704761,20.890790230331));
#48162=CARTESIAN_POINT('Ctrl Pts',(-65.0270169440246,1.75730832877218,20.8537442668083));
#48163=CARTESIAN_POINT('Ctrl Pts',(-64.4074925486692,1.6546296264723,20.8166983032856));
#48164=CARTESIAN_POINT('Ctrl Pts',(-63.9728656675012,1.31519757324487,20.7796523397629));
#48165=CARTESIAN_POINT('Ctrl Pts',(-63.5773660666821,1.00632288699473,20.7459414387119));
#48166=CARTESIAN_POINT('Ctrl Pts',(-63.3349716882235,0.501403518382684,
20.7122305376608));
#48167=CARTESIAN_POINT('Ctrl Pts',(-63.3318013787731,-0.000864016794193591,
20.6785196366098));
#48168=CARTESIAN_POINT('Ctrl Pts',(-64.4698297828114,1.98517432567173,22.));
#48169=CARTESIAN_POINT('Ctrl Pts',(-64.4011635904059,1.95974978038732,22.));
#48170=CARTESIAN_POINT('Ctrl Pts',(-64.3342007656382,1.9304357713801,22.));
#48171=CARTESIAN_POINT('Ctrl Pts',(-64.2691302660859,1.89752626078927,22.));
#48172=CARTESIAN_POINT('Ctrl Pts',(-64.2022499741923,1.86370144478923,22.));
#48173=CARTESIAN_POINT('Ctrl Pts',(-64.137367961524,1.82607765547919,22.));
#48174=CARTESIAN_POINT('Ctrl Pts',(-64.0747206099689,1.78492942875572,22.));
#48175=CARTESIAN_POINT('Ctrl Pts',(-64.0217852175796,1.7501602410142,22.));
#48176=CARTESIAN_POINT('Ctrl Pts',(-63.9704456655167,1.71287362002867,22.));
#48177=CARTESIAN_POINT('Ctrl Pts',(-63.9208673056515,1.67321717698682,22.));
#48178=CARTESIAN_POINT('Ctrl Pts',(-63.8988414814125,1.65559929195073,22.));
#48179=CARTESIAN_POINT('Ctrl Pts',(-63.8771635659829,1.63751349743234,22.));
#48180=CARTESIAN_POINT('Ctrl Pts',(-63.8558496107188,1.61897201296729,22.));
#48181=CARTESIAN_POINT('Ctrl Pts',(-63.8441378985455,1.60878373366256,22.));
#48182=CARTESIAN_POINT('Ctrl Pts',(-63.8325360961551,1.59845785925715,22.));
#48183=CARTESIAN_POINT('Ctrl Pts',(-63.8210470007987,1.5879963754255,22.));
#48184=CARTESIAN_POINT('Ctrl Pts',(-63.8104526359383,1.57834959530439,22.));
#48185=CARTESIAN_POINT('Ctrl Pts',(-63.7999526722261,1.56858598842988,22.));
#48186=CARTESIAN_POINT('Ctrl Pts',(-63.7895651937358,1.55872256958795,22.));
#48187=CARTESIAN_POINT('Ctrl Pts',(-63.7364801435462,1.50831571822785,22.));
#48188=CARTESIAN_POINT('Ctrl Pts',(-63.6862350752816,1.45522053846771,22.));
#48189=CARTESIAN_POINT('Ctrl Pts',(-63.639048665253,1.39969641403416,22.));
#48190=CARTESIAN_POINT('Ctrl Pts',(-63.5922286928517,1.34460347579176,22.));
#48191=CARTESIAN_POINT('Ctrl Pts',(-63.5484195492875,1.28711828831824,22.));
#48192=CARTESIAN_POINT('Ctrl Pts',(-63.5078796466337,1.22746999892216,22.));
#48193=CARTESIAN_POINT('Ctrl Pts',(-63.4741871309004,1.17789659599364,22.));
#48194=CARTESIAN_POINT('Ctrl Pts',(-63.4427533858106,1.12682844545201,22.));
#48195=CARTESIAN_POINT('Ctrl Pts',(-63.413754367486,1.07439061084202,22.));
#48196=CARTESIAN_POINT('Ctrl Pts',(-63.4016500392281,1.0525028091188,22.));
#48197=CARTESIAN_POINT('Ctrl Pts',(-63.3899702272225,1.03037633270466,22.));
#48198=CARTESIAN_POINT('Ctrl Pts',(-63.3787291685026,1.00802019356891,22.));
#48199=CARTESIAN_POINT('Ctrl Pts',(-63.3735259415793,0.997672052174805,
22.));
#48200=CARTESIAN_POINT('Ctrl Pts',(-63.3684167321731,0.987274704423447,
22.));
#48201=CARTESIAN_POINT('Ctrl Pts',(-63.3634030175405,0.976829046042575,
22.));
#48202=CARTESIAN_POINT('Ctrl Pts',(-63.3581740167297,0.965934856774388,
22.));
#48203=CARTESIAN_POINT('Ctrl Pts',(-63.3530525040039,0.954995586464713,
22.));
#48204=CARTESIAN_POINT('Ctrl Pts',(-63.3480415178798,0.944016502307831,
22.));
#48205=CARTESIAN_POINT('Ctrl Pts',(-63.3195013216555,0.881484855154736,
22.));
#48206=CARTESIAN_POINT('Ctrl Pts',(-63.2945220500091,0.817619969386109,
22.));
#48207=CARTESIAN_POINT('Ctrl Pts',(-63.273327165115,0.752626219156414,22.));
#48208=CARTESIAN_POINT('Ctrl Pts',(-63.2541166188611,0.693717409259875,
22.));
#48209=CARTESIAN_POINT('Ctrl Pts',(-63.2380153357379,0.633880618070606,
22.));
#48210=CARTESIAN_POINT('Ctrl Pts',(-63.2252264587662,0.573263190512467,
22.));
#48211=CARTESIAN_POINT('Ctrl Pts',(-63.2100966383573,0.501550029564721,
22.));
#48212=CARTESIAN_POINT('Ctrl Pts',(-63.199602249042,0.428742773422576,22.));
#48213=CARTESIAN_POINT('Ctrl Pts',(-63.1936681155555,0.35526466203955,22.));
#48214=CARTESIAN_POINT('Ctrl Pts',(-63.1923616383022,0.339087492894985,
22.));
#48215=CARTESIAN_POINT('Ctrl Pts',(-63.1912764288138,0.32287788806267,22.));
#48216=CARTESIAN_POINT('Ctrl Pts',(-63.1904120545575,0.306640528882653,
22.));
#48217=CARTESIAN_POINT('Ctrl Pts',(-63.18952016631,0.289886316551054,22.));
#48218=CARTESIAN_POINT('Ctrl Pts',(-63.1888633864288,0.273096407564662,
22.));
#48219=CARTESIAN_POINT('Ctrl Pts',(-63.1884417974656,0.256310042500943,
22.));
#48220=CARTESIAN_POINT('Ctrl Pts',(-63.1867198704081,0.187748247191763,
22.));
#48221=CARTESIAN_POINT('Ctrl Pts',(-63.1889096770048,0.119158552219121,
22.));
#48222=CARTESIAN_POINT('Ctrl Pts',(-63.1948905827374,0.0508793566118494,
22.));
#48223=CARTESIAN_POINT('Ctrl Pts',(-63.2008702728702,-0.0173859614684271,
22.));
#48224=CARTESIAN_POINT('Ctrl Pts',(-63.2106399749853,-0.0853419781943991,
22.));
#48225=CARTESIAN_POINT('Ctrl Pts',(-63.2241287349498,-0.152635471586587,
22.));
#48226=CARTESIAN_POINT('Ctrl Pts',(-63.2338917748016,-0.201341880440236,
22.));
#48227=CARTESIAN_POINT('Ctrl Pts',(-63.2456041790335,-0.249700946127146,
22.));
#48228=CARTESIAN_POINT('Ctrl Pts',(-63.2592532629054,-0.29756907509214,
22.));
#48229=CARTESIAN_POINT('Ctrl Pts',(-63.2694917264426,-0.333475960682568,
22.));
#48230=CARTESIAN_POINT('Ctrl Pts',(-63.2808201731573,-0.369106450149086,
22.));
#48231=CARTESIAN_POINT('Ctrl Pts',(-63.2932371663006,-0.40439575621736,
22.));
#48232=CARTESIAN_POINT('Ctrl Pts',(-63.2973637241401,-0.416123503903528,
22.));
#48233=CARTESIAN_POINT('Ctrl Pts',(-63.3016073023407,-0.427804352958856,
22.));
#48234=CARTESIAN_POINT('Ctrl Pts',(-63.3059672772019,-0.439435804918062,
22.));
#48235=CARTESIAN_POINT('Ctrl Pts',(-63.3290918712168,-0.501127124918587,
22.));
#48236=CARTESIAN_POINT('Ctrl Pts',(-63.3554889558621,-0.561434936785673,
22.));
#48237=CARTESIAN_POINT('Ctrl Pts',(-63.3851084989722,-0.620025088688961,
22.));
#48238=CARTESIAN_POINT('Ctrl Pts',(-63.4059501828406,-0.661251836151812,
22.));
#48239=CARTESIAN_POINT('Ctrl Pts',(-63.4283882195983,-0.701627610070203,
22.));
#48240=CARTESIAN_POINT('Ctrl Pts',(-63.4524155940285,-0.74102463102569,
22.));
#48241=CARTESIAN_POINT('Ctrl Pts',(-63.4601281158564,-0.753670639642036,
22.));
#48242=CARTESIAN_POINT('Ctrl Pts',(-63.4680055619416,-0.76621742722543,
22.));
#48243=CARTESIAN_POINT('Ctrl Pts',(-63.476044336448,-0.778655072921202,
22.));
#48244=CARTESIAN_POINT('Ctrl Pts',(-63.5102900794466,-0.831640315592426,
22.));
#48245=CARTESIAN_POINT('Ctrl Pts',(-63.5473913229322,-0.882541662833814,
22.));
#48246=CARTESIAN_POINT('Ctrl Pts',(-63.5873138038648,-0.931043840655609,
22.));
#48247=CARTESIAN_POINT('Ctrl Pts',(-63.624120899027,-0.975761108544703,
22.));
#48248=CARTESIAN_POINT('Ctrl Pts',(-63.6633266818169,-1.01843913681673,
22.));
#48249=CARTESIAN_POINT('Ctrl Pts',(-63.7049257741094,-1.05879788933142,
22.));
#48250=CARTESIAN_POINT('Ctrl Pts',(-63.7127105119292,-1.06635051343315,
22.));
#48251=CARTESIAN_POINT('Ctrl Pts',(-63.7205791168682,-1.07382181318668,
22.));
#48252=CARTESIAN_POINT('Ctrl Pts',(-63.7285300176229,-1.08121113172717,
22.));
#48253=CARTESIAN_POINT('Origin',(-65.,8.88178419700125E-15,17.));
#48254=CARTESIAN_POINT('Origin',(-32.5,56.2916512459885,13.));
#48255=CARTESIAN_POINT('Ctrl Pts',(-31.4059736530045,55.03520293743,13.));
#48256=CARTESIAN_POINT('Ctrl Pts',(-31.3544234714595,55.0705532050083,13.));
#48257=CARTESIAN_POINT('Ctrl Pts',(-31.3051813503225,55.1089326491167,13.));
#48258=CARTESIAN_POINT('Ctrl Pts',(-31.2583086630186,55.1500094432508,13.));
#48259=CARTESIAN_POINT('Ctrl Pts',(-31.2285772760959,55.1760644900209,13.));
#48260=CARTESIAN_POINT('Ctrl Pts',(-31.1997994779263,55.203205850304,13.));
#48261=CARTESIAN_POINT('Ctrl Pts',(-31.1719948709674,55.2313585594901,13.));
#48262=CARTESIAN_POINT('Ctrl Pts',(-31.1530079458905,55.2505831930488,13.));
#48263=CARTESIAN_POINT('Ctrl Pts',(-31.1344748967249,55.2702795828656,13.));
#48264=CARTESIAN_POINT('Ctrl Pts',(-31.1164029934988,55.2904256041521,13.));
#48265=CARTESIAN_POINT('Ctrl Pts',(-31.1068068849154,55.3011230611586,13.));
#48266=CARTESIAN_POINT('Ctrl Pts',(-31.0973410263878,55.3119472603811,13.));
#48267=CARTESIAN_POINT('Ctrl Pts',(-31.088015636226,55.3228838806201,13.));
#48268=CARTESIAN_POINT('Ctrl Pts',(-31.0452129476489,55.3730819679982,13.));
#48269=CARTESIAN_POINT('Ctrl Pts',(-31.0053166512349,55.4257004125729,13.));
#48270=CARTESIAN_POINT('Ctrl Pts',(-30.9684112132021,55.4803964719602,13.));
#48271=CARTESIAN_POINT('Ctrl Pts',(-30.9417896427002,55.5198512265645,13.));
#48272=CARTESIAN_POINT('Ctrl Pts',(-30.9167247740352,55.5603881852279,13.));
#48273=CARTESIAN_POINT('Ctrl Pts',(-30.8932580441631,55.6018923087211,13.));
#48274=CARTESIAN_POINT('Ctrl Pts',(-30.8868285869199,55.6132636838069,13.));
#48275=CARTESIAN_POINT('Ctrl Pts',(-30.8805191492575,55.624707716983,13.));
#48276=CARTESIAN_POINT('Ctrl Pts',(-30.8743307097694,55.6362221640537,13.));
#48277=CARTESIAN_POINT('Ctrl Pts',(-30.8680004790577,55.6480004332951,13.));
#48278=CARTESIAN_POINT('Ctrl Pts',(-30.8618007206828,55.6598452669412,13.));
#48279=CARTESIAN_POINT('Ctrl Pts',(-30.8557343741951,55.6717493030395,13.));
#48280=CARTESIAN_POINT('Ctrl Pts',(-30.8249262845843,55.7322042426952,13.));
#48281=CARTESIAN_POINT('Ctrl Pts',(-30.7975367124524,55.7942196204653,13.));
#48282=CARTESIAN_POINT('Ctrl Pts',(-30.7736505521297,55.8574477165599,13.));
#48283=CARTESIAN_POINT('Ctrl Pts',(-30.7494182330752,55.9215921155367,13.));
#48284=CARTESIAN_POINT('Ctrl Pts',(-30.7287909250581,55.9869854552535,13.));
#48285=CARTESIAN_POINT('Ctrl Pts',(-30.7118943735469,56.0533023283581,13.));
#48286=CARTESIAN_POINT('Ctrl Pts',(-30.7014256020703,56.0943909605036,13.));
#48287=CARTESIAN_POINT('Ctrl Pts',(-30.6923897620258,56.1358348151177,13.));
#48288=CARTESIAN_POINT('Ctrl Pts',(-30.6848255185714,56.1775614120725,13.));
#48289=CARTESIAN_POINT('Ctrl Pts',(-30.6786294263425,56.2117408835145,13.));
#48290=CARTESIAN_POINT('Ctrl Pts',(-30.6734208465201,56.2461101541398,13.));
#48291=CARTESIAN_POINT('Ctrl Pts',(-30.6692248691864,56.2806305246086,13.));
#48292=CARTESIAN_POINT('Ctrl Pts',(-30.6675094773726,56.2947430796119,13.));
#48293=CARTESIAN_POINT('Ctrl Pts',(-30.6659632509433,56.3088834625076,13.));
#48294=CARTESIAN_POINT('Ctrl Pts',(-30.6645900225956,56.3230249695405,13.));
#48295=CARTESIAN_POINT('Ctrl Pts',(-30.6577774083435,56.3931812785896,13.));
#48296=CARTESIAN_POINT('Ctrl Pts',(-30.6552023639047,56.4634862436249,13.));
#48297=CARTESIAN_POINT('Ctrl Pts',(-30.656979948111,56.5335953126756,13.));
#48298=CARTESIAN_POINT('Ctrl Pts',(-30.6571775468153,56.541388733181,13.));
#48299=CARTESIAN_POINT('Ctrl Pts',(-30.6574289761758,56.5491797596165,13.));
#48300=CARTESIAN_POINT('Ctrl Pts',(-30.6577344296099,56.5569679370673,13.));
#48301=CARTESIAN_POINT('Ctrl Pts',(-30.6603769077943,56.6243434735906,13.));
#48302=CARTESIAN_POINT('Ctrl Pts',(-30.6670582139718,56.6915049782423,13.));
#48303=CARTESIAN_POINT('Ctrl Pts',(-30.6775414626437,56.7582070441046,13.));
#48304=CARTESIAN_POINT('Ctrl Pts',(-30.6888193174903,56.8299649733794,13.));
#48305=CARTESIAN_POINT('Ctrl Pts',(-30.704496956143,56.9011921151415,13.));
#48306=CARTESIAN_POINT('Ctrl Pts',(-30.7243435713014,56.9715867176024,13.));
#48307=CARTESIAN_POINT('Ctrl Pts',(-30.7279780724868,56.9844780476379,13.));
#48308=CARTESIAN_POINT('Ctrl Pts',(-30.7317525557216,56.9973414427362,13.));
#48309=CARTESIAN_POINT('Ctrl Pts',(-30.7356658273112,57.0101750195627,13.));
#48310=CARTESIAN_POINT('Ctrl Pts',(-30.7390274221048,57.0211993719635,13.));
#48311=CARTESIAN_POINT('Ctrl Pts',(-30.7424887106291,57.032192762231,13.));
#48312=CARTESIAN_POINT('Ctrl Pts',(-30.7460479824822,57.0431526563695,13.));
#48313=CARTESIAN_POINT('Ctrl Pts',(-30.767999129186,57.1107457636177,13.));
#48314=CARTESIAN_POINT('Ctrl Pts',(-30.7936779401901,57.1770813814884,13.));
#48315=CARTESIAN_POINT('Ctrl Pts',(-30.8228134384578,57.241892040805,13.));
#48316=CARTESIAN_POINT('Ctrl Pts',(-30.8525629752182,57.3080686022655,13.));
#48317=CARTESIAN_POINT('Ctrl Pts',(-30.8859166602457,57.3726561595602,13.));
#48318=CARTESIAN_POINT('Ctrl Pts',(-30.9226411453944,57.435369889801,13.));
#48319=CARTESIAN_POINT('Ctrl Pts',(-30.9595879477009,57.4984632669779,13.));
#48320=CARTESIAN_POINT('Ctrl Pts',(-30.9999468758072,57.5596610608135,13.));
#48321=CARTESIAN_POINT('Ctrl Pts',(-31.0435306576476,57.6186586679229,13.));
#48322=CARTESIAN_POINT('Ctrl Pts',(-31.0543033137161,57.633241177825,13.));
#48323=CARTESIAN_POINT('Ctrl Pts',(-31.0652732109609,57.6476891598953,13.));
#48324=CARTESIAN_POINT('Ctrl Pts',(-31.0764379480169,57.6619977668291,13.));
#48325=CARTESIAN_POINT('Ctrl Pts',(-31.0851682201236,57.6731863896666,13.));
#48326=CARTESIAN_POINT('Ctrl Pts',(-31.0940187402904,57.6842909720356,13.));
#48327=CARTESIAN_POINT('Ctrl Pts',(-31.1029745493948,57.6952926418324,13.));
#48328=CARTESIAN_POINT('Ctrl Pts',(-31.1505373073925,57.7537206132213,13.));
#48329=CARTESIAN_POINT('Ctrl Pts',(-31.2011482673078,57.8093550197329,13.));
#48330=CARTESIAN_POINT('Ctrl Pts',(-31.2545510979645,57.8619011539994,13.));
#48331=CARTESIAN_POINT('Ctrl Pts',(-31.3080118292081,57.9145042600028,13.));
#48332=CARTESIAN_POINT('Ctrl Pts',(-31.364270980967,57.9640134082748,13.));
#48333=CARTESIAN_POINT('Ctrl Pts',(-31.4231195455734,58.0101134374941,13.));
#48334=CARTESIAN_POINT('Ctrl Pts',(-31.4806288819684,58.0551643593974,13.));
#48335=CARTESIAN_POINT('Ctrl Pts',(-31.5406117297693,58.0969603996382,13.));
#48336=CARTESIAN_POINT('Ctrl Pts',(-31.6029105622421,58.1351753157717,13.));
#48337=CARTESIAN_POINT('Ctrl Pts',(-31.6163051636256,58.1433917389083,13.));
#48338=CARTESIAN_POINT('Ctrl Pts',(-31.62980694879,58.151442469068,13.));
#48339=CARTESIAN_POINT('Ctrl Pts',(-31.6434145443377,58.1593240060195,13.));
#48340=CARTESIAN_POINT('Ctrl Pts',(-31.6549388802988,58.1659989163223,13.));
#48341=CARTESIAN_POINT('Ctrl Pts',(-31.666539109872,58.1725524712207,13.));
#48342=CARTESIAN_POINT('Ctrl Pts',(-31.6782133743559,58.178984818602,13.));
#48343=CARTESIAN_POINT('Ctrl Pts',(-32.7283737736498,58.3336705852723,13.));
#48344=CARTESIAN_POINT('Ctrl Pts',(-32.8014565014342,58.3184742869048,13.));
#48345=CARTESIAN_POINT('Ctrl Pts',(-32.873478859746,58.2989977860273,13.));
#48346=CARTESIAN_POINT('Ctrl Pts',(-32.9441813035447,58.2754925548875,13.));
#48347=CARTESIAN_POINT('Ctrl Pts',(-33.0130334318814,58.252602466454,13.));
#48348=CARTESIAN_POINT('Ctrl Pts',(-33.0806343841369,58.2258909044567,13.));
#48349=CARTESIAN_POINT('Ctrl Pts',(-33.1467189154995,58.1955520781456,13.));
#48350=CARTESIAN_POINT('Ctrl Pts',(-33.1614684627314,58.1887806909176,13.));
#48351=CARTESIAN_POINT('Ctrl Pts',(-33.1761442892263,58.1818275347425,13.));
#48352=CARTESIAN_POINT('Ctrl Pts',(-33.19073701805,58.174697608363,13.));
#48353=CARTESIAN_POINT('Ctrl Pts',(-33.257702590687,58.1419786009295,13.));
#48354=CARTESIAN_POINT('Ctrl Pts',(-33.3227883262805,58.1056063852406,13.));
#48355=CARTESIAN_POINT('Ctrl Pts',(-33.3857181641543,58.0658123205629,13.));
#48356=CARTESIAN_POINT('Ctrl Pts',(-33.4298991918482,58.0378741797226,13.));
#48357=CARTESIAN_POINT('Ctrl Pts',(-33.4730169952496,58.0082484488949,13.));
#48358=CARTESIAN_POINT('Ctrl Pts',(-33.5149645802173,57.9770049688462,13.));
#48359=CARTESIAN_POINT('Ctrl Pts',(-33.5309116531909,57.9651272396118,13.));
#48360=CARTESIAN_POINT('Ctrl Pts',(-33.5466894884539,57.9530156286815,13.));
#48361=CARTESIAN_POINT('Ctrl Pts',(-33.5622917807054,57.9406737249562,13.));
#48362=CARTESIAN_POINT('Ctrl Pts',(-33.5771528452482,57.9289181556535,13.));
#48363=CARTESIAN_POINT('Ctrl Pts',(-33.5918591269232,57.9169497163141,13.));
#48364=CARTESIAN_POINT('Ctrl Pts',(-33.6063795974092,57.9047932102742,13.));
#48365=CARTESIAN_POINT('Ctrl Pts',(-33.6620452142588,57.8581900779513,13.));
#48366=CARTESIAN_POINT('Ctrl Pts',(-33.7150448947231,57.8087799684573,13.));
#48367=CARTESIAN_POINT('Ctrl Pts',(-33.7651216105449,57.7567754486693,13.));
#48368=CARTESIAN_POINT('Ctrl Pts',(-33.8141231389414,57.7058875078106,13.));
#48369=CARTESIAN_POINT('Ctrl Pts',(-33.8603263530544,57.6525145642833,13.));
#48370=CARTESIAN_POINT('Ctrl Pts',(-33.9034486472843,57.5968301465233,13.));
#48371=CARTESIAN_POINT('Ctrl Pts',(-33.9456250982487,57.5423671093153,13.));
#48372=CARTESIAN_POINT('Ctrl Pts',(-33.9848546824741,57.4856922167148,13.));
#48373=CARTESIAN_POINT('Ctrl Pts',(-34.0208263214491,57.4269537422269,13.));
#48374=CARTESIAN_POINT('Ctrl Pts',(-34.0325140426356,57.4078687371424,13.));
#48375=CARTESIAN_POINT('Ctrl Pts',(-34.0438574259773,57.388565808898,13.));
#48376=CARTESIAN_POINT('Ctrl Pts',(-34.0548446057422,57.3690498892147,13.));
#48377=CARTESIAN_POINT('Ctrl Pts',(-34.0610436453445,57.3580388780562,13.));
#48378=CARTESIAN_POINT('Ctrl Pts',(-34.067129818108,57.3469588598396,13.));
#48379=CARTESIAN_POINT('Ctrl Pts',(-34.0730927269274,57.3358266058508,13.));
#48380=CARTESIAN_POINT('Ctrl Pts',(-34.1053441707905,57.275615847065,13.));
#48381=CARTESIAN_POINT('Ctrl Pts',(-34.1340531805922,57.213774929567,13.));
#48382=CARTESIAN_POINT('Ctrl Pts',(-34.1589642501542,57.1504676177922,13.));
#48383=CARTESIAN_POINT('Ctrl Pts',(-34.1625594232719,57.1413310873482,13.));
#48384=CARTESIAN_POINT('Ctrl Pts',(-34.1660754068789,57.1321639877973,13.));
#48385=CARTESIAN_POINT('Ctrl Pts',(-34.1695113451333,57.1229667871477,13.));
#48386=CARTESIAN_POINT('Ctrl Pts',(-34.1937894815808,57.0579799114317,13.));
#48387=CARTESIAN_POINT('Ctrl Pts',(-34.2140754401802,56.9914902794409,13.));
#48388=CARTESIAN_POINT('Ctrl Pts',(-34.2304117433282,56.9238636615718,13.));
#48389=CARTESIAN_POINT('Ctrl Pts',(-34.245652193415,56.8607734945473,13.));
#48390=CARTESIAN_POINT('Ctrl Pts',(-34.2574544360998,56.7966929502099,13.));
#48391=CARTESIAN_POINT('Ctrl Pts',(-34.2658134374967,56.7319255341061,13.));
#48392=CARTESIAN_POINT('Ctrl Pts',(-34.2676584011686,56.7176303421134,13.));
#48393=CARTESIAN_POINT('Ctrl Pts',(-34.2693354843638,56.7033017407945,13.));
#48394=CARTESIAN_POINT('Ctrl Pts',(-34.27084439597,56.6889430967533,13.));
#48395=CARTESIAN_POINT('Ctrl Pts',(-34.2720238222203,56.6777198006816,13.));
#48396=CARTESIAN_POINT('Ctrl Pts',(-34.2731003471717,56.6664788449441,13.));
#48397=CARTESIAN_POINT('Ctrl Pts',(-34.2740729516962,56.6552348561548,13.));
#48398=CARTESIAN_POINT('Ctrl Pts',(-34.2799651734903,56.5871166496992,13.));
#48399=CARTESIAN_POINT('Ctrl Pts',(-34.2820614503506,56.5187616008007,13.));
#48400=CARTESIAN_POINT('Ctrl Pts',(-34.2804207734206,56.4505176929745,13.));
#48401=CARTESIAN_POINT('Ctrl Pts',(-34.2787876667987,56.3825886718839,13.));
#48402=CARTESIAN_POINT('Ctrl Pts',(-34.2734516847768,56.3147686814055,13.));
#48403=CARTESIAN_POINT('Ctrl Pts',(-34.2644214384179,56.2474134553717,13.));
#48404=CARTESIAN_POINT('Ctrl Pts',(-34.2555845575853,56.1815005132143,13.));
#48405=CARTESIAN_POINT('Ctrl Pts',(-34.2432095215078,56.1160317619071,13.));
#48406=CARTESIAN_POINT('Ctrl Pts',(-34.2272624366924,56.0513669976104,13.));
#48407=CARTESIAN_POINT('Ctrl Pts',(-34.2239018012959,56.0377397611393,13.));
#48408=CARTESIAN_POINT('Ctrl Pts',(-34.2203823922543,56.0241483513653,13.));
#48409=CARTESIAN_POINT('Ctrl Pts',(-34.2167036732636,56.010596345236,13.));
#48410=CARTESIAN_POINT('Ctrl Pts',(-34.2132180508017,55.9977556860044,13.));
#48411=CARTESIAN_POINT('Ctrl Pts',(-34.2095887843185,55.9849487309035,13.));
#48412=CARTESIAN_POINT('Ctrl Pts',(-34.2058217802814,55.9721990639717,13.));
#48413=CARTESIAN_POINT('Ctrl Pts',(-34.1873069911305,55.9095345718023,13.));
#48414=CARTESIAN_POINT('Ctrl Pts',(-34.1654391518089,55.8481392503641,13.));
#48415=CARTESIAN_POINT('Ctrl Pts',(-34.1402348458881,55.7883322345209,13.));
#48416=CARTESIAN_POINT('Ctrl Pts',(-34.1155097070604,55.7296622289178,13.));
#48417=CARTESIAN_POINT('Ctrl Pts',(-34.0875733532636,55.6725199272576,13.));
#48418=CARTESIAN_POINT('Ctrl Pts',(-34.0564019232237,55.6172367682145,13.));
#48419=CARTESIAN_POINT('Ctrl Pts',(-34.0262427202972,55.5637488143458,13.));
#48420=CARTESIAN_POINT('Ctrl Pts',(-33.9930547257666,55.5120006932486,13.));
#48421=CARTESIAN_POINT('Ctrl Pts',(-33.9567849770258,55.4623304145917,13.));
#48422=CARTESIAN_POINT('Ctrl Pts',(-33.950749031927,55.454064377869,13.));
#48423=CARTESIAN_POINT('Ctrl Pts',(-33.9446276728907,55.44585598451,13.));
#48424=CARTESIAN_POINT('Ctrl Pts',(-33.9384205797355,55.4377069137227,13.));
#48425=CARTESIAN_POINT('Ctrl Pts',(-33.931849519021,55.4290800029336,13.));
#48426=CARTESIAN_POINT('Ctrl Pts',(-33.9251823737702,55.4205195760217,13.));
#48427=CARTESIAN_POINT('Ctrl Pts',(-33.9184205240576,55.4120266023845,13.));
#48428=CARTESIAN_POINT('Origin',(-32.5,56.2916512459885,23.5459252805377));
#48429=CARTESIAN_POINT('Ctrl Pts',(-31.4730118547325,54.5098571360137,21.7959252805377));
#48430=CARTESIAN_POINT('Ctrl Pts',(-31.5577251735552,54.4600031121465,21.7905813053169));
#48431=CARTESIAN_POINT('Ctrl Pts',(-32.2577698823492,54.1148344325097,21.7481913665734));
#48432=CARTESIAN_POINT('Ctrl Pts',(-33.9070787897524,54.3119235461293,21.6687554643073));
#48433=CARTESIAN_POINT('Ctrl Pts',(-34.9261604045136,56.4001058936205,21.5576175737392));
#48434=CARTESIAN_POINT('Ctrl Pts',(-33.7248161346881,58.3888336702691,21.4464796831712));
#48435=CARTESIAN_POINT('Ctrl Pts',(-31.4022507610406,58.4580789101429,21.3353417926031));
#48436=CARTESIAN_POINT('Ctrl Pts',(-30.0845341595457,56.5443222204948,21.2242039020351));
#48437=CARTESIAN_POINT('Ctrl Pts',(-30.7258866583527,55.004043700614,21.1443983980133));
#48438=CARTESIAN_POINT('Ctrl Pts',(-31.3789145578643,54.5633564487824,21.1016388575141));
#48439=CARTESIAN_POINT('Ctrl Pts',(-31.4704172621348,54.5115691325664,21.0959252805377));
#48440=CARTESIAN_POINT('Ctrl Pts',(-31.4716734168817,54.5151354051885,21.8540747194623));
#48441=CARTESIAN_POINT('Ctrl Pts',(-31.8806518858733,54.2831085316556,21.8286245525962));
#48442=CARTESIAN_POINT('Ctrl Pts',(-33.082939422317,54.0422681540074,21.7661284222074));
#48443=CARTESIAN_POINT('Ctrl Pts',(-34.7256560234758,55.3208993649632,21.6665863282959));
#48444=CARTESIAN_POINT('Ctrl Pts',(-34.5234929724835,57.6345755616839,21.5554484377278));
#48445=CARTESIAN_POINT('Ctrl Pts',(-32.4687454188576,58.7202753686331,21.4443105471598));
#48446=CARTESIAN_POINT('Ctrl Pts',(-30.4428342940784,57.5824199368057,21.3331726565918));
#48447=CARTESIAN_POINT('Ctrl Pts',(-30.3182849616345,55.5637298511604,21.2364273806926));
#48448=CARTESIAN_POINT('Ctrl Pts',(-31.1131094829785,54.725326778543,21.1767280683161));
#48449=CARTESIAN_POINT('Ctrl Pts',(-31.47496098746,54.5139076530797,21.1540747194623));
#48450=CARTESIAN_POINT('Ctrl Pts',(-34.0692874532608,56.8510195406194,22.));
#48451=CARTESIAN_POINT('Ctrl Pts',(-33.8832841873681,57.3728449537375,21.9629540364773));
#48452=CARTESIAN_POINT('Ctrl Pts',(-32.9525520823054,58.2072244344894,21.888862109432));
#48453=CARTESIAN_POINT('Ctrl Pts',(-31.1328156874419,57.7104505124287,21.7777242188639));
#48454=CARTESIAN_POINT('Ctrl Pts',(-30.5680805647129,55.9126012127397,21.6665863282959));
#48455=CARTESIAN_POINT('Ctrl Pts',(-31.7699104961033,54.4629042731491,21.5554484377278));
#48456=CARTESIAN_POINT('Ctrl Pts',(-33.640865440432,54.686479644594,21.4443105471598));
#48457=CARTESIAN_POINT('Ctrl Pts',(-34.4671411285653,56.3795867334953,21.3331726565917));
#48458=CARTESIAN_POINT('Ctrl Pts',(-33.493086107989,57.992055635258,21.2220347660237));
#48459=CARTESIAN_POINT('Ctrl Pts',(-31.6099402690806,58.0481999689383,21.1108968754557));
#48460=CARTESIAN_POINT('Ctrl Pts',(-30.5415300692557,56.4965179419503,20.9997589848876));
#48461=CARTESIAN_POINT('Ctrl Pts',(-31.2657026944405,54.7573377854331,20.8886210943196));
#48462=CARTESIAN_POINT('Ctrl Pts',(-33.1196550861102,54.4225228075051,20.7774832037515));
#48463=CARTESIAN_POINT('Ctrl Pts',(-34.4064234335583,55.7985469486803,20.6663453131835));
#48464=CARTESIAN_POINT('Ctrl Pts',(-33.9482241472934,57.6259127164006,20.5552074226154));
#48465=CARTESIAN_POINT('Ctrl Pts',(-32.1644471988302,58.2320149921632,20.4440695320474));
#48466=CARTESIAN_POINT('Ctrl Pts',(-30.6878063720739,57.0620797446064,20.3329316414794));
#48467=CARTESIAN_POINT('Ctrl Pts',(-30.8698865063134,55.1869628453693,20.2217937509113));
#48468=CARTESIAN_POINT('Ctrl Pts',(-32.5440282170451,54.3229796221853,20.1106558603433));
#48469=CARTESIAN_POINT('Ctrl Pts',(-34.1778702970046,55.2609439349858,19.9995179697752));
#48470=CARTESIAN_POINT('Ctrl Pts',(-34.2759387179252,57.1423263023632,19.8883800792072));
#48471=CARTESIAN_POINT('Ctrl Pts',(-32.7484702637604,58.2450761614137,19.7772421886392));
#48472=CARTESIAN_POINT('Ctrl Pts',(-30.9935741723466,57.559834032996,19.6661042980711));
#48473=CARTESIAN_POINT('Ctrl Pts',(-30.6175267185128,55.7138098219725,19.5549664075031));
#48474=CARTESIAN_POINT('Ctrl Pts',(-31.9645284111714,54.3966904172638,19.443828516935));
#48475=CARTESIAN_POINT('Ctrl Pts',(-33.801653320123,54.8140501505304,19.332690626367));
#48476=CARTESIAN_POINT('Ctrl Pts',(-34.4473601842239,56.5838749230434,19.221552735799));
#48477=CARTESIAN_POINT('Ctrl Pts',(-33.3106261867332,58.0862240501872,19.1104148452309));
#48478=CARTESIAN_POINT('Ctrl Pts',(-31.4319168476017,57.9459803376677,18.9992769546629));
#48479=CARTESIAN_POINT('Ctrl Pts',(-30.530836130646,56.2915104462365,18.8881390640948));
#48480=CARTESIAN_POINT('Ctrl Pts',(-31.4321534351977,54.6371694303799,18.7770011735268));
#48481=CARTESIAN_POINT('Ctrl Pts',(-33.3108828106914,54.4971943834675,18.6658632829587));
#48482=CARTESIAN_POINT('Ctrl Pts',(-34.4474019535353,55.9997060533366,18.5547253923907));
#48483=CARTESIAN_POINT('Ctrl Pts',(-33.8014420032618,57.7694384689281,18.4435875018226));
#48484=CARTESIAN_POINT('Ctrl Pts',(-31.9642574280497,58.1865354801138,18.3324496112546));
#48485=CARTESIAN_POINT('Ctrl Pts',(-30.6174441046762,56.8692234623569,18.2213117206866));
#48486=CARTESIAN_POINT('Ctrl Pts',(-30.9937555419292,55.023253044843,18.1101738301185));
#48487=CARTESIAN_POINT('Ctrl Pts',(-32.748749613628,54.3382618854518,17.9990359395505));
#48488=CARTESIAN_POINT('Ctrl Pts',(-34.2760603429608,55.4412301607017,17.8878980489825));
#48489=CARTESIAN_POINT('Ctrl Pts',(-34.1777228984872,57.3225984997458,17.7767601584144));
#48490=CARTESIAN_POINT('Ctrl Pts',(-32.5437466583566,58.2603291256887,17.6656222678464));
#48491=CARTESIAN_POINT('Ctrl Pts',(-30.8697286057113,57.3961065620164,17.5544843772783));
#48492=CARTESIAN_POINT('Ctrl Pts',(-30.6879164487935,55.5209635222085,17.4433464867103));
#48493=CARTESIAN_POINT('Ctrl Pts',(-32.1647249167202,54.3512396961698,17.3322085961422));
#48494=CARTESIAN_POINT('Ctrl Pts',(-33.9484144706509,54.9575965674438,17.2210707055742));
#48495=CARTESIAN_POINT('Ctrl Pts',(-34.4063538334575,56.7850288151987,17.1099328150062));
#48496=CARTESIAN_POINT('Ctrl Pts',(-33.1193859129776,58.1608669785734,16.9987949244381));
#48497=CARTESIAN_POINT('Ctrl Pts',(-31.2654870420352,57.825790783565,16.8876570338701));
#48498=CARTESIAN_POINT('Ctrl Pts',(-30.5415518818472,56.086499271487,16.776519143302));
#48499=CARTESIAN_POINT('Ctrl Pts',(-31.6102064945166,54.534985688252,16.665381252734));
#48500=CARTESIAN_POINT('Ctrl Pts',(-33.4932991936999,54.5913680119553,16.5542433621659));
#48501=CARTESIAN_POINT('Ctrl Pts',(-34.46721387611,56.2040388622933,16.4431054715979));
#48502=CARTESIAN_POINT('Ctrl Pts',(-33.6405153879953,57.896902321018,16.3319675810299));
#48503=CARTESIAN_POINT('Ctrl Pts',(-31.7698902309214,58.1204612659856,16.2208296904618));
#48504=CARTESIAN_POINT('Ctrl Pts',(-30.5675428254988,56.6700896595284,16.1096917998938));
#48505=CARTESIAN_POINT('Ctrl Pts',(-31.1339953874406,54.8733290813849,15.9985539093257));
#48506=CARTESIAN_POINT('Ctrl Pts',(-32.9507674628268,54.3747748653499,15.8874160187577));
#48507=CARTESIAN_POINT('Ctrl Pts',(-34.3549469673912,55.6307593394112,15.7762781281896));
#48508=CARTESIAN_POINT('Ctrl Pts',(-34.0612724762645,57.4916656705044,15.6651402376216));
#48509=CARTESIAN_POINT('Ctrl Pts',(-32.3385475813956,58.2541851899138,15.5540023470536));
#48510=CARTESIAN_POINT('Ctrl Pts',(-30.7636019166367,57.2203751334698,15.4428644564855));
#48511=CARTESIAN_POINT('Ctrl Pts',(-30.7780011089404,55.3364935710292,15.3317265659175));
#48512=CARTESIAN_POINT('Ctrl Pts',(-32.3685654164946,54.326878659382,15.2205886753495));
#48513=CARTESIAN_POINT('Ctrl Pts',(-34.0794332859622,55.1156423809378,15.1094507847814));
#48514=CARTESIAN_POINT('Ctrl Pts',(-34.3446279626791,56.9808203482265,14.9983128942134));
#48515=CARTESIAN_POINT('Ctrl Pts',(-32.9214137338773,58.2151940311283,14.8871750036453));
#48516=CARTESIAN_POINT('Ctrl Pts',(-31.1124747588704,57.6889271671125,14.7760371130773));
#48517=CARTESIAN_POINT('Ctrl Pts',(-30.5735533254956,55.8837178487831,14.6648992225092));
#48518=CARTESIAN_POINT('Ctrl Pts',(-31.7979304751287,54.4518945101648,14.5537613319412));
#48519=CARTESIAN_POINT('Ctrl Pts',(-33.6649196338359,54.704021546316,14.4426234413732));
#48520=CARTESIAN_POINT('Ctrl Pts',(-34.4656450190373,56.4093237108058,14.3314855508051));
#48521=CARTESIAN_POINT('Ctrl Pts',(-33.4671924688587,58.0069196157817,14.2203476602371));
#48522=CARTESIAN_POINT('Ctrl Pts',(-31.5834591995985,58.0345095641669,14.109209769669));
#48523=CARTESIAN_POINT('Ctrl Pts',(-30.5386430838269,56.4668442614587,13.998071879101));
#48524=CARTESIAN_POINT('Ctrl Pts',(-31.289085272834,54.7388173343014,13.886933988533));
#48525=CARTESIAN_POINT('Ctrl Pts',(-33.1478792814866,54.4321278475435,13.7757960979649));
#48526=CARTESIAN_POINT('Ctrl Pts',(-34.4136863832883,55.8274592952635,13.6646582073969));
#48527=CARTESIAN_POINT('Ctrl Pts',(-33.9278258993099,57.6477147792301,13.5535203168288));
#48528=CARTESIAN_POINT('Ctrl Pts',(-32.135157735345,58.2266620964951,13.4423824262608));
#48529=CARTESIAN_POINT('Ctrl Pts',(-30.6762385450867,57.0346478668883,13.3312445356927));
#48530=CARTESIAN_POINT('Ctrl Pts',(-30.8870198365664,55.1622083892051,13.2201066451247));
#48531=CARTESIAN_POINT('Ctrl Pts',(-32.5733973317359,54.3242660615774,13.1089687545567));
#48532=CARTESIAN_POINT('Ctrl Pts',(-34.1941640560837,55.2856728893476,12.9978308639886));
#48533=CARTESIAN_POINT('Ctrl Pts',(-34.2610507255277,57.1708124199609,12.8866929734206));
#48534=CARTESIAN_POINT('Ctrl Pts',(-33.2357187233791,57.8857569315589,12.8126010463752));
#48535=CARTESIAN_POINT('Ctrl Pts',(-32.6851664226308,57.947329172377,12.7755550828525));
#48536=CARTESIAN_POINT('Ctrl Pts',(-34.1913483771213,56.8945278288422,22.0748149723825));
#48537=CARTESIAN_POINT('Ctrl Pts',(-33.9908775702891,57.4569414030947,22.0377690088598));
#48538=CARTESIAN_POINT('Ctrl Pts',(-32.9877520867064,58.3562198480607,21.9636770818145));
#48539=CARTESIAN_POINT('Ctrl Pts',(-31.0264745706939,57.8208062977086,21.8525391912464));
#48540=CARTESIAN_POINT('Ctrl Pts',(-30.4178137218822,55.8831182794813,21.7414013006784));
#48541=CARTESIAN_POINT('Ctrl Pts',(-31.7131233223058,54.3206622992212,21.6302634101103));
#48542=CARTESIAN_POINT('Ctrl Pts',(-33.7296032235388,54.5616276117724,21.5191255195423));
#48543=CARTESIAN_POINT('Ctrl Pts',(-34.6201475538814,56.386426453537,21.4079876289742));
#48544=CARTESIAN_POINT('Ctrl Pts',(-33.5703294502221,58.1243149802617,21.2968497384062));
#48545=CARTESIAN_POINT('Ctrl Pts',(-31.5407104330673,58.1848262826732,21.1857118478381));
#48546=CARTESIAN_POINT('Ctrl Pts',(-30.3891980993524,56.5124527014652,21.0745739572701));
#48547=CARTESIAN_POINT('Ctrl Pts',(-31.1696976769262,54.6379971776317,20.9634360667021));
#48548=CARTESIAN_POINT('Ctrl Pts',(-33.16785254804,54.2771399182574,20.852298176134));
#48549=CARTESIAN_POINT('Ctrl Pts',(-34.5547071690116,55.7601927478842,20.741160285566));
#48550=CARTESIAN_POINT('Ctrl Pts',(-34.0608686325396,57.7296930578618,20.6300223949979));
#48551=CARTESIAN_POINT('Ctrl Pts',(-32.1383475286711,58.3829386428886,20.5188845044299));
#48552=CARTESIAN_POINT('Ctrl Pts',(-30.5468519357281,57.1220045302883,20.4077466138619));
#48553=CARTESIAN_POINT('Ctrl Pts',(-30.7430944653628,55.1010389526641,20.2966087232938));
#48554=CARTESIAN_POINT('Ctrl Pts',(-32.5474527807459,54.1698541532471,20.1854708327258));
#48555=CARTESIAN_POINT('Ctrl Pts',(-34.3083769152439,55.1807743737308,20.0743329421577));
#48556=CARTESIAN_POINT('Ctrl Pts',(-34.4140732070396,57.2084927545773,19.9631950515897));
#48557=CARTESIAN_POINT('Ctrl Pts',(-32.7677965572851,58.3970157244132,19.8520571610217));
#48558=CARTESIAN_POINT('Ctrl Pts',(-30.8764026956559,57.658474700953,19.7409192704536));
#48559=CARTESIAN_POINT('Ctrl Pts',(-30.4711058525308,55.6688646731958,19.6297813798856));
#48560=CARTESIAN_POINT('Ctrl Pts',(-31.9228788353097,54.2492982559658,19.5186434893175));
#48561=CARTESIAN_POINT('Ctrl Pts',(-33.9028973633798,54.6991206935758,19.4075055987495));
#48562=CARTESIAN_POINT('Ctrl Pts',(-34.5988280256839,56.6066044057275,19.2963677081814));
#48563=CARTESIAN_POINT('Ctrl Pts',(-33.3736775933143,58.2258079192613,19.1852298176134));
#48564=CARTESIAN_POINT('Ctrl Pts',(-31.3488401518244,58.0746558947685,19.0740919270453));
#48565=CARTESIAN_POINT('Ctrl Pts',(-30.3776723743012,56.2914994946751,18.9629540364773));
#48566=CARTESIAN_POINT('Ctrl Pts',(-31.3490951414668,54.5084819942419,18.8518161459093));
#48567=CARTESIAN_POINT('Ctrl Pts',(-33.3739541777695,54.3576195324661,18.7406782553412));
#48568=CARTESIAN_POINT('Ctrl Pts',(-34.5988730438588,55.9769982314792,18.6295403647732));
#48569=CARTESIAN_POINT('Ctrl Pts',(-33.9026696100581,57.8843824030853,18.5184024742052));
#48570=CARTESIAN_POINT('Ctrl Pts',(-31.9225867748193,58.3339216837985,18.4072645836371));
#48571=CARTESIAN_POINT('Ctrl Pts',(-30.471016812898,56.9141476718634,18.2961266930691));
#48572=CARTESIAN_POINT('Ctrl Pts',(-30.8765981723664,54.9245956217347,18.184988802501));
#48573=CARTESIAN_POINT('Ctrl Pts',(-32.7680976352962,54.1863250879512,18.073850911933));
#48574=CARTESIAN_POINT('Ctrl Pts',(-34.4142042922057,55.3750834626414,17.9627130213649));
#48575=CARTESIAN_POINT('Ctrl Pts',(-34.308218051906,57.4027867240152,17.8515751307969));
#48576=CARTESIAN_POINT('Ctrl Pts',(-32.5471493221094,58.4134550812175,17.7404372402288));
#48577=CARTESIAN_POINT('Ctrl Pts',(-30.7429242830763,57.4820123251428,17.6292993496608));
#48578=CARTESIAN_POINT('Ctrl Pts',(-30.5469705743374,55.4610185737053,17.5181614590928));
#48579=CARTESIAN_POINT('Ctrl Pts',(-32.1386468477677,54.2003123272238,17.4070235685247));
#48580=CARTESIAN_POINT('Ctrl Pts',(-34.0610737594595,54.8538323104841,17.2958856779567));
#48581=CARTESIAN_POINT('Ctrl Pts',(-34.5546321553377,56.8234042713873,17.1847477873886));
#48582=CARTESIAN_POINT('Ctrl Pts',(-33.1675624383217,58.3062566576535,17.0736098968206));
#48583=CARTESIAN_POINT('Ctrl Pts',(-31.169465250837,57.9451178634435,16.9624720062526));
#48584=CARTESIAN_POINT('Ctrl Pts',(-30.3892216085515,56.07054232269,16.8513341156845));
#48585=CARTESIAN_POINT('Ctrl Pts',(-31.5409973658138,54.3983502869775,16.7401962251165));
#48586=CARTESIAN_POINT('Ctrl Pts',(-33.5705591099766,54.4591180905408,16.6290583345485));
#48587=CARTESIAN_POINT('Ctrl Pts',(-34.620225959811,56.1972242736254,16.5179204439804));
#48588=CARTESIAN_POINT('Ctrl Pts',(-33.7292259436341,58.0217605353874,16.4067825534124));
#48589=CARTESIAN_POINT('Ctrl Pts',(-31.7131014808755,58.2627081437914,16.2956446628443));
#48590=CARTESIAN_POINT('Ctrl Pts',(-30.4172341567138,56.6995250203254,16.1845067722763));
#48591=CARTESIAN_POINT('Ctrl Pts',(-31.0277460290708,54.7630104056166,16.0733688817082));
#48592=CARTESIAN_POINT('Ctrl Pts',(-32.9858286575395,54.2256780880443,15.9622309911402));
#48593=CARTESIAN_POINT('Ctrl Pts',(-34.4992268060413,55.5793544317117,15.8510931005721));
#48594=CARTESIAN_POINT('Ctrl Pts',(-34.182709986298,57.5850041273933,15.7399552100041));
#48595=CARTESIAN_POINT('Ctrl Pts',(-32.3259896326697,58.4068332632833,15.628817319436));
#48596=CARTESIAN_POINT('Ctrl Pts',(-30.6285429420654,57.2926123105923,15.517679428868));
#48597=CARTESIAN_POINT('Ctrl Pts',(-30.6440621195648,55.2622003445105,15.4065415382999));
#48598=CARTESIAN_POINT('Ctrl Pts',(-32.3583422883758,54.1740564618943,15.295403647732));
#48599=CARTESIAN_POINT('Ctrl Pts',(-34.202283363977,55.0241711031691,15.1842657571639));
#48600=CARTESIAN_POINT('Ctrl Pts',(-34.4881051776634,57.0344246876612,15.0731278665959));
#48601=CARTESIAN_POINT('Ctrl Pts',(-32.9541917628979,58.364809328792,14.9619899760278));
#48602=CARTESIAN_POINT('Ctrl Pts',(-31.0045515020698,57.79760884265,14.8508520854598));
#48603=CARTESIAN_POINT('Ctrl Pts',(-30.4237121600868,55.851988335345,14.7397141948917));
#48604=CARTESIAN_POINT('Ctrl Pts',(-31.7433227264704,54.3087961846243,14.6285763043237));
#48605=CARTESIAN_POINT('Ctrl Pts',(-33.7555283788647,54.5805339421248,14.5174384137556));
#48606=CARTESIAN_POINT('Ctrl Pts',(-34.6185350752899,56.4184764060234,14.4063005231876));
#48607=CARTESIAN_POINT('Ctrl Pts',(-33.542421775035,58.1403350977259,14.2951626326195));
#48608=CARTESIAN_POINT('Ctrl Pts',(-31.5121696365421,58.1700710229888,14.1840247420515));
#48609=CARTESIAN_POINT('Ctrl Pts',(-30.3860865609853,56.4804709690945,14.0728868514835));
#48610=CARTESIAN_POINT('Ctrl Pts',(-31.1948989782791,54.618036185208,13.9617489609154));
#48611=CARTESIAN_POINT('Ctrl Pts',(-33.1982720527306,54.287492048995,13.8506110703474));
#48612=CARTESIAN_POINT('Ctrl Pts',(-34.5625350390513,55.7913539289481,13.7394731797794));
#48613=CARTESIAN_POINT('Ctrl Pts',(-34.0388837861359,57.7531909093916,13.6283352892113));
#48614=CARTESIAN_POINT('Ctrl Pts',(-32.1067798981332,58.3771693930405,13.5171973986433));
#48615=CARTESIAN_POINT('Ctrl Pts',(-30.5343843502893,57.0924389706047,13.4060595080752));
#48616=CARTESIAN_POINT('Ctrl Pts',(-30.7615604451029,55.0743590673614,13.2949216175072));
#48617=CARTESIAN_POINT('Ctrl Pts',(-32.5791062578488,54.1712406533262,13.1837837269391));
#48618=CARTESIAN_POINT('Ctrl Pts',(-34.3259380210302,55.2074267736725,13.0726458363711));
#48619=CARTESIAN_POINT('Ctrl Pts',(-34.3980272100313,57.2391945540909,12.9615079458031));
#48620=CARTESIAN_POINT('Ctrl Pts',(-33.2929437441301,58.0097482451375,12.8874160187577));
#48621=CARTESIAN_POINT('Ctrl Pts',(-32.6995688729705,58.0761096433421,12.850370055235));
#48622=CARTESIAN_POINT('Ctrl Pts',(-34.3134093009819,56.9380361170651,22.149629944765));
#48623=CARTESIAN_POINT('Ctrl Pts',(-34.0984709532102,57.5410378524519,22.1125839812423));
#48624=CARTESIAN_POINT('Ctrl Pts',(-33.0229520911074,58.5052152616321,22.0384920541969));
#48625=CARTESIAN_POINT('Ctrl Pts',(-30.9201334539457,57.9311620829883,21.9273541636289));
#48626=CARTESIAN_POINT('Ctrl Pts',(-30.2675468790515,55.8536353462229,21.8162162730609));
#48627=CARTESIAN_POINT('Ctrl Pts',(-31.6563361485083,54.1784203252934,21.7050783824928));
#48628=CARTESIAN_POINT('Ctrl Pts',(-33.8183410066456,54.4367755789509,21.5939404919248));
#48629=CARTESIAN_POINT('Ctrl Pts',(-34.7731539791975,56.3932661735786,21.4828026013567));
#48630=CARTESIAN_POINT('Ctrl Pts',(-33.6475727924551,58.2565743252655,21.3716647107887));
#48631=CARTESIAN_POINT('Ctrl Pts',(-31.4714805970539,58.321452596408,21.2605268202206));
#48632=CARTESIAN_POINT('Ctrl Pts',(-30.2368661294491,56.52838746098,21.1493889296526));
#48633=CARTESIAN_POINT('Ctrl Pts',(-31.0736926594119,54.5186565698305,21.0382510390845));
#48634=CARTESIAN_POINT('Ctrl Pts',(-33.2160500099699,54.1317570290096,20.9271131485165));
#48635=CARTESIAN_POINT('Ctrl Pts',(-34.702990904465,55.7218385470883,20.8159752579485));
#48636=CARTESIAN_POINT('Ctrl Pts',(-34.1735131177858,57.8334733993229,20.7048373673804));
#48637=CARTESIAN_POINT('Ctrl Pts',(-32.112247858512,58.533862293614,20.5936994768124));
#48638=CARTESIAN_POINT('Ctrl Pts',(-30.4058974993823,57.18192931597,20.4825615862443));
#48639=CARTESIAN_POINT('Ctrl Pts',(-30.6163024244123,55.0151150599589,20.3714236956763));
#48640=CARTESIAN_POINT('Ctrl Pts',(-32.5508773444466,54.0167286843088,20.2602858051082));
#48641=CARTESIAN_POINT('Ctrl Pts',(-34.4388835334834,55.1006048124758,20.1491479145402));
#48642=CARTESIAN_POINT('Ctrl Pts',(-34.5522076961539,57.2746592067913,20.0380100239722));
#48643=CARTESIAN_POINT('Ctrl Pts',(-32.7871228508099,58.5489552874127,19.9268721334041));
#48644=CARTESIAN_POINT('Ctrl Pts',(-30.7592312189652,57.7571153689101,19.8157342428361));
#48645=CARTESIAN_POINT('Ctrl Pts',(-30.3246849865488,55.623919524419,19.7045963522681));
#48646=CARTESIAN_POINT('Ctrl Pts',(-31.8812292594479,54.101906094668,19.5934584617));
#48647=CARTESIAN_POINT('Ctrl Pts',(-34.0041414066367,54.5841912366211,19.482320571132));
#48648=CARTESIAN_POINT('Ctrl Pts',(-34.7502958671439,56.6293338884117,19.3711826805639));
#48649=CARTESIAN_POINT('Ctrl Pts',(-33.4367289998955,58.3653917883353,19.2600447899959));
#48650=CARTESIAN_POINT('Ctrl Pts',(-31.2657634560471,58.2033314518695,19.1489068994278));
#48651=CARTESIAN_POINT('Ctrl Pts',(-30.2245086179564,56.2914885431137,19.0377690088598));
#48652=CARTESIAN_POINT('Ctrl Pts',(-31.266036847736,54.379794558104,18.9266311182918));
#48653=CARTESIAN_POINT('Ctrl Pts',(-33.4370255448476,54.2180446814646,18.8154932277237));
#48654=CARTESIAN_POINT('Ctrl Pts',(-34.7503441341823,55.9542904096218,18.7043553371557));
#48655=CARTESIAN_POINT('Ctrl Pts',(-34.0038972168544,57.9993263372425,18.5932174465876));
#48656=CARTESIAN_POINT('Ctrl Pts',(-31.8809161215889,58.4813078874833,18.4820795560196));
#48657=CARTESIAN_POINT('Ctrl Pts',(-30.3245895211199,56.9590718813698,18.3709416654516));
#48658=CARTESIAN_POINT('Ctrl Pts',(-30.7594408028035,54.8259381986264,18.2598037748835));
#48659=CARTESIAN_POINT('Ctrl Pts',(-32.7874456569645,54.0343882904504,18.1486658843155));
#48660=CARTESIAN_POINT('Ctrl Pts',(-34.5523482414506,55.3089367645812,18.0375279937474));
#48661=CARTESIAN_POINT('Ctrl Pts',(-34.4387132053247,57.4829749482845,17.9263901031794));
#48662=CARTESIAN_POINT('Ctrl Pts',(-32.5505519858621,58.5665810367465,17.8152522126113));
#48663=CARTESIAN_POINT('Ctrl Pts',(-30.6161199604413,57.5679180882692,17.7041143220433));
#48664=CARTESIAN_POINT('Ctrl Pts',(-30.4060246998813,55.4010736252019,17.5929764314752));
#48665=CARTESIAN_POINT('Ctrl Pts',(-32.112568778815,54.0493849582778,17.4818385409072));
#48666=CARTESIAN_POINT('Ctrl Pts',(-34.1737330482682,54.7500680535245,17.3707006503392));
#48667=CARTESIAN_POINT('Ctrl Pts',(-34.7029104772177,56.8617797275759,17.2595627597711));
#48668=CARTESIAN_POINT('Ctrl Pts',(-33.2157389636659,58.4516463367336,17.1484248692031));
#48669=CARTESIAN_POINT('Ctrl Pts',(-31.0734434596387,58.064444943322,17.0372869786351));
#48670=CARTESIAN_POINT('Ctrl Pts',(-30.2368913352558,56.054585373893,16.926149088067));
#48671=CARTESIAN_POINT('Ctrl Pts',(-31.471788237111,54.2617148857029,16.815011197499));
#48672=CARTESIAN_POINT('Ctrl Pts',(-33.6478190262533,54.3268681691262,16.7038733069309));
#48673=CARTESIAN_POINT('Ctrl Pts',(-34.7732380435121,56.1904096849576,16.5927354163629));
#48674=CARTESIAN_POINT('Ctrl Pts',(-33.8179364992731,58.1466187497567,16.4815975257948));
#48675=CARTESIAN_POINT('Ctrl Pts',(-31.6563127308296,58.4049550215973,16.3704596352268));
#48676=CARTESIAN_POINT('Ctrl Pts',(-30.2669254879289,56.7289603811225,16.2593217446588));
#48677=CARTESIAN_POINT('Ctrl Pts',(-30.9214966707009,54.6526917298483,16.1481838540907));
#48678=CARTESIAN_POINT('Ctrl Pts',(-33.0208898522522,54.0765813107388,16.0370459635227));
#48679=CARTESIAN_POINT('Ctrl Pts',(-34.6435066446915,55.5279495240122,15.9259080729546));
#48680=CARTESIAN_POINT('Ctrl Pts',(-34.3041474963316,57.6783425842823,15.8147701823866));
#48681=CARTESIAN_POINT('Ctrl Pts',(-32.3134316839437,58.5594813366528,15.7036322918185));
#48682=CARTESIAN_POINT('Ctrl Pts',(-30.4934839674941,57.364849487715,15.5924944012505));
#48683=CARTESIAN_POINT('Ctrl Pts',(-30.5101231301892,55.1879071179917,15.4813565106825));
#48684=CARTESIAN_POINT('Ctrl Pts',(-32.348119160257,54.0212342644067,15.3702186201144));
#48685=CARTESIAN_POINT('Ctrl Pts',(-34.3251334419918,54.9326998254003,15.2590807295464));
#48686=CARTESIAN_POINT('Ctrl Pts',(-34.6315823926477,57.088029027096,15.1479428389784));
#48687=CARTESIAN_POINT('Ctrl Pts',(-32.9869697919185,58.5144246264557,15.0368049484103));
#48688=CARTESIAN_POINT('Ctrl Pts',(-30.8966282452692,57.9062905181876,14.9256670578423));
#48689=CARTESIAN_POINT('Ctrl Pts',(-30.2738709946779,55.8202588219069,14.8145291672742));
#48690=CARTESIAN_POINT('Ctrl Pts',(-31.6887149778123,54.1656978590838,14.7033912767062));
#48691=CARTESIAN_POINT('Ctrl Pts',(-33.8461371238934,54.4570463379336,14.5922533861381));
#48692=CARTESIAN_POINT('Ctrl Pts',(-34.7714251315426,56.4276291012411,14.4811154955701));
#48693=CARTESIAN_POINT('Ctrl Pts',(-33.6176510812113,58.2737505796701,14.369977605002));
#48694=CARTESIAN_POINT('Ctrl Pts',(-31.4408800734857,58.3056324818107,14.258839714434));
#48695=CARTESIAN_POINT('Ctrl Pts',(-30.2335300381437,56.4940976767304,14.147701823866));
#48696=CARTESIAN_POINT('Ctrl Pts',(-31.1007126837241,54.4972550361147,14.0365639332979));
#48697=CARTESIAN_POINT('Ctrl Pts',(-33.2486648239747,54.1428562504465,13.9254260427299));
#48698=CARTESIAN_POINT('Ctrl Pts',(-34.7113836948143,55.7552485626327,13.8142881521619));
#48699=CARTESIAN_POINT('Ctrl Pts',(-34.149941672962,57.8586670395532,13.7031502615938));
#48700=CARTESIAN_POINT('Ctrl Pts',(-32.0784020609214,58.5276766895861,13.5920123710258));
#48701=CARTESIAN_POINT('Ctrl Pts',(-30.3925301554919,57.1502300743211,13.4808744804577));
#48702=CARTESIAN_POINT('Ctrl Pts',(-30.6361010536393,54.9865097455178,13.3697365898897));
#48703=CARTESIAN_POINT('Ctrl Pts',(-32.5848151839618,54.0182152450749,13.2585986993216));
#48704=CARTESIAN_POINT('Ctrl Pts',(-34.4577119859767,55.1291806579975,13.1474608087536));
#48705=CARTESIAN_POINT('Ctrl Pts',(-34.5350036945349,57.3075766882209,13.0363229181856));
#48706=CARTESIAN_POINT('Ctrl Pts',(-33.3501687648812,58.133739558716,12.9622309911402));
#48707=CARTESIAN_POINT('Ctrl Pts',(-32.7139713233102,58.2048901143072,12.9251850276175));
#48708=CARTESIAN_POINT('Ctrl Pts',(-34.4354702248425,56.9815444052879,22.2244449171475));
#48709=CARTESIAN_POINT('Ctrl Pts',(-34.2060643361312,57.6251343018091,22.1873989536248));
#48710=CARTESIAN_POINT('Ctrl Pts',(-33.0581520955084,58.6542106752035,22.1133070265794));
#48711=CARTESIAN_POINT('Ctrl Pts',(-30.8137923371977,58.0415178682682,22.0021691360114));
#48712=CARTESIAN_POINT('Ctrl Pts',(-30.1172800362208,55.8241524129645,21.8910312454434));
#48713=CARTESIAN_POINT('Ctrl Pts',(-31.5995489747108,54.0361783513656,21.7798933548753));
#48714=CARTESIAN_POINT('Ctrl Pts',(-33.9070787897524,54.3119235461293,21.6687554643073));
#48715=CARTESIAN_POINT('Ctrl Pts',(-34.9261604045136,56.4001058936205,21.5576175737392));
#48716=CARTESIAN_POINT('Ctrl Pts',(-33.7248161346881,58.3888336702691,21.4464796831712));
#48717=CARTESIAN_POINT('Ctrl Pts',(-31.4022507610406,58.4580789101429,21.3353417926031));
#48718=CARTESIAN_POINT('Ctrl Pts',(-30.0845341595457,56.5443222204948,21.2242039020351));
#48719=CARTESIAN_POINT('Ctrl Pts',(-30.9776876418977,54.3993159620291,21.113066011467));
#48720=CARTESIAN_POINT('Ctrl Pts',(-33.2642474718997,53.9863741397618,21.001928120899));
#48721=CARTESIAN_POINT('Ctrl Pts',(-34.8512746399183,55.6834843462922,20.8907902303309));
#48722=CARTESIAN_POINT('Ctrl Pts',(-34.2861576030319,57.9372537407841,20.7796523397629));
#48723=CARTESIAN_POINT('Ctrl Pts',(-32.0861481883531,58.6847859443394,20.6685144491949));
#48724=CARTESIAN_POINT('Ctrl Pts',(-30.2649430630365,57.2418541016518,20.5573765586268));
#48725=CARTESIAN_POINT('Ctrl Pts',(-30.4895103834619,54.9291911672537,20.4462386680588));
#48726=CARTESIAN_POINT('Ctrl Pts',(-32.5543019081473,53.8636032153705,20.3351007774908));
#48727=CARTESIAN_POINT('Ctrl Pts',(-34.5693901517228,55.0204352512209,20.2239628869227));
#48728=CARTESIAN_POINT('Ctrl Pts',(-34.6903421852682,57.3408256590054,20.1128249963547));
#48729=CARTESIAN_POINT('Ctrl Pts',(-32.8064491443347,58.7008948504121,20.0016871057866));
#48730=CARTESIAN_POINT('Ctrl Pts',(-30.6420597422744,57.8557560368672,19.8905492152186));
#48731=CARTESIAN_POINT('Ctrl Pts',(-30.1782641205668,55.5789743756422,19.7794113246505));
#48732=CARTESIAN_POINT('Ctrl Pts',(-31.8395796835861,53.9545139333702,19.6682734340825));
#48733=CARTESIAN_POINT('Ctrl Pts',(-34.1053854498936,54.4692617796665,19.5571355435145));
#48734=CARTESIAN_POINT('Ctrl Pts',(-34.9017637086039,56.6520633710957,19.4459976529464));
#48735=CARTESIAN_POINT('Ctrl Pts',(-33.4997804064767,58.5049756574094,19.3348597623784));
#48736=CARTESIAN_POINT('Ctrl Pts',(-31.1826867602698,58.3320070089704,19.2237218718103));
#48737=CARTESIAN_POINT('Ctrl Pts',(-30.0713448616116,56.2914775915524,19.1125839812423));
#48738=CARTESIAN_POINT('Ctrl Pts',(-31.1829785540051,54.2511071219659,19.0014460906742));
#48739=CARTESIAN_POINT('Ctrl Pts',(-33.5000969119257,54.0784698304632,18.8903082001062));
#48740=CARTESIAN_POINT('Ctrl Pts',(-34.9018152245058,55.9315825877643,18.7791703095382));
#48741=CARTESIAN_POINT('Ctrl Pts',(-34.1051248236508,58.1142702713998,18.6680324189701));
#48742=CARTESIAN_POINT('Ctrl Pts',(-31.8392454683584,58.628694091168,18.5568945284021));
#48743=CARTESIAN_POINT('Ctrl Pts',(-30.1781622293418,57.0039960908762,18.445756637834));
#48744=CARTESIAN_POINT('Ctrl Pts',(-30.6422834332407,54.7272807755181,18.334618747266));
#48745=CARTESIAN_POINT('Ctrl Pts',(-32.8067936786327,53.8824514929496,18.223480856698));
#48746=CARTESIAN_POINT('Ctrl Pts',(-34.6904921906955,55.242790066521,18.1123429661299));
#48747=CARTESIAN_POINT('Ctrl Pts',(-34.5692083587435,57.5631631725538,18.0012050755619));
#48748=CARTESIAN_POINT('Ctrl Pts',(-32.5539546496148,58.7197069922753,17.8900671849939));
#48749=CARTESIAN_POINT('Ctrl Pts',(-30.4893156378063,57.6538238513956,17.7789292944258));
#48750=CARTESIAN_POINT('Ctrl Pts',(-30.2650788254252,55.3411286766987,17.6677914038578));
#48751=CARTESIAN_POINT('Ctrl Pts',(-32.0864907098624,53.8984575893318,17.5566535132897));
#48752=CARTESIAN_POINT('Ctrl Pts',(-34.2863923370768,54.6463037965648,17.4455156227217));
#48753=CARTESIAN_POINT('Ctrl Pts',(-34.8511887990978,56.9001551837646,17.3343777321536));
#48754=CARTESIAN_POINT('Ctrl Pts',(-33.26391548901,58.5970360158137,17.2232398415856));
#48755=CARTESIAN_POINT('Ctrl Pts',(-30.9774216684405,58.1837720232006,17.1121019510176));
#48756=CARTESIAN_POINT('Ctrl Pts',(-30.0845610619601,56.0386284250959,17.0009640604495));
#48757=CARTESIAN_POINT('Ctrl Pts',(-31.4025791084081,54.1250794844285,16.8898261698815));
#48758=CARTESIAN_POINT('Ctrl Pts',(-33.72507894253,54.1946182477114,16.7786882793134));
#48759=CARTESIAN_POINT('Ctrl Pts',(-34.9262501272131,56.1835950962899,16.6675503887454));
#48760=CARTESIAN_POINT('Ctrl Pts',(-33.9066470549119,58.2714769641261,16.5564124981773));
#48761=CARTESIAN_POINT('Ctrl Pts',(-31.5995239807838,58.5472018994032,16.4452746076093));
#48762=CARTESIAN_POINT('Ctrl Pts',(-30.1166168191438,56.7583957419196,16.3341367170413));
#48763=CARTESIAN_POINT('Ctrl Pts',(-30.8152473123311,54.5423730540801,16.2229988264732));
#48764=CARTESIAN_POINT('Ctrl Pts',(-33.0559510469649,53.9274845334332,16.1118609359052));
#48765=CARTESIAN_POINT('Ctrl Pts',(-34.7877864833416,55.4765446163128,16.0007230453371));
#48766=CARTESIAN_POINT('Ctrl Pts',(-34.4255850063652,57.7716810411711,15.8895851547691));
#48767=CARTESIAN_POINT('Ctrl Pts',(-32.3008737352177,58.7121294100224,15.778447264201));
#48768=CARTESIAN_POINT('Ctrl Pts',(-30.3584249929228,57.4370866648374,15.667309373633));
#48769=CARTESIAN_POINT('Ctrl Pts',(-30.3761841408135,55.1136138914731,15.5561714830649));
#48770=CARTESIAN_POINT('Ctrl Pts',(-32.3378960321382,53.868412066919,15.4450335924969));
#48771=CARTESIAN_POINT('Ctrl Pts',(-34.4479835200066,54.8412285476315,15.3338957019289));
#48772=CARTESIAN_POINT('Ctrl Pts',(-34.7750596076319,57.1416333665308,15.2227578113608));
#48773=CARTESIAN_POINT('Ctrl Pts',(-33.0197478209391,58.6640399241194,15.1116199207928));
#48774=CARTESIAN_POINT('Ctrl Pts',(-30.7887049884687,58.0149721937252,15.0004820302248));
#48775=CARTESIAN_POINT('Ctrl Pts',(-30.1240298292691,55.7885293084689,14.8893441396567));
#48776=CARTESIAN_POINT('Ctrl Pts',(-31.6341072291541,54.0225995335433,14.7782062490887));
#48777=CARTESIAN_POINT('Ctrl Pts',(-33.9367458689222,54.3335587337424,14.6670683585206));
#48778=CARTESIAN_POINT('Ctrl Pts',(-34.9243151877952,56.4367817964587,14.5559304679526));
#48779=CARTESIAN_POINT('Ctrl Pts',(-33.6928803873875,58.4071660616143,14.4447925773845));
#48780=CARTESIAN_POINT('Ctrl Pts',(-31.3695905104292,58.4411939406326,14.3336546868165));
#48781=CARTESIAN_POINT('Ctrl Pts',(-30.0809735153022,56.5077243843662,14.2225167962484));
#48782=CARTESIAN_POINT('Ctrl Pts',(-31.0065263891691,54.3764738870215,14.1113789056804));
#48783=CARTESIAN_POINT('Ctrl Pts',(-33.2990575952188,53.998220451898,14.0002410151124));
#48784=CARTESIAN_POINT('Ctrl Pts',(-34.8602323505772,55.7191431963174,13.8891031245444));
#48785=CARTESIAN_POINT('Ctrl Pts',(-34.2609995597881,57.9641431697148,13.7779652339763));
#48786=CARTESIAN_POINT('Ctrl Pts',(-32.0500242237096,58.6781839861315,13.6668273434083));
#48787=CARTESIAN_POINT('Ctrl Pts',(-30.2506759606945,57.2080211780376,13.5556894528402));
#48788=CARTESIAN_POINT('Ctrl Pts',(-30.5106416621758,54.8986604236741,13.4445515622722));
#48789=CARTESIAN_POINT('Ctrl Pts',(-32.5905241100747,53.8651898368236,13.3334136717041));
#48790=CARTESIAN_POINT('Ctrl Pts',(-34.5894859509232,55.0509345423224,13.2222757811361));
#48791=CARTESIAN_POINT('Ctrl Pts',(-34.6719801790384,57.3759588223509,13.111137890568));
#48792=CARTESIAN_POINT('Ctrl Pts',(-33.4073937856322,58.2577308722945,13.0370459635227));
#48793=CARTESIAN_POINT('Ctrl Pts',(-32.7283737736498,58.3336705852723,13.));
#48794=CARTESIAN_POINT('Ctrl Pts',(-34.0692874532608,56.8510195406194,22.));
#48795=CARTESIAN_POINT('Ctrl Pts',(-34.0553305059911,56.9114179004355,22.));
#48796=CARTESIAN_POINT('Ctrl Pts',(-34.0377835201519,56.9707365361911,22.));
#48797=CARTESIAN_POINT('Ctrl Pts',(-34.016946081917,57.0288042521019,22.));
#48798=CARTESIAN_POINT('Ctrl Pts',(-33.9947315403611,57.0907095436074,22.));
#48799=CARTESIAN_POINT('Ctrl Pts',(-33.9687774174665,57.1511938546424,22.));
#48800=CARTESIAN_POINT('Ctrl Pts',(-33.939384889976,57.2100521415623,22.));
#48801=CARTESIAN_POINT('Ctrl Pts',(-33.9136664284218,57.2615531426173,22.));
#48802=CARTESIAN_POINT('Ctrl Pts',(-33.885314254798,57.3118096210154,22.));
#48803=CARTESIAN_POINT('Ctrl Pts',(-33.8544948148318,57.3606781624761,22.));
#48804=CARTESIAN_POINT('Ctrl Pts',(-33.8390317669697,57.3851969920325,22.));
#48805=CARTESIAN_POINT('Ctrl Pts',(-33.8229471373064,57.4093662970835,22.));
#48806=CARTESIAN_POINT('Ctrl Pts',(-33.806259181183,57.4331668560883,22.));
#48807=CARTESIAN_POINT('Ctrl Pts',(-33.7986346988757,57.4440409822962,22.));
#48808=CARTESIAN_POINT('Ctrl Pts',(-33.7908831157288,57.4548394645451,22.));
#48809=CARTESIAN_POINT('Ctrl Pts',(-33.7830191798836,57.4655431488209,22.));
#48810=CARTESIAN_POINT('Ctrl Pts',(-33.7433624664543,57.5195203109348,22.));
#48811=CARTESIAN_POINT('Ctrl Pts',(-33.7007840161423,57.5711878025655,22.));
#48812=CARTESIAN_POINT('Ctrl Pts',(-33.6555819716312,57.6203464168009,22.));
#48813=CARTESIAN_POINT('Ctrl Pts',(-33.6095776367408,57.6703775465096,22.));
#48814=CARTESIAN_POINT('Ctrl Pts',(-33.5608552988351,57.7178108518149,22.));
#48815=CARTESIAN_POINT('Ctrl Pts',(-33.5096779793303,57.7624205360032,22.));
#48816=CARTESIAN_POINT('Ctrl Pts',(-33.4668687974939,57.7997359737901,22.));
#48817=CARTESIAN_POINT('Ctrl Pts',(-33.4223407451604,57.8350756826701,22.));
#48818=CARTESIAN_POINT('Ctrl Pts',(-33.3762247080186,57.8682921421139,22.));
#48819=CARTESIAN_POINT('Ctrl Pts',(-33.3549779646827,57.8835957465012,22.));
#48820=CARTESIAN_POINT('Ctrl Pts',(-33.3333938801953,57.8984484230221,22.));
#48821=CARTESIAN_POINT('Ctrl Pts',(-33.3114840049174,57.912834383224,22.));
#48822=CARTESIAN_POINT('Ctrl Pts',(-33.3019191647998,57.919114629347,22.));
#48823=CARTESIAN_POINT('Ctrl Pts',(-33.2922923778332,57.9253057103697,22.));
#48824=CARTESIAN_POINT('Ctrl Pts',(-33.2826166375141,57.9313989825554,22.));
#48825=CARTESIAN_POINT('Ctrl Pts',(-33.2232320152636,57.9687962932603,22.));
#48826=CARTESIAN_POINT('Ctrl Pts',(-33.1618957173518,58.0025854530302,22.));
#48827=CARTESIAN_POINT('Ctrl Pts',(-33.0988929672382,58.0325387704092,22.));
#48828=CARTESIAN_POINT('Ctrl Pts',(-33.0425620163395,58.0593201227707,22.));
#48829=CARTESIAN_POINT('Ctrl Pts',(-32.9848978605312,58.0830352046557,22.));
#48830=CARTESIAN_POINT('Ctrl Pts',(-32.9260772832472,58.1034986372925,22.));
#48831=CARTESIAN_POINT('Ctrl Pts',(-32.8619970286523,58.1257918896507,22.));
#48832=CARTESIAN_POINT('Ctrl Pts',(-32.7965441149127,58.1442273323773,22.));
#48833=CARTESIAN_POINT('Ctrl Pts',(-32.7300260672774,58.1589105502835,22.));
#48834=CARTESIAN_POINT('Ctrl Pts',(-32.7043629429456,58.1645754376354,22.));
#48835=CARTESIAN_POINT('Ctrl Pts',(-32.6785410407311,58.1696813145167,22.));
#48836=CARTESIAN_POINT('Ctrl Pts',(-32.6525772949456,58.1742323470501,22.));
#48837=CARTESIAN_POINT('Ctrl Pts',(-32.6411872717747,58.1762288373267,22.));
#48838=CARTESIAN_POINT('Ctrl Pts',(-32.6297705135126,58.1781183496289,22.));
#48839=CARTESIAN_POINT('Ctrl Pts',(-32.6183418171519,58.179899377155,22.));
#48840=CARTESIAN_POINT('Ctrl Pts',(-32.5492442274088,58.1906674215093,22.));
#48841=CARTESIAN_POINT('Ctrl Pts',(-32.4795878660141,58.1974963222478,22.));
#48842=CARTESIAN_POINT('Ctrl Pts',(-32.4097184968443,58.2005474581331,22.));
#48843=CARTESIAN_POINT('Ctrl Pts',(-32.3382311065414,58.2036692516242,22.));
#48844=CARTESIAN_POINT('Ctrl Pts',(-32.2665198680424,58.2028364327149,22.));
#48845=CARTESIAN_POINT('Ctrl Pts',(-32.1949302795206,58.1981713779267,22.));
#48846=CARTESIAN_POINT('Ctrl Pts',(-32.1401596273381,58.1946023101545,22.));
#48847=CARTESIAN_POINT('Ctrl Pts',(-32.0854595447284,58.188789106956,22.));
#48848=CARTESIAN_POINT('Ctrl Pts',(-32.0309802701514,58.1807666255737,22.));
#48849=CARTESIAN_POINT('Ctrl Pts',(-31.9970690900808,58.1757729502195,22.));
#48850=CARTESIAN_POINT('Ctrl Pts',(-31.9632434082658,58.169922934266,22.));
#48851=CARTESIAN_POINT('Ctrl Pts',(-31.9295394677765,58.1632216306335,22.));
#48852=CARTESIAN_POINT('Ctrl Pts',(-31.9106295176357,58.1594617937797,22.));
#48853=CARTESIAN_POINT('Ctrl Pts',(-31.8917516814693,58.155432366928,22.));
#48854=CARTESIAN_POINT('Ctrl Pts',(-31.8729463796414,58.1511420898627,22.));
#48855=CARTESIAN_POINT('Ctrl Pts',(-31.800021211719,58.1345048043629,22.));
#48856=CARTESIAN_POINT('Ctrl Pts',(-31.7281115870151,58.1139365946459,22.));
#48857=CARTESIAN_POINT('Ctrl Pts',(-31.657588471888,58.0895522802274,22.));
#48858=CARTESIAN_POINT('Ctrl Pts',(-31.604840310165,58.071313894726,22.));
#48859=CARTESIAN_POINT('Ctrl Pts',(-31.5528674075064,58.0509395358675,22.));
#48860=CARTESIAN_POINT('Ctrl Pts',(-31.5018252351889,58.0284581681865,22.));
#48861=CARTESIAN_POINT('Ctrl Pts',(-31.4859023718045,58.0214449920221,22.));
#48862=CARTESIAN_POINT('Ctrl Pts',(-31.4700701035993,58.0142266520307,22.));
#48863=CARTESIAN_POINT('Ctrl Pts',(-31.4543332256613,58.00680370711,22.));
#48864=CARTESIAN_POINT('Ctrl Pts',(-31.4391437429754,57.999638963646,22.));
#48865=CARTESIAN_POINT('Ctrl Pts',(-31.4240509122303,57.9922872148405,22.));
#48866=CARTESIAN_POINT('Ctrl Pts',(-31.4090641623582,57.9847522751755,22.));
#48867=CARTESIAN_POINT('Ctrl Pts',(-31.341765130632,57.9509161100361,22.));
#48868=CARTESIAN_POINT('Ctrl Pts',(-31.2765704047312,57.9133737616798,22.));
#48869=CARTESIAN_POINT('Ctrl Pts',(-31.213852322156,57.8722119391998,22.));
#48870=CARTESIAN_POINT('Ctrl Pts',(-31.1658528011761,57.8407098957608,22.));
#48871=CARTESIAN_POINT('Ctrl Pts',(-31.1193037579286,57.807086816115,22.));
#48872=CARTESIAN_POINT('Ctrl Pts',(-31.0743783982804,57.7713618605751,22.));
#48873=CARTESIAN_POINT('Ctrl Pts',(-31.0639523774024,57.7630710169348,22.));
#48874=CARTESIAN_POINT('Ctrl Pts',(-31.0536138415293,57.7546668979799,22.));
#48875=CARTESIAN_POINT('Ctrl Pts',(-31.0433632440414,57.7461514510325,22.));
#48876=CARTESIAN_POINT('Ctrl Pts',(-31.6652099567911,54.8483531313949,20.8714803633902));
#48877=CARTESIAN_POINT('Ctrl Pts',(-31.5910191767377,54.8903425066551,20.8771939403667));
#48878=CARTESIAN_POINT('Ctrl Pts',(-31.5202697708326,54.9380868086678,20.8829075173431));
#48879=CARTESIAN_POINT('Ctrl Pts',(-31.453999322188,54.9913986485313,20.8886210943196));
#48880=CARTESIAN_POINT('Ctrl Pts',(-31.0243118193789,55.3370645042722,20.9256670578423));
#48881=CARTESIAN_POINT('Ctrl Pts',(-30.7829209443173,55.9167912231112,20.9627130213649));
#48882=CARTESIAN_POINT('Ctrl Pts',(-30.840293873424,56.4652682536955,20.9997589848876));
#48883=CARTESIAN_POINT('Ctrl Pts',(-30.8976668025307,57.0137452842797,21.0368049484103));
#48884=CARTESIAN_POINT('Ctrl Pts',(-31.2538035358057,57.530972626609,21.073850911933));
#48885=CARTESIAN_POINT('Ctrl Pts',(-31.7457295422612,57.780228908827,21.1108968754557));
#48886=CARTESIAN_POINT('Ctrl Pts',(-32.2376555487168,58.0294851910449,21.1479428389784));
#48887=CARTESIAN_POINT('Ctrl Pts',(-32.8653708283529,58.0107704131515,21.184988802501));
#48888=CARTESIAN_POINT('Ctrl Pts',(-33.3415709716004,57.7326682072443,21.2220347660237));
#48889=CARTESIAN_POINT('Ctrl Pts',(-33.8177711148478,57.4545660013371,21.2590807295464));
#48890=CARTESIAN_POINT('Ctrl Pts',(-34.1424561217066,56.9170763674162,21.2961266930691));
#48891=CARTESIAN_POINT('Ctrl Pts',(-34.1670860104471,56.3661470356389,21.3331726565918));
#48892=CARTESIAN_POINT('Ctrl Pts',(-34.1917158991876,55.8152177038615,21.3702186201144));
#48893=CARTESIAN_POINT('Ctrl Pts',(-33.9162906698098,55.2508486742278,21.4072645836371));
#48894=CARTESIAN_POINT('Ctrl Pts',(-33.4667522310661,54.9314015975034,21.4443105471598));
#48895=CARTESIAN_POINT('Ctrl Pts',(-33.0172137923224,54.611954520779,21.4813565106825));
#48896=CARTESIAN_POINT('Ctrl Pts',(-32.3935621442129,54.537429396964,21.5184024742052));
#48897=CARTESIAN_POINT('Ctrl Pts',(-31.881431331593,54.741782991655,21.5554484377278));
#48898=CARTESIAN_POINT('Ctrl Pts',(-31.8075551488135,54.7712615216341,21.5607924129486));
#48899=CARTESIAN_POINT('Ctrl Pts',(-31.7359995810404,54.8065431837031,21.5661363881694));
#48900=CARTESIAN_POINT('Ctrl Pts',(-31.6673136634551,54.8469650373412,21.5714803633902));
#48901=CARTESIAN_POINT('Ctrl Pts',(-30.5157034944334,56.8250975324092,22.));
#48902=CARTESIAN_POINT('Ctrl Pts',(-30.3383199129809,56.1652717359214,21.9629540364773));
#48903=CARTESIAN_POINT('Ctrl Pts',(-30.6971298707754,54.6659551967235,21.8888621094319));
#48904=CARTESIAN_POINT('Ctrl Pts',(-32.8915770858134,53.8933186298579,21.7777242188639));
#48905=CARTESIAN_POINT('Ctrl Pts',(-34.7256560234758,55.3208993649632,21.6665863282959));
#48906=CARTESIAN_POINT('Ctrl Pts',(-34.5234929724835,57.6345755616839,21.5554484377278));
#48907=CARTESIAN_POINT('Ctrl Pts',(-32.4687454188576,58.7202753686331,21.4443105471598));
#48908=CARTESIAN_POINT('Ctrl Pts',(-30.4428342940784,57.5824199368057,21.3331726565918));
#48909=CARTESIAN_POINT('Ctrl Pts',(-30.2997559892122,55.2634130835606,21.2220347660237));
#48910=CARTESIAN_POINT('Ctrl Pts',(-32.1706430815575,53.8854124812075,21.1108968754557));
#48911=CARTESIAN_POINT('Ctrl Pts',(-34.3429657642117,54.7099453599152,20.9997589848876));
#48912=CARTESIAN_POINT('Ctrl Pts',(-34.8284152391772,56.982193672835,20.8886210943196));
#48913=CARTESIAN_POINT('Ctrl Pts',(-33.18263271582,58.6223996095027,20.7774832037515));
#48914=CARTESIAN_POINT('Ctrl Pts',(-30.9120322857352,58.129235673502,20.6663453131835));
#48915=CARTESIAN_POINT('Ctrl Pts',(-30.0949149346207,55.954114599854,20.5552074226154));
#48916=CARTESIAN_POINT('Ctrl Pts',(-31.479200108132,54.0879422836221,20.4440695320474));
#48917=CARTESIAN_POINT('Ctrl Pts',(-33.7978345552325,54.2388509530007,20.3329316414794));
#48918=CARTESIAN_POINT('Ctrl Pts',(-34.9285465373885,56.2687104209715,20.2217937509113));
#48919=CARTESIAN_POINT('Ctrl Pts',(-33.8363822214011,58.3195681810162,20.1106558603433));
#48920=CARTESIAN_POINT('Ctrl Pts',(-31.5210121579647,58.5142504249981,19.9995179697753));
#48921=CARTESIAN_POINT('Ctrl Pts',(-30.101720741136,56.674562508041,19.8883800792072));
#48922=CARTESIAN_POINT('Ctrl Pts',(-30.8776015421155,54.484391533643,19.7772421886392));
#48923=CARTESIAN_POINT('Ctrl Pts',(-33.1384820439344,53.9484258880499,19.6661042980711));
#48924=CARTESIAN_POINT('Ctrl Pts',(-34.8149526935152,55.5572409773789,19.5549664075031));
#48925=CARTESIAN_POINT('Ctrl Pts',(-34.3725208876465,57.8382701189333,19.443828516935));
#48926=CARTESIAN_POINT('Ctrl Pts',(-32.2161494783462,58.7036614639378,19.332690626367));
#48927=CARTESIAN_POINT('Ctrl Pts',(-30.3195896701686,57.3613125035425,19.221552735799));
#48928=CARTESIAN_POINT('Ctrl Pts',(-30.4187841646359,55.039890462752,19.1104148452309));
#48929=CARTESIAN_POINT('Ctrl Pts',(-32.4229391156973,53.8642192630766,18.9992769546629));
#48930=CARTESIAN_POINT('Ctrl Pts',(-34.4976287681445,54.9104040861686,18.8881390640948));
#48931=CARTESIAN_POINT('Ctrl Pts',(-34.7438661544312,57.2208600991234,18.7770011735268));
#48932=CARTESIAN_POINT('Ctrl Pts',(-32.9362674024074,58.680800710823,18.6658632829587));
#48933=CARTESIAN_POINT('Ctrl Pts',(-30.7293481493446,57.9539257225797,18.5547253923907));
#48934=CARTESIAN_POINT('Ctrl Pts',(-30.1431266157477,55.7055520544288,18.4435875018226));
#48935=CARTESIAN_POINT('Ctrl Pts',(-31.7141780195174,53.9936416231339,18.3324496112546));
#48936=CARTESIAN_POINT('Ctrl Pts',(-34.004501193851,54.3851254608372,18.2213117206866));
#48937=CARTESIAN_POINT('Ctrl Pts',(-34.9177373632483,56.5216739711636,18.1101738301186));
#48938=CARTESIAN_POINT('Ctrl Pts',(-33.6179911050581,58.4476800725015,17.9990359395505));
#48939=CARTESIAN_POINT('Ctrl Pts',(-31.2949349095266,58.4002485379024,17.8878980489825));
#48940=CARTESIAN_POINT('Ctrl Pts',(-30.0748884576731,56.4227939888947,17.7767601584144));
#48941=CARTESIAN_POINT('Ctrl Pts',(-31.0745741031468,54.3253030000451,17.6656222678464));
#48942=CARTESIAN_POINT('Ctrl Pts',(-33.3789682374394,54.0276328606133,17.5544843772783));
#48943=CARTESIAN_POINT('Ctrl Pts',(-34.8788327758259,55.8022444250302,17.4433464867103));
#48944=CARTESIAN_POINT('Ctrl Pts',(-34.2013246967004,58.0248156029211,17.3322085961422));
#48945=CARTESIAN_POINT('Ctrl Pts',(-31.9665748283507,58.6610017894909,17.2210707055742));
#48946=CARTESIAN_POINT('Ctrl Pts',(-30.2200750690644,57.1284945533303,17.1099328150062));
#48947=CARTESIAN_POINT('Ctrl Pts',(-30.5604164551708,54.8300151475111,16.9987949244381));
#48948=CARTESIAN_POINT('Ctrl Pts',(-32.6760806562328,53.8693878387091,16.8876570338701));
#48949=CARTESIAN_POINT('Ctrl Pts',(-34.6305762357544,55.1258856969253,16.776519143302));
#48950=CARTESIAN_POINT('Ctrl Pts',(-34.6349312243122,57.4494219828794,16.665381252734));
#48951=CARTESIAN_POINT('Ctrl Pts',(-32.6851594514901,58.7132375833447,16.554243362166));
#48952=CARTESIAN_POINT('Ctrl Pts',(-30.5659091328683,57.7605477465697,16.4431054715979));
#48953=CARTESIAN_POINT('Ctrl Pts',(-30.2169541190139,55.4633602843958,16.3319675810299));
#48954=CARTESIAN_POINT('Ctrl Pts',(-31.9576968915284,53.9243169328215,16.2208296904618));
#48955=CARTESIAN_POINT('Ctrl Pts',(-34.1948158493603,54.5521215254953,16.1096917998938));
#48956=CARTESIAN_POINT('Ctrl Pts',(-34.880650639758,56.7721373989267,15.9985539093257));
#48957=CARTESIAN_POINT('Ctrl Pts',(-33.387448901162,58.5523588475275,15.8874160187577));
#48958=CARTESIAN_POINT('Ctrl Pts',(-31.0819551189948,58.2633289901972,15.7762781281897));
#48959=CARTESIAN_POINT('Ctrl Pts',(-30.0744138980993,56.1696001333951,15.6651402376216));
#48960=CARTESIAN_POINT('Ctrl Pts',(-31.2870391443611,54.1875860438059,15.5540023470536));
#48961=CARTESIAN_POINT('Ctrl Pts',(-33.6099012175602,54.1314466960921,15.4428644564855));
#48962=CARTESIAN_POINT('Ctrl Pts',(-34.916858119472,56.052567070093,15.3317265659175));
#48963=CARTESIAN_POINT('Ctrl Pts',(-34.0116373750326,58.1925239040739,15.2205886753494));
#48964=CARTESIAN_POINT('Ctrl Pts',(-31.722797799219,58.5925904319764,15.1094507847814));
#48965=CARTESIAN_POINT('Ctrl Pts',(-30.1453402095974,56.8865812380663,14.9983128942134));
#48966=CARTESIAN_POINT('Ctrl Pts',(-30.723129434303,54.6360258563356,14.8871750036453));
#48967=CARTESIAN_POINT('Ctrl Pts',(-32.9273084298409,53.9008832080614,14.7760371130773));
#48968=CARTESIAN_POINT('Ctrl Pts',(-34.7403671916158,55.3540375815297,14.6648992225092));
#48969=CARTESIAN_POINT('Ctrl Pts',(-34.5027924192342,57.6654005284895,14.5537613319412));
#48970=CARTESIAN_POINT('Ctrl Pts',(-32.4320391047204,58.7193548713018,14.4426234413732));
#48971=CARTESIAN_POINT('Ctrl Pts',(-30.4234910234841,57.5512051672244,14.3314855508051));
#48972=CARTESIAN_POINT('Ctrl Pts',(-30.3155954476549,55.2301702471531,14.2203476602371));
#48973=CARTESIAN_POINT('Ctrl Pts',(-32.2071095510683,53.8807233800597,14.109209769669));
#48974=CARTESIAN_POINT('Ctrl Pts',(-34.3667107654438,54.7380212138031,13.998071879101));
#48975=CARTESIAN_POINT('Ctrl Pts',(-34.817688121868,57.0173840749687,13.886933988533));
#48976=CARTESIAN_POINT('Ctrl Pts',(-33.1472639077745,58.6324557555082,13.7757960979649));
#48977=CARTESIAN_POINT('Ctrl Pts',(-30.8843823888258,58.105001931136,13.6646582073969));
#48978=CARTESIAN_POINT('Ctrl Pts',(-30.1003126229301,55.9176887906373,13.5535203168288));
#48979=CARTESIAN_POINT('Ctrl Pts',(-31.5126666412309,54.0728255670593,13.4423824262608));
#48980=CARTESIAN_POINT('Ctrl Pts',(-33.8288126996591,54.2585627611561,13.3312445356927));
#48981=CARTESIAN_POINT('Ctrl Pts',(-34.9285321027134,56.3058411531895,13.2201066451247));
#48982=CARTESIAN_POINT('Ctrl Pts',(-33.8056871835127,58.3388651889263,13.1089687545567));
#48983=CARTESIAN_POINT('Ctrl Pts',(-31.4871369476881,58.5005967837941,12.9978308639886));
#48984=CARTESIAN_POINT('Ctrl Pts',(-30.0968376198179,56.6352191751131,12.8866929734206));
#48985=CARTESIAN_POINT('Ctrl Pts',(-30.6354003368774,55.1906968075748,12.8126010463752));
#48986=CARTESIAN_POINT('Ctrl Pts',(-31.1506898940642,54.7420190959221,12.7755550828525));
#48987=CARTESIAN_POINT('Ctrl Pts',(-30.6408436601533,56.7914556061658,22.0748149723825));
#48988=CARTESIAN_POINT('Ctrl Pts',(-30.4746468195517,56.1732418919888,22.0377690088598));
#48989=CARTESIAN_POINT('Ctrl Pts',(-30.8108283357527,54.7684801331151,21.9636770818145));
#48990=CARTESIAN_POINT('Ctrl Pts',(-32.8668821769258,54.0445700885951,21.8525391912464));
#48991=CARTESIAN_POINT('Ctrl Pts',(-34.5852944581392,55.3821200801757,21.7414013006784));
#48992=CARTESIAN_POINT('Ctrl Pts',(-34.3958808715705,57.5498836968622,21.6302634101103));
#48993=CARTESIAN_POINT('Ctrl Pts',(-32.4707164969967,58.5671135683041,21.5191255195423));
#48994=CARTESIAN_POINT('Ctrl Pts',(-30.5725699745224,57.5010172797825,21.4079876289743));
#48995=CARTESIAN_POINT('Ctrl Pts',(-30.4385149394808,55.3282591857861,21.2968497384062));
#48996=CARTESIAN_POINT('Ctrl Pts',(-32.1914140597048,54.0371625432278,21.1857118478382));
#48997=CARTESIAN_POINT('Ctrl Pts',(-34.2267386577774,54.8096960454343,21.0745739572701));
#48998=CARTESIAN_POINT('Ctrl Pts',(-34.6815731376677,56.9386444383885,20.9634360667021));
#48999=CARTESIAN_POINT('Ctrl Pts',(-33.1395823093187,58.4754103689113,20.852298176134));
#49000=CARTESIAN_POINT('Ctrl Pts',(-31.0121778750478,58.0133479424405,20.741160285566));
#49001=CARTESIAN_POINT('Ctrl Pts',(-30.2465922382936,55.9754014346164,20.6300223949979));
#49002=CARTESIAN_POINT('Ctrl Pts',(-31.5435771139257,54.2269197519467,20.5188845044299));
#49003=CARTESIAN_POINT('Ctrl Pts',(-33.715986287666,54.3683113275635,20.4077466138618));
#49004=CARTESIAN_POINT('Ctrl Pts',(-34.7753896299934,56.2701571899581,20.2966087232938));
#49005=CARTESIAN_POINT('Ctrl Pts',(-33.7521029354263,58.1916770817759,20.1854708327258));
#49006=CARTESIAN_POINT('Ctrl Pts',(-31.5827522761609,58.3740816403381,20.0743329421577));
#49007=CARTESIAN_POINT('Ctrl Pts',(-30.2529688348836,56.6504141115413,19.9631950515897));
#49008=CARTESIAN_POINT('Ctrl Pts',(-30.9799185150648,54.5983668288005,19.8520571610217));
#49009=CARTESIAN_POINT('Ctrl Pts',(-33.0982160108274,54.0962019934802,19.7409192704536));
#49010=CARTESIAN_POINT('Ctrl Pts',(-34.6689596108848,55.6035567484657,19.6297813798856));
#49011=CARTESIAN_POINT('Ctrl Pts',(-34.2544298798073,57.7407322048549,19.5186434893175));
#49012=CARTESIAN_POINT('Ctrl Pts',(-32.2340505839621,58.55154742375,19.4075055987495));
#49013=CARTESIAN_POINT('Ctrl Pts',(-30.4570978042841,57.2938540432474,19.2963677081815));
#49014=CARTESIAN_POINT('Ctrl Pts',(-30.5500365726333,55.1188330761248,19.1852298176134));
#49015=CARTESIAN_POINT('Ctrl Pts',(-32.4277989800397,54.017305880809,19.0740919270454));
#49016=CARTESIAN_POINT('Ctrl Pts',(-34.3716477998814,54.9975127909389,18.9629540364773));
#49017=CARTESIAN_POINT('Ctrl Pts',(-34.6023561625368,57.1622593055708,18.8518161459093));
#49018=CARTESIAN_POINT('Ctrl Pts',(-32.9087540872943,58.5301283898668,18.7406782553412));
#49019=CARTESIAN_POINT('Ctrl Pts',(-30.8410147603585,57.8490939583302,18.6295403647732));
#49020=CARTESIAN_POINT('Ctrl Pts',(-30.2917634374419,55.7425145495773,18.5184024742052));
#49021=CARTESIAN_POINT('Ctrl Pts',(-31.7637360833391,54.1385661866875,18.4072645836371));
#49022=CARTESIAN_POINT('Ctrl Pts',(-33.9096194419575,54.505360996219,18.2961266930691));
#49023=CARTESIAN_POINT('Ctrl Pts',(-34.7652621391801,56.507167529275,18.184988802501));
#49024=CARTESIAN_POINT('Ctrl Pts',(-33.5474847105914,58.3117095641174,18.073850911933));
#49025=CARTESIAN_POINT('Ctrl Pts',(-31.3709326471137,58.2672693113572,17.9627130213649));
#49026=CARTESIAN_POINT('Ctrl Pts',(-30.2278287362276,56.4145234383322,17.8515751307969));
#49027=CARTESIAN_POINT('Ctrl Pts',(-31.164468951247,54.4493112541897,17.7404372402288));
#49028=CARTESIAN_POINT('Ctrl Pts',(-33.3235358811423,54.1704137580971,17.6292993496608));
#49029=CARTESIAN_POINT('Ctrl Pts',(-34.7288110794959,55.8331089911408,17.5181614590927));
#49030=CARTESIAN_POINT('Ctrl Pts',(-34.0940302203501,57.9155131502695,17.4070235685248));
#49031=CARTESIAN_POINT('Ctrl Pts',(-32.0002154229856,58.5115780925632,17.2958856779567));
#49032=CARTESIAN_POINT('Ctrl Pts',(-30.363859116905,57.0757188165044,17.1847477873887));
#49033=CARTESIAN_POINT('Ctrl Pts',(-30.6827367866064,54.9221936012213,17.0736098968206));
#49034=CARTESIAN_POINT('Ctrl Pts',(-32.6649760846936,54.0221484988997,16.9624720062526));
#49035=CARTESIAN_POINT('Ctrl Pts',(-34.4962109015046,55.1994049989002,16.8513341156845));
#49036=CARTESIAN_POINT('Ctrl Pts',(-34.5002912415971,57.3764068757753,16.7401962251165));
#49037=CARTESIAN_POINT('Ctrl Pts',(-32.6734823234101,58.5605196227415,16.6290583345484));
#49038=CARTESIAN_POINT('Ctrl Pts',(-30.6878830671828,57.6679114137473,16.5179204439804));
#49039=CARTESIAN_POINT('Ctrl Pts',(-30.3609349903662,55.5155966653536,16.4067825534124));
#49040=CARTESIAN_POINT('Ctrl Pts',(-31.9918973755157,54.0736134756683,16.2956446628443));
#49041=CARTESIAN_POINT('Ctrl Pts',(-34.0879318551292,54.6618254114249,16.1845067722763));
#49042=CARTESIAN_POINT('Ctrl Pts',(-34.7305142993751,56.7418354170222,16.0733688817082));
#49043=CARTESIAN_POINT('Ctrl Pts',(-33.331481709642,58.4097867454715,15.9622309911402));
#49044=CARTESIAN_POINT('Ctrl Pts',(-31.1713844814461,58.1389846298839,15.8510931005721));
#49045=CARTESIAN_POINT('Ctrl Pts',(-30.2273841048745,56.1772973179708,15.7399552100041));
#49046=CARTESIAN_POINT('Ctrl Pts',(-31.3635348303942,54.3202794529552,15.6288173194361));
#49047=CARTESIAN_POINT('Ctrl Pts',(-33.539905013914,54.2676805475375,15.517679428868));
#49048=CARTESIAN_POINT('Ctrl Pts',(-34.764438345137,56.0676449746847,15.4065415383));
#49049=CARTESIAN_POINT('Ctrl Pts',(-33.916305578051,58.0726448845937,15.2954036477319));
#49050=CARTESIAN_POINT('Ctrl Pts',(-31.7718122544331,58.447481114776,15.1842657571639));
#49051=CARTESIAN_POINT('Ctrl Pts',(-30.2938374304302,56.8490618262286,15.0731278665959));
#49052=CARTESIAN_POINT('Ctrl Pts',(-30.8351882301687,54.7404382942198,14.9619899760278));
#49053=CARTESIAN_POINT('Ctrl Pts',(-32.90036011462,54.0516576047428,14.8508520854598));
#49054=CARTESIAN_POINT('Ctrl Pts',(-34.5990778627046,55.4131684266542,14.7397141948917));
#49055=CARTESIAN_POINT('Ctrl Pts',(-34.3764858039968,57.5787646792666,14.6285763043237));
#49056=CARTESIAN_POINT('Ctrl Pts',(-32.4363250759318,58.566251122372,14.5174384137557));
#49057=CARTESIAN_POINT('Ctrl Pts',(-30.5544465922265,57.4717710776139,14.4063005231876));
#49058=CARTESIAN_POINT('Ctrl Pts',(-30.453355478433,55.2971128173438,14.2951626326196));
#49059=CARTESIAN_POINT('Ctrl Pts',(-32.2255807620059,54.0327691614409,14.1840247420515));
#49060=CARTESIAN_POINT('Ctrl Pts',(-34.2489861744447,54.8360012884289,14.0728868514835));
#49061=CARTESIAN_POINT('Ctrl Pts',(-34.6715225287502,56.9716155488274,13.9617489609154));
#49062=CARTESIAN_POINT('Ctrl Pts',(-33.1064440441824,58.4848323215015,13.8506110703474));
#49063=CARTESIAN_POINT('Ctrl Pts',(-30.9862717259461,57.9906425072237,13.7394731797794));
#49064=CARTESIAN_POINT('Ctrl Pts',(-30.2516495200118,55.9412728283577,13.6283352892113));
#49065=CARTESIAN_POINT('Ctrl Pts',(-31.5749330715706,54.2127563749733,13.5171973986433));
#49066=CARTESIAN_POINT('Ctrl Pts',(-33.7450107875056,54.386780005505,13.4060595080752));
#49067=CARTESIAN_POINT('Ctrl Pts',(-34.7753761056448,56.3049462630692,13.2949216175072));
#49068=CARTESIAN_POINT('Ctrl Pts',(-33.723343687939,58.2097571189556,13.1837837269391));
#49069=CARTESIAN_POINT('Ctrl Pts',(-31.5510134146689,58.3612890695025,13.0726458363711));
#49070=CARTESIAN_POINT('Ctrl Pts',(-30.248393668858,56.613551975949,12.9615079458031));
#49071=CARTESIAN_POINT('Ctrl Pts',(-30.7529917906697,55.2601287803101,12.8874160187577));
#49072=CARTESIAN_POINT('Ctrl Pts',(-31.2357844803776,54.8397470430914,12.850370055235));
#49073=CARTESIAN_POINT('Ctrl Pts',(-30.7659838258732,56.7578136799223,22.149629944765));
#49074=CARTESIAN_POINT('Ctrl Pts',(-30.6109737261224,56.1812120480563,22.1125839812423));
#49075=CARTESIAN_POINT('Ctrl Pts',(-30.92452680073,54.8710050695066,22.0384920541969));
#49076=CARTESIAN_POINT('Ctrl Pts',(-32.8421872680382,54.1958215473324,21.9273541636289));
#49077=CARTESIAN_POINT('Ctrl Pts',(-34.4449328928026,55.4433407953881,21.8162162730609));
#49078=CARTESIAN_POINT('Ctrl Pts',(-34.2682687706575,57.4651918320407,21.7050783824928));
#49079=CARTESIAN_POINT('Ctrl Pts',(-32.4726875751359,58.4139517679751,21.5939404919248));
#49080=CARTESIAN_POINT('Ctrl Pts',(-30.7023056549664,57.4196146227593,21.4828026013567));
#49081=CARTESIAN_POINT('Ctrl Pts',(-30.5772738897496,55.3931052880117,21.3716647107887));
#49082=CARTESIAN_POINT('Ctrl Pts',(-32.2121850378521,54.1889126052481,21.2605268202207));
#49083=CARTESIAN_POINT('Ctrl Pts',(-34.1105115513431,54.9094467309533,21.1493889296526));
#49084=CARTESIAN_POINT('Ctrl Pts',(-34.5347310361582,56.8950952039422,21.0382510390846));
#49085=CARTESIAN_POINT('Ctrl Pts',(-33.0965319028176,58.3284211283196,20.9271131485165));
#49086=CARTESIAN_POINT('Ctrl Pts',(-31.1123234643604,57.8974602113791,20.8159752579485));
#49087=CARTESIAN_POINT('Ctrl Pts',(-30.3982695419667,55.9966882693789,20.7048373673804));
#49088=CARTESIAN_POINT('Ctrl Pts',(-31.6079541197193,54.3658972202714,20.5936994768124));
#49089=CARTESIAN_POINT('Ctrl Pts',(-33.6341380200995,54.4977717021263,20.4825615862443));
#49090=CARTESIAN_POINT('Ctrl Pts',(-34.6222327225984,56.2716039589447,20.3714236956763));
#49091=CARTESIAN_POINT('Ctrl Pts',(-33.6678236494516,58.0637859825355,20.2602858051082));
#49092=CARTESIAN_POINT('Ctrl Pts',(-31.6444923943572,58.2339128556783,20.1491479145402));
#49093=CARTESIAN_POINT('Ctrl Pts',(-30.4042169286311,56.6262657150416,20.0380100239722));
#49094=CARTESIAN_POINT('Ctrl Pts',(-31.0822354880141,54.712342123958,19.9268721334041));
#49095=CARTESIAN_POINT('Ctrl Pts',(-33.0579499777205,54.2439780989104,19.8157342428361));
#49096=CARTESIAN_POINT('Ctrl Pts',(-34.5229665282545,55.6498725195525,19.7045963522681));
#49097=CARTESIAN_POINT('Ctrl Pts',(-34.1363388719682,57.6431942907766,19.5934584617));
#49098=CARTESIAN_POINT('Ctrl Pts',(-32.251951689578,58.3994333835622,19.482320571132));
#49099=CARTESIAN_POINT('Ctrl Pts',(-30.5946059383997,57.2263955829523,19.371182680564));
#49100=CARTESIAN_POINT('Ctrl Pts',(-30.6812889806306,55.1977756894976,19.2600447899959));
#49101=CARTESIAN_POINT('Ctrl Pts',(-32.4326588443821,54.1703924985414,19.1489068994279));
#49102=CARTESIAN_POINT('Ctrl Pts',(-34.2456668316182,55.0846214957092,19.0377690088598));
#49103=CARTESIAN_POINT('Ctrl Pts',(-34.4608461706423,57.1036585120183,18.9266311182918));
#49104=CARTESIAN_POINT('Ctrl Pts',(-32.8812407721812,58.3794560689105,18.8154932277237));
#49105=CARTESIAN_POINT('Ctrl Pts',(-30.9526813713723,57.7442621940807,18.7043553371557));
#49106=CARTESIAN_POINT('Ctrl Pts',(-30.440400259136,55.7794770447257,18.5932174465876));
#49107=CARTESIAN_POINT('Ctrl Pts',(-31.8132941471607,54.2834907502409,18.4820795560196));
#49108=CARTESIAN_POINT('Ctrl Pts',(-33.814737690064,54.625596531601,18.3709416654516));
#49109=CARTESIAN_POINT('Ctrl Pts',(-34.6127869151118,56.4926610873864,18.2598037748835));
#49110=CARTESIAN_POINT('Ctrl Pts',(-33.4769783161247,58.1757390557332,18.1486658843155));
#49111=CARTESIAN_POINT('Ctrl Pts',(-31.4469303847008,58.1342900848119,18.0375279937474));
#49112=CARTESIAN_POINT('Ctrl Pts',(-30.3807690147821,56.4062528877698,17.9263901031794));
#49113=CARTESIAN_POINT('Ctrl Pts',(-31.2543637993472,54.5733195083342,17.8152522126114));
#49114=CARTESIAN_POINT('Ctrl Pts',(-33.2681035248452,54.3131946555809,17.7041143220433));
#49115=CARTESIAN_POINT('Ctrl Pts',(-34.5787893831659,55.8639735572515,17.5929764314753));
#49116=CARTESIAN_POINT('Ctrl Pts',(-33.9867357439999,57.8062106976179,17.4818385409072));
#49117=CARTESIAN_POINT('Ctrl Pts',(-32.0338560176206,58.3621543956355,17.3707006503392));
#49118=CARTESIAN_POINT('Ctrl Pts',(-30.5076431647456,57.0229430796784,17.2595627597712));
#49119=CARTESIAN_POINT('Ctrl Pts',(-30.8050571180421,55.0143720549316,17.1484248692031));
#49120=CARTESIAN_POINT('Ctrl Pts',(-32.6538715131544,54.1749091590902,17.0372869786351));
#49121=CARTESIAN_POINT('Ctrl Pts',(-34.3618455672547,55.2729243008751,16.926149088067));
#49122=CARTESIAN_POINT('Ctrl Pts',(-34.3656512588821,57.3033917686711,16.815011197499));
#49123=CARTESIAN_POINT('Ctrl Pts',(-32.6618051953302,58.4078016621386,16.7038733069309));
#49124=CARTESIAN_POINT('Ctrl Pts',(-30.8098570014971,57.5752750809247,16.5927354163629));
#49125=CARTESIAN_POINT('Ctrl Pts',(-30.5049158617185,55.5678330463115,16.4815975257948));
#49126=CARTESIAN_POINT('Ctrl Pts',(-32.0260978595029,54.2229100185152,16.3704596352268));
#49127=CARTESIAN_POINT('Ctrl Pts',(-33.9810478608982,54.7715292973545,16.2593217446587));
#49128=CARTESIAN_POINT('Ctrl Pts',(-34.580377958992,56.7115334351178,16.1481838540907));
#49129=CARTESIAN_POINT('Ctrl Pts',(-33.2755145181222,58.2672146434155,16.0370459635227));
#49130=CARTESIAN_POINT('Ctrl Pts',(-31.2608138438975,58.0146402695706,15.9259080729546));
#49131=CARTESIAN_POINT('Ctrl Pts',(-30.3803543116497,56.1849945025464,15.8147701823866));
#49132=CARTESIAN_POINT('Ctrl Pts',(-31.4400305164273,54.4529728621045,15.7036322918186));
#49133=CARTESIAN_POINT('Ctrl Pts',(-33.4699088102677,54.4039143989828,15.5924944012505));
#49134=CARTESIAN_POINT('Ctrl Pts',(-34.6120185708019,56.0827228792765,15.4813565106825));
#49135=CARTESIAN_POINT('Ctrl Pts',(-33.8209737810694,57.9527658651135,15.3702186201144));
#49136=CARTESIAN_POINT('Ctrl Pts',(-31.8208267096473,58.3023717975755,15.2590807295464));
#49137=CARTESIAN_POINT('Ctrl Pts',(-30.4423346512631,56.811542414391,15.1479428389783));
#49138=CARTESIAN_POINT('Ctrl Pts',(-30.9472470260343,54.8448507321039,15.0368049484103));
#49139=CARTESIAN_POINT('Ctrl Pts',(-32.873411799399,54.2024320014245,14.9256670578423));
#49140=CARTESIAN_POINT('Ctrl Pts',(-34.4577885337935,55.4722992717785,14.8145291672742));
#49141=CARTESIAN_POINT('Ctrl Pts',(-34.2501791887594,57.4921288300438,14.7033912767062));
#49142=CARTESIAN_POINT('Ctrl Pts',(-32.4406110471432,58.4131473734421,14.5922533861381));
#49143=CARTESIAN_POINT('Ctrl Pts',(-30.685402160969,57.3923369880037,14.4811154955701));
#49144=CARTESIAN_POINT('Ctrl Pts',(-30.5911155092112,55.3640553875343,14.3699776050021));
#49145=CARTESIAN_POINT('Ctrl Pts',(-32.2440519729435,54.1848149428223,14.258839714434));
#49146=CARTESIAN_POINT('Ctrl Pts',(-34.1312615834455,54.9339813630547,14.147701823866));
#49147=CARTESIAN_POINT('Ctrl Pts',(-34.5253569356325,56.9258470226862,14.0365639332979));
#49148=CARTESIAN_POINT('Ctrl Pts',(-33.0656241805903,58.3372088874948,13.9254260427299));
#49149=CARTESIAN_POINT('Ctrl Pts',(-31.0881610630665,57.8762830833115,13.8142881521618));
#49150=CARTESIAN_POINT('Ctrl Pts',(-30.4029864170935,55.964856866078,13.7031502615938));
#49151=CARTESIAN_POINT('Ctrl Pts',(-31.6371995019103,54.3526871828874,13.5920123710258));
#49152=CARTESIAN_POINT('Ctrl Pts',(-33.661208875352,54.5149972498541,13.4808744804577));
#49153=CARTESIAN_POINT('Ctrl Pts',(-34.6222201085763,56.3040513729488,13.3697365898897));
#49154=CARTESIAN_POINT('Ctrl Pts',(-33.6410001923652,58.0806490489849,13.2585986993216));
#49155=CARTESIAN_POINT('Ctrl Pts',(-31.6148898816497,58.2219813552109,13.1474608087536));
#49156=CARTESIAN_POINT('Ctrl Pts',(-30.3999497178981,56.5918847767849,13.0363229181856));
#49157=CARTESIAN_POINT('Ctrl Pts',(-30.8705832444619,55.3295607530454,12.9622309911402));
#49158=CARTESIAN_POINT('Ctrl Pts',(-31.320879066691,54.9374749902607,12.9251850276175));
#49159=CARTESIAN_POINT('Ctrl Pts',(-30.8911239915931,56.7241717536789,22.2244449171475));
#49160=CARTESIAN_POINT('Ctrl Pts',(-30.7473006326931,56.1891822041237,22.1873989536248));
#49161=CARTESIAN_POINT('Ctrl Pts',(-31.0382252657072,54.9735300058982,22.1133070265794));
#49162=CARTESIAN_POINT('Ctrl Pts',(-32.8174923591508,54.3470730060695,22.0021691360114));
#49163=CARTESIAN_POINT('Ctrl Pts',(-34.304571327466,55.5045615106007,21.8910312454433));
#49164=CARTESIAN_POINT('Ctrl Pts',(-34.1406566697445,57.3804999672191,21.7798933548753));
#49165=CARTESIAN_POINT('Ctrl Pts',(-32.474658653275,58.2607899676461,21.6687554643073));
#49166=CARTESIAN_POINT('Ctrl Pts',(-30.8320413354105,57.3382119657361,21.5576175737392));
#49167=CARTESIAN_POINT('Ctrl Pts',(-30.7160328400182,55.4579513902372,21.4464796831712));
#49168=CARTESIAN_POINT('Ctrl Pts',(-32.2329560159994,54.3406626672683,21.3353417926031));
#49169=CARTESIAN_POINT('Ctrl Pts',(-33.9942844449089,55.0091974164725,21.2242039020351));
#49170=CARTESIAN_POINT('Ctrl Pts',(-34.3878889346486,56.8515459694957,21.1130660114671));
#49171=CARTESIAN_POINT('Ctrl Pts',(-33.0534814963164,58.1814318877282,21.001928120899));
#49172=CARTESIAN_POINT('Ctrl Pts',(-31.2124690536731,57.7815724803175,20.890790230331));
#49173=CARTESIAN_POINT('Ctrl Pts',(-30.5499468456396,56.0179751041415,20.7796523397629));
#49174=CARTESIAN_POINT('Ctrl Pts',(-31.672331125513,54.504874688596,20.6685144491949));
#49175=CARTESIAN_POINT('Ctrl Pts',(-33.552289752533,54.6272320766892,20.5573765586268));
#49176=CARTESIAN_POINT('Ctrl Pts',(-34.4690758152034,56.2730507279312,20.4462386680588));
#49177=CARTESIAN_POINT('Ctrl Pts',(-33.5835443634768,57.9358948832952,20.3351007774908));
#49178=CARTESIAN_POINT('Ctrl Pts',(-31.7062325125535,58.0937440710183,20.2239628869227));
#49179=CARTESIAN_POINT('Ctrl Pts',(-30.5554650223787,56.602117318542,20.1128249963547));
#49180=CARTESIAN_POINT('Ctrl Pts',(-31.1845524609634,54.8263174191154,20.0016871057866));
#49181=CARTESIAN_POINT('Ctrl Pts',(-33.0176839446135,54.3917542043407,19.8905492152186));
#49182=CARTESIAN_POINT('Ctrl Pts',(-34.3769734456241,55.6961882906393,19.7794113246506));
#49183=CARTESIAN_POINT('Ctrl Pts',(-34.018247864129,57.5456563766984,19.6682734340825));
#49184=CARTESIAN_POINT('Ctrl Pts',(-32.2698527951939,58.2473193433743,19.5571355435145));
#49185=CARTESIAN_POINT('Ctrl Pts',(-30.7321140725153,57.1589371226573,19.4459976529464));
#49186=CARTESIAN_POINT('Ctrl Pts',(-30.812541388628,55.2767183028703,19.3348597623784));
#49187=CARTESIAN_POINT('Ctrl Pts',(-32.4375187087245,54.3234791162739,19.2237218718103));
#49188=CARTESIAN_POINT('Ctrl Pts',(-34.1196858633551,55.1717302004793,19.1125839812423));
#49189=CARTESIAN_POINT('Ctrl Pts',(-34.3193361787479,57.0450577184658,19.0014460906742));
#49190=CARTESIAN_POINT('Ctrl Pts',(-32.8537274570681,58.2287837479543,18.8903082001062));
#49191=CARTESIAN_POINT('Ctrl Pts',(-31.0643479823862,57.6394304298312,18.7791703095382));
#49192=CARTESIAN_POINT('Ctrl Pts',(-30.5890370808302,55.8164395398742,18.6680324189701));
#49193=CARTESIAN_POINT('Ctrl Pts',(-31.8628522109823,54.4284153137944,18.5568945284021));
#49194=CARTESIAN_POINT('Ctrl Pts',(-33.7198559381705,54.7458320669828,18.445756637834));
#49195=CARTESIAN_POINT('Ctrl Pts',(-34.4603116910435,56.4781546454978,18.334618747266));
#49196=CARTESIAN_POINT('Ctrl Pts',(-33.406471921658,58.039768547349,18.223480856698));
#49197=CARTESIAN_POINT('Ctrl Pts',(-31.522928122288,58.0013108582667,18.1123429661299));
#49198=CARTESIAN_POINT('Ctrl Pts',(-30.5337092933366,56.3979823372073,18.0012050755619));
#49199=CARTESIAN_POINT('Ctrl Pts',(-31.3442586474474,54.6973277624788,17.8900671849938));
#49200=CARTESIAN_POINT('Ctrl Pts',(-33.212671168548,54.4559755530648,17.7789292944258));
#49201=CARTESIAN_POINT('Ctrl Pts',(-34.4287676868359,55.8948381233621,17.6677914038578));
#49202=CARTESIAN_POINT('Ctrl Pts',(-33.8794412676495,57.6969082449663,17.5566535132897));
#49203=CARTESIAN_POINT('Ctrl Pts',(-32.0674966122556,58.2127306987079,17.4455156227217));
#49204=CARTESIAN_POINT('Ctrl Pts',(-30.6514272125861,56.9701673428525,17.3343777321536));
#49205=CARTESIAN_POINT('Ctrl Pts',(-30.9273774494778,55.1065505086418,17.2232398415856));
#49206=CARTESIAN_POINT('Ctrl Pts',(-32.6427669416152,54.3276698192808,17.1121019510175));
#49207=CARTESIAN_POINT('Ctrl Pts',(-34.2274802330049,55.3464436028498,17.0009640604495));
#49208=CARTESIAN_POINT('Ctrl Pts',(-34.231011276167,57.2303766615671,16.8898261698814));
#49209=CARTESIAN_POINT('Ctrl Pts',(-32.6501280672502,58.2550837015355,16.7786882793134));
#49210=CARTESIAN_POINT('Ctrl Pts',(-30.9318309358115,57.4826387481023,16.6675503887454));
#49211=CARTESIAN_POINT('Ctrl Pts',(-30.6488967330708,55.6200694272693,16.5564124981774));
#49212=CARTESIAN_POINT('Ctrl Pts',(-32.0602983434901,54.372206561362,16.4452746076093));
#49213=CARTESIAN_POINT('Ctrl Pts',(-33.8741638666671,54.8812331832842,16.3341367170413));
#49214=CARTESIAN_POINT('Ctrl Pts',(-34.4302416186091,56.6812314532133,16.2229988264732));
#49215=CARTESIAN_POINT('Ctrl Pts',(-33.2195473266022,58.1246425413596,16.1118609359052));
#49216=CARTESIAN_POINT('Ctrl Pts',(-31.3502432063489,57.8902959092574,16.0007230453371));
#49217=CARTESIAN_POINT('Ctrl Pts',(-30.5333245184248,56.1926916871221,15.8895851547691));
#49218=CARTESIAN_POINT('Ctrl Pts',(-31.5165262024604,54.5856662712538,15.778447264201));
#49219=CARTESIAN_POINT('Ctrl Pts',(-33.3999126066214,54.5401482504283,15.667309373633));
#49220=CARTESIAN_POINT('Ctrl Pts',(-34.4595987964669,56.0978007838681,15.556171483065));
#49221=CARTESIAN_POINT('Ctrl Pts',(-33.7256419840878,57.8328868456334,15.4450335924969));
#49222=CARTESIAN_POINT('Ctrl Pts',(-31.8698411648614,58.1572624803751,15.3338957019289));
#49223=CARTESIAN_POINT('Ctrl Pts',(-30.590831872096,56.7740230025534,15.2227578113608));
#49224=CARTESIAN_POINT('Ctrl Pts',(-31.0593058218999,54.9492631699881,15.1116199207928));
#49225=CARTESIAN_POINT('Ctrl Pts',(-32.8464634841781,54.353206398106,15.0004820302248));
#49226=CARTESIAN_POINT('Ctrl Pts',(-34.3164992048823,55.531430116903,14.8893441396567));
#49227=CARTESIAN_POINT('Ctrl Pts',(-34.123872573522,57.4054929808209,14.7782062490887));
#49228=CARTESIAN_POINT('Ctrl Pts',(-32.4448970183546,58.2600436245124,14.6670683585206));
#49229=CARTESIAN_POINT('Ctrl Pts',(-30.8163577297114,57.3129028983934,14.5559304679526));
#49230=CARTESIAN_POINT('Ctrl Pts',(-30.7288755399893,55.4309979577248,14.4447925773845));
#49231=CARTESIAN_POINT('Ctrl Pts',(-32.2625231838812,54.3368607242037,14.3336546868165));
#49232=CARTESIAN_POINT('Ctrl Pts',(-34.0135369924464,55.0319614376805,14.2225167962484));
#49233=CARTESIAN_POINT('Ctrl Pts',(-34.3791913425147,56.880078496545,14.1113789056804));
#49234=CARTESIAN_POINT('Ctrl Pts',(-33.0248043169983,58.1895854534881,14.0002410151124));
#49235=CARTESIAN_POINT('Ctrl Pts',(-31.1900504001867,57.7619236593993,13.8891031245443));
#49236=CARTESIAN_POINT('Ctrl Pts',(-30.5543233141752,55.9884409037984,13.7779652339763));
#49237=CARTESIAN_POINT('Ctrl Pts',(-31.69946593225,54.4926179908013,13.6668273434083));
#49238=CARTESIAN_POINT('Ctrl Pts',(-33.5774069631985,54.6432144942031,13.5556894528402));
#49239=CARTESIAN_POINT('Ctrl Pts',(-34.4690641115077,56.3031564828284,13.4445515622722));
#49240=CARTESIAN_POINT('Ctrl Pts',(-33.5586566967914,57.9515409790141,13.3334136717041));
#49241=CARTESIAN_POINT('Ctrl Pts',(-31.6787663486305,58.0826736409194,13.2222757811361));
#49242=CARTESIAN_POINT('Ctrl Pts',(-30.5515057669383,56.5702175776209,13.111137890568));
#49243=CARTESIAN_POINT('Ctrl Pts',(-30.9881746982542,55.3989927257806,13.0370459635227));
#49244=CARTESIAN_POINT('Ctrl Pts',(-31.4059736530045,55.03520293743,13.));
#49245=CARTESIAN_POINT('Ctrl Pts',(-31.6688940285233,54.8502492137286,21.3785196366098));
#49246=CARTESIAN_POINT('Ctrl Pts',(-31.8552973625104,54.7413392620857,21.3641270219409));
#49247=CARTESIAN_POINT('Ctrl Pts',(-32.0614196306261,54.6673572529872,21.349734407272));
#49248=CARTESIAN_POINT('Ctrl Pts',(-32.2736902248208,54.6382999126305,21.3353417926031));
#49249=CARTESIAN_POINT('Ctrl Pts',(-32.8200654923026,54.5635075836697,21.2982958290804));
#49250=CARTESIAN_POINT('Ctrl Pts',(-33.4071749686058,54.7863525000711,21.2612498655578));
#49251=CARTESIAN_POINT('Ctrl Pts',(-33.7663304550473,55.2048330504423,21.2242039020351));
#49252=CARTESIAN_POINT('Ctrl Pts',(-34.1254859414888,55.6233136008135,21.1871579385124));
#49253=CARTESIAN_POINT('Ctrl Pts',(-34.2566874380687,56.2374297851546,21.1501119749897));
#49254=CARTESIAN_POINT('Ctrl Pts',(-34.0998869466366,56.7661355303639,21.113066011467));
#49255=CARTESIAN_POINT('Ctrl Pts',(-33.9430864552046,57.2948412755732,21.0760200479444));
#49256=CARTESIAN_POINT('Ctrl Pts',(-33.4982839757605,57.7381365816507,21.0389740844217));
#49257=CARTESIAN_POINT('Ctrl Pts',(-32.9690473289312,57.893141000121,21.001928120899));
#49258=CARTESIAN_POINT('Ctrl Pts',(-32.4398106821019,58.0481454185913,20.9648821573763));
#49259=CARTESIAN_POINT('Ctrl Pts',(-31.8261398678875,57.9148589494544,20.9278361938536));
#49260=CARTESIAN_POINT('Ctrl Pts',(-31.4088840927747,57.5542828188566,20.890790230331));
#49261=CARTESIAN_POINT('Ctrl Pts',(-30.9916283176619,57.1937066882589,20.8537442668083));
#49262=CARTESIAN_POINT('Ctrl Pts',(-30.7707875816508,56.6058408962002,20.8166983032856));
#49263=CARTESIAN_POINT('Ctrl Pts',(-30.8474312602907,56.0597245975799,20.7796523397629));
#49264=CARTESIAN_POINT('Ctrl Pts',(-30.9171750925773,55.5627724129274,20.7459414387119));
#49265=CARTESIAN_POINT('Ctrl Pts',(-31.2332522390469,55.1003910850246,20.7122305376608));
#49266=CARTESIAN_POINT('Ctrl Pts',(-31.666645377609,54.8465106721999,20.6785196366098));
#49267=CARTESIAN_POINT('Ctrl Pts',(-30.5157034944334,56.8250975324092,22.));
#49268=CARTESIAN_POINT('Ctrl Pts',(-30.5033891751538,56.7529213757994,22.));
#49269=CARTESIAN_POINT('Ctrl Pts',(-30.4952952696159,56.6802754208432,22.));
#49270=CARTESIAN_POINT('Ctrl Pts',(-30.4912615438001,56.607470311302,22.));
#49271=CARTESIAN_POINT('Ctrl Pts',(-30.4871154839524,56.5326376738947,22.));
#49272=CARTESIAN_POINT('Ctrl Pts',(-30.487259104724,56.4576358814836,22.));
#49273=CARTESIAN_POINT('Ctrl Pts',(-30.4915726828735,56.3828069694704,22.));
#49274=CARTESIAN_POINT('Ctrl Pts',(-30.4952175802641,56.3195778597398,22.));
#49275=CARTESIAN_POINT('Ctrl Pts',(-30.5018408843279,56.2564719495607,22.));
#49276=CARTESIAN_POINT('Ctrl Pts',(-30.5113973391135,56.1937062820743,22.));
#49277=CARTESIAN_POINT('Ctrl Pts',(-30.5156431766697,56.1658201219624,22.));
#49278=CARTESIAN_POINT('Ctrl Pts',(-30.5204683060506,56.1380012967317,22.));
#49279=CARTESIAN_POINT('Ctrl Pts',(-30.5258701615125,56.1102698241508,22.));
#49280=CARTESIAN_POINT('Ctrl Pts',(-30.5288380312313,56.0950336893984,22.));
#49281=CARTESIAN_POINT('Ctrl Pts',(-30.5319800053069,56.079823934807,22.));
#49282=CARTESIAN_POINT('Ctrl Pts',(-30.5352957613589,56.0646439756259,22.));
#49283=CARTESIAN_POINT('Ctrl Pts',(-30.5383537435174,56.050644138601,22.));
#49284=CARTESIAN_POINT('Ctrl Pts',(-30.5415601340454,56.0366676410989,22.));
#49285=CARTESIAN_POINT('Ctrl Pts',(-30.5449092364481,56.0227386583762,22.));
#49286=CARTESIAN_POINT('Ctrl Pts',(-30.562023288202,55.9515609807379,22.));
#49287=CARTESIAN_POINT('Ctrl Pts',(-30.582885617709,55.8814985818673,22.));
#49288=CARTESIAN_POINT('Ctrl Pts',(-30.6073807784317,55.8128705897534,22.));
#49289=CARTESIAN_POINT('Ctrl Pts',(-30.6316859828533,55.744774797435,22.));
#49290=CARTESIAN_POINT('Ctrl Pts',(-30.6595684038256,55.6780903688681,22.));
#49291=CARTESIAN_POINT('Ctrl Pts',(-30.6909586479405,55.6131557366303,22.));
#49292=CARTESIAN_POINT('Ctrl Pts',(-30.717046572308,55.5591896136386,22.));
#49293=CARTESIAN_POINT('Ctrl Pts',(-30.7455582375738,55.5064323069469,22.));
#49294=CARTESIAN_POINT('Ctrl Pts',(-30.7764732244705,55.4550987628743,22.));
#49295=CARTESIAN_POINT('Ctrl Pts',(-30.7893770627354,55.4336722698765,22.));
#49296=CARTESIAN_POINT('Ctrl Pts',(-30.8026998040084,55.4124940848702,22.));
#49297=CARTESIAN_POINT('Ctrl Pts',(-30.8164407555073,55.3915810450032,22.));
#49298=CARTESIAN_POINT('Ctrl Pts',(-30.8228008343902,55.3819013235337,22.));
#49299=CARTESIAN_POINT('Ctrl Pts',(-30.8292505148999,55.3722784163222,22.));
#49300=CARTESIAN_POINT('Ctrl Pts',(-30.8357897592665,55.3627140504885,22.));
#49301=CARTESIAN_POINT('Ctrl Pts',(-30.842610586495,55.3527378386747,22.));
#49302=CARTESIAN_POINT('Ctrl Pts',(-30.8495241989623,55.342832182411,22.));
#49303=CARTESIAN_POINT('Ctrl Pts',(-30.8565275508905,55.3330023510939,22.));
#49304=CARTESIAN_POINT('Ctrl Pts',(-30.8964137687943,55.2770184739607,22.));
#49305=CARTESIAN_POINT('Ctrl Pts',(-30.9392347488862,55.223452024519,22.));
#49306=CARTESIAN_POINT('Ctrl Pts',(-30.9849250921345,55.1725987747036,22.));
#49307=CARTESIAN_POINT('Ctrl Pts',(-31.0263368675617,55.1265075613009,22.));
#49308=CARTESIAN_POINT('Ctrl Pts',(-31.070106455774,55.0826451744756,22.));
#49309=CARTESIAN_POINT('Ctrl Pts',(-31.1162077188352,55.0412612463575,22.));
#49310=CARTESIAN_POINT('Ctrl Pts',(-31.1707480896715,54.9923017464142,22.));
#49311=CARTESIAN_POINT('Ctrl Pts',(-31.2285529377195,54.9468098709297,22.));
#49312=CARTESIAN_POINT('Ctrl Pts',(-31.2892182914168,54.9049320829473,22.));
#49313=CARTESIAN_POINT('Ctrl Pts',(-31.3025747483259,54.8957120119093,22.));
#49314=CARTESIAN_POINT('Ctrl Pts',(-31.316069903986,54.8866673619299,22.));
#49315=CARTESIAN_POINT('Ctrl Pts',(-31.3296994894175,54.8778000986119,22.));
#49316=CARTESIAN_POINT('Ctrl Pts',(-31.3437625465174,54.8686508232369,22.));
#49317=CARTESIAN_POINT('Ctrl Pts',(-31.35797403863,54.8596873154124,22.));
#49318=CARTESIAN_POINT('Ctrl Pts',(-31.3723000273365,54.8509292655043,22.));
#49319=CARTESIAN_POINT('Ctrl Pts',(-31.4308133755576,54.8151577153162,22.));
#49320=CARTESIAN_POINT('Ctrl Pts',(-31.4913062998034,54.7827600287089,22.));
#49321=CARTESIAN_POINT('Ctrl Pts',(-31.5534255550724,54.7538008858545,22.));
#49322=CARTESIAN_POINT('Ctrl Pts',(-31.6155323755621,54.7248475399232,22.));
#49323=CARTESIAN_POINT('Ctrl Pts',(-31.6792660307875,54.6993312183976,22.));
#49324=CARTESIAN_POINT('Ctrl Pts',(-31.7442852730188,54.6773670392608,22.));
#49325=CARTESIAN_POINT('Ctrl Pts',(-31.791347955944,54.6614687734097,22.));
#49326=CARTESIAN_POINT('Ctrl Pts',(-31.8390844862475,54.6474326075963,22.));
#49327=CARTESIAN_POINT('Ctrl Pts',(-31.8873641955329,54.6353193456783,22.));
#49328=CARTESIAN_POINT('Ctrl Pts',(-31.9235796702862,54.6262329709327,22.));
#49329=CARTESIAN_POINT('Ctrl Pts',(-31.9601007697018,54.6182288634993,22.));
#49330=CARTESIAN_POINT('Ctrl Pts',(-31.9968706813336,54.6113381701107,22.));
#49331=CARTESIAN_POINT('Ctrl Pts',(-32.0090868552777,54.6090488551438,22.));
#49332=CARTESIAN_POINT('Ctrl Pts',(-32.0213209008061,54.6068842729294,22.));
#49333=CARTESIAN_POINT('Ctrl Pts',(-32.03357036514,54.6048451279784,22.));
#49334=CARTESIAN_POINT('Ctrl Pts',(-32.0985567096936,54.5940269752194,22.));
#49335=CARTESIAN_POINT('Ctrl Pts',(-32.1639811762486,54.5867347457029,22.));
#49336=CARTESIAN_POINT('Ctrl Pts',(-32.2295294708426,54.583092151071,22.));
#49337=CARTESIAN_POINT('Ctrl Pts',(-32.2756530618083,54.5805290097125,22.));
#49338=CARTESIAN_POINT('Ctrl Pts',(-32.3218379339147,54.5797739344473,22.));
#49339=CARTESIAN_POINT('Ctrl Pts',(-32.3679699516131,54.5808847307995,22.));
#49340=CARTESIAN_POINT('Ctrl Pts',(-32.3827771688533,54.5812412684867,22.));
#49341=CARTESIAN_POINT('Ctrl Pts',(-32.3975809348718,54.5817902377288,22.));
#49342=CARTESIAN_POINT('Ctrl Pts',(-32.4123708490685,54.5825334834863,22.));
#49343=CARTESIAN_POINT('Ctrl Pts',(-32.4753792589169,54.5856998800376,22.));
#49344=CARTESIAN_POINT('Ctrl Pts',(-32.5380109271213,54.5923812630455,22.));
#49345=CARTESIAN_POINT('Ctrl Pts',(-32.599975776176,54.6027055704928,22.));
#49346=CARTESIAN_POINT('Ctrl Pts',(-32.6570986727596,54.6122231333627,22.));
#49347=CARTESIAN_POINT('Ctrl Pts',(-32.7136552659116,54.6248370045788,22.));
#49348=CARTESIAN_POINT('Ctrl Pts',(-32.7694005056339,54.6406824777883,22.));
#49349=CARTESIAN_POINT('Ctrl Pts',(-32.7798334333406,54.6436480166809,22.));
#49350=CARTESIAN_POINT('Ctrl Pts',(-32.7902378797118,54.6467268441195,22.));
#49351=CARTESIAN_POINT('Ctrl Pts',(-32.8006124898339,54.6499179279034,22.));
#49352=CARTESIAN_POINT('Origin',(-32.5,56.2916512459885,17.));
#49353=CARTESIAN_POINT('Origin',(32.5,56.2916512459885,13.));
#49354=CARTESIAN_POINT('Ctrl Pts',(31.9588970197441,54.7159724828016,13.));
#49355=CARTESIAN_POINT('Ctrl Pts',(32.0152863485799,54.6890038458289,13.));
#49356=CARTESIAN_POINT('Ctrl Pts',(32.0731449906843,54.6655486354191,13.));
#49357=CARTESIAN_POINT('Ctrl Pts',(32.1321548891936,54.6454940895918,13.));
#49358=CARTESIAN_POINT('Ctrl Pts',(32.1695849277563,54.6327734708036,13.));
#49359=CARTESIAN_POINT('Ctrl Pts',(32.2074789471058,54.6214218413018,13.));
#49360=CARTESIAN_POINT('Ctrl Pts',(32.2457622247192,54.6114186950782,13.));
#49361=CARTESIAN_POINT('Ctrl Pts',(32.2719048889137,54.6045878041797,13.));
#49362=CARTESIAN_POINT('Ctrl Pts',(32.2982291704566,54.5983858679889,13.));
#49363=CARTESIAN_POINT('Ctrl Pts',(32.3247122732464,54.5928081200755,13.));
#49364=CARTESIAN_POINT('Ctrl Pts',(32.3387744982338,54.5898463996645,13.));
#49365=CARTESIAN_POINT('Ctrl Pts',(32.3528813591965,54.5870608477191,13.));
#49366=CARTESIAN_POINT('Ctrl Pts',(32.3670153450051,54.5844531528782,13.));
#49367=CARTESIAN_POINT('Ctrl Pts',(32.4318895160093,54.5724839855584,13.));
#49368=CARTESIAN_POINT('Ctrl Pts',(32.4974065808839,54.564242006131,13.));
#49369=CARTESIAN_POINT('Ctrl Pts',(32.5632274830034,54.5596289937387,13.));
#49370=CARTESIAN_POINT('Ctrl Pts',(32.6107070715096,54.5563014196231,13.));
#49371=CARTESIAN_POINT('Ctrl Pts',(32.6583455247626,54.5548630893557,13.));
#49372=CARTESIAN_POINT('Ctrl Pts',(32.7060224975765,54.5552923689741,13.));
#49373=CARTESIAN_POINT('Ctrl Pts',(32.7190852578705,54.5554099850144,13.));
#49374=CARTESIAN_POINT('Ctrl Pts',(32.7321509321603,54.555667872943,13.));
#49375=CARTESIAN_POINT('Ctrl Pts',(32.7452170875462,54.5560657581446,13.));
#49376=CARTESIAN_POINT('Ctrl Pts',(32.7585822784109,54.5564727494519,13.));
#49377=CARTESIAN_POINT('Ctrl Pts',(32.7719398790819,54.5570260108108,13.));
#49378=CARTESIAN_POINT('Ctrl Pts',(32.7852820453889,54.5577244070497,13.));
#49379=CARTESIAN_POINT('Ctrl Pts',(32.853041605873,54.561271284004,13.));
#49380=CARTESIAN_POINT('Ctrl Pts',(32.9204432863695,54.5685589035957,13.));
#49381=CARTESIAN_POINT('Ctrl Pts',(32.9871435056369,54.5794869269798,13.));
#49382=CARTESIAN_POINT('Ctrl Pts',(33.0548103384148,54.5905733182847,13.));
#49383=CARTESIAN_POINT('Ctrl Pts',(33.1217562800348,54.6054062113063,13.));
#49384=CARTESIAN_POINT('Ctrl Pts',(33.1876366469328,54.6239318015843,13.));
#49385=CARTESIAN_POINT('Ctrl Pts',(33.2284548198869,54.6354098910918,13.));
#49386=CARTESIAN_POINT('Ctrl Pts',(33.2688641590369,54.6483065465144,13.));
#49387=CARTESIAN_POINT('Ctrl Pts',(33.3087825622703,54.662619012904,13.));
#49388=CARTESIAN_POINT('Ctrl Pts',(33.3414809094137,54.6743427783,13.));
#49389=CARTESIAN_POINT('Ctrl Pts',(33.3738498710885,54.6870166551149,13.));
#49390=CARTESIAN_POINT('Ctrl Pts',(33.4058433876126,54.7006430223894,13.));
#49391=CARTESIAN_POINT('Ctrl Pts',(33.4189228879679,54.7062137159227,13.));
#49392=CARTESIAN_POINT('Ctrl Pts',(33.4319419054982,54.7119448243245,13.));
#49393=CARTESIAN_POINT('Ctrl Pts',(33.4448753978619,54.7178263149849,13.));
#49394=CARTESIAN_POINT('Ctrl Pts',(33.5090388472157,54.7470045692029,13.));
#49395=CARTESIAN_POINT('Ctrl Pts',(33.5712122520923,54.7799269958923,13.));
#49396=CARTESIAN_POINT('Ctrl Pts',(33.6310396925136,54.816520963373,13.));
#49397=CARTESIAN_POINT('Ctrl Pts',(33.6376901818306,54.8205887922503,13.));
#49398=CARTESIAN_POINT('Ctrl Pts',(33.6443116826016,54.8247020426775,13.));
#49399=CARTESIAN_POINT('Ctrl Pts',(33.6509037041525,54.8288606547027,13.));
#49400=CARTESIAN_POINT('Ctrl Pts',(33.7079313851622,54.8648368720406,13.));
#49401=CARTESIAN_POINT('Ctrl Pts',(33.7627542963076,54.9042038022191,13.));
#49402=CARTESIAN_POINT('Ctrl Pts',(33.815278351599,54.9466335926782,13.));
#49403=CARTESIAN_POINT('Ctrl Pts',(33.8717836154444,54.9922794684867,13.));
#49404=CARTESIAN_POINT('Ctrl Pts',(33.9256293125948,55.0414702768426,13.));
#49405=CARTESIAN_POINT('Ctrl Pts',(33.9766695218208,55.0938552564678,13.));
#49406=CARTESIAN_POINT('Ctrl Pts',(33.9860164683474,55.1034484695595,13.));
#49407=CARTESIAN_POINT('Ctrl Pts',(33.9952692319585,55.1131489427183,13.));
#49408=CARTESIAN_POINT('Ctrl Pts',(34.0044267784923,55.122954700519,13.));
#49409=CARTESIAN_POINT('Ctrl Pts',(34.0122933717197,55.1313781256821,13.));
#49410=CARTESIAN_POINT('Ctrl Pts',(34.0200833037881,55.1398724075814,13.));
#49411=CARTESIAN_POINT('Ctrl Pts',(34.0277952352549,55.1484347978079,13.));
#49412=CARTESIAN_POINT('Ctrl Pts',(34.0753570092449,55.2012416037971,13.));
#49413=CARTESIAN_POINT('Ctrl Pts',(34.1199659342344,55.2566479177833,13.));
#49414=CARTESIAN_POINT('Ctrl Pts',(34.1615258635099,55.3142853318928,13.));
#49415=CARTESIAN_POINT('Ctrl Pts',(34.203961681234,55.3731374724492,13.));
#49416=CARTESIAN_POINT('Ctrl Pts',(34.2432193073913,55.4343163955046,13.));
#49417=CARTESIAN_POINT('Ctrl Pts',(34.279168752062,55.4974776038552,13.));
#49418=CARTESIAN_POINT('Ctrl Pts',(34.3153358231695,55.5610211699543,13.));
#49419=CARTESIAN_POINT('Ctrl Pts',(34.3481552082549,55.6265719324186,13.));
#49420=CARTESIAN_POINT('Ctrl Pts',(34.3774567489378,55.6938154068255,13.));
#49421=CARTESIAN_POINT('Ctrl Pts',(34.3846992417049,55.7104360474361,13.));
#49422=CARTESIAN_POINT('Ctrl Pts',(34.3917266096341,55.7271602398749,13.));
#49423=CARTESIAN_POINT('Ctrl Pts',(34.3985358555223,55.7439834808493,13.));
#49424=CARTESIAN_POINT('Ctrl Pts',(34.4038603586493,55.7571384470005,13.));
#49425=CARTESIAN_POINT('Ctrl Pts',(34.4090519562624,55.7703555309735,13.));
#49426=CARTESIAN_POINT('Ctrl Pts',(34.4141017841657,55.78361234165,13.));
#49427=CARTESIAN_POINT('Ctrl Pts',(34.4409205170208,55.8540168922319,13.));
#49428=CARTESIAN_POINT('Ctrl Pts',(34.4637958508171,55.9256644804537,13.));
#49429=CARTESIAN_POINT('Ctrl Pts',(34.4826007269245,55.9981857629538,13.));
#49430=CARTESIAN_POINT('Ctrl Pts',(34.5014259920285,56.0707856759206,13.));
#49431=CARTESIAN_POINT('Ctrl Pts',(34.5161726006451,56.1442621127221,13.));
#49432=CARTESIAN_POINT('Ctrl Pts',(34.5266721187438,56.2182764863688,13.));
#49433=CARTESIAN_POINT('Ctrl Pts',(34.5369326971032,56.2906064993641,13.));
#49434=CARTESIAN_POINT('Ctrl Pts',(34.5431377093135,56.3634511943331,13.));
#49435=CARTESIAN_POINT('Ctrl Pts',(34.5450833843614,56.4365110275565,13.));
#49436=CARTESIAN_POINT('Ctrl Pts',(34.5455017158085,56.4522193164544,13.));
#49437=CARTESIAN_POINT('Ctrl Pts',(34.5457229607325,56.4679375826975,13.));
#49438=CARTESIAN_POINT('Ctrl Pts',(34.5457447745363,56.4836628867631,13.));
#49439=CARTESIAN_POINT('Ctrl Pts',(34.545763248735,56.4969807103663,13.));
#49440=CARTESIAN_POINT('Ctrl Pts',(34.5456386792457,56.5103035820178,13.));
#49441=CARTESIAN_POINT('Ctrl Pts',(34.5453721234943,56.52362996598,13.));
#49442=CARTESIAN_POINT('Ctrl Pts',(34.1542537360139,57.5104384051693,13.));
#49443=CARTESIAN_POINT('Ctrl Pts',(34.1045519887874,57.5661317580794,13.));
#49444=CARTESIAN_POINT('Ctrl Pts',(34.0516736631994,57.6187667032821,13.));
#49445=CARTESIAN_POINT('Ctrl Pts',(33.9959663128832,57.6682442041037,13.));
#49446=CARTESIAN_POINT('Ctrl Pts',(33.9417168531154,57.7164268528026,13.));
#49447=CARTESIAN_POINT('Ctrl Pts',(33.8847834892842,57.7616152150798,13.));
#49448=CARTESIAN_POINT('Ctrl Pts',(33.8254670336605,57.8036766866523,13.));
#49449=CARTESIAN_POINT('Ctrl Pts',(33.8122280670726,57.8130644764474,13.));
#49450=CARTESIAN_POINT('Ctrl Pts',(33.7988685443533,57.8222975377499,13.));
#49451=CARTESIAN_POINT('Ctrl Pts',(33.7853974830175,57.8313702492573,13.));
#49452=CARTESIAN_POINT('Ctrl Pts',(33.7235792094515,57.8730046348467,13.));
#49453=CARTESIAN_POINT('Ctrl Pts',(33.6595370839855,57.9111844300756,13.));
#49454=CARTESIAN_POINT('Ctrl Pts',(33.5936094996551,57.9457862388347,13.));
#49455=CARTESIAN_POINT('Ctrl Pts',(33.5473238504462,57.9700790625212,13.));
#49456=CARTESIAN_POINT('Ctrl Pts',(33.5001083178125,57.9926073121088,13.));
#49457=CARTESIAN_POINT('Ctrl Pts',(33.4520768825943,58.0133132482739,13.));
#49458=CARTESIAN_POINT('Ctrl Pts',(33.4338169281544,58.0211849566518,13.));
#49459=CARTESIAN_POINT('Ctrl Pts',(33.4154390450392,58.0287931599074,13.));
#49460=CARTESIAN_POINT('Ctrl Pts',(33.396949493977,58.036134191934,13.));
#49461=CARTESIAN_POINT('Ctrl Pts',(33.3793383499135,58.0431264640644,13.));
#49462=CARTESIAN_POINT('Ctrl Pts',(33.3616202465401,58.0498782555098,13.));
#49463=CARTESIAN_POINT('Ctrl Pts',(33.3438321782917,58.0563750966341,13.));
#49464=CARTESIAN_POINT('Ctrl Pts',(33.2756398801499,58.0812813720512,13.));
#49465=CARTESIAN_POINT('Ctrl Pts',(33.2063496366854,58.1024753903028,13.));
#49466=CARTESIAN_POINT('Ctrl Pts',(33.1362740500475,58.1198408416597,13.));
#49467=CARTESIAN_POINT('Ctrl Pts',(33.0677030438195,58.1368334425108,13.));
#49468=CARTESIAN_POINT('Ctrl Pts',(32.9983791190584,58.150160130782,13.));
#49469=CARTESIAN_POINT('Ctrl Pts',(32.9285938583003,58.1596629269119,13.));
#49470=CARTESIAN_POINT('Ctrl Pts',(32.860339265009,58.1689572890441,13.));
#49471=CARTESIAN_POINT('Ctrl Pts',(32.791642581611,58.1745936618249,13.));
#49472=CARTESIAN_POINT('Ctrl Pts',(32.7227877556981,58.1763767799635,13.));
#49473=CARTESIAN_POINT('Ctrl Pts',(32.7004157900083,58.1769561417917,13.));
#49474=CARTESIAN_POINT('Ctrl Pts',(32.6780272661526,58.1771283364136,13.));
#49475=CARTESIAN_POINT('Ctrl Pts',(32.6556323879924,58.1768855536512,13.));
#49476=CARTESIAN_POINT('Ctrl Pts',(32.6429970562573,58.176748574083,13.));
#49477=CARTESIAN_POINT('Ctrl Pts',(32.6303583960511,58.1764793454784,13.));
#49478=CARTESIAN_POINT('Ctrl Pts',(32.6177361302722,58.1760772493224,13.));
#49479=CARTESIAN_POINT('Ctrl Pts',(32.5494663659828,58.1739024409108,13.));
#49480=CARTESIAN_POINT('Ctrl Pts',(32.4815560589164,58.1678447148808,13.));
#49481=CARTESIAN_POINT('Ctrl Pts',(32.414274786044,58.1577646784655,13.));
#49482=CARTESIAN_POINT('Ctrl Pts',(32.4045647301645,58.1563099242274,13.));
#49483=CARTESIAN_POINT('Ctrl Pts',(32.3948677953976,58.1547713052596,13.));
#49484=CARTESIAN_POINT('Ctrl Pts',(32.3851848149706,58.1531483143848,13.));
#49485=CARTESIAN_POINT('Ctrl Pts',(32.3167654615574,58.141680359132,13.));
#49486=CARTESIAN_POINT('Ctrl Pts',(32.2490407706809,58.1260036975248,13.));
#49487=CARTESIAN_POINT('Ctrl Pts',(32.1823062478466,58.1063380403939,13.));
#49488=CARTESIAN_POINT('Ctrl Pts',(32.1200483333545,58.087991572208,13.));
#49489=CARTESIAN_POINT('Ctrl Pts',(32.0586518297553,58.0661723398642,13.));
#49490=CARTESIAN_POINT('Ctrl Pts',(31.9983820977037,58.041027736788,13.));
#49491=CARTESIAN_POINT('Ctrl Pts',(31.9850796184089,58.0354779267854,13.));
#49492=CARTESIAN_POINT('Ctrl Pts',(31.9718321459703,58.0297660234088,13.));
#49493=CARTESIAN_POINT('Ctrl Pts',(31.958642741509,58.0238934578502,13.));
#49494=CARTESIAN_POINT('Ctrl Pts',(31.9483333675334,58.0193032222019,13.));
#49495=CARTESIAN_POINT('Ctrl Pts',(31.9380601504676,58.0146150415553,13.));
#49496=CARTESIAN_POINT('Ctrl Pts',(31.9278362669042,58.0098353466313,13.));
#49497=CARTESIAN_POINT('Ctrl Pts',(31.8658980540082,57.9808790542455,13.));
#49498=CARTESIAN_POINT('Ctrl Pts',(31.8056527013631,57.9485169554678,13.));
#49499=CARTESIAN_POINT('Ctrl Pts',(31.7473720762079,57.9129741300425,13.));
#49500=CARTESIAN_POINT('Ctrl Pts',(31.6893603665029,57.8775953044864,13.));
#49501=CARTESIAN_POINT('Ctrl Pts',(31.6332945173391,57.8390642098787,13.));
#49502=CARTESIAN_POINT('Ctrl Pts',(31.5794782979512,57.797566170682,13.));
#49503=CARTESIAN_POINT('Ctrl Pts',(31.5268144518495,57.7569567340729,13.));
#49504=CARTESIAN_POINT('Ctrl Pts',(31.4763043636122,57.7135052606753,13.));
#49505=CARTESIAN_POINT('Ctrl Pts',(31.4282765727933,57.6673622960735,13.));
#49506=CARTESIAN_POINT('Ctrl Pts',(31.4181553624129,57.6576382874454,13.));
#49507=CARTESIAN_POINT('Ctrl Pts',(31.4081445655515,57.6477946903051,13.));
#49508=CARTESIAN_POINT('Ctrl Pts',(31.3982475480844,57.6378328286724,13.));
#49509=CARTESIAN_POINT('Ctrl Pts',(31.388870014372,57.6283938543947,13.));
#49510=CARTESIAN_POINT('Ctrl Pts',(31.3795934914324,57.6188473326524,13.));
#49511=CARTESIAN_POINT('Ctrl Pts',(31.3704354504481,57.6092101706513,13.));
#49512=CARTESIAN_POINT('Ctrl Pts',(31.3254237976821,57.5618436442967,13.));
#49513=CARTESIAN_POINT('Ctrl Pts',(31.2831878041685,57.5122078768965,13.));
#49514=CARTESIAN_POINT('Ctrl Pts',(31.2439955572223,57.4604767978076,13.));
#49515=CARTESIAN_POINT('Ctrl Pts',(31.2055484074953,57.4097291959668,13.));
#49516=CARTESIAN_POINT('Ctrl Pts',(31.1700298957995,57.356964452788,13.));
#49517=CARTESIAN_POINT('Ctrl Pts',(31.1377389872556,57.3023276232579,13.));
#49518=CARTESIAN_POINT('Ctrl Pts',(31.1064966595101,57.2494650123209,13.));
#49519=CARTESIAN_POINT('Ctrl Pts',(31.0782754670358,57.1948493079198,13.));
#49520=CARTESIAN_POINT('Ctrl Pts',(31.053394616225,57.1386036480321,13.));
#49521=CARTESIAN_POINT('Ctrl Pts',(31.0492539851721,57.1292433360518,13.));
#49522=CARTESIAN_POINT('Ctrl Pts',(31.045205981956,57.1198378750144,13.));
#49523=CARTESIAN_POINT('Ctrl Pts',(31.0412522209115,57.1103878272416,13.));
#49524=CARTESIAN_POINT('Ctrl Pts',(31.037066626976,57.1003836660893,13.));
#49525=CARTESIAN_POINT('Ctrl Pts',(31.0329866520609,57.090329535243,13.));
#49526=CARTESIAN_POINT('Ctrl Pts',(31.0290124456509,57.0802271145803,13.));
#49527=CARTESIAN_POINT('Origin',(32.5,56.2916512459885,23.5459252805377));
#49528=CARTESIAN_POINT('Ctrl Pts',(31.4704151231923,54.5113563798656,21.7959252805377));
#49529=CARTESIAN_POINT('Ctrl Pts',(31.3848836142506,54.5597932517276,21.7905813053169));
#49530=CARTESIAN_POINT('Ctrl Pts',(30.7359364258277,54.9934653968669,21.7481913665734));
#49531=CARTESIAN_POINT('Ctrl Pts',(30.0819661342964,56.5203533893187,21.6687554643073));
#49532=CARTESIAN_POINT('Ctrl Pts',(31.3808442960309,58.4469950837992,21.5576175737392));
#49533=CARTESIAN_POINT('Ctrl Pts',(33.7038051725687,58.4009643313194,21.4464796831712));
#49534=CARTESIAN_POINT('Ctrl Pts',(34.9250559921582,56.4241863460988,21.3353417926031));
#49535=CARTESIAN_POINT('Ctrl Pts',(33.9265523881077,54.326131973266,21.2242039020351));
#49536=CARTESIAN_POINT('Ctrl Pts',(32.2719558287363,54.111420270443,21.1443983980133));
#49537=CARTESIAN_POINT('Ctrl Pts',(31.5637955304719,54.4566153915593,21.1016388575141));
#49538=CARTESIAN_POINT('Ctrl Pts',(31.4731950477465,54.5099653993635,21.0959252805377));
#49539=CARTESIAN_POINT('Ctrl Pts',(31.4756555660462,54.5128362942924,21.8540747194623));
#49540=CARTESIAN_POINT('Ctrl Pts',(31.0702251268552,54.7510086370429,21.8286245525962));
#49541=CARTESIAN_POINT('Ctrl Pts',(30.2605073082537,55.6718001447715,21.7661284222074));
#49542=CARTESIAN_POINT('Ctrl Pts',(30.5464763025825,57.7337498950934,21.6665863282959));
#49543=CARTESIAN_POINT('Ctrl Pts',(32.6512600365403,58.7155097146097,21.5554484377278));
#49544=CARTESIAN_POINT('Ctrl Pts',(34.6188774786828,57.4788960204646,21.4443105471598));
#49545=CARTESIAN_POINT('Ctrl Pts',(34.6464212862449,55.1554778495401,21.3331726565918));
#49546=CARTESIAN_POINT('Ctrl Pts',(32.9604590994426,54.0382699285555,21.2364273806926));
#49547=CARTESIAN_POINT('Ctrl Pts',(31.8369684898523,54.3074066165865,21.1767280683161));
#49548=CARTESIAN_POINT('Ctrl Pts',(31.4729484072307,54.5150696468519,21.1540747194623));
#49549=CARTESIAN_POINT('Ctrl Pts',(32.1997834265915,57.930378193668,22.));
#49550=CARTESIAN_POINT('Ctrl Pts',(32.7446991236384,58.0302073467771,21.9629540364773));
#49551=CARTESIAN_POINT('Ctrl Pts',(33.932658940673,57.64135965021,21.888862109432));
#49552=CARTESIAN_POINT('Ctrl Pts',(34.4123083746051,55.8170344416491,21.7777242188639));
#49553=CARTESIAN_POINT('Ctrl Pts',(33.1376927310287,54.4290349887,21.6665863282959));
#49554=CARTESIAN_POINT('Ctrl Pts',(31.2813034436656,54.7450016890464,21.5554484377278));
#49555=CARTESIAN_POINT('Ctrl Pts',(30.5394479035103,56.4770839121465,21.4443105471598));
#49556=CARTESIAN_POINT('Ctrl Pts',(31.592583816614,58.0392131556089,21.3331726565918));
#49557=CARTESIAN_POINT('Ctrl Pts',(33.4760503309402,58.0018912265999,21.2220347660237));
#49558=CARTESIAN_POINT('Ctrl Pts',(34.4662456663514,56.3991112663237,21.1108968754557));
#49559=CARTESIAN_POINT('Ctrl Pts',(33.6566547164314,54.6979998974762,20.9997589848876));
#49560=CARTESIAN_POINT('Ctrl Pts',(31.7883942259045,54.4555617097706,20.8886210943196));
#49561=CARTESIAN_POINT('Ctrl Pts',(30.5714597638967,55.8937240769523,20.7774832037515));
#49562=CARTESIAN_POINT('Ctrl Pts',(31.1197474481277,57.6961102078823,20.6663453131835));
#49563=CARTESIAN_POINT('Ctrl Pts',(32.9313922508809,58.212980865287,20.5552074226155));
#49564=CARTESIAN_POINT('Ctrl Pts',(34.3481806801685,56.9712358625612,20.4440695320474));
#49565=CARTESIAN_POINT('Ctrl Pts',(34.07330745085,55.1074597880137,20.3329316414794));
#49566=CARTESIAN_POINT('Ctrl Pts',(32.3583685299806,54.3275873674106,20.2217937509113));
#49567=CARTESIAN_POINT('Ctrl Pts',(30.7730662696611,55.3454449973685,20.1106558603433));
#49568=CARTESIAN_POINT('Ctrl Pts',(30.7684461524674,57.2293758831938,19.9995179697753));
#49569=CARTESIAN_POINT('Ctrl Pts',(32.3487368516327,58.2549968011428,19.8883800792072));
#49570=CARTESIAN_POINT('Ctrl Pts',(34.0674804546367,57.4835452530785,19.7772421886392));
#49571=CARTESIAN_POINT('Ctrl Pts',(34.3514914067379,55.6211396100854,19.6661042980711));
#49572=CARTESIAN_POINT('Ctrl Pts',(32.9408112840734,54.3724608681775,19.5549664075031));
#49573=CARTESIAN_POINT('Ctrl Pts',(31.1266515903785,54.8804388458657,19.443828516935));
#49574=CARTESIAN_POINT('Ctrl Pts',(30.569533272628,56.680115536781,19.332690626367));
#49575=CARTESIAN_POINT('Ctrl Pts',(31.7793930425298,58.1242264572701,19.2215527357989));
#49576=CARTESIAN_POINT('Ctrl Pts',(33.6488325332889,57.8909605038465,19.1104148452309));
#49577=CARTESIAN_POINT('Ctrl Pts',(34.4667325774588,56.1938286494099,18.9992769546628));
#49578=CARTESIAN_POINT('Ctrl Pts',(33.4844599893276,54.586234926953,18.8881390640949));
#49579=CARTESIAN_POINT('Ctrl Pts',(31.6011000083735,54.539628102072,18.7770011735268));
#49580=CARTESIAN_POINT('Ctrl Pts',(30.5405133840023,56.0966679300985,18.6658632829588));
#49581=CARTESIAN_POINT('Ctrl Pts',(31.2734670813294,57.8321781984269,18.5547253923907));
#49582=CARTESIAN_POINT('Ctrl Pts',(33.1290802689521,58.1576266764213,18.4435875018227));
#49583=CARTESIAN_POINT('Ctrl Pts',(34.4088891521439,56.7751266813415,18.3324496112546));
#49584=CARTESIAN_POINT('Ctrl Pts',(33.9414701461048,54.9500961372979,18.2213117206866));
#49585=CARTESIAN_POINT('Ctrl Pts',(32.1546571679518,54.353006198509,18.1101738301185));
#49586=CARTESIAN_POINT('Ctrl Pts',(30.683940400427,55.5303800574079,17.9990359395505));
#49587=CARTESIAN_POINT('Ctrl Pts',(30.8754835799078,57.4045540686174,17.8878980489824));
#49588=CARTESIAN_POINT('Ctrl Pts',(32.5539650619684,58.260075505098,17.7767601584144));
#49589=CARTESIAN_POINT('Ctrl Pts',(34.1830517108038,57.3138758937664,17.6656222678464));
#49590=CARTESIAN_POINT('Ctrl Pts',(34.2716220416359,55.4320224695077,17.5544843772783));
#49591=CARTESIAN_POINT('Ctrl Pts',(32.7386066261983,54.3369970132152,17.4433464867103));
#49592=CARTESIAN_POINT('Ctrl Pts',(30.9871918598181,55.0310887434669,17.3322085961422));
#49593=CARTESIAN_POINT('Ctrl Pts',(30.6204675405577,56.8789876280276,17.2210707055742));
#49594=CARTESIAN_POINT('Ctrl Pts',(31.9741005967726,58.1892908612604,17.1099328150062));
#49595=CARTESIAN_POINT('Ctrl Pts',(33.8090953408664,57.7626630339378,16.9987949244381));
#49596=CARTESIAN_POINT('Ctrl Pts',(34.4458602733144,55.989601434697,16.8876570338701));
#49597=CARTESIAN_POINT('Ctrl Pts',(33.3015572300411,54.4930094532091,16.776519143302));
#49598=CARTESIAN_POINT('Ctrl Pts',(31.4235797638343,54.6427347026374,16.665381252734));
#49599=CARTESIAN_POINT('Ctrl Pts',(30.5308619472251,56.3017319641806,16.554243362166));
#49600=CARTESIAN_POINT('Ctrl Pts',(31.4405185218662,57.9515022300391,16.4431054715979));
#49601=CARTESIAN_POINT('Ctrl Pts',(33.3199305087784,58.0819920662063,16.3319675810299));
#49602=CARTESIAN_POINT('Ctrl Pts',(34.4488508023651,56.573762645781,16.2208296904618));
#49603=CARTESIAN_POINT('Ctrl Pts',(33.7939658550683,54.8073134617672,16.1096917998938));
#49604=CARTESIAN_POINT('Ctrl Pts',(31.9546992860713,54.3994954851817,15.9985539093257));
#49605=CARTESIAN_POINT('Ctrl Pts',(30.6145526446347,55.7235891349781,15.8874160187577));
#49606=CARTESIAN_POINT('Ctrl Pts',(31.0001773500497,57.5676364772256,15.7762781281896));
#49607=CARTESIAN_POINT('Ctrl Pts',(32.7586067359929,58.2437600667033,15.6651402376216));
#49608=CARTESIAN_POINT('Ctrl Pts',(34.2803304439162,57.1330963140847,15.5540023470536));
#49609=CARTESIAN_POINT('Ctrl Pts',(34.1724975057335,55.2522483481541,15.4428644564855));
#49610=CARTESIAN_POINT('Ctrl Pts',(32.5338086340801,54.3227776419367,15.3317265659175));
#49611=CARTESIAN_POINT('Ctrl Pts',(30.8641743343578,55.195439274664,15.2205886753495));
#49612=CARTESIAN_POINT('Ctrl Pts',(30.6918298216846,57.0714761554116,15.1094507847814));
#49613=CARTESIAN_POINT('Ctrl Pts',(32.1745239717376,58.2337304551949,14.9983128942134));
#49614=CARTESIAN_POINT('Ctrl Pts',(33.9551300366822,57.618377625218,14.8871750036453));
#49615=CARTESIAN_POINT('Ctrl Pts',(34.4038390465812,55.788657104035,14.7760371130773));
#49616=CARTESIAN_POINT('Ctrl Pts',(33.1099426465396,54.4193328057006,14.6648992225092));
#49617=CARTESIAN_POINT('Ctrl Pts',(31.2577587039999,54.7637628485765,14.5537613319412));
#49618=CARTESIAN_POINT('Ctrl Pts',(30.5426125496714,56.5066863904104,14.4426234413731));
#49619=CARTESIAN_POINT('Ctrl Pts',(31.6190848424819,58.0527859832773,14.3314855508051));
#49620=CARTESIAN_POINT('Ctrl Pts',(33.5018697389164,57.9868986634345,14.2203476602371));
#49621=CARTESIAN_POINT('Ctrl Pts',(34.4676299603036,56.3693327876154,14.109209769669));
#49622=CARTESIAN_POINT('Ctrl Pts',(33.6324000499911,54.680662853446,13.998071879101));
#49623=CARTESIAN_POINT('Ctrl Pts',(31.7606637541616,54.466551391645,13.886933988533));
#49624=CARTESIAN_POINT('Ctrl Pts',(30.5656658770528,55.9229694665903,13.7757960979649));
#49625=CARTESIAN_POINT('Ctrl Pts',(31.1411547963289,57.7168562799665,13.6646582073969));
#49626=CARTESIAN_POINT('Ctrl Pts',(32.9604725206547,58.2062164962561,13.5535203168288));
#49627=CARTESIAN_POINT('Ctrl Pts',(34.3581896580209,56.9431939941263,13.4423824262608));
#49628=CARTESIAN_POINT('Ctrl Pts',(34.0553346792797,55.0837258210724,13.3312445356927));
#49629=CARTESIAN_POINT('Ctrl Pts',(32.3283638467564,54.3300480294051,13.2201066451247));
#49630=CARTESIAN_POINT('Ctrl Pts',(30.7594958530051,55.3715226379038,13.1089687545567));
#49631=CARTESIAN_POINT('Ctrl Pts',(30.7817150891479,57.2558511192949,12.9978308639886));
#49632=CARTESIAN_POINT('Ctrl Pts',(32.3808507372123,58.2563466091157,12.8866929734206));
#49633=CARTESIAN_POINT('Ctrl Pts',(33.5126766583316,57.7258551932599,12.8126010463752));
#49634=CARTESIAN_POINT('Ctrl Pts',(33.8412759334222,57.2798490351089,12.7755550828525));
#49635=CARTESIAN_POINT('Ctrl Pts',(32.1764322475374,58.057840198652,22.0748149723825));
#49636=CARTESIAN_POINT('Ctrl Pts',(32.7637320936893,58.1654341743444,22.0377690088598));
#49637=CARTESIAN_POINT('Ctrl Pts',(34.0440927468328,57.7463414713666,21.9636770818144));
#49638=CARTESIAN_POINT('Ctrl Pts',(34.5610498473198,55.7801182186225,21.8525391912464));
#49639=CARTESIAN_POINT('Ctrl Pts',(33.1872931810462,54.2841586241499,21.7414013006783));
#49640=CARTESIAN_POINT('Ctrl Pts',(31.186511869781,54.624701565945,21.6302634101103));
#49641=CARTESIAN_POINT('Ctrl Pts',(30.3869539804389,56.4915070712039,21.5191255195423));
#49642=CARTESIAN_POINT('Ctrl Pts',(31.5220039764197,58.1751404650056,21.4079876289743));
#49643=CARTESIAN_POINT('Ctrl Pts',(33.551968611483,58.1349155948397,21.2968497384062));
#49644=CARTESIAN_POINT('Ctrl Pts',(34.6191824416203,56.4074696262487,21.1857118478381));
#49645=CARTESIAN_POINT('Ctrl Pts',(33.7466206069902,54.5740439227394,21.0745739572701));
#49646=CARTESIAN_POINT('Ctrl Pts',(31.7330447371731,54.312748623095,20.963436066702));
#49647=CARTESIAN_POINT('Ctrl Pts',(30.4214557589377,55.8627728590725,20.852298176134));
#49648=CARTESIAN_POINT('Ctrl Pts',(31.0123898691881,57.8053505883218,20.741160285566));
#49649=CARTESIAN_POINT('Ctrl Pts',(32.9649464200545,58.3624240204495,20.6300223949979));
#49650=CARTESIAN_POINT('Ctrl Pts',(34.4919342294714,57.0240947100387,20.5188845044299));
#49651=CARTESIAN_POINT('Ctrl Pts',(34.195681054595,55.0153520590646,20.4077466138619));
#49652=CARTESIAN_POINT('Ctrl Pts',(32.3473522766853,54.1748202940218,20.2966087232938));
#49653=CARTESIAN_POINT('Ctrl Pts',(30.6387434429966,55.2718480227484,20.1854708327258));
#49654=CARTESIAN_POINT('Ctrl Pts',(30.633763967948,57.3023131486426,20.0743329421578));
#49655=CARTESIAN_POINT('Ctrl Pts',(32.3369714356807,58.4077080025366,19.9631950515897));
#49656=CARTESIAN_POINT('Ctrl Pts',(34.1894008281341,57.5762520948665,19.8520571610217));
#49657=CARTESIAN_POINT('Ctrl Pts',(34.4955024680363,55.5689864691375,19.7409192704536));
#49658=CARTESIAN_POINT('Ctrl Pts',(32.9750980761269,54.2231841055976,19.6297813798856));
#49659=CARTESIAN_POINT('Ctrl Pts',(31.0198310233036,54.770673175488,19.5186434893175));
#49660=CARTESIAN_POINT('Ctrl Pts',(30.4193794230349,56.7103307214639,19.4075055987495));
#49661=CARTESIAN_POINT('Ctrl Pts',(31.7233434317421,58.2667661958427,19.2963677081815));
#49662=CARTESIAN_POINT('Ctrl Pts',(33.7381900057411,58.0153565570662,19.1852298176134));
#49663=CARTESIAN_POINT('Ctrl Pts',(34.6197072252154,56.1862198990258,19.0740919270454));
#49664=CARTESIAN_POINT('Ctrl Pts',(33.561032382455,54.4535857484765,18.9629540364773));
#49665=CARTESIAN_POINT('Ctrl Pts',(31.5311825670481,54.4033537929088,18.8518161459093));
#49666=CARTESIAN_POINT('Ctrl Pts',(30.3881023351889,56.0815019108803,18.7406782553412));
#49667=CARTESIAN_POINT('Ctrl Pts',(31.1780659864649,57.9520020985391,18.6295403647732));
#49668=CARTESIAN_POINT('Ctrl Pts',(33.1780108320884,58.3027643211953,18.5184024742051));
#49669=CARTESIAN_POINT('Ctrl Pts',(34.5573646739319,56.8127319385431,18.4072645836371));
#49670=CARTESIAN_POINT('Ctrl Pts',(34.053589297625,54.8457484885378,18.296126693069));
#49671=CARTESIAN_POINT('Ctrl Pts',(32.1277960183002,54.2022162300801,18.1849888025011));
#49672=CARTESIAN_POINT('Ctrl Pts',(30.5426852645059,55.4711675374879,18.073850911933));
#49673=CARTESIAN_POINT('Ctrl Pts',(30.7491268855679,57.4911168882046,17.962713021365));
#49674=CARTESIAN_POINT('Ctrl Pts',(32.5581625245214,58.4131817337352,17.8515751307969));
#49675=CARTESIAN_POINT('Ctrl Pts',(34.3139613451725,57.3933856640393,17.7404372402289));
#49676=CARTESIAN_POINT('Ctrl Pts',(34.4094207748664,55.3651595869833,17.6292993496608));
#49677=CARTESIAN_POINT('Ctrl Pts',(32.7571657150207,54.1849618325449,17.5181614590928));
#49678=CARTESIAN_POINT('Ctrl Pts',(30.869523959759,54.9330407897143,17.4070235685247));
#49679=CARTESIAN_POINT('Ctrl Pts',(30.4742754149858,56.924671305202,17.2958856779567));
#49680=CARTESIAN_POINT('Ctrl Pts',(31.9331955561555,58.3368913815559,17.1847477873886));
#49681=CARTESIAN_POINT('Ctrl Pts',(33.9109182327756,57.8770799672243,17.0736098968206));
#49682=CARTESIAN_POINT('Ctrl Pts',(34.5972114500352,55.9661076643609,16.9624720062525));
#49683=CARTESIAN_POINT('Ctrl Pts',(33.3639032430821,54.3531090936767,16.8513341156845));
#49684=CARTESIAN_POINT('Ctrl Pts',(31.339854600407,54.5144801395667,16.7401962251165));
#49685=CARTESIAN_POINT('Ctrl Pts',(30.3777001989226,56.3025160536559,16.6290583345484));
#49686=CARTESIAN_POINT('Ctrl Pts',(31.358110873882,58.0806072860715,16.5179204439804));
#49687=CARTESIAN_POINT('Ctrl Pts',(33.3837056158788,58.2212467668585,16.4067825534123));
#49688=CARTESIAN_POINT('Ctrl Pts',(34.6004345857622,56.5957055842903,16.2956446628443));
#49689=CARTESIAN_POINT('Ctrl Pts',(33.8946119587414,54.6918600176664,16.1845067722763));
#49690=CARTESIAN_POINT('Ctrl Pts',(31.9122851899249,54.252321505187,16.0733688817082));
#49691=CARTESIAN_POINT('Ctrl Pts',(30.467900451878,55.6794046320458,15.9622309911402));
#49692=CARTESIAN_POINT('Ctrl Pts',(30.8835194758665,57.6668840279746,15.8510931005722));
#49693=CARTESIAN_POINT('Ctrl Pts',(32.7787214556042,58.3955972623921,15.7399552100041));
#49694=CARTESIAN_POINT('Ctrl Pts',(34.4188065263637,57.1985448475426,15.6288173194361));
#49695=CARTESIAN_POINT('Ctrl Pts',(34.3025862222909,55.1714024344819,15.517679428868));
#49696=CARTESIAN_POINT('Ctrl Pts',(32.5364383072491,54.1696364627501,15.4065415383));
#49697=CARTESIAN_POINT('Ctrl Pts',(30.7369379943181,55.1101746880588,15.2954036477319));
#49698=CARTESIAN_POINT('Ctrl Pts',(30.5511883337254,57.1321318043788,15.1842657571639));
#49699=CARTESIAN_POINT('Ctrl Pts',(32.1492080841852,58.3847875365432,15.0731278665959));
#49700=CARTESIAN_POINT('Ctrl Pts',(34.0683116696875,57.7215718789046,14.9619899760278));
#49701=CARTESIAN_POINT('Ctrl Pts',(34.5519217655404,55.7495336601205,14.8508520854598));
#49702=CARTESIAN_POINT('Ctrl Pts',(33.1573846641151,54.2737017945638,14.7397141948917));
#49703=CARTESIAN_POINT('Ctrl Pts',(31.1611357940719,54.644921989334,14.6285763043237));
#49704=CARTESIAN_POINT('Ctrl Pts',(30.390364776299,56.5234120631583,14.5174384137557));
#49705=CARTESIAN_POINT('Ctrl Pts',(31.5505662815605,58.1897690023091,14.4063005231876));
#49706=CARTESIAN_POINT('Ctrl Pts',(33.5797962817342,58.1187568934329,14.2951626326196));
#49707=CARTESIAN_POINT('Ctrl Pts',(34.6206744074961,56.3753749443396,14.1840247420515));
#49708=CARTESIAN_POINT('Ctrl Pts',(33.7204793856121,54.555358384138,14.0728868514835));
#49709=CARTESIAN_POINT('Ctrl Pts',(31.7031573584894,54.324593094651,13.9617489609155));
#49710=CARTESIAN_POINT('Ctrl Pts',(30.4152112171297,55.8942929876505,13.8506110703474));
#49711=CARTESIAN_POINT('Ctrl Pts',(31.0354623047469,57.8277103129715,13.7394731797794));
#49712=CARTESIAN_POINT('Ctrl Pts',(32.9962885855616,58.3551335112704,13.6283352892113));
#49713=CARTESIAN_POINT('Ctrl Pts',(34.5027217167555,56.9938717138819,13.5171973986433));
#49714=CARTESIAN_POINT('Ctrl Pts',(34.1763103408583,54.9897720377719,13.4060595080752));
#49715=CARTESIAN_POINT('Ctrl Pts',(32.3150137958213,54.1774723490436,13.2949216175072));
#49716=CARTESIAN_POINT('Ctrl Pts',(30.6241175042368,55.2999540111744,13.1837837269392));
#49717=CARTESIAN_POINT('Ctrl Pts',(30.6480649772843,57.3308476580601,13.0726458363711));
#49718=CARTESIAN_POINT('Ctrl Pts',(32.3715831750057,58.4091628000752,12.9615079458031));
#49719=CARTESIAN_POINT('Ctrl Pts',(33.5914437753637,57.8374091717517,12.8874160187577));
#49720=CARTESIAN_POINT('Ctrl Pts',(33.9456018676194,57.3567121584624,12.850370055235));
#49721=CARTESIAN_POINT('Ctrl Pts',(32.1530810684833,58.1853022036361,22.149629944765));
#49722=CARTESIAN_POINT('Ctrl Pts',(32.7827650637402,58.3006610019118,22.1125839812423));
#49723=CARTESIAN_POINT('Ctrl Pts',(34.1555265529925,57.8513232925233,22.038492054197));
#49724=CARTESIAN_POINT('Ctrl Pts',(34.7097913200344,55.7432019955959,21.9273541636289));
#49725=CARTESIAN_POINT('Ctrl Pts',(33.2368936310637,54.1392822595999,21.8162162730609));
#49726=CARTESIAN_POINT('Ctrl Pts',(31.0917202958965,54.5044014428435,21.7050783824928));
#49727=CARTESIAN_POINT('Ctrl Pts',(30.2344600573676,56.5059302302613,21.5939404919248));
#49728=CARTESIAN_POINT('Ctrl Pts',(31.4514241362253,58.3110677744024,21.4828026013567));
#49729=CARTESIAN_POINT('Ctrl Pts',(33.6278868920259,58.2679399630795,21.3716647107887));
#49730=CARTESIAN_POINT('Ctrl Pts',(34.7721192168892,56.4158279861738,21.2605268202206));
#49731=CARTESIAN_POINT('Ctrl Pts',(33.836586497549,54.4500879480027,21.1493889296526));
#49732=CARTESIAN_POINT('Ctrl Pts',(31.6776952484416,54.1699355364193,21.0382510390845));
#49733=CARTESIAN_POINT('Ctrl Pts',(30.2714517539786,55.8318216411929,20.9271131485165));
#49734=CARTESIAN_POINT('Ctrl Pts',(30.9050322902485,57.9145909687611,20.8159752579484));
#49735=CARTESIAN_POINT('Ctrl Pts',(32.9985005892281,58.5118671756121,20.7048373673804));
#49736=CARTESIAN_POINT('Ctrl Pts',(34.6356877787742,57.0769535575161,20.5936994768124));
#49737=CARTESIAN_POINT('Ctrl Pts',(34.3180546583401,54.9232443301155,20.4825615862444));
#49738=CARTESIAN_POINT('Ctrl Pts',(32.3363360233899,54.022053220633,20.3714236956763));
#49739=CARTESIAN_POINT('Ctrl Pts',(30.5044206163321,55.1982510481284,20.2602858051083));
#49740=CARTESIAN_POINT('Ctrl Pts',(30.4990817834285,57.3752504140915,20.1491479145402));
#49741=CARTESIAN_POINT('Ctrl Pts',(32.3252060197288,58.5604192039304,20.0380100239722));
#49742=CARTESIAN_POINT('Ctrl Pts',(34.3113212016315,57.6689589366545,19.9268721334042));
#49743=CARTESIAN_POINT('Ctrl Pts',(34.6395135293347,55.5168333281896,19.8157342428361));
#49744=CARTESIAN_POINT('Ctrl Pts',(33.0093848681805,54.0739073430178,19.7045963522681));
#49745=CARTESIAN_POINT('Ctrl Pts',(30.9130104562287,54.6609075051103,19.5934584617));
#49746=CARTESIAN_POINT('Ctrl Pts',(30.269225573442,56.740545906147,19.482320571132));
#49747=CARTESIAN_POINT('Ctrl Pts',(31.6672938209545,58.4093059344153,19.3711826805639));
#49748=CARTESIAN_POINT('Ctrl Pts',(33.8275474781934,58.1397526102859,19.2600447899959));
#49749=CARTESIAN_POINT('Ctrl Pts',(34.7726818729719,56.1786111486417,19.1489068994278));
#49750=CARTESIAN_POINT('Ctrl Pts',(33.6376047755825,54.3209365700001,19.0377690088598));
#49751=CARTESIAN_POINT('Ctrl Pts',(31.4612651257226,54.2670794837456,18.9266311182918));
#49752=CARTESIAN_POINT('Ctrl Pts',(30.2356912863756,56.0663358916623,18.8154932277237));
#49753=CARTESIAN_POINT('Ctrl Pts',(31.0826648916003,58.0718259986511,18.7043553371557));
#49754=CARTESIAN_POINT('Ctrl Pts',(33.2269413952246,58.4479019659695,18.5932174465876));
#49755=CARTESIAN_POINT('Ctrl Pts',(34.7058401957198,56.8503371957446,18.4820795560196));
#49756=CARTESIAN_POINT('Ctrl Pts',(34.1657084491453,54.7414008397776,18.3709416654516));
#49757=CARTESIAN_POINT('Ctrl Pts',(32.1009348686486,54.0514262616511,18.2598037748835));
#49758=CARTESIAN_POINT('Ctrl Pts',(30.4014301285847,55.4119550175679,18.1486658843155));
#49759=CARTESIAN_POINT('Ctrl Pts',(30.622770191228,57.5776797077918,18.0375279937474));
#49760=CARTESIAN_POINT('Ctrl Pts',(32.5623599870745,58.5662879623725,17.9263901031794));
#49761=CARTESIAN_POINT('Ctrl Pts',(34.4448709795413,57.4728954343121,17.8152522126114));
#49762=CARTESIAN_POINT('Ctrl Pts',(34.5472195080969,55.2982967044589,17.7041143220433));
#49763=CARTESIAN_POINT('Ctrl Pts',(32.7757248038431,54.0329266518745,17.5929764314753));
#49764=CARTESIAN_POINT('Ctrl Pts',(30.7518560596998,54.8349928359617,17.4818385409072));
#49765=CARTESIAN_POINT('Ctrl Pts',(30.328083289414,56.9703549823765,17.3707006503392));
#49766=CARTESIAN_POINT('Ctrl Pts',(31.8922905155382,58.4844919018513,17.2595627597711));
#49767=CARTESIAN_POINT('Ctrl Pts',(34.0127411246847,57.9914969005107,17.1484248692031));
#49768=CARTESIAN_POINT('Ctrl Pts',(34.7485626267561,55.9426138940248,17.037286978635));
#49769=CARTESIAN_POINT('Ctrl Pts',(33.426249256123,54.2132087341443,16.926149088067));
#49770=CARTESIAN_POINT('Ctrl Pts',(31.2561294369797,54.3862255764958,16.815011197499));
#49771=CARTESIAN_POINT('Ctrl Pts',(30.2245384506201,56.3033001431311,16.7038733069309));
#49772=CARTESIAN_POINT('Ctrl Pts',(31.275703225898,58.2097123421038,16.5927354163629));
#49773=CARTESIAN_POINT('Ctrl Pts',(33.4474807229792,58.3605014675107,16.4815975257949));
#49774=CARTESIAN_POINT('Ctrl Pts',(34.7520183691595,56.6176485227996,16.3704596352268));
#49775=CARTESIAN_POINT('Ctrl Pts',(33.9952580624144,54.5764065735656,16.2593217446588));
#49776=CARTESIAN_POINT('Ctrl Pts',(31.8698710937785,54.1051475251923,16.1481838540907));
#49777=CARTESIAN_POINT('Ctrl Pts',(30.3212482591212,55.6352201291136,16.0370459635227));
#49778=CARTESIAN_POINT('Ctrl Pts',(30.7668616016832,57.7661315787236,15.9259080729546));
#49779=CARTESIAN_POINT('Ctrl Pts',(32.7988361752155,58.547434458081,15.8147701823866));
#49780=CARTESIAN_POINT('Ctrl Pts',(34.5572826088111,57.2639933810004,15.7036322918185));
#49781=CARTESIAN_POINT('Ctrl Pts',(34.4326749388484,55.0905565208099,15.5924944012505));
#49782=CARTESIAN_POINT('Ctrl Pts',(32.539067980418,54.0164952835633,15.4813565106825));
#49783=CARTESIAN_POINT('Ctrl Pts',(30.6097016542784,55.0249101014537,15.3702186201144));
#49784=CARTESIAN_POINT('Ctrl Pts',(30.4105468457662,57.192787453346,15.2590807295464));
#49785=CARTESIAN_POINT('Ctrl Pts',(32.1238921966328,58.5358446178915,15.1479428389784));
#49786=CARTESIAN_POINT('Ctrl Pts',(34.1814933026927,57.8247661325911,15.0368049484103));
#49787=CARTESIAN_POINT('Ctrl Pts',(34.7000044844997,55.710410216206,14.9256670578423));
#49788=CARTESIAN_POINT('Ctrl Pts',(33.2048266816905,54.128070783427,14.8145291672742));
#49789=CARTESIAN_POINT('Ctrl Pts',(31.064512884144,54.5260811300915,14.7033912767062));
#49790=CARTESIAN_POINT('Ctrl Pts',(30.2381170029266,56.5401377359063,14.5922533861381));
#49791=CARTESIAN_POINT('Ctrl Pts',(31.4820477206391,58.3267520213408,14.4811154955701));
#49792=CARTESIAN_POINT('Ctrl Pts',(33.6577228245521,58.2506151234314,14.369977605002));
#49793=CARTESIAN_POINT('Ctrl Pts',(34.7737188546885,56.3814171010637,14.258839714434));
#49794=CARTESIAN_POINT('Ctrl Pts',(33.8085587212332,54.4300539148302,14.147701823866));
#49795=CARTESIAN_POINT('Ctrl Pts',(31.6456509628172,54.182634797657,14.0365639332979));
#49796=CARTESIAN_POINT('Ctrl Pts',(30.2647565572066,55.8656165087107,13.9254260427299));
#49797=CARTESIAN_POINT('Ctrl Pts',(30.9297698131648,57.9385643459764,13.8142881521619));
#49798=CARTESIAN_POINT('Ctrl Pts',(33.0321046504684,58.5040505262847,13.7031502615938));
#49799=CARTESIAN_POINT('Ctrl Pts',(34.6472537754902,57.0445494336376,13.5920123710258));
#49800=CARTESIAN_POINT('Ctrl Pts',(34.2972860024369,54.8958182544712,13.4808744804577));
#49801=CARTESIAN_POINT('Ctrl Pts',(32.3016637448862,54.0248966686821,13.3697365898897));
#49802=CARTESIAN_POINT('Ctrl Pts',(30.4887391554684,55.2283853844451,13.2585986993216));
#49803=CARTESIAN_POINT('Ctrl Pts',(30.5144148654208,57.4058441968251,13.1474608087536));
#49804=CARTESIAN_POINT('Ctrl Pts',(32.3623156127991,58.5619789910347,13.0363229181856));
#49805=CARTESIAN_POINT('Ctrl Pts',(33.6702108923958,57.9489631502434,12.9622309911402));
#49806=CARTESIAN_POINT('Ctrl Pts',(34.0499278018167,57.4335752818158,12.9251850276175));
#49807=CARTESIAN_POINT('Ctrl Pts',(32.1297298894291,58.3127642086202,22.2244449171475));
#49808=CARTESIAN_POINT('Ctrl Pts',(32.8017980337912,58.4358878294791,22.1873989536248));
#49809=CARTESIAN_POINT('Ctrl Pts',(34.2669603591523,57.95630511368,22.1133070265794));
#49810=CARTESIAN_POINT('Ctrl Pts',(34.858532792749,55.7062857725693,22.0021691360114));
#49811=CARTESIAN_POINT('Ctrl Pts',(33.2864940810812,53.9944058950499,21.8910312454434));
#49812=CARTESIAN_POINT('Ctrl Pts',(30.9969287220119,54.384101319742,21.7798933548753));
#49813=CARTESIAN_POINT('Ctrl Pts',(30.0819661342964,56.5203533893187,21.6687554643073));
#49814=CARTESIAN_POINT('Ctrl Pts',(31.3808442960309,58.4469950837992,21.5576175737392));
#49815=CARTESIAN_POINT('Ctrl Pts',(33.7038051725687,58.4009643313194,21.4464796831712));
#49816=CARTESIAN_POINT('Ctrl Pts',(34.9250559921582,56.4241863460988,21.3353417926031));
#49817=CARTESIAN_POINT('Ctrl Pts',(33.9265523881077,54.326131973266,21.2242039020351));
#49818=CARTESIAN_POINT('Ctrl Pts',(31.6223457597102,54.0271224497437,21.113066011467));
#49819=CARTESIAN_POINT('Ctrl Pts',(30.1214477490197,55.8008704233132,21.001928120899));
#49820=CARTESIAN_POINT('Ctrl Pts',(30.7976747113088,58.0238313492005,20.890790230331));
#49821=CARTESIAN_POINT('Ctrl Pts',(33.0320547584019,58.6613103307746,20.7796523397629));
#49822=CARTESIAN_POINT('Ctrl Pts',(34.7794413280769,57.1298124049937,20.6685144491949));
#49823=CARTESIAN_POINT('Ctrl Pts',(34.4404282620852,54.8311366011664,20.5573765586268));
#49824=CARTESIAN_POINT('Ctrl Pts',(32.3253197700946,53.8692861472442,20.4462386680588));
#49825=CARTESIAN_POINT('Ctrl Pts',(30.3700977896676,55.1246540735083,20.3351007774907));
#49826=CARTESIAN_POINT('Ctrl Pts',(30.364399598909,57.4481876795404,20.2239628869227));
#49827=CARTESIAN_POINT('Ctrl Pts',(32.3134406037768,58.7131304053242,20.1128249963547));
#49828=CARTESIAN_POINT('Ctrl Pts',(34.4332415751289,57.7616657784424,20.0016871057866));
#49829=CARTESIAN_POINT('Ctrl Pts',(34.7835245906331,55.4646801872418,19.8905492152186));
#49830=CARTESIAN_POINT('Ctrl Pts',(33.043671660234,53.9246305804379,19.7794113246506));
#49831=CARTESIAN_POINT('Ctrl Pts',(30.8061898891538,54.5511418347326,19.6682734340825));
#49832=CARTESIAN_POINT('Ctrl Pts',(30.1190717238489,56.77076109083,19.5571355435145));
#49833=CARTESIAN_POINT('Ctrl Pts',(31.6112442101669,58.5518456729879,19.4459976529464));
#49834=CARTESIAN_POINT('Ctrl Pts',(33.9169049506455,58.2641486635057,19.3348597623784));
#49835=CARTESIAN_POINT('Ctrl Pts',(34.9256565207284,56.1710023982575,19.2237218718104));
#49836=CARTESIAN_POINT('Ctrl Pts',(33.71417716871,54.1882873915237,19.1125839812423));
#49837=CARTESIAN_POINT('Ctrl Pts',(31.3913476843971,54.1308051745824,19.0014460906743));
#49838=CARTESIAN_POINT('Ctrl Pts',(30.0832802375622,56.0511698724442,18.8903082001062));
#49839=CARTESIAN_POINT('Ctrl Pts',(30.9872637967357,58.1916498987633,18.7791703095382));
#49840=CARTESIAN_POINT('Ctrl Pts',(33.275871958361,58.5930396107435,18.6680324189701));
#49841=CARTESIAN_POINT('Ctrl Pts',(34.8543157175076,56.8879424529462,18.5568945284021));
#49842=CARTESIAN_POINT('Ctrl Pts',(34.2778276006656,54.6370531910173,18.445756637834));
#49843=CARTESIAN_POINT('Ctrl Pts',(32.0740737189969,53.9006362932223,18.334618747266));
#49844=CARTESIAN_POINT('Ctrl Pts',(30.2601749926635,55.3527424976477,18.223480856698));
#49845=CARTESIAN_POINT('Ctrl Pts',(30.4964134968881,57.664242527379,18.1123429661299));
#49846=CARTESIAN_POINT('Ctrl Pts',(32.5665574496276,58.7193941910096,18.0012050755619));
#49847=CARTESIAN_POINT('Ctrl Pts',(34.57578061391,57.552405204585,17.8900671849938));
#49848=CARTESIAN_POINT('Ctrl Pts',(34.6850182413274,55.2314338219344,17.7789292944258));
#49849=CARTESIAN_POINT('Ctrl Pts',(32.7942838926656,53.8808914712041,17.6677914038577));
#49850=CARTESIAN_POINT('Ctrl Pts',(30.6341881596407,54.7369448822092,17.5566535132897));
#49851=CARTESIAN_POINT('Ctrl Pts',(30.181891163842,57.0160386595509,17.4455156227217));
#49852=CARTESIAN_POINT('Ctrl Pts',(31.8513854749211,58.6320924221469,17.3343777321536));
#49853=CARTESIAN_POINT('Ctrl Pts',(34.1145640165938,58.105913833797,17.2232398415856));
#49854=CARTESIAN_POINT('Ctrl Pts',(34.899913803477,55.9191201236888,17.1121019510176));
#49855=CARTESIAN_POINT('Ctrl Pts',(33.4885952691639,54.0733083746118,17.0009640604495));
#49856=CARTESIAN_POINT('Ctrl Pts',(31.1724042735525,54.2579710134251,16.8898261698815));
#49857=CARTESIAN_POINT('Ctrl Pts',(30.0713767023175,56.3040842326063,16.7786882793134));
#49858=CARTESIAN_POINT('Ctrl Pts',(31.1932955779139,58.3388173981362,16.6675503887454));
#49859=CARTESIAN_POINT('Ctrl Pts',(33.5112558300795,58.4997561681628,16.5564124981773));
#49860=CARTESIAN_POINT('Ctrl Pts',(34.9036021525568,56.6395914613089,16.4452746076093));
#49861=CARTESIAN_POINT('Ctrl Pts',(34.0959041660874,54.4609531294646,16.3341367170413));
#49862=CARTESIAN_POINT('Ctrl Pts',(31.8274569976321,53.9579735451976,16.2229988264732));
#49863=CARTESIAN_POINT('Ctrl Pts',(30.1745960663645,55.5910356261813,16.1118609359052));
#49864=CARTESIAN_POINT('Ctrl Pts',(30.6502037274999,57.8653791294726,16.0007230453371));
#49865=CARTESIAN_POINT('Ctrl Pts',(32.8189508948268,58.6992716537698,15.8895851547691));
#49866=CARTESIAN_POINT('Ctrl Pts',(34.6957586912586,57.3294419144583,15.778447264201));
#49867=CARTESIAN_POINT('Ctrl Pts',(34.5627636554058,55.0097106071378,15.667309373633));
#49868=CARTESIAN_POINT('Ctrl Pts',(32.541697653587,53.8633541043766,15.556171483065));
#49869=CARTESIAN_POINT('Ctrl Pts',(30.4824653142387,54.9396455148486,15.4450335924969));
#49870=CARTESIAN_POINT('Ctrl Pts',(30.269905357807,57.2534431023133,15.3338957019289));
#49871=CARTESIAN_POINT('Ctrl Pts',(32.0985763090804,58.6869016992398,15.2227578113608));
#49872=CARTESIAN_POINT('Ctrl Pts',(34.2946749356979,57.9279603862777,15.1116199207928));
#49873=CARTESIAN_POINT('Ctrl Pts',(34.848087203459,55.6712867722916,15.0004820302248));
#49874=CARTESIAN_POINT('Ctrl Pts',(33.2522686992661,53.9824397722901,14.8893441396567));
#49875=CARTESIAN_POINT('Ctrl Pts',(30.9678899742159,54.4072402708491,14.7782062490887));
#49876=CARTESIAN_POINT('Ctrl Pts',(30.0858692295542,56.5568634086541,14.6670683585206));
#49877=CARTESIAN_POINT('Ctrl Pts',(31.4135291597177,58.4637350403728,14.5559304679526));
#49878=CARTESIAN_POINT('Ctrl Pts',(33.73564936737,58.3824733534297,14.4447925773845));
#49879=CARTESIAN_POINT('Ctrl Pts',(34.926763301881,56.387459257788,14.3336546868165));
#49880=CARTESIAN_POINT('Ctrl Pts',(33.8966380568543,54.3047494455222,14.2225167962484));
#49881=CARTESIAN_POINT('Ctrl Pts',(31.588144567145,54.040676500663,14.1113789056804));
#49882=CARTESIAN_POINT('Ctrl Pts',(30.1143018972834,55.8369400297709,14.0002410151124));
#49883=CARTESIAN_POINT('Ctrl Pts',(30.8240773215828,58.0494183789814,13.8891031245444));
#49884=CARTESIAN_POINT('Ctrl Pts',(33.0679207153753,58.652967541299,13.7779652339763));
#49885=CARTESIAN_POINT('Ctrl Pts',(34.7917858342248,57.0952271533931,13.6668273434083));
#49886=CARTESIAN_POINT('Ctrl Pts',(34.4182616640155,54.8018644711708,13.5556894528402));
#49887=CARTESIAN_POINT('Ctrl Pts',(32.2883136939512,53.8723209883206,13.4445515622722));
#49888=CARTESIAN_POINT('Ctrl Pts',(30.3533608067,55.1568167577159,13.3334136717041));
#49889=CARTESIAN_POINT('Ctrl Pts',(30.3807647535574,57.4808407355902,13.2222757811361));
#49890=CARTESIAN_POINT('Ctrl Pts',(32.3530480505924,58.7147951819942,13.1111378905681));
#49891=CARTESIAN_POINT('Ctrl Pts',(33.7489780094279,58.0605171287351,13.0370459635227));
#49892=CARTESIAN_POINT('Ctrl Pts',(34.1542537360139,57.5104384051693,13.));
#49893=CARTESIAN_POINT('Ctrl Pts',(32.1997834265915,57.930378193668,22.));
#49894=CARTESIAN_POINT('Ctrl Pts',(32.2590684210022,57.9484903047673,22.));
#49895=CARTESIAN_POINT('Ctrl Pts',(32.3192133660458,57.9629534896909,22.));
#49896=CARTESIAN_POINT('Ctrl Pts',(32.3799202087184,57.9739415995511,22.));
#49897=CARTESIAN_POINT('Ctrl Pts',(32.444639033103,57.9856558894244,22.));
#49898=CARTESIAN_POINT('Ctrl Pts',(32.5099970425744,57.9934211178934,22.));
#49899=CARTESIAN_POINT('Ctrl Pts',(32.5756660758642,57.9973955895089,22.));
#49900=CARTESIAN_POINT('Ctrl Pts',(32.6331264799928,58.0008732521725,22.));
#49901=CARTESIAN_POINT('Ctrl Pts',(32.6908259516985,58.0014477926639,22.));
#49902=CARTESIAN_POINT('Ctrl Pts',(32.7485570677748,57.9991916498582,22.));
#49903=CARTESIAN_POINT('Ctrl Pts',(32.7775225242247,57.9980596744068,22.));
#49904=CARTESIAN_POINT('Ctrl Pts',(32.8064960744379,57.9962146309829,22.));
#49905=CARTESIAN_POINT('Ctrl Pts',(32.835451944398,57.9936627183818,22.));
#49906=CARTESIAN_POINT('Ctrl Pts',(32.8486814477591,57.9924967877302,22.));
#49907=CARTESIAN_POINT('Ctrl Pts',(32.8619089919324,57.9911829627172,22.));
#49908=CARTESIAN_POINT('Ctrl Pts',(32.8751106150215,57.9897244385923,22.));
#49909=CARTESIAN_POINT('Ctrl Pts',(32.9416845684884,57.9823693038058,22.));
#49910=CARTESIAN_POINT('Ctrl Pts',(33.0077191568773,57.9713290351855,22.));
#49911=CARTESIAN_POINT('Ctrl Pts',(33.0728927906167,57.9567622281301,22.));
#49912=CARTESIAN_POINT('Ctrl Pts',(33.1392231872555,57.9419368756937,22.));
#49913=CARTESIAN_POINT('Ctrl Pts',(33.2046628033558,57.9234587511869,22.));
#49914=CARTESIAN_POINT('Ctrl Pts',(33.2688845825783,57.9014427391656,22.));
#49915=CARTESIAN_POINT('Ctrl Pts',(33.3226052862653,57.8830266243757,22.));
#49916=CARTESIAN_POINT('Ctrl Pts',(33.3754743938636,57.8621340596232,22.));
#49917=CARTESIAN_POINT('Ctrl Pts',(33.4272987060795,57.8388046347794,22.));
#49918=CARTESIAN_POINT('Ctrl Pts',(33.4511753909343,57.8280562176558,22.));
#49919=CARTESIAN_POINT('Ctrl Pts',(33.4748302313212,57.8167901903403,22.));
#49920=CARTESIAN_POINT('Ctrl Pts',(33.4982437788543,57.8050086614947,22.));
#49921=CARTESIAN_POINT('Ctrl Pts',(33.5084650463737,57.7998653931392,22.));
#49922=CARTESIAN_POINT('Ctrl Pts',(33.5186400681057,57.7946238947706,22.));
#49923=CARTESIAN_POINT('Ctrl Pts',(33.528754861639,57.7892910972011,22.));
#49924=CARTESIAN_POINT('Ctrl Pts',(33.5908341911969,57.7565611658687,22.));
#49925=CARTESIAN_POINT('Ctrl Pts',(33.6507646084389,57.7203369576125,22.));
#49926=CARTESIAN_POINT('Ctrl Pts',(33.7082063151528,57.6807516371278,22.));
#49927=CARTESIAN_POINT('Ctrl Pts',(33.759565116146,57.6453582842258,22.));
#49928=CARTESIAN_POINT('Ctrl Pts',(33.808935052041,57.6072772063167,22.));
#49929=CARTESIAN_POINT('Ctrl Pts',(33.8560671885274,57.566568812704,22.));
#49930=CARTESIAN_POINT('Ctrl Pts',(33.9074138354698,57.5222203135644,22.));
#49931=CARTESIAN_POINT('Ctrl Pts',(33.9561058514871,57.4747541508594,22.));
#49932=CARTESIAN_POINT('Ctrl Pts',(34.0020809130285,57.4244894418761,22.));
#49933=CARTESIAN_POINT('Ctrl Pts',(34.0198184128282,57.4050969661376,22.));
#49934=CARTESIAN_POINT('Ctrl Pts',(34.0371511842955,57.3852874792601,22.));
#49935=CARTESIAN_POINT('Ctrl Pts',(34.0540743682382,57.3650777298663,22.));
#49936=CARTESIAN_POINT('Ctrl Pts',(34.0614983915351,57.3562119247771,22.));
#49937=CARTESIAN_POINT('Ctrl Pts',(34.0688431367373,57.347269477393,22.));
#49938=CARTESIAN_POINT('Ctrl Pts',(34.0760999004165,57.3382624488906,22.));
#49939=CARTESIAN_POINT('Ctrl Pts',(34.1199740931949,57.2838062033321,22.));
#49940=CARTESIAN_POINT('Ctrl Pts',(34.1607162740126,57.2268964747805,22.));
#49941=CARTESIAN_POINT('Ctrl Pts',(34.1982933189745,57.1679133931306,22.));
#49942=CARTESIAN_POINT('Ctrl Pts',(34.2367405668772,57.107564391112,22.));
#49943=CARTESIAN_POINT('Ctrl Pts',(34.2718749445021,57.0450442239911,22.));
#49944=CARTESIAN_POINT('Ctrl Pts',(34.3036296838761,56.9807132904727,22.));
#49945=CARTESIAN_POINT('Ctrl Pts',(34.3279241124351,56.9314959673484,22.));
#49946=CARTESIAN_POINT('Ctrl Pts',(34.3502397773158,56.8812176908655,22.));
#49947=CARTESIAN_POINT('Ctrl Pts',(34.3705317464917,56.8300260001665,22.));
#49948=CARTESIAN_POINT('Ctrl Pts',(34.3831626883555,56.7981612134855,22.));
#49949=CARTESIAN_POINT('Ctrl Pts',(34.3950092682846,56.765942300049,22.));
#49950=CARTESIAN_POINT('Ctrl Pts',(34.4060577406907,56.7334031737725,22.));
#49951=CARTESIAN_POINT('Ctrl Pts',(34.4122566000748,56.7151467614053,22.));
#49952=CARTESIAN_POINT('Ctrl Pts',(34.4182059308302,56.6967833656075,22.));
#49953=CARTESIAN_POINT('Ctrl Pts',(34.4238930916556,56.6783523613184,22.));
#49954=CARTESIAN_POINT('Ctrl Pts',(34.4459473654135,56.6068786635096,22.));
#49955=CARTESIAN_POINT('Ctrl Pts',(34.4640895873943,56.5343189897469,22.));
#49956=CARTESIAN_POINT('Ctrl Pts',(34.4782337109615,56.4610520163694,22.));
#49957=CARTESIAN_POINT('Ctrl Pts',(34.4888128880618,56.4062515698597,22.));
#49958=CARTESIAN_POINT('Ctrl Pts',(34.4971546283919,56.3510545308308,22.));
#49959=CARTESIAN_POINT('Ctrl Pts',(34.5032062803039,56.2956100237494,22.));
#49960=CARTESIAN_POINT('Ctrl Pts',(34.5050941235412,56.27831383103,22.));
#49961=CARTESIAN_POINT('Ctrl Pts',(34.5067589921265,56.2609935141503,22.));
#49962=CARTESIAN_POINT('Ctrl Pts',(34.5081989725347,56.2436535052303,22.));
#49963=CARTESIAN_POINT('Ctrl Pts',(34.5095888645054,56.2269166530962,22.));
#49964=CARTESIAN_POINT('Ctrl Pts',(34.5107684790971,56.2101700013467,22.));
#49965=CARTESIAN_POINT('Ctrl Pts',(34.51173640528,56.1934236229305,22.));
#49966=CARTESIAN_POINT('Ctrl Pts',(34.5160829441441,56.118222862889,22.));
#49967=CARTESIAN_POINT('Ctrl Pts',(34.5161676811359,56.042991394141,22.));
#49968=CARTESIAN_POINT('Ctrl Pts',(34.511879539708,55.9680950252592,22.));
#49969=CARTESIAN_POINT('Ctrl Pts',(34.5085977311836,55.9107751942845,22.));
#49970=CARTESIAN_POINT('Ctrl Pts',(34.5027538123388,55.8536509962994,22.));
#49971=CARTESIAN_POINT('Ctrl Pts',(34.4942777735197,55.7968820122819,22.));
#49972=CARTESIAN_POINT('Ctrl Pts',(34.4923107028765,55.783707390942,22.));
#49973=CARTESIAN_POINT('Ctrl Pts',(34.4902017904221,55.7705518962168,22.));
#49974=CARTESIAN_POINT('Ctrl Pts',(34.4879524958972,55.7574168944054,22.));
#49975=CARTESIAN_POINT('Ctrl Pts',(31.6674621971265,54.8470528177236,20.8714803633902));
#49976=CARTESIAN_POINT('Ctrl Pts',(31.740921452131,54.8037964055072,20.8771939403667));
#49977=CARTESIAN_POINT('Ctrl Pts',(31.8176439327865,54.7663977740574,20.8829075173431));
#49978=CARTESIAN_POINT('Ctrl Pts',(31.896948563991,54.7356618022518,20.8886210943196));
#49979=CARTESIAN_POINT('Ctrl Pts',(32.4111477227468,54.5363744390058,20.9256670578423));
#49980=CARTESIAN_POINT('Ctrl Pts',(33.0339012195891,54.617187168241,20.9627130213649));
#49981=CARTESIAN_POINT('Ctrl Pts',(33.4802097929969,54.9411120943332,20.9997589848876));
#49982=CARTESIAN_POINT('Ctrl Pts',(33.9265183664047,55.2650370204254,21.0368049484103));
#49983=CARTESIAN_POINT('Ctrl Pts',(34.1963820163781,55.8320741433745,21.073850911933));
#49984=CARTESIAN_POINT('Ctrl Pts',(34.1662812854629,56.3827226982285,21.1108968754557));
#49985=CARTESIAN_POINT('Ctrl Pts',(34.1361805545477,56.9333712530824,21.1479428389783));
#49986=CARTESIAN_POINT('Ctrl Pts',(33.8061154427439,57.4676312398411,21.184988802501));
#49987=CARTESIAN_POINT('Ctrl Pts',(33.327171801121,57.740981554722,21.2220347660237));
#49988=CARTESIAN_POINT('Ctrl Pts',(32.8482281594981,58.0143318696029,21.2590807295464));
#49989=CARTESIAN_POINT('Ctrl Pts',(32.220405988056,58.0267725126059,21.2961266930691));
#49990=CARTESIAN_POINT('Ctrl Pts',(31.7309722501511,57.772637960197,21.3331726565918));
#49991=CARTESIAN_POINT('Ctrl Pts',(31.2415385122461,57.5185034077881,21.3702186201144));
#49992=CARTESIAN_POINT('Ctrl Pts',(30.8904932078782,56.9977936599673,21.4072645836371));
#49993=CARTESIAN_POINT('Ctrl Pts',(30.8386131457201,56.4487584155402,21.4443105471598));
#49994=CARTESIAN_POINT('Ctrl Pts',(30.786733083562,55.8997231711131,21.4813565106825));
#49995=CARTESIAN_POINT('Ctrl Pts',(31.0340182636138,55.3223624300798,21.5184024742052));
#49996=CARTESIAN_POINT('Ctrl Pts',(31.4670590682002,54.9810209428387,21.5554484377278));
#49997=CARTESIAN_POINT('Ctrl Pts',(31.5295263145409,54.9317815581341,21.5607924129486));
#49998=CARTESIAN_POINT('Ctrl Pts',(31.5958589129293,54.8874534513961,21.5661363881694));
#49999=CARTESIAN_POINT('Ctrl Pts',(31.6652082225275,54.8481806306042,21.5714803633902));
#50000=CARTESIAN_POINT('Ctrl Pts',(33.9541262883781,54.8399232067375,22.));
#50001=CARTESIAN_POINT('Ctrl Pts',(33.4713921772736,54.3563916207415,21.9629540364773));
#50002=CARTESIAN_POINT('Ctrl Pts',(31.9935412717563,53.9174716604953,21.8888621094319));
#50003=CARTESIAN_POINT('Ctrl Pts',(30.2271943832588,55.4316007569426,21.7777242188639));
#50004=CARTESIAN_POINT('Ctrl Pts',(30.5464763025825,57.7337498950934,21.6665863282959));
#50005=CARTESIAN_POINT('Ctrl Pts',(32.6512600365403,58.7155097146097,21.5554484377278));
#50006=CARTESIAN_POINT('Ctrl Pts',(34.6188774786828,57.4788960204646,21.4443105471598));
#50007=CARTESIAN_POINT('Ctrl Pts',(34.6464212862449,55.1554778495401,21.3331726565918));
#50008=CARTESIAN_POINT('Ctrl Pts',(32.7096416422032,53.872064985086,21.2220347660237));
#50009=CARTESIAN_POINT('Ctrl Pts',(30.5808145803544,54.8033004251176,21.1108968754557));
#50010=CARTESIAN_POINT('Ctrl Pts',(30.2087196709517,57.0968534624393,20.9997589848876));
#50011=CARTESIAN_POINT('Ctrl Pts',(31.9338196700205,58.6533891775714,20.8886210943196));
#50012=CARTESIAN_POINT('Ctrl Pts',(34.1771709144469,58.0482026788783,20.7774832037515));
#50013=CARTESIAN_POINT('Ctrl Pts',(34.8853786224564,55.8352230845946,20.6663453131835));
#50014=CARTESIAN_POINT('Ctrl Pts',(33.4102272112105,54.0400181863803,20.5552074226154));
#50015=CARTESIAN_POINT('Ctrl Pts',(31.1019320194545,54.3057581512874,20.4440695320474));
#50016=CARTESIAN_POINT('Ctrl Pts',(30.0733055503939,56.3892087930031,20.3329316414794));
#50017=CARTESIAN_POINT('Ctrl Pts',(31.2658594095642,58.3833638027877,20.2217937509113));
#50018=CARTESIAN_POINT('Ctrl Pts',(33.5880364581139,58.4629506390537,20.1106558603433));
#50019=CARTESIAN_POINT('Ctrl Pts',(34.914321242052,56.5551224909764,19.9995179697752));
#50020=CARTESIAN_POINT('Ctrl Pts',(34.0307504904903,54.406136137217,19.8883800792072));
#50021=CARTESIAN_POINT('Ctrl Pts',(31.7460664163078,53.9829831393046,19.7772421886392));
#50022=CARTESIAN_POINT('Ctrl Pts',(30.151466320847,55.6729802447186,19.6661042980711));
#50023=CARTESIAN_POINT('Ctrl Pts',(30.7065057264144,57.9292539322016,19.5549664075031));
#50024=CARTESIAN_POINT('Ctrl Pts',(32.9031507850421,58.6866113101155,19.443828516935));
#50025=CARTESIAN_POINT('Ctrl Pts',(34.7307873556619,57.2518345802401,19.332690626367));
#50026=CARTESIAN_POINT('Ctrl Pts',(34.5165589620033,54.9381911555042,19.221552735799));
#50027=CARTESIAN_POINT('Ctrl Pts',(32.4565512804853,53.8633851007703,19.1104148452309));
#50028=CARTESIAN_POINT('Ctrl Pts',(30.4363127049828,55.0111985872154,18.9992769546629));
#50029=CARTESIAN_POINT('Ctrl Pts',(30.3049905142645,57.3310249135316,18.8881390640948));
#50030=CARTESIAN_POINT('Ctrl Pts',(32.1827853990159,58.6995007346589,18.7770011735268));
#50031=CARTESIAN_POINT('Ctrl Pts',(34.3509304054687,57.8640446119295,18.6658632829587));
#50032=CARTESIAN_POINT('Ctrl Pts',(34.8248978208363,55.5893590092039,18.5547253923907));
#50033=CARTESIAN_POINT('Ctrl Pts',(33.1708598946486,53.9574894553413,18.4435875018226));
#50034=CARTESIAN_POINT('Ctrl Pts',(30.902776298825,54.462104659654,18.3324496112546));
#50035=CARTESIAN_POINT('Ctrl Pts',(30.0966496704334,56.6413246029078,18.2213117206866));
#50036=CARTESIAN_POINT('Ctrl Pts',(31.4903368545417,58.5004845570079,18.1101738301185));
#50037=CARTESIAN_POINT('Ctrl Pts',(33.8081801660464,58.3378743316585,17.9990359395505));
#50038=CARTESIAN_POINT('Ctrl Pts',(34.9286313357969,56.3023329102471,17.8878980489824));
#50039=CARTESIAN_POINT('Ctrl Pts',(33.8261287013398,54.2570144404017,17.7767601584144));
#50040=CARTESIAN_POINT('Ctrl Pts',(31.5098054272241,54.0740221130605,17.6656222678464));
#50041=CARTESIAN_POINT('Ctrl Pts',(30.0998184751403,55.9208508807133,17.5544843772783));
#50042=CARTESIAN_POINT('Ctrl Pts',(30.8867448926705,58.1070774278645,17.4433464867103));
#50043=CARTESIAN_POINT('Ctrl Pts',(33.1503020054966,58.6316238024116,17.3322085961423));
#50044=CARTESIAN_POINT('Ctrl Pts',(34.8186303177654,57.0143667589708,17.2210707055742));
#50045=CARTESIAN_POINT('Ctrl Pts',(34.3646900051272,54.7356000103461,17.1099328150062));
#50046=CARTESIAN_POINT('Ctrl Pts',(32.2039777837733,53.881104604526,16.9987949244381));
#50047=CARTESIAN_POINT('Ctrl Pts',(30.3142180540518,55.2330098770949,16.8876570338701));
#50048=CARTESIAN_POINT('Ctrl Pts',(30.4251293279101,57.5539016004218,16.776519143302));
#50049=CARTESIAN_POINT('Ctrl Pts',(32.4351932585659,58.7194412594432,16.665381252734));
#50050=CARTESIAN_POINT('Ctrl Pts',(34.5045755346152,57.6627971861383,16.554243362166));
#50051=CARTESIAN_POINT('Ctrl Pts',(34.7391470903975,55.3511276839614,16.4431054715979));
#50052=CARTESIAN_POINT('Ctrl Pts',(32.924201920686,53.9003300643712,16.3319675810299));
#50053=CARTESIAN_POINT('Ctrl Pts',(30.7209799221891,54.6383358417407,16.2208296904618));
#50054=CARTESIAN_POINT('Ctrl Pts',(30.1461151763815,56.8896399584928,16.1096917998938));
#50055=CARTESIAN_POINT('Ctrl Pts',(31.7257879044833,58.5935982250311,15.9985539093258));
#50056=CARTESIAN_POINT('Ctrl Pts',(34.0141057438103,58.1905583158083,15.8874160187577));
#50057=CARTESIAN_POINT('Ctrl Pts',(34.9165454246276,56.0494272304867,15.7762781281897));
#50058=CARTESIAN_POINT('Ctrl Pts',(33.6070936729406,54.130006533605,15.6651402376216));
#50059=CARTESIAN_POINT('Ctrl Pts',(31.284306526822,54.1891637565984,15.5540023470536));
#50060=CARTESIAN_POINT('Ctrl Pts',(30.074257404191,56.1727516226363,15.4428644564855));
#50061=CARTESIAN_POINT('Ctrl Pts',(31.0845179881232,58.2651696619898,15.3317265659175));
#50062=CARTESIAN_POINT('Ctrl Pts',(33.3903853125313,58.551203914661,15.2205886753495));
#50063=CARTESIAN_POINT('Ctrl Pts',(34.881272858026,56.7690439832157,15.1094507847814));
#50064=CARTESIAN_POINT('Ctrl Pts',(34.192554360499,54.5499210682071,14.9983128942134));
#50065=CARTESIAN_POINT('Ctrl Pts',(31.9546216431227,53.9250235318367,14.8871750036453));
#50066=CARTESIAN_POINT('Ctrl Pts',(30.2158799584561,55.4663271929179,14.7760371130773));
#50067=CARTESIAN_POINT('Ctrl Pts',(30.5678191761536,57.7630592969624,14.6648992225092));
#50068=CARTESIAN_POINT('Ctrl Pts',(32.6883055651204,58.7129949703237,14.5537613319412));
#50069=CARTESIAN_POINT('Ctrl Pts',(34.6364334330514,57.4466471822884,14.4426234413732));
#50070=CARTESIAN_POINT('Ctrl Pts',(34.6290601547835,55.1231186965397,14.3314855508051));
#50071=CARTESIAN_POINT('Ctrl Pts',(32.6729327631563,53.8691609424835,14.2203476602371));
#50072=CARTESIAN_POINT('Ctrl Pts',(30.5585204707244,54.8325367623412,14.109209769669));
#50073=CARTESIAN_POINT('Ctrl Pts',(30.2211615693062,57.1314551632494,13.998071879101));
#50074=CARTESIAN_POINT('Ctrl Pts',(31.969659013309,58.6616944230992,13.886933988533));
#50075=CARTESIAN_POINT('Ctrl Pts',(34.2035641928434,58.0226004643432,13.7757960979649));
#50076=CARTESIAN_POINT('Ctrl Pts',(34.8782165391171,55.7991607039093,13.6646582073969));
#50077=CARTESIAN_POINT('Ctrl Pts',(33.3759826838065,54.0264798110272,13.5535203168288));
#50078=CARTESIAN_POINT('Ctrl Pts',(31.072107305341,54.3271826722053,13.4423824262608));
#50079=CARTESIAN_POINT('Ctrl Pts',(30.0748873839319,56.4258925346357,13.3312445356927));
#50080=CARTESIAN_POINT('Ctrl Pts',(31.2980228170538,58.4019167094404,13.2201066451247));
#50081=CARTESIAN_POINT('Ctrl Pts',(33.6200956257376,58.4460163820148,13.1089687545567));
#50082=CARTESIAN_POINT('Ctrl Pts',(34.9194345180072,56.5189590291238,12.9978308639886));
#50083=CARTESIAN_POINT('Ctrl Pts',(33.9991195898382,54.3822352088321,12.8866929734206));
#50084=CARTESIAN_POINT('Ctrl Pts',(32.4788453194858,54.1263833506296,12.8126010463752));
#50085=CARTESIAN_POINT('Ctrl Pts',(31.8326342444893,54.3482983416318,12.7755550828525));
#50086=CARTESIAN_POINT('Ctrl Pts',(33.8624214427591,54.931476806163,22.0748149723825));
#50087=CARTESIAN_POINT('Ctrl Pts',(33.4101310816148,54.4784392630848,22.0377690088598));
#50088=CARTESIAN_POINT('Ctrl Pts',(32.0254812207533,54.067199902189,21.9636770818144));
#50089=CARTESIAN_POINT('Ctrl Pts',(30.3705294497321,55.4858400606075,21.8525391912464));
#50090=CARTESIAN_POINT('Ctrl Pts',(30.6696757733001,57.6428035756159,21.7414013006784));
#50091=CARTESIAN_POINT('Ctrl Pts',(32.6417207837188,58.5626484614684,21.6302634101103));
#50092=CARTESIAN_POINT('Ctrl Pts',(34.4852499295344,57.4040221256554,21.5191255195423));
#50093=CARTESIAN_POINT('Ctrl Pts',(34.5110566798406,55.2271309148553,21.4079876289742));
#50094=CARTESIAN_POINT('Ctrl Pts',(32.6964205385155,54.0246568103569,21.2968497384062));
#50095=CARTESIAN_POINT('Ctrl Pts',(30.7018484988177,54.8971636496158,21.1857118478381));
#50096=CARTESIAN_POINT('Ctrl Pts',(30.3532198498733,57.0460731790885,21.0745739572701));
#50097=CARTESIAN_POINT('Ctrl Pts',(31.969525977078,58.5044455719579,20.9634360667021));
#50098=CARTESIAN_POINT('Ctrl Pts',(34.0713997025409,57.9374253143107,20.852298176134));
#50099=CARTESIAN_POINT('Ctrl Pts',(34.7349441106375,55.8640078431202,20.741160285566));
#50100=CARTESIAN_POINT('Ctrl Pts',(33.352823499752,54.1820180001326,20.6300223949979));
#50101=CARTESIAN_POINT('Ctrl Pts',(31.1901015335782,54.4309990063087,20.5188845044299));
#50102=CARTESIAN_POINT('Ctrl Pts',(30.2263456554001,56.3830563013939,20.4077466138619));
#50103=CARTESIAN_POINT('Ctrl Pts',(31.3436908009795,58.2514494163732,20.2966087232938));
#50104=CARTESIAN_POINT('Ctrl Pts',(33.5194191611043,58.3260170884914,20.1854708327258));
#50105=CARTESIAN_POINT('Ctrl Pts',(34.7620614565391,56.5385066096463,20.0743329421577));
#50106=CARTESIAN_POINT('Ctrl Pts',(33.9342133200027,54.5250466289289,19.9631950515897));
#50107=CARTESIAN_POINT('Ctrl Pts',(31.7936134302447,54.1285798828619,19.8520571610216));
#50108=CARTESIAN_POINT('Ctrl Pts',(30.2995771969099,55.7119968893621,19.7409192704536));
#50109=CARTESIAN_POINT('Ctrl Pts',(30.8196129006621,57.8259781007111,19.6297813798856));
#50110=CARTESIAN_POINT('Ctrl Pts',(32.8777259778579,58.5355725422314,19.5186434893175));
#50111=CARTESIAN_POINT('Ctrl Pts',(34.5901021815509,57.1912803731282,19.4075055987495));
#50112=CARTESIAN_POINT('Ctrl Pts',(34.3893841562315,55.0235474616526,19.2963677081814));
#50113=CARTESIAN_POINT('Ctrl Pts',(32.4592913850741,54.0165243251615,19.1852298176134));
#50114=CARTESIAN_POINT('Ctrl Pts',(30.5664596711081,55.091950661044,19.0740919270453));
#50115=CARTESIAN_POINT('Ctrl Pts',(30.4434193478743,57.265476547833,18.9629540364773));
#50116=CARTESIAN_POINT('Ctrl Pts',(32.2027906188127,58.5476490919252,18.8518161459092));
#50117=CARTESIAN_POINT('Ctrl Pts',(34.2342010069002,57.7648812228701,18.7406782553413));
#50118=CARTESIAN_POINT('Ctrl Pts',(34.6782775462125,55.6336492484138,18.6295403647732));
#50119=CARTESIAN_POINT('Ctrl Pts',(33.1285519441202,54.1046939645864,18.5184024742052));
#50120=CARTESIAN_POINT('Ctrl Pts',(31.0035056193152,54.5774854822095,18.4072645836371));
#50121=CARTESIAN_POINT('Ctrl Pts',(30.2482175725494,56.6192723633811,18.2961266930691));
#50122=CARTESIAN_POINT('Ctrl Pts',(31.5540115185798,58.3611839203272,18.184988802501));
#50123=CARTESIAN_POINT('Ctrl Pts',(33.7256794498927,58.2088287503543,18.073850911933));
#50124=CARTESIAN_POINT('Ctrl Pts',(34.7754690805686,56.3016592683637,17.9627130213649));
#50125=CARTESIAN_POINT('Ctrl Pts',(33.7424960562255,54.3853293299944,17.8515751307969));
#50126=CARTESIAN_POINT('Ctrl Pts',(31.5722523007556,54.2138774604954,17.7404372402288));
#50127=CARTESIAN_POINT('Ctrl Pts',(30.2511865357786,55.9442355004157,17.6292993496608));
#50128=CARTESIAN_POINT('Ctrl Pts',(30.9884852378827,57.9925871122213,17.5181614590928));
#50129=CARTESIAN_POINT('Ctrl Pts',(33.1092905434961,58.4840528357393,17.4070235685247));
#50130=CARTESIAN_POINT('Ctrl Pts',(34.6724053048228,56.9687885206333,17.2958856779567));
#50131=CARTESIAN_POINT('Ctrl Pts',(34.2470928538934,54.833732778786,17.1847477873887));
#50132=CARTESIAN_POINT('Ctrl Pts',(32.2226465004149,54.0331263438891,17.0736098968206));
#50133=CARTESIAN_POINT('Ctrl Pts',(30.4520649505092,55.2997733652982,16.9624720062526));
#50134=CARTESIAN_POINT('Ctrl Pts',(30.5559815765657,57.4742974595635,16.8513341156845));
#50135=CARTESIAN_POINT('Ctrl Pts',(32.4392803122598,58.5663320624232,16.7401962251165));
#50136=CARTESIAN_POINT('Ctrl Pts',(34.3781564667511,57.5763255173654,16.6290583345484));
#50137=CARTESIAN_POINT('Ctrl Pts',(34.5979347074811,55.4104420425189,16.5179204439804));
#50138=CARTESIAN_POINT('Ctrl Pts',(32.897449518258,54.0511393452008,16.4067825534124));
#50139=CARTESIAN_POINT('Ctrl Pts',(30.833174277585,54.7426025998055,16.2956446628443));
#50140=CARTESIAN_POINT('Ctrl Pts',(30.2945635237363,56.8519276476706,16.1845067722763));
#50141=CARTESIAN_POINT('Ctrl Pts',(31.7746137879455,58.4484253511043,16.0733688817082));
#50142=CARTESIAN_POINT('Ctrl Pts',(33.9186182785215,58.070803256654,15.9622309911402));
#50143=CARTESIAN_POINT('Ctrl Pts',(34.7641453704728,56.0647031498647,15.8510931005722));
#50144=CARTESIAN_POINT('Ctrl Pts',(33.5372745278126,54.2663312092653,15.7399552100041));
#50145=CARTESIAN_POINT('Ctrl Pts',(31.3609745460778,54.3217576668876,15.6288173194361));
#50146=CARTESIAN_POINT('Ctrl Pts',(30.2272374802945,56.1802500577385,15.517679428868));
#50147=CARTESIAN_POINT('Ctrl Pts',(31.1737857225787,58.14070921924,15.4065415383));
#50148=CARTESIAN_POINT('Ctrl Pts',(33.3342329354787,58.4087046487412,15.2954036477319));
#50149=CARTESIAN_POINT('Ctrl Pts',(34.731097277289,56.7389370883627,15.1842657571639));
#50150=CARTESIAN_POINT('Ctrl Pts',(34.0858129876403,54.6597637265374,15.0731278665959));
#50151=CARTESIAN_POINT('Ctrl Pts',(31.9890160684358,54.0742755128362,14.9619899760278));
#50152=CARTESIAN_POINT('Ctrl Pts',(30.3599285720183,55.5183764650323,14.8508520854598));
#50153=CARTESIAN_POINT('Ctrl Pts',(30.6896726531005,57.6702645725732,14.7397141948917));
#50154=CARTESIAN_POINT('Ctrl Pts',(32.6764300265812,58.5602923101728,14.6285763043237));
#50155=CARTESIAN_POINT('Ctrl Pts',(34.5016987131585,57.373807068692,14.5174384137556));
#50156=CARTESIAN_POINT('Ctrl Pts',(34.4947904325672,55.1968125001003,14.4063005231876));
#50157=CARTESIAN_POINT('Ctrl Pts',(32.6620267142976,54.0219359119425,14.2951626326196));
#50158=CARTESIAN_POINT('Ctrl Pts',(30.6809603729032,54.9245561897684,14.1840247420515));
#50159=CARTESIAN_POINT('Ctrl Pts',(30.3648770967316,57.0784927148031,14.0728868514835));
#50160=CARTESIAN_POINT('Ctrl Pts',(32.0031051030322,58.5122270450561,13.9617489609154));
#50161=CARTESIAN_POINT('Ctrl Pts',(34.0961284820971,57.9134377099717,13.8506110703474));
#50162=CARTESIAN_POINT('Ctrl Pts',(34.7282337059124,55.8302197456797,13.7394731797794));
#50163=CARTESIAN_POINT('Ctrl Pts',(33.3207386122115,54.1693334258776,13.6283352892113));
#50164=CARTESIAN_POINT('Ctrl Pts',(31.1621577226746,54.4510723843451,13.5171973986433));
#50165=CARTESIAN_POINT('Ctrl Pts',(30.2278277302022,56.417426573495,13.4060595080752));
#50166=CARTESIAN_POINT('Ctrl Pts',(31.3738258149643,58.2688322792311,13.2949216175072));
#50167=CARTESIAN_POINT('Ctrl Pts',(33.549456509137,58.3101507946959,13.1837837269392));
#50168=CARTESIAN_POINT('Ctrl Pts',(34.7668522624408,56.5046238057481,13.0726458363711));
#50169=CARTESIAN_POINT('Ctrl Pts',(33.9045772301757,54.5026530186945,12.9615079458031));
#50170=CARTESIAN_POINT('Ctrl Pts',(32.4801794448133,54.2629365232493,12.8874160187577));
#50171=CARTESIAN_POINT('Ctrl Pts',(31.8747218362409,54.4708563886884,12.850370055235));
#50172=CARTESIAN_POINT('Ctrl Pts',(33.7707165971401,55.0230304055885,22.149629944765));
#50173=CARTESIAN_POINT('Ctrl Pts',(33.3488699859559,54.6004869054281,22.1125839812423));
#50174=CARTESIAN_POINT('Ctrl Pts',(32.0574211697503,54.2169281438828,22.0384920541969));
#50175=CARTESIAN_POINT('Ctrl Pts',(30.5138645162054,55.5400793642725,21.9273541636289));
#50176=CARTESIAN_POINT('Ctrl Pts',(30.7928752440177,57.5518572561383,21.8162162730608));
#50177=CARTESIAN_POINT('Ctrl Pts',(32.6321815308973,58.4097872083271,21.7050783824928));
#50178=CARTESIAN_POINT('Ctrl Pts',(34.351622380386,57.3291482308462,21.5939404919247));
#50179=CARTESIAN_POINT('Ctrl Pts',(34.3756920734363,55.2987839801705,21.4828026013567));
#50180=CARTESIAN_POINT('Ctrl Pts',(32.6831994348279,54.1772486356277,21.3716647107887));
#50181=CARTESIAN_POINT('Ctrl Pts',(30.8228824172809,54.9910268741142,21.2605268202206));
#50182=CARTESIAN_POINT('Ctrl Pts',(30.4977200287949,56.9952928957376,21.1493889296526));
#50183=CARTESIAN_POINT('Ctrl Pts',(32.0052322841356,58.3555019663445,21.0382510390846));
#50184=CARTESIAN_POINT('Ctrl Pts',(33.965628490635,57.826647949743,20.9271131485165));
#50185=CARTESIAN_POINT('Ctrl Pts',(34.5845095988185,55.8927926016459,20.8159752579485));
#50186=CARTESIAN_POINT('Ctrl Pts',(33.2954197882935,54.324017813885,20.7048373673804));
#50187=CARTESIAN_POINT('Ctrl Pts',(31.2782710477019,54.55623986133,20.5936994768124));
#50188=CARTESIAN_POINT('Ctrl Pts',(30.3793857604063,56.3769038097847,20.4825615862443));
#50189=CARTESIAN_POINT('Ctrl Pts',(31.4215221923948,58.1195350299587,20.3714236956763));
#50190=CARTESIAN_POINT('Ctrl Pts',(33.4508018640946,58.1890835379289,20.2602858051083));
#50191=CARTESIAN_POINT('Ctrl Pts',(34.6098016710262,56.5218907283163,20.1491479145402));
#50192=CARTESIAN_POINT('Ctrl Pts',(33.8376761495152,54.6439571206407,20.0380100239722));
#50193=CARTESIAN_POINT('Ctrl Pts',(31.8411604441815,54.2741766264192,19.9268721334041));
#50194=CARTESIAN_POINT('Ctrl Pts',(30.4476880729728,55.7510135340056,19.8157342428361));
#50195=CARTESIAN_POINT('Ctrl Pts',(30.9327200749098,57.7227022692206,19.7045963522681));
#50196=CARTESIAN_POINT('Ctrl Pts',(32.8523011706738,58.3845337743473,19.5934584617));
#50197=CARTESIAN_POINT('Ctrl Pts',(34.44941700744,57.1307261660161,19.482320571132));
#50198=CARTESIAN_POINT('Ctrl Pts',(34.2622093504597,55.1089037678012,19.3711826805639));
#50199=CARTESIAN_POINT('Ctrl Pts',(32.4620314896629,54.1696635495527,19.2600447899959));
#50200=CARTESIAN_POINT('Ctrl Pts',(30.6966066372334,55.1727027348726,19.1489068994278));
#50201=CARTESIAN_POINT('Ctrl Pts',(30.5818481814842,57.1999281821345,19.0377690088598));
#50202=CARTESIAN_POINT('Ctrl Pts',(32.2227958386095,58.3957974491916,18.9266311182918));
#50203=CARTESIAN_POINT('Ctrl Pts',(34.1174716083317,57.6657178338107,18.8154932277237));
#50204=CARTESIAN_POINT('Ctrl Pts',(34.5316572715886,55.6779394876238,18.7043553371557));
#50205=CARTESIAN_POINT('Ctrl Pts',(33.0862439935918,54.2518984738315,18.5932174465876));
#50206=CARTESIAN_POINT('Ctrl Pts',(31.1042349398054,54.692866304765,18.4820795560196));
#50207=CARTESIAN_POINT('Ctrl Pts',(30.3997854746655,56.5972201238544,18.3709416654515));
#50208=CARTESIAN_POINT('Ctrl Pts',(31.617686182618,58.2218832836466,18.2598037748835));
#50209=CARTESIAN_POINT('Ctrl Pts',(33.6431787337389,58.0797831690501,18.1486658843155));
#50210=CARTESIAN_POINT('Ctrl Pts',(34.6223068253404,56.3009856264801,18.0375279937474));
#50211=CARTESIAN_POINT('Ctrl Pts',(33.6588634111112,54.5136442195871,17.9263901031794));
#50212=CARTESIAN_POINT('Ctrl Pts',(31.6346991742871,54.3537328079304,17.8152522126114));
#50213=CARTESIAN_POINT('Ctrl Pts',(30.4025545964168,55.9676201201181,17.7041143220433));
#50214=CARTESIAN_POINT('Ctrl Pts',(31.0902255830949,57.878096796578,17.5929764314753));
#50215=CARTESIAN_POINT('Ctrl Pts',(33.0682790814955,58.336481869067,17.4818385409072));
#50216=CARTESIAN_POINT('Ctrl Pts',(34.5261802918802,56.9232102822958,17.3707006503392));
#50217=CARTESIAN_POINT('Ctrl Pts',(34.1294957026596,54.9318655472259,17.2595627597711));
#50218=CARTESIAN_POINT('Ctrl Pts',(32.2413152170565,54.1851480832521,17.1484248692031));
#50219=CARTESIAN_POINT('Ctrl Pts',(30.5899118469666,55.3665368535015,17.0372869786351));
#50220=CARTESIAN_POINT('Ctrl Pts',(30.6868338252212,57.3946933187051,16.926149088067));
#50221=CARTESIAN_POINT('Ctrl Pts',(32.4433673659537,58.4132228654032,16.815011197499));
#50222=CARTESIAN_POINT('Ctrl Pts',(34.2517373988869,57.4898538485926,16.7038733069309));
#50223=CARTESIAN_POINT('Ctrl Pts',(34.4567223245648,55.4697564010764,16.5927354163629));
#50224=CARTESIAN_POINT('Ctrl Pts',(32.87069711583,54.2019486260304,16.4815975257949));
#50225=CARTESIAN_POINT('Ctrl Pts',(30.9453686329808,54.8468693578704,16.3704596352268));
#50226=CARTESIAN_POINT('Ctrl Pts',(30.4430118710911,56.8142153368483,16.2593217446588));
#50227=CARTESIAN_POINT('Ctrl Pts',(31.8234396714077,58.3032524771776,16.1481838540907));
#50228=CARTESIAN_POINT('Ctrl Pts',(33.8231308132328,57.9510481974995,16.0370459635227));
#50229=CARTESIAN_POINT('Ctrl Pts',(34.611745316318,56.0799790692429,15.9259080729546));
#50230=CARTESIAN_POINT('Ctrl Pts',(33.4674553826844,54.4026558849256,15.8147701823866));
#50231=CARTESIAN_POINT('Ctrl Pts',(31.4376425653338,54.4543515771768,15.7036322918186));
#50232=CARTESIAN_POINT('Ctrl Pts',(30.3802175563979,56.1877484928406,15.5924944012505));
#50233=CARTESIAN_POINT('Ctrl Pts',(31.2630534570341,58.0162487764902,15.4813565106825));
#50234=CARTESIAN_POINT('Ctrl Pts',(33.278080558426,58.2662053828213,15.3702186201144));
#50235=CARTESIAN_POINT('Ctrl Pts',(34.5809216965521,56.7088301935099,15.2590807295464));
#50236=CARTESIAN_POINT('Ctrl Pts',(33.9790716147817,54.7696063848677,15.1479428389783));
#50237=CARTESIAN_POINT('Ctrl Pts',(32.0234104937489,54.2235274938358,15.0368049484103));
#50238=CARTESIAN_POINT('Ctrl Pts',(30.5039771855803,55.5704257371467,14.9256670578423));
#50239=CARTESIAN_POINT('Ctrl Pts',(30.8115261300475,57.577469848184,14.8145291672742));
#50240=CARTESIAN_POINT('Ctrl Pts',(32.6645544880419,58.4075896500218,14.7033912767062));
#50241=CARTESIAN_POINT('Ctrl Pts',(34.3669639932659,57.3009669550956,14.5922533861381));
#50242=CARTESIAN_POINT('Ctrl Pts',(34.3605207103508,55.2705063036608,14.4811154955701));
#50243=CARTESIAN_POINT('Ctrl Pts',(32.651120665439,54.1747108814015,14.3699776050021));
#50244=CARTESIAN_POINT('Ctrl Pts',(30.803400275082,55.0165756171955,14.258839714434));
#50245=CARTESIAN_POINT('Ctrl Pts',(30.5085926241571,57.0255302663568,14.147701823866));
#50246=CARTESIAN_POINT('Ctrl Pts',(32.0365511927554,58.3627596670131,14.0365639332979));
#50247=CARTESIAN_POINT('Ctrl Pts',(33.9886927713508,57.8042749556,13.9254260427299));
#50248=CARTESIAN_POINT('Ctrl Pts',(34.5782508727078,55.86127878745,13.8142881521619));
#50249=CARTESIAN_POINT('Ctrl Pts',(33.2654945406164,54.312187040728,13.7031502615938));
#50250=CARTESIAN_POINT('Ctrl Pts',(31.2522081400082,54.574962096485,13.5920123710258));
#50251=CARTESIAN_POINT('Ctrl Pts',(30.3807680764725,56.4089606123543,13.4808744804577));
#50252=CARTESIAN_POINT('Ctrl Pts',(31.4496288128749,58.135747849022,13.3697365898897));
#50253=CARTESIAN_POINT('Ctrl Pts',(33.4788173925363,58.1742852073771,13.2585986993216));
#50254=CARTESIAN_POINT('Ctrl Pts',(34.6142700068744,56.4902885823724,13.1474608087536));
#50255=CARTESIAN_POINT('Ctrl Pts',(33.8100348705131,54.6230708285569,13.0363229181856));
#50256=CARTESIAN_POINT('Ctrl Pts',(32.4815135701408,54.3994896958689,12.9622309911402));
#50257=CARTESIAN_POINT('Ctrl Pts',(31.9168094279925,54.593414435745,12.9251850276175));
#50258=CARTESIAN_POINT('Ctrl Pts',(33.6790117515211,55.1145840050141,22.2244449171475));
#50259=CARTESIAN_POINT('Ctrl Pts',(33.2876088902971,54.7225345477714,22.1873989536248));
#50260=CARTESIAN_POINT('Ctrl Pts',(32.0893611187473,54.3666563855765,22.1133070265794));
#50261=CARTESIAN_POINT('Ctrl Pts',(30.6571995826787,55.5943186679374,22.0021691360114));
#50262=CARTESIAN_POINT('Ctrl Pts',(30.9160747147354,57.4609109366607,21.8910312454433));
#50263=CARTESIAN_POINT('Ctrl Pts',(32.6226422780758,58.2569259551857,21.7798933548753));
#50264=CARTESIAN_POINT('Ctrl Pts',(34.2179948312376,57.2542743360371,21.6687554643072));
#50265=CARTESIAN_POINT('Ctrl Pts',(34.2403274670321,55.3704370454857,21.5576175737392));
#50266=CARTESIAN_POINT('Ctrl Pts',(32.6699783311403,54.3298404608986,21.4464796831711));
#50267=CARTESIAN_POINT('Ctrl Pts',(30.9439163357442,55.0848900986124,21.3353417926032));
#50268=CARTESIAN_POINT('Ctrl Pts',(30.6422202077165,56.9445126123869,21.2242039020351));
#50269=CARTESIAN_POINT('Ctrl Pts',(32.0409385911931,58.206558360731,21.1130660114671));
#50270=CARTESIAN_POINT('Ctrl Pts',(33.8598572787291,57.7158705851754,21.001928120899));
#50271=CARTESIAN_POINT('Ctrl Pts',(34.4340750869996,55.9215773601716,20.890790230331));
#50272=CARTESIAN_POINT('Ctrl Pts',(33.238016076835,54.4660176276373,20.7796523397629));
#50273=CARTESIAN_POINT('Ctrl Pts',(31.3664405618256,54.6814807163513,20.6685144491949));
#50274=CARTESIAN_POINT('Ctrl Pts',(30.5324258654125,56.3707513181755,20.5573765586268));
#50275=CARTESIAN_POINT('Ctrl Pts',(31.4993535838102,57.9876206435441,20.4462386680588));
#50276=CARTESIAN_POINT('Ctrl Pts',(33.3821845670849,58.0521499873667,20.3351007774907));
#50277=CARTESIAN_POINT('Ctrl Pts',(34.4575418855134,56.5052748469861,20.2239628869227));
#50278=CARTESIAN_POINT('Ctrl Pts',(33.7411389790275,54.7628676123527,20.1128249963547));
#50279=CARTESIAN_POINT('Ctrl Pts',(31.8887074581184,54.4197733699765,20.0016871057866));
#50280=CARTESIAN_POINT('Ctrl Pts',(30.5957989490357,55.7900301786492,19.8905492152186));
#50281=CARTESIAN_POINT('Ctrl Pts',(31.0458272491576,57.61942643773,19.7794113246505));
#50282=CARTESIAN_POINT('Ctrl Pts',(32.8268763634895,58.2334950064634,19.6682734340825));
#50283=CARTESIAN_POINT('Ctrl Pts',(34.308731833329,57.0701719589039,19.5571355435145));
#50284=CARTESIAN_POINT('Ctrl Pts',(34.1350345446879,55.1942600739497,19.4459976529464));
#50285=CARTESIAN_POINT('Ctrl Pts',(32.4647715942516,54.3228027739439,19.3348597623784));
#50286=CARTESIAN_POINT('Ctrl Pts',(30.8267536033587,55.2534548087013,19.2237218718103));
#50287=CARTESIAN_POINT('Ctrl Pts',(30.7202770150941,57.1343798164359,19.1125839812423));
#50288=CARTESIAN_POINT('Ctrl Pts',(32.2428010584064,58.2439458064581,19.0014460906742));
#50289=CARTESIAN_POINT('Ctrl Pts',(34.0007422097631,57.5665544447512,18.8903082001062));
#50290=CARTESIAN_POINT('Ctrl Pts',(34.3850369969648,55.7222297268338,18.7791703095382));
#50291=CARTESIAN_POINT('Ctrl Pts',(33.0439360430634,54.3991029830766,18.6680324189701));
#50292=CARTESIAN_POINT('Ctrl Pts',(31.2049642602956,54.8082471273204,18.5568945284021));
#50293=CARTESIAN_POINT('Ctrl Pts',(30.5513533767816,56.5751678843277,18.445756637834));
#50294=CARTESIAN_POINT('Ctrl Pts',(31.681360846656,58.0825826469659,18.334618747266));
#50295=CARTESIAN_POINT('Ctrl Pts',(33.5606780175853,57.9507375877459,18.223480856698));
#50296=CARTESIAN_POINT('Ctrl Pts',(34.469144570112,56.3003119845966,18.1123429661299));
#50297=CARTESIAN_POINT('Ctrl Pts',(33.5752307659969,54.6419591091798,18.0012050755619));
#50298=CARTESIAN_POINT('Ctrl Pts',(31.6971460478186,54.4935881553653,17.8900671849938));
#50299=CARTESIAN_POINT('Ctrl Pts',(30.5539226570551,55.9910047398206,17.7789292944258));
#50300=CARTESIAN_POINT('Ctrl Pts',(31.1919659283071,57.7636064809346,17.6677914038578));
#50301=CARTESIAN_POINT('Ctrl Pts',(33.027267619495,58.1889109023948,17.5566535132897));
#50302=CARTESIAN_POINT('Ctrl Pts',(34.3799552789376,56.8776320439583,17.4455156227217));
#50303=CARTESIAN_POINT('Ctrl Pts',(34.0118985514257,55.0299983156659,17.3343777321536));
#50304=CARTESIAN_POINT('Ctrl Pts',(32.2599839336981,54.3371698226151,17.2232398415856));
#50305=CARTESIAN_POINT('Ctrl Pts',(30.7277587434239,55.4333003417049,17.1121019510176));
#50306=CARTESIAN_POINT('Ctrl Pts',(30.8176860738768,57.3150891778467,17.0009640604495));
#50307=CARTESIAN_POINT('Ctrl Pts',(32.4474544196475,58.2601136683833,16.8898261698815));
#50308=CARTESIAN_POINT('Ctrl Pts',(34.1253183310228,57.4033821798196,16.7786882793134));
#50309=CARTESIAN_POINT('Ctrl Pts',(34.3155099416484,55.5290707596339,16.6675503887454));
#50310=CARTESIAN_POINT('Ctrl Pts',(32.843944713402,54.3527579068599,16.5564124981773));
#50311=CARTESIAN_POINT('Ctrl Pts',(31.0575629883768,54.9511361159353,16.4452746076093));
#50312=CARTESIAN_POINT('Ctrl Pts',(30.5914602184459,56.776503026026,16.3341367170413));
#50313=CARTESIAN_POINT('Ctrl Pts',(31.87226555487,58.158079603251,16.2229988264732));
#50314=CARTESIAN_POINT('Ctrl Pts',(33.727643347944,57.8312931383451,16.1118609359052));
#50315=CARTESIAN_POINT('Ctrl Pts',(34.4593452621631,56.095254988621,16.0007230453371));
#50316=CARTESIAN_POINT('Ctrl Pts',(33.3976362375564,54.5389805605859,15.8895851547691));
#50317=CARTESIAN_POINT('Ctrl Pts',(31.5143105845896,54.5869454874661,15.7784472642011));
#50318=CARTESIAN_POINT('Ctrl Pts',(30.5331976325014,56.1952469279427,15.667309373633));
#50319=CARTESIAN_POINT('Ctrl Pts',(31.3523211914896,57.8917883337404,15.556171483065));
#50320=CARTESIAN_POINT('Ctrl Pts',(33.2219281813735,58.1237061169015,15.4450335924969));
#50321=CARTESIAN_POINT('Ctrl Pts',(34.4307461158152,56.6787232986569,15.3338957019289));
#50322=CARTESIAN_POINT('Ctrl Pts',(33.872330241923,54.879449043198,15.2227578113608));
#50323=CARTESIAN_POINT('Ctrl Pts',(32.0578049190619,54.3727794748353,15.1116199207928));
#50324=CARTESIAN_POINT('Ctrl Pts',(30.6480257991425,55.6224750092611,15.0004820302248));
#50325=CARTESIAN_POINT('Ctrl Pts',(30.9333796069945,57.4846751237948,14.8893441396567));
#50326=CARTESIAN_POINT('Ctrl Pts',(32.6526789495027,58.254886989871,14.7782062490887));
#50327=CARTESIAN_POINT('Ctrl Pts',(34.2322292733731,57.2281268414992,14.6670683585206));
#50328=CARTESIAN_POINT('Ctrl Pts',(34.2262509881345,55.3442001072214,14.5559304679526));
#50329=CARTESIAN_POINT('Ctrl Pts',(32.6402146165803,54.3274858508605,14.4447925773845));
#50330=CARTESIAN_POINT('Ctrl Pts',(30.9258401772609,55.1085950446227,14.3336546868165));
#50331=CARTESIAN_POINT('Ctrl Pts',(30.6523081515825,56.9725678179105,14.2225167962485));
#50332=CARTESIAN_POINT('Ctrl Pts',(32.0699972824786,58.21329228897,14.1113789056804));
#50333=CARTESIAN_POINT('Ctrl Pts',(33.8812570606045,57.6951122012284,14.0002410151124));
#50334=CARTESIAN_POINT('Ctrl Pts',(34.4282680395032,55.8923378292205,13.8891031245443));
#50335=CARTESIAN_POINT('Ctrl Pts',(33.2102504690214,54.4550406555783,13.7779652339763));
#50336=CARTESIAN_POINT('Ctrl Pts',(31.3422585573418,54.6988518086249,13.6668273434082));
#50337=CARTESIAN_POINT('Ctrl Pts',(30.5337084227428,56.4004946512136,13.5556894528402));
#50338=CARTESIAN_POINT('Ctrl Pts',(31.5254318107855,58.0026634188128,13.4445515622722));
#50339=CARTESIAN_POINT('Ctrl Pts',(33.4081782759357,58.0384196200583,13.3334136717041));
#50340=CARTESIAN_POINT('Ctrl Pts',(34.4616877513079,56.4759533589966,13.2222757811361));
#50341=CARTESIAN_POINT('Ctrl Pts',(33.7154925108507,54.7434886384194,13.111137890568));
#50342=CARTESIAN_POINT('Ctrl Pts',(32.4828476954683,54.5360428684886,13.0370459635227));
#50343=CARTESIAN_POINT('Ctrl Pts',(31.9588970197441,54.7159724828016,13.));
#50344=CARTESIAN_POINT('Ctrl Pts',(31.667262219952,54.851191363199,21.3785196366098));
#50345=CARTESIAN_POINT('Ctrl Pts',(31.479741769716,54.9581664087852,21.3641270219409));
#50346=CARTESIAN_POINT('Ctrl Pts',(31.3126103376672,55.0996825231224,21.349734407272));
#50347=CARTESIAN_POINT('Ctrl Pts',(31.1813106469723,55.2689855779558,21.3353417926031));
#50348=CARTESIAN_POINT('Ctrl Pts',(30.843350959735,55.7047642698706,21.2982958290805));
#50349=CARTESIAN_POINT('Ctrl Pts',(30.7427855837258,56.3246384411287,21.2612498655578));
#50350=CARTESIAN_POINT('Ctrl Pts',(30.9256226263006,56.8449164848152,21.2242039020351));
#50351=CARTESIAN_POINT('Ctrl Pts',(31.1084596688754,57.3651945285016,21.1871579385124));
#50352=CARTESIAN_POINT('Ctrl Pts',(31.5746991300343,57.7858764446163,21.1501119749897));
#50353=CARTESIAN_POINT('Ctrl Pts',(32.110971975203,57.9144361067477,21.1130660114671));
#50354=CARTESIAN_POINT('Ctrl Pts',(32.6472448203718,58.0429957688791,21.0760200479444));
#50355=CARTESIAN_POINT('Ctrl Pts',(33.2535510495504,57.8794331770273,21.0389740844217));
#50356=CARTESIAN_POINT('Ctrl Pts',(33.6524071321848,57.4986030102674,21.001928120899));
#50357=CARTESIAN_POINT('Ctrl Pts',(34.0512632148192,57.1177728435075,20.9648821573763));
#50358=CARTESIAN_POINT('Ctrl Pts',(34.2426691509094,56.5196751018395,20.9278361938536));
#50359=CARTESIAN_POINT('Ctrl Pts',(34.1390289505937,55.9780329422498,20.890790230331));
#50360=CARTESIAN_POINT('Ctrl Pts',(34.035388750278,55.4363907826601,20.8537442668083));
#50361=CARTESIAN_POINT('Ctrl Pts',(33.6367024135565,54.9512042051487,20.8166983032856));
#50362=CARTESIAN_POINT('Ctrl Pts',(33.1254299926942,54.7445214311787,20.7796523397629));
#50363=CARTESIAN_POINT('Ctrl Pts',(32.6601848660756,54.5564452717343,20.7459414387119));
#50364=CARTESIAN_POINT('Ctrl Pts',(32.1017123235945,54.5989854456511,20.7122305376608));
#50365=CARTESIAN_POINT('Ctrl Pts',(31.6651488727496,54.8473747039336,20.6785196366098));
#50366=CARTESIAN_POINT('Ctrl Pts',(33.9541262883781,54.8399232067375,22.));
#50367=CARTESIAN_POINT('Ctrl Pts',(33.89777705666,54.7931706099734,22.));
#50368=CARTESIAN_POINT('Ctrl Pts',(33.8389107618346,54.7498380989977,22.));
#50369=CARTESIAN_POINT('Ctrl Pts',(33.7778765460594,54.7099422292599,22.));
#50370=CARTESIAN_POINT('Ctrl Pts',(33.715142612768,54.6689353153684,22.));
#50371=CARTESIAN_POINT('Ctrl Pts',(33.650117347963,54.6315587953775,22.));
#50372=CARTESIAN_POINT('Ctrl Pts',(33.5831568242514,54.5978800039331,22.));
#50373=CARTESIAN_POINT('Ctrl Pts',(33.5265763653167,54.5694220204725,22.));
#50374=CARTESIAN_POINT('Ctrl Pts',(33.4686133977542,54.5436050120003,22.));
#50375=CARTESIAN_POINT('Ctrl Pts',(33.4094785141808,54.5204983074666,22.));
#50376=CARTESIAN_POINT('Ctrl Pts',(33.3832054797345,54.5102322308723,22.));
#50377=CARTESIAN_POINT('Ctrl Pts',(33.3567011132798,54.5005015028803,22.));
#50378=CARTESIAN_POINT('Ctrl Pts',(33.3299840335543,54.4913139103876,22.));
#50379=CARTESIAN_POINT('Ctrl Pts',(33.3153052179449,54.4862660916334,22.));
#50380=CARTESIAN_POINT('Ctrl Pts',(33.3005621960478,54.4813822417937,22.));
#50381=CARTESIAN_POINT('Ctrl Pts',(33.2857580867441,54.4766637893069,22.));
#50382=CARTESIAN_POINT('Ctrl Pts',(33.2721048858946,54.4723121611084,22.));
#50383=CARTESIAN_POINT('Ctrl Pts',(33.2583976935292,54.4681007280097,22.));
#50384=CARTESIAN_POINT('Ctrl Pts',(33.2446602942607,54.4640366443286,22.));
#50385=CARTESIAN_POINT('Ctrl Pts',(33.1744615986776,54.4432690035566,22.));
#50386=CARTESIAN_POINT('Ctrl Pts',(33.1033546242792,54.4263051056874,22.));
#50387=CARTESIAN_POINT('Ctrl Pts',(33.0316734669243,54.4132045353738,22.));
#50388=CARTESIAN_POINT('Ctrl Pts',(32.9605481884268,54.4002055584262,22.));
#50389=CARTESIAN_POINT('Ctrl Pts',(32.8888565785142,54.3910102235798,22.));
#50390=CARTESIAN_POINT('Ctrl Pts',(32.8169264247183,54.385727650947,22.));
#50391=CARTESIAN_POINT('Ctrl Pts',(32.7571464345771,54.3813373900725,22.));
#50392=CARTESIAN_POINT('Ctrl Pts',(32.6972014393332,54.3796505588106,22.));
#50393=CARTESIAN_POINT('Ctrl Pts',(32.6372877973872,54.3807569468898,22.));
#50394=CARTESIAN_POINT('Ctrl Pts',(32.6122799917386,54.3812187505318,22.));
#50395=CARTESIAN_POINT('Ctrl Pts',(32.5872777755307,54.3821674889425,22.));
#50396=CARTESIAN_POINT('Ctrl Pts',(32.5622960765392,54.3836109807431,22.));
#50397=CARTESIAN_POINT('Ctrl Pts',(32.5507331510584,54.3842791093651,22.));
#50398=CARTESIAN_POINT('Ctrl Pts',(32.5391746273353,54.3850532424606,22.));
#50399=CARTESIAN_POINT('Ctrl Pts',(32.527622019984,54.3859342108815,22.));
#50400=CARTESIAN_POINT('Ctrl Pts',(32.515571956249,54.3868531138873,22.));
#50401=CARTESIAN_POINT('Ctrl Pts',(32.5035366027722,54.3878876490277,22.));
#50402=CARTESIAN_POINT('Ctrl Pts',(32.4915220458572,54.3890378132825,22.));
#50403=CARTESIAN_POINT('Ctrl Pts',(32.4230954842055,54.3955883490906,22.));
#50404=CARTESIAN_POINT('Ctrl Pts',(32.3552950943228,54.4058891778563,22.));
#50405=CARTESIAN_POINT('Ctrl Pts',(32.2884097213901,54.420031548574,22.));
#50406=CARTESIAN_POINT('Ctrl Pts',(32.2277876728082,54.4328495900548,22.));
#50407=CARTESIAN_POINT('Ctrl Pts',(32.1679169373136,54.448823971587,22.));
#50408=CARTESIAN_POINT('Ctrl Pts',(32.1090267714104,54.4680568733301,22.));
#50409=CARTESIAN_POINT('Ctrl Pts',(32.0393564154629,54.4908104704681,22.));
#50410=CARTESIAN_POINT('Ctrl Pts',(31.9710568700512,54.5181250014914,22.));
#50411=CARTESIAN_POINT('Ctrl Pts',(31.9044569620169,54.5497238479896,22.));
#50412=CARTESIAN_POINT('Ctrl Pts',(31.8897939177248,54.5566808438692,22.));
#50413=CARTESIAN_POINT('Ctrl Pts',(31.875213443077,54.5638456669608,22.));
#50414=CARTESIAN_POINT('Ctrl Pts',(31.8607193748282,54.571215603018,22.));
#50415=CARTESIAN_POINT('Ctrl Pts',(31.8457643400607,54.5788199310837,22.));
#50416=CARTESIAN_POINT('Ctrl Pts',(31.8308959671421,54.5866456914889,22.));
#50417=CARTESIAN_POINT('Ctrl Pts',(31.8161482776472,54.594673337877,22.));
#50418=CARTESIAN_POINT('Ctrl Pts',(31.7559125282455,54.6274616126968,22.));
#50419=CARTESIAN_POINT('Ctrl Pts',(31.6976088413824,54.6636511833295,22.));
#50420=CARTESIAN_POINT('Ctrl Pts',(31.6414698545344,54.702968470454,22.));
#50421=CARTESIAN_POINT('Ctrl Pts',(31.5853421058314,54.7422778868741,22.));
#50422=CARTESIAN_POINT('Ctrl Pts',(31.5313774894568,54.7847146962881,22.));
#50423=CARTESIAN_POINT('Ctrl Pts',(31.4798463246642,54.8300409282343,22.));
#50424=CARTESIAN_POINT('Ctrl Pts',(31.4425466815923,54.8628492740225,22.));
#50425=CARTESIAN_POINT('Ctrl Pts',(31.4065227401674,54.8971722385251,22.));
#50426=CARTESIAN_POINT('Ctrl Pts',(31.3718924923334,54.9329270614585,22.));
#50427=CARTESIAN_POINT('Ctrl Pts',(31.3459157227865,54.9597473949422,22.));
#50428=CARTESIAN_POINT('Ctrl Pts',(31.3207234116099,54.987373540647,22.));
#50429=CARTESIAN_POINT('Ctrl Pts',(31.2963709389138,55.0157718708887,22.));
#50430=CARTESIAN_POINT('Ctrl Pts',(31.2882802398916,55.0252067379589,22.));
#50431=CARTESIAN_POINT('Ctrl Pts',(31.2802886269196,55.0347194487898,22.));
#50432=CARTESIAN_POINT('Ctrl Pts',(31.2723979365543,55.0443082314195,22.));
#50433=CARTESIAN_POINT('Ctrl Pts',(31.2305359635494,55.0951789842957,22.));
#50434=CARTESIAN_POINT('Ctrl Pts',(31.1915084684126,55.1481921233583,22.));
#50435=CARTESIAN_POINT('Ctrl Pts',(31.1555797357851,55.2031373176633,22.));
#50436=CARTESIAN_POINT('Ctrl Pts',(31.130298191857,55.2417999489858,22.));
#50437=CARTESIAN_POINT('Ctrl Pts',(31.1065518383838,55.2814196840771,22.));
#50438=CARTESIAN_POINT('Ctrl Pts',(31.0844478042592,55.3219265813484,22.));
#50439=CARTESIAN_POINT('Ctrl Pts',(31.0773529644809,55.3349282779815,22.));
#50440=CARTESIAN_POINT('Ctrl Pts',(31.0704265009656,55.3480232015208,22.));
#50441=CARTESIAN_POINT('Ctrl Pts',(31.0636752117837,55.3612032672917,22.));
#50442=CARTESIAN_POINT('Ctrl Pts',(31.0349131819519,55.417353349843,22.));
#50443=CARTESIAN_POINT('Ctrl Pts',(31.0093835905525,55.4749346571281,22.));
#50444=CARTESIAN_POINT('Ctrl Pts',(30.9873422740719,55.5337599434685,22.));
#50445=CARTESIAN_POINT('Ctrl Pts',(30.9670232664277,55.5879886209558,22.));
#50446=CARTESIAN_POINT('Ctrl Pts',(30.9496688942649,55.6432750194153,22.));
#50447=CARTESIAN_POINT('Ctrl Pts',(30.9355188507018,55.6994745658575,22.));
#50448=CARTESIAN_POINT('Ctrl Pts',(30.9328706183904,55.7099925161458,22.));
#50449=CARTESIAN_POINT('Ctrl Pts',(30.9303347375364,55.7205424451195,22.));
#50450=CARTESIAN_POINT('Ctrl Pts',(30.9279109916838,55.7311226632894,22.));
#50451=CARTESIAN_POINT('Origin',(32.5,56.2916512459885,17.));
#50452=CARTESIAN_POINT('Origin',(32.5,-56.2916512459885,12.));
#50453=CARTESIAN_POINT('Origin',(-32.5,-56.2916512459885,12.));
#50454=CARTESIAN_POINT('Origin',(-65.,8.88178419700125E-15,12.));
#50455=CARTESIAN_POINT('Origin',(-32.5,56.2916512459885,12.));
#50456=CARTESIAN_POINT('Origin',(32.5,56.2916512459885,12.));
#50457=CARTESIAN_POINT('Origin',(65.,0.,7.));
#50458=CARTESIAN_POINT('Ctrl Pts',(66.6351293272515,-0.319230454628274,
7.));
#50459=CARTESIAN_POINT('Ctrl Pts',(66.6302897730466,-0.381554702499113,
7.));
#50460=CARTESIAN_POINT('Ctrl Pts',(66.6216732730344,-0.44339471174141,7.));
#50461=CARTESIAN_POINT('Ctrl Pts',(66.6095363361247,-0.504531338372354,
7.));
#50462=CARTESIAN_POINT('Ctrl Pts',(66.6018369189696,-0.543315126686597,
7.));
#50463=CARTESIAN_POINT('Ctrl Pts',(66.5927196857359,-0.581816142971907,
7.));
#50464=CARTESIAN_POINT('Ctrl Pts',(66.5822397317414,-0.619979888881646,
7.));
#50465=CARTESIAN_POINT('Ctrl Pts',(66.575055633828,-0.646141462444073,7.));
#50466=CARTESIAN_POINT('Ctrl Pts',(66.5672309976242,-0.672144564830664,
7.));
#50467=CARTESIAN_POINT('Ctrl Pts',(66.5587815172138,-0.69797162244664,7.));
#50468=CARTESIAN_POINT('Ctrl Pts',(66.5543304405506,-0.711576981338436,
7.));
#50469=CARTESIAN_POINT('Ctrl Pts',(66.5497059365671,-0.725133118782638,
7.));
#50470=CARTESIAN_POINT('Ctrl Pts',(66.5449151805486,-0.738624321418645,
7.));
#50471=CARTESIAN_POINT('Ctrl Pts',(66.5228385616516,-0.800794078740785,
7.));
#50472=CARTESIAN_POINT('Ctrl Pts',(66.4972129908327,-0.861656594198672,
7.));
#50473=CARTESIAN_POINT('Ctrl Pts',(66.4682928032974,-0.920967263964251,
7.));
#50474=CARTESIAN_POINT('Ctrl Pts',(66.4474370017557,-0.963739170488886,
7.));
#50475=CARTESIAN_POINT('Ctrl Pts',(66.4248666023715,-1.00570421528168,7.));
#50476=CARTESIAN_POINT('Ctrl Pts',(66.4006603561211,-1.04676903354864,7.));
#50477=CARTESIAN_POINT('Ctrl Pts',(66.3939846942071,-1.05809399655503,7.));
#50478=CARTESIAN_POINT('Ctrl Pts',(66.3871845393328,-1.06935047365006,7.));
#50479=CARTESIAN_POINT('Ctrl Pts',(66.3802613712345,-1.08053645690262,7.));
#50480=CARTESIAN_POINT('Ctrl Pts',(66.3732910164015,-1.09179868126564,7.));
#50481=CARTESIAN_POINT('Ctrl Pts',(66.366200339596,-1.10298231859776,7.));
#50482=CARTESIAN_POINT('Ctrl Pts',(66.3589938162138,-1.11408178950634,7.));
#50483=CARTESIAN_POINT('Ctrl Pts',(66.3220437716818,-1.17099216398268,7.));
#50484=CARTESIAN_POINT('Ctrl Pts',(66.2820328735632,-1.22572189932463,7.));
#50485=CARTESIAN_POINT('Ctrl Pts',(66.2392195753837,-1.27802354449959,7.));
#50486=CARTESIAN_POINT('Ctrl Pts',(66.1957886599383,-1.33107968419999,7.));
#50487=CARTESIAN_POINT('Ctrl Pts',(66.1494735385541,-1.38163817167118,7.));
#50488=CARTESIAN_POINT('Ctrl Pts',(66.1004928624473,-1.4294273768642,7.));
#50489=CARTESIAN_POINT('Ctrl Pts',(66.0701495070252,-1.45903262027388,7.));
#50490=CARTESIAN_POINT('Ctrl Pts',(66.0387821884129,-1.48757476196839,7.));
#50491=CARTESIAN_POINT('Ctrl Pts',(66.0064342586826,-1.51498409802404,7.));
#50492=CARTESIAN_POINT('Ctrl Pts',(65.9799267074793,-1.53744471250548,7.));
#50493=CARTESIAN_POINT('Ctrl Pts',(65.9527605447791,-1.55914459463409,7.));
#50494=CARTESIAN_POINT('Ctrl Pts',(65.9249567188516,-1.58004262988225,7.));
#50495=CARTESIAN_POINT('Ctrl Pts',(65.9136073282091,-1.58857310933178,7.));
#50496=CARTESIAN_POINT('Ctrl Pts',(65.9021495271597,-1.59697130994429,7.));
#50497=CARTESIAN_POINT('Ctrl Pts',(65.8906044505495,-1.60522061987257,7.));
#50498=CARTESIAN_POINT('Ctrl Pts',(65.8332561981394,-1.64619769814996,7.));
#50499=CARTESIAN_POINT('Ctrl Pts',(65.7736595595987,-1.68357914693718,7.));
#50500=CARTESIAN_POINT('Ctrl Pts',(65.7120551181349,-1.71709301891337,7.));
#50501=CARTESIAN_POINT('Ctrl Pts',(65.7052145748788,-1.7208143916827,7.));
#50502=CARTESIAN_POINT('Ctrl Pts',(65.6983492298898,-1.72448805150504,7.));
#50503=CARTESIAN_POINT('Ctrl Pts',(65.6914593790745,-1.72811360467692,7.));
#50504=CARTESIAN_POINT('Ctrl Pts',(65.6317930119872,-1.75951103144934,7.));
#50505=CARTESIAN_POINT('Ctrl Pts',(65.5702916681948,-1.78730397727615,7.));
#50506=CARTESIAN_POINT('Ctrl Pts',(65.5072864772923,-1.81157490046553,7.));
#50507=CARTESIAN_POINT('Ctrl Pts',(65.4395015551736,-1.83768707653506,7.));
#50508=CARTESIAN_POINT('Ctrl Pts',(65.3699753257072,-1.8597233626146,7.));
#50509=CARTESIAN_POINT('Ctrl Pts',(65.2990847711215,-1.87773280074392,7.));
#50510=CARTESIAN_POINT('Ctrl Pts',(65.2861211425482,-1.88102615439428,7.));
#50511=CARTESIAN_POINT('Ctrl Pts',(65.273111817892,-1.88418469346294,7.));
#50512=CARTESIAN_POINT('Ctrl Pts',(65.2600590170115,-1.88720850989751,7.));
#50513=CARTESIAN_POINT('Ctrl Pts',(65.2488130849708,-1.8898137464623,7.));
#50514=CARTESIAN_POINT('Ctrl Pts',(65.2375439537823,-1.89231686461017,7.));
#50515=CARTESIAN_POINT('Ctrl Pts',(65.2262547951763,-1.89471805491894,7.));
#50516=CARTESIAN_POINT('Ctrl Pts',(65.1567411013721,-1.90950353306807,7.));
#50517=CARTESIAN_POINT('Ctrl Pts',(65.0864519774429,-1.92043226303064,7.));
#50518=CARTESIAN_POINT('Ctrl Pts',(65.015754733485,-1.92760520158657,7.));
#50519=CARTESIAN_POINT('Ctrl Pts',(64.9435658003622,-1.93492948684464,7.));
#50520=CARTESIAN_POINT('Ctrl Pts',(64.8709504430061,-1.93833807716963,7.));
#50521=CARTESIAN_POINT('Ctrl Pts',(64.7982722133132,-1.93789067648535,7.));
#50522=CARTESIAN_POINT('Ctrl Pts',(64.7251526999959,-1.93744055929852,7.));
#50523=CARTESIAN_POINT('Ctrl Pts',(64.6519684871839,-1.93308764503148,7.));
#50524=CARTESIAN_POINT('Ctrl Pts',(64.5790772350591,-1.92484184820796,7.));
#50525=CARTESIAN_POINT('Ctrl Pts',(64.5610671587141,-1.92280446476361,7.));
#50526=CARTESIAN_POINT('Ctrl Pts',(64.5430749514638,-1.92052917538604,7.));
#50527=CARTESIAN_POINT('Ctrl Pts',(64.5251060094438,-1.918015636991,7.));
#50528=CARTESIAN_POINT('Ctrl Pts',(64.5110402167059,-1.91604808041119,7.));
#50529=CARTESIAN_POINT('Ctrl Pts',(64.4969870785069,-1.91393415852473,7.));
#50530=CARTESIAN_POINT('Ctrl Pts',(64.4829704724909,-1.91167739719604,7.));
#50531=CARTESIAN_POINT('Ctrl Pts',(64.4085834936561,-1.89970062785533,7.));
#50532=CARTESIAN_POINT('Ctrl Pts',(64.3350918230921,-1.88368734542449,7.));
#50533=CARTESIAN_POINT('Ctrl Pts',(64.2628790838146,-1.86371221650546,7.));
#50534=CARTESIAN_POINT('Ctrl Pts',(64.1905873443837,-1.84371523495678,7.));
#50535=CARTESIAN_POINT('Ctrl Pts',(64.1195762103623,-1.81974781469441,7.));
#50536=CARTESIAN_POINT('Ctrl Pts',(64.0502233636653,-1.79183341398573,7.));
#50537=CARTESIAN_POINT('Ctrl Pts',(63.9824494701887,-1.76455453921426,7.));
#50538=CARTESIAN_POINT('Ctrl Pts',(63.9162581817051,-1.73350624801242,7.));
#50539=CARTESIAN_POINT('Ctrl Pts',(63.8520110122706,-1.69866187357367,7.));
#50540=CARTESIAN_POINT('Ctrl Pts',(63.838191558037,-1.69116690932713,7.));
#50541=CARTESIAN_POINT('Ctrl Pts',(63.8244621192021,-1.6834961317264,7.));
#50542=CARTESIAN_POINT('Ctrl Pts',(63.8108264207747,-1.67564897964534,7.));
#50543=CARTESIAN_POINT('Ctrl Pts',(63.7992831576295,-1.66900599455042,7.));
#50544=CARTESIAN_POINT('Ctrl Pts',(63.7878070738684,-1.66223660984747,7.));
#50545=CARTESIAN_POINT('Ctrl Pts',(63.7763989699203,-1.65534250909262,7.));
#50546=CARTESIAN_POINT('Ctrl Pts',(63.1173724903363,-0.82323218010314,7.));
#50547=CARTESIAN_POINT('Ctrl Pts',(63.0939903977405,-0.752339169259015,
7.));
#50548=CARTESIAN_POINT('Ctrl Pts',(63.0748445296609,-0.680224887837059,
7.));
#50549=CARTESIAN_POINT('Ctrl Pts',(63.0598471165382,-0.607239755689072,
7.));
#50550=CARTESIAN_POINT('Ctrl Pts',(63.045242974325,-0.536168482222122,7.));
#50551=CARTESIAN_POINT('Ctrl Pts',(63.0345730321078,-0.464270523370859,
7.));
#50552=CARTESIAN_POINT('Ctrl Pts',(63.0278019508404,-0.391872562027795,
7.));
#50553=CARTESIAN_POINT('Ctrl Pts',(63.0262906434644,-0.37571331527496,7.));
#50554=CARTESIAN_POINT('Ctrl Pts',(63.0249735943724,-0.359527041219007,
7.));
#50555=CARTESIAN_POINT('Ctrl Pts',(63.0238511666502,-0.343324371082198,
7.));
#50556=CARTESIAN_POINT('Ctrl Pts',(63.0187005423293,-0.268973154322249,
7.));
#50557=CARTESIAN_POINT('Ctrl Pts',(63.01765302891,-0.194423668235733,6.99999999999999));
#50558=CARTESIAN_POINT('Ctrl Pts',(63.0206465481523,-0.12003052841074,6.99999999999999));
#50559=CARTESIAN_POINT('Ctrl Pts',(63.0227481861389,-0.0678018851499504,
6.99999999999999));
#50560=CARTESIAN_POINT('Ctrl Pts',(63.0268427413453,-0.0156503278706247,
7.));
#50561=CARTESIAN_POINT('Ctrl Pts',(63.0329233152646,0.0362966145553371,
7.));
#50562=CARTESIAN_POINT('Ctrl Pts',(63.0352354056611,0.0560490307420095,
7.));
#50563=CARTESIAN_POINT('Ctrl Pts',(63.0378347616354,0.0757718045552192,
7.));
#50564=CARTESIAN_POINT('Ctrl Pts',(63.0407214327064,0.0954576795021992,
7.));
#50565=CARTESIAN_POINT('Ctrl Pts',(63.0434693777868,0.114197501908112,7.));
#50566=CARTESIAN_POINT('Ctrl Pts',(63.0464788570236,0.132909725458142,7.));
#50567=CARTESIAN_POINT('Ctrl Pts',(63.0497439150678,0.151555112925564,7.));
#50568=CARTESIAN_POINT('Ctrl Pts',(63.0622655749108,0.223061100370353,7.));
#50569=CARTESIAN_POINT('Ctrl Pts',(63.0785510720888,0.293661818487745,7.));
#50570=CARTESIAN_POINT('Ctrl Pts',(63.0985450712042,0.363028530688884,7.));
#50571=CARTESIAN_POINT('Ctrl Pts',(63.1181095249786,0.430904988345293,7.));
#50572=CARTESIAN_POINT('Ctrl Pts',(63.1412253033662,0.497600711033835,7.));
#50573=CARTESIAN_POINT('Ctrl Pts',(63.1678836569475,0.562784339004564,6.99999999999999));
#50574=CARTESIAN_POINT('Ctrl Pts',(63.1939574715792,0.626538682555551,6.99999999999999));
#50575=CARTESIAN_POINT('Ctrl Pts',(63.2234205960509,0.688847180656012,7.));
#50576=CARTESIAN_POINT('Ctrl Pts',(63.2563003834741,0.749366435300762,7.));
#50577=CARTESIAN_POINT('Ctrl Pts',(63.2669864354346,0.769035415863878,7.));
#50578=CARTESIAN_POINT('Ctrl Pts',(63.2780336415092,0.788515094659923,7.));
#50579=CARTESIAN_POINT('Ctrl Pts',(63.2894436729518,0.807792724382841,7.));
#50580=CARTESIAN_POINT('Ctrl Pts',(63.295878298058,0.818664238701439,7.));
#50581=CARTESIAN_POINT('Ctrl Pts',(63.3024290949643,0.829472548346211,7.));
#50582=CARTESIAN_POINT('Ctrl Pts',(63.3090867443576,0.84020027364224,7.));
#50583=CARTESIAN_POINT('Ctrl Pts',(63.3451024516196,0.898233761293134,7.));
#50584=CARTESIAN_POINT('Ctrl Pts',(63.3843017903414,0.95401501249512,7.));
#50585=CARTESIAN_POINT('Ctrl Pts',(63.4266709047228,1.00724100891289,7.));
#50586=CARTESIAN_POINT('Ctrl Pts',(63.4327868740794,1.01492416603856,7.));
#50587=CARTESIAN_POINT('Ctrl Pts',(63.4389689569011,1.02255401965522,7.));
#50588=CARTESIAN_POINT('Ctrl Pts',(63.4452171764818,1.0301295944151,7.));
#50589=CARTESIAN_POINT('Ctrl Pts',(63.4893586672679,1.08364838631147,7.));
#50590=CARTESIAN_POINT('Ctrl Pts',(63.5367987510512,1.13446181353169,7.));
#50591=CARTESIAN_POINT('Ctrl Pts',(63.5871991852977,1.18242370280982,7.));
#50592=CARTESIAN_POINT('Ctrl Pts',(63.6342187269732,1.22716827863463,7.));
#50593=CARTESIAN_POINT('Ctrl Pts',(63.6838158179949,1.26943087720979,7.));
#50594=CARTESIAN_POINT('Ctrl Pts',(63.7357299599167,1.30905529564257,7.));
#50595=CARTESIAN_POINT('Ctrl Pts',(63.7471862227157,1.31779949778129,7.));
#50596=CARTESIAN_POINT('Ctrl Pts',(63.7587553478436,1.32641507643739,7.));
#50597=CARTESIAN_POINT('Ctrl Pts',(63.77043456489,1.33490009624518,7.));
#50598=CARTESIAN_POINT('Ctrl Pts',(63.7795655910972,1.34153384043588,7.));
#50599=CARTESIAN_POINT('Ctrl Pts',(63.7887633889848,1.34808730275802,7.));
#50600=CARTESIAN_POINT('Ctrl Pts',(63.7980157939078,1.35455228241838,7.));
#50601=CARTESIAN_POINT('Ctrl Pts',(63.8540658570817,1.39371642637854,7.));
#50602=CARTESIAN_POINT('Ctrl Pts',(63.9122195646569,1.42971188595968,7.));
#50603=CARTESIAN_POINT('Ctrl Pts',(63.972145843803,1.46241564583361,7.));
#50604=CARTESIAN_POINT('Ctrl Pts',(64.0317950323209,1.49496818815331,7.));
#50605=CARTESIAN_POINT('Ctrl Pts',(64.0932015439653,1.52425966109842,6.99999999999999));
#50606=CARTESIAN_POINT('Ctrl Pts',(64.1560527983145,1.5501195510723,6.99999999999999));
#50607=CARTESIAN_POINT('Ctrl Pts',(64.2175568100927,1.57542512363411,6.99999999999999));
#50608=CARTESIAN_POINT('Ctrl Pts',(64.2804452599182,1.59744473903897,7.));
#50609=CARTESIAN_POINT('Ctrl Pts',(64.3444233294929,1.615969062658,7.));
#50610=CARTESIAN_POINT('Ctrl Pts',(64.3578992521757,1.61987090518782,7.));
#50611=CARTESIAN_POINT('Ctrl Pts',(64.3714234816407,1.62361749280583,6.99999999999999));
#50612=CARTESIAN_POINT('Ctrl Pts',(64.3849931908178,1.62720657514001,6.99999999999999));
#50613=CARTESIAN_POINT('Ctrl Pts',(64.3978648606924,1.63061103151825,6.99999999999999));
#50614=CARTESIAN_POINT('Ctrl Pts',(64.4107792255323,1.63387407358145,7.));
#50615=CARTESIAN_POINT('Ctrl Pts',(64.4237128647624,1.63698901050256,7.));
#50616=CARTESIAN_POINT('Ctrl Pts',(64.4872431918316,1.65228965078473,7.));
#50617=CARTESIAN_POINT('Ctrl Pts',(64.5513507145775,1.66405191394776,6.99999999999999));
#50618=CARTESIAN_POINT('Ctrl Pts',(64.6157505858482,1.67213050415234,6.99999999999999));
#50619=CARTESIAN_POINT('Ctrl Pts',(64.6789248746032,1.68005535214111,6.99999999999999));
#50620=CARTESIAN_POINT('Ctrl Pts',(64.7423813716982,1.68443544216709,7.));
#50621=CARTESIAN_POINT('Ctrl Pts',(64.8058448174403,1.6850843166444,7.));
#50622=CARTESIAN_POINT('Ctrl Pts',(64.8672458808394,1.68571210453794,7.));
#50623=CARTESIAN_POINT('Ctrl Pts',(64.9286541091596,1.68284715375553,7.));
#50624=CARTESIAN_POINT('Ctrl Pts',(64.9898031296817,1.67627454332248,7.));
#50625=CARTESIAN_POINT('Ctrl Pts',(64.9999907153199,1.67517952935362,7.));
#50626=CARTESIAN_POINT('Ctrl Pts',(65.0101710540749,1.67398149897561,7.));
#50627=CARTESIAN_POINT('Ctrl Pts',(65.0203428468639,1.67267933134471,7.));
#50628=CARTESIAN_POINT('Ctrl Pts',(65.0310998269281,1.67130224949331,7.));
#50629=CARTESIAN_POINT('Ctrl Pts',(65.0418472497685,1.66980870242007,7.));
#50630=CARTESIAN_POINT('Ctrl Pts',(65.0525835864496,1.66819940096574,7.));
#50631=CARTESIAN_POINT('Origin',(65.,0.,-3.54592528053767));
#50632=CARTESIAN_POINT('Ctrl Pts',(67.0565599569794,0.00149374744778701,
-1.79592528053768));
#50633=CARTESIAN_POINT('Ctrl Pts',(67.0573792182402,0.0997825133646294,
-1.79058130531689));
#50634=CARTESIAN_POINT('Ctrl Pts',(67.0062893847297,0.87860858511394,-1.74819136657341));
#50635=CARTESIAN_POINT('Ctrl Pts',(66.0109392265833,2.20843178543789,-1.66875546430726));
#50636=CARTESIAN_POINT('Ctrl Pts',(63.6930089313552,2.04686416993215,-1.55761757373922));
#50637=CARTESIAN_POINT('Ctrl Pts',(62.5713939614548,0.0121365548742175,
-1.44647968317118));
#50638=CARTESIAN_POINT('Ctrl Pts',(63.67270376601,-2.03388137208553,-1.33534179260313));
#50639=CARTESIAN_POINT('Ctrl Pts',(65.9889058463299,-2.21817250383822,-1.22420390203509));
#50640=CARTESIAN_POINT('Ctrl Pts',(67.0021432190354,-0.892617277286194,
-1.14439839801327));
#50641=CARTESIAN_POINT('Ctrl Pts',(67.057275270459,-0.106740644746498,-1.10163885751414));
#50642=CARTESIAN_POINT('Ctrl Pts',(67.0563730581704,-0.00160407492545608,
-1.09592528053768));
#50643=CARTESIAN_POINT('Ctrl Pts',(67.052679279082,-0.0023836951352286,
-1.85407471946232));
#50644=CARTESIAN_POINT('Ctrl Pts',(67.0491241057456,0.467845902355832,-1.82862455259619));
#50645=CARTESIAN_POINT('Ctrl Pts',(66.6565276815742,1.62960580042267,-1.76612842220737));
#50646=CARTESIAN_POINT('Ctrl Pts',(64.7278715623352,2.41277602144419,-1.66658632829587));
#50647=CARTESIAN_POINT('Ctrl Pts',(62.8252644286755,1.08095990301173,-1.55544843772783));
#50648=CARTESIAN_POINT('Ctrl Pts',(62.9123886677794,-1.24138962897177,-1.44431054715979));
#50649=CARTESIAN_POINT('Ctrl Pts',(64.9107473342681,-2.42691462884512,-1.33317265659175));
#50650=CARTESIAN_POINT('Ctrl Pts',(66.7212428925551,-1.52545313603055,-1.23642738069259));
#50651=CARTESIAN_POINT('Ctrl Pts',(67.0499074437772,-0.417918813768391,
-1.17672806831612));
#50652=CARTESIAN_POINT('Ctrl Pts',(67.0520762837074,0.0011613687935982,
-1.15407471946233));
#50653=CARTESIAN_POINT('Ctrl Pts',(63.7309291201476,1.07935865304851,-2.));
#50654=CARTESIAN_POINT('Ctrl Pts',(63.3720166889934,0.657362393039509,-1.96295403647732));
#50655=CARTESIAN_POINT('Ctrl Pts',(63.1146663550338,-0.565736448038655,
-1.88886210943196));
#50656=CARTESIAN_POINT('Ctrl Pts',(64.4549392280646,-1.89346495741705,-1.77772421886392));
#50657=CARTESIAN_POINT('Ctrl Pts',(66.2941885938804,-1.48351678997984,-1.66658632829587));
#50658=CARTESIAN_POINT('Ctrl Pts',(66.9487863029052,0.282071400691234,-1.55544843772784));
#50659=CARTESIAN_POINT('Ctrl Pts',(65.8196738053231,1.79060584233582,-1.44431054715979));
#50660=CARTESIAN_POINT('Ctrl Pts',(63.9402861076227,1.65960613559166,-1.33317265659175));
#50661=CARTESIAN_POINT('Ctrl Pts',(63.0308759410067,0.00984037007930143,
-1.22203476602371));
#50662=CARTESIAN_POINT('Ctrl Pts',(63.9238225935869,-1.64907962812726,-1.11089687545567));
#50663=CARTESIAN_POINT('Ctrl Pts',(65.8018090473224,-1.79850365805791,-0.999758984887623));
#50664=CARTESIAN_POINT('Ctrl Pts',(66.9458893611786,-0.301774776475126,
-0.888621094319584));
#50665=CARTESIAN_POINT('Ctrl Pts',(66.3088756966202,1.47119119673887,-0.777483203751541));
#50666=CARTESIAN_POINT('Ctrl Pts',(64.4738329478959,1.89754943555687,-0.666345313183499));
#50667=CARTESIAN_POINT('Ctrl Pts',(63.1203970290852,0.587064100833473,-0.555207422615458));
#50668=CARTESIAN_POINT('Ctrl Pts',(63.4873829445486,-1.26077017125901,-0.444069532047416));
#50669=CARTESIAN_POINT('Ctrl Pts',(65.2388844462753,-1.95460593523975,-0.332931641479374));
#50670=CARTESIAN_POINT('Ctrl Pts',(66.7717322843115,-0.859369365311608,
-0.221793750911332));
#50671=CARTESIAN_POINT('Ctrl Pts',(66.6828934802986,1.02245805795664,-0.11065586034329));
#50672=CARTESIAN_POINT('Ctrl Pts',(65.0536831830854,1.96841785926001,0.000482030224751804));
#50673=CARTESIAN_POINT('Ctrl Pts',(63.3753360623109,1.1126625548375,0.111619920792793));
#50674=CARTESIAN_POINT('Ctrl Pts',(63.1840622672629,-0.761525447206207,
0.222757811360836));
#50675=CARTESIAN_POINT('Ctrl Pts',(64.654936873825,-1.93868054946276,0.333895701928877));
#50676=CARTESIAN_POINT('Ctrl Pts',(66.4416516727014,-1.34133936965715,0.445033592496918));
#50677=CARTESIAN_POINT('Ctrl Pts',(66.9088063462926,0.483744952595409,0.55617148306496));
#50678=CARTESIAN_POINT('Ctrl Pts',(65.6288089236944,1.86605203086771,0.667309373633002));
#50679=CARTESIAN_POINT('Ctrl Pts',(63.7732555621069,1.54034052425233,0.778447264201044));
#50680=CARTESIAN_POINT('Ctrl Pts',(63.0405552967276,-0.195262133588717,
0.889585154769085));
#50681=CARTESIAN_POINT('Ctrl Pts',(64.1013569898796,-1.7521391457636,1.00072304533713));
#50682=CARTESIAN_POINT('Ctrl Pts',(65.9846968214939,-1.70526332739895,1.11186093590517));
#50683=CARTESIAN_POINT('Ctrl Pts',(66.9667324851762,-0.0975406463695941,
1.22299882647321));
#50684=CARTESIAN_POINT('Ctrl Pts',(66.148595600912,1.59946209441983,1.33413671704125));
#50685=CARTESIAN_POINT('Ctrl Pts',(64.2791361371736,1.83245904107737,1.4452746076093));
#50686=CARTESIAN_POINT('Ctrl Pts',(63.0694915422322,0.38818544592543,1.55641249817734));
#50687=CARTESIAN_POINT('Ctrl Pts',(63.6268632321408,-1.41139869019814,1.66755038874538));
#50688=CARTESIAN_POINT('Ctrl Pts',(65.441082578101,-1.91911359883674,1.77868827931342));
#50689=CARTESIAN_POINT('Ctrl Pts',(66.8515740381086,-0.670242066229968,
1.88982616988146));
#50690=CARTESIAN_POINT('Ctrl Pts',(66.5672987827578,1.19210963065828,2.0009640604495));
#50691=CARTESIAN_POINT('Ctrl Pts',(64.8484571771716,1.9633098631627,2.11210195101754));
#50692=CARTESIAN_POINT('Ctrl Pts',(63.2683244359328,0.937470312465883,2.22323984158559));
#50693=CARTESIAN_POINT('Ctrl Pts',(63.2732139770213,-0.946446446867291,
2.33437773215363));
#50694=CARTESIAN_POINT('Ctrl Pts',(64.8586503480276,-1.96407003995016,2.44551562272167));
#50695=CARTESIAN_POINT('Ctrl Pts',(66.5734656584983,-1.18395805139742,2.55665351328971));
#50696=CARTESIAN_POINT('Ctrl Pts',(66.8480700074314,0.679844168596883,2.66779140385775));
#50697=CARTESIAN_POINT('Ctrl Pts',(65.4311149200231,1.92137731111722,2.7789292944258));
#50698=CARTESIAN_POINT('Ctrl Pts',(63.6195554571419,1.40425201087122,2.89006718499384));
#50699=CARTESIAN_POINT('Ctrl Pts',(63.0715325396447,-0.398201080226104,
3.00120507556188));
#50700=CARTESIAN_POINT('Ctrl Pts',(64.2886577589191,-1.83617620668518,3.11234296612993));
#50701=CARTESIAN_POINT('Ctrl Pts',(66.1568825986246,-1.59347842751063,3.22348085669796));
#50702=CARTESIAN_POINT('Ctrl Pts',(66.9661996758679,0.107748227638466,3.33461874726601));
#50703=CARTESIAN_POINT('Ctrl Pts',(65.9758318915686,1.71035170808285,3.44575663783405));
#50704=CARTESIAN_POINT('Ctrl Pts',(64.0922741102298,1.74745087340983,3.55689452840209));
#50705=CARTESIAN_POINT('Ctrl Pts',(63.0395681301103,0.185088436867106,3.66803241897013));
#50706=CARTESIAN_POINT('Ctrl Pts',(63.7812676733087,-1.54668754499179,3.77917030953817));
#50707=CARTESIAN_POINT('Ctrl Pts',(65.6384867364955,-1.86276287627795,3.89030820010621));
#50708=CARTESIAN_POINT('Ctrl Pts',(66.9112916488297,-0.473830221762714,
4.00144609067426));
#50709=CARTESIAN_POINT('Ctrl Pts',(66.4346696394808,1.34880460837872,4.11258398124229));
#50710=CARTESIAN_POINT('Ctrl Pts',(64.6448782388305,1.93686328389463,4.22372187181034));
#50711=CARTESIAN_POINT('Ctrl Pts',(63.1801338135814,0.752089030319261,4.33485976237838));
#50712=CARTESIAN_POINT('Ctrl Pts',(63.3811335473526,-1.12108084233401,4.44599765294643));
#50713=CARTESIAN_POINT('Ctrl Pts',(65.0639001046135,-1.96811270537376,4.55713554351446));
#50714=CARTESIAN_POINT('Ctrl Pts',(66.6881781710758,-1.0137086906561,4.66827343408251));
#50715=CARTESIAN_POINT('Ctrl Pts',(66.7672476130381,0.868554387592538,4.77941132465054));
#50716=CARTESIAN_POINT('Ctrl Pts',(65.2287352713998,1.95581977940926,4.8905492152186));
#50717=CARTESIAN_POINT('Ctrl Pts',(63.4808589446452,1.25290115725713,5.00168710578663));
#50718=CARTESIAN_POINT('Ctrl Pts',(63.1234696485087,-0.596812123952619,
5.11282499635468));
#50719=CARTESIAN_POINT('Ctrl Pts',(64.4836898753931,-1.90025645848877,5.22396288692272));
#50720=CARTESIAN_POINT('Ctrl Pts',(66.3164945930014,-1.46437458763454,5.33510077749075));
#50721=CARTESIAN_POINT('Ctrl Pts',(66.9442969223188,0.31186611096645,5.44623866805881));
#50722=CARTESIAN_POINT('Ctrl Pts',(65.7924621445391,1.80265190489436,5.55737655862683));
#50723=CARTESIAN_POINT('Ctrl Pts',(63.9152779448642,1.64345059076357,5.66851444919488));
#50724=CARTESIAN_POINT('Ctrl Pts',(63.0309518163246,-0.0200209171529675,
5.77965233976292));
#50725=CARTESIAN_POINT('Ctrl Pts',(63.9489184664916,-1.66516462760289,5.89079023033097));
#50726=CARTESIAN_POINT('Ctrl Pts',(65.8289506914941,-1.78616905068824,6.001928120899));
#50727=CARTESIAN_POINT('Ctrl Pts',(66.9502374569467,-0.272263260809144,
6.11306601146705));
#50728=CARTESIAN_POINT('Ctrl Pts',(66.2864448139981,1.49082960024053,6.22420390203509));
#50729=CARTESIAN_POINT('Ctrl Pts',(64.4451643957601,1.88938584790038,6.33534179260314));
#50730=CARTESIAN_POINT('Ctrl Pts',(63.1117120727514,0.558493595662749,6.44647968317117));
#50731=CARTESIAN_POINT('Ctrl Pts',(63.5066690059847,-1.28345183053528,6.55761757373921));
#50732=CARTESIAN_POINT('Ctrl Pts',(65.2684140085621,-1.95091987271333,6.66875546430726));
#50733=CARTESIAN_POINT('Ctrl Pts',(66.7846240008828,-0.832135508767304,
6.77989335487529));
#50734=CARTESIAN_POINT('Ctrl Pts',(66.6670561422041,1.04722013035562,6.89103124544334));
#50735=CARTESIAN_POINT('Ctrl Pts',(65.0241955006465,1.97020693527806,7.00216913601138));
#50736=CARTESIAN_POINT('Ctrl Pts',(63.3579443006206,1.08544634211747,7.11330702657943));
#50737=CARTESIAN_POINT('Ctrl Pts',(63.2516046182892,-0.159901738299191,
7.18739895362479));
#50738=CARTESIAN_POINT('Ctrl Pts',(63.4735576439471,-0.667480137268199,
7.22444491714747));
#50739=CARTESIAN_POINT('Ctrl Pts',(63.6322193753412,1.16331236980974,-2.07481497238249));
#50740=CARTESIAN_POINT('Ctrl Pts',(63.2453903360215,0.708492771249616,-2.03776900885981));
#50741=CARTESIAN_POINT('Ctrl Pts',(62.9680230067985,-0.609740058317773,
-1.96367708181445));
#50742=CARTESIAN_POINT('Ctrl Pts',(64.4125437948732,-2.04074076818053,-1.85253919124641));
#50743=CARTESIAN_POINT('Ctrl Pts',(66.3948520224261,-1.59890637623528,-1.74140130067836));
#50744=CARTESIAN_POINT('Ctrl Pts',(67.1003650694627,0.304011228025913,-1.63026341011032));
#50745=CARTESIAN_POINT('Ctrl Pts',(65.8834289457431,1.92988115670317,-1.51912551954228));
#50746=CARTESIAN_POINT('Ctrl Pts',(63.8578603822002,1.78869214703849,-1.40798762897424));
#50747=CARTESIAN_POINT('Ctrl Pts',(62.8777152811561,0.0106057650109386,
-1.2968497384062));
#50748=CARTESIAN_POINT('Ctrl Pts',(63.8401163177279,-1.77734687611335,-1.18571184783815));
#50749=CARTESIAN_POINT('Ctrl Pts',(65.8641746469915,-1.93839327331801,-1.07457395727011));
#50750=CARTESIAN_POINT('Ctrl Pts',(67.0972428003859,-0.325247154297195,
-0.963436066702072));
#50751=CARTESIAN_POINT('Ctrl Pts',(66.4106815043556,1.58562208464048,-0.852298176134029));
#50752=CARTESIAN_POINT('Ctrl Pts',(64.4329070892513,2.04514294157383,-0.741160285565989));
#50753=CARTESIAN_POINT('Ctrl Pts',(62.9741994190526,0.632726599672811,-0.630022394997946));
#50754=CARTESIAN_POINT('Ctrl Pts',(63.3697299072724,-1.35883427771699,-0.518884504429905));
#50755=CARTESIAN_POINT('Ctrl Pts',(65.2574651442524,-2.10663735927426,-0.407746613861863));
#50756=CARTESIAN_POINT('Ctrl Pts',(66.9095395923399,-0.926212070546681,
-0.296608723293821));
#50757=CARTESIAN_POINT('Ctrl Pts',(66.8137908073226,1.10198598313284,-0.185470832725779));
#50758=CARTESIAN_POINT('Ctrl Pts',(65.0578587207854,2.12152359010982,-0.0743329421577371));
#50759=CARTESIAN_POINT('Ctrl Pts',(63.2489678938882,1.19920668612863,0.036804948410304));
#50760=CARTESIAN_POINT('Ctrl Pts',(63.0428166102798,-0.820757743645065,
0.147942838978346));
#50761=CARTESIAN_POINT('Ctrl Pts',(64.6280974800075,-2.08947327927542,0.259080729546388));
#50762=CARTESIAN_POINT('Ctrl Pts',(66.5537849435622,-1.44567023799533,0.370218620114429));
#50763=CARTESIAN_POINT('Ctrl Pts',(67.0572754273494,0.521371173147926,0.481356510682472));
#50764=CARTESIAN_POINT('Ctrl Pts',(65.6777183812947,2.0111956337088,0.592494401250513));
#50765=CARTESIAN_POINT('Ctrl Pts',(63.6778380150419,1.66014992377277,0.703632291818555));
#50766=CARTESIAN_POINT('Ctrl Pts',(62.8881475079326,-0.210449839557629,
0.814770182386596));
#50767=CARTESIAN_POINT('Ctrl Pts',(64.0314595368616,-1.88842247767948,0.925908072954638));
#50768=CARTESIAN_POINT('Ctrl Pts',(66.0612876356907,-1.83790060601567,1.03704596352268));
#50769=CARTESIAN_POINT('Ctrl Pts',(67.1197071257548,-0.105127466352823,
1.14818385409072));
#50770=CARTESIAN_POINT('Ctrl Pts',(66.2379346445003,1.72387003543738,1.25932174465876));
#50771=CARTESIAN_POINT('Ctrl Pts',(64.2230665440017,1.97498974380222,1.37045963522681));
#50772=CARTESIAN_POINT('Ctrl Pts',(62.9193344468026,0.418378941744459,1.48159752579485));
#50773=CARTESIAN_POINT('Ctrl Pts',(63.5200591267976,-1.52117885042514,1.59273541636289));
#50774=CARTESIAN_POINT('Ctrl Pts',(65.4753904717057,-2.06838438946254,1.70387330693093));
#50775=CARTESIAN_POINT('Ctrl Pts',(66.995591526567,-0.722374239748755,1.81501119749897));
#50776=CARTESIAN_POINT('Ctrl Pts',(66.6892050256144,1.28483324388725,1.92614908806702));
#50777=CARTESIAN_POINT('Ctrl Pts',(64.8366700078289,2.11601828839369,2.03728697863506));
#50778=CARTESIAN_POINT('Ctrl Pts',(63.1336327841659,1.01038779625362,2.1484248692031));
#50779=CARTESIAN_POINT('Ctrl Pts',(63.1389026391995,-1.02006210437422,2.25956275977114));
#50780=CARTESIAN_POINT('Ctrl Pts',(64.8476560148535,-2.11683759257733,2.37070065033918));
#50781=CARTESIAN_POINT('Ctrl Pts',(66.6958515678104,-1.2760476257233,2.48183854090722));
#50782=CARTESIAN_POINT('Ctrl Pts',(66.9918149484855,0.732723204319577,2.59297643147526));
#50783=CARTESIAN_POINT('Ctrl Pts',(65.4646475180941,2.07082417580246,2.70411432204331));
#50784=CARTESIAN_POINT('Ctrl Pts',(63.5121829449299,1.51347629442987,2.81525221261135));
#50785=CARTESIAN_POINT('Ctrl Pts',(62.9215341952643,-0.429173603222882,
2.92639010317939));
#50786=CARTESIAN_POINT('Ctrl Pts',(64.2333287680788,-1.97899603468615,3.03752799374743));
#50787=CARTESIAN_POINT('Ctrl Pts',(66.2468662141139,-1.71742095225948,3.14866588431547));
#50788=CARTESIAN_POINT('Ctrl Pts',(67.1191328739459,0.116129004648158,3.25980377488352));
#50789=CARTESIAN_POINT('Ctrl Pts',(66.051733181654,1.84338476660971,3.37094166545155));
#50790=CARTESIAN_POINT('Ctrl Pts',(64.0216701807284,1.88336954628659,3.4820795560196));
#50791=CARTESIAN_POINT('Ctrl Pts',(62.8870835583976,0.199484821387334,3.59321744658764));
#50792=CARTESIAN_POINT('Ctrl Pts',(63.686473317166,-1.66699062284605,3.70435533715568));
#50793=CARTESIAN_POINT('Ctrl Pts',(65.6881489451415,-2.00765064501606,3.81549322772372));
#50794=CARTESIAN_POINT('Ctrl Pts',(67.0599540394824,-0.510685263521469,
3.92663111829177));
#50795=CARTESIAN_POINT('Ctrl Pts',(66.5462598400307,1.45371613128933,4.03776900885981));
#50796=CARTESIAN_POINT('Ctrl Pts',(64.6172564731933,2.08751466476979,4.14890689942785));
#50797=CARTESIAN_POINT('Ctrl Pts',(63.0385825971008,0.810587351755158,4.26004478999589));
#50798=CARTESIAN_POINT('Ctrl Pts',(63.2552163137658,-1.20827975739151,4.37118268056393));
#50799=CARTESIAN_POINT('Ctrl Pts',(65.0688703258357,-2.12119470101482,4.48232057113198));
#50800=CARTESIAN_POINT('Ctrl Pts',(66.8194865472274,-1.09255608031047,4.59345846170002));
#50801=CARTESIAN_POINT('Ctrl Pts',(66.9047060983459,0.936111514078455,4.70459635226806));
#50802=CARTESIAN_POINT('Ctrl Pts',(65.2465265552648,2.1079456175936,4.8157342428361));
#50803=CARTESIAN_POINT('Ctrl Pts',(63.3626984633988,1.35035320305219,4.92687213340414));
#50804=CARTESIAN_POINT('Ctrl Pts',(62.9775110302329,-0.643232834874305,
5.03801002397219));
#50805=CARTESIAN_POINT('Ctrl Pts',(64.4435306995345,-2.04806051976078,5.14914791454023));
#50806=CARTESIAN_POINT('Ctrl Pts',(66.4188930069729,-1.57827527209692,5.26028580510827));
#50807=CARTESIAN_POINT('Ctrl Pts',(67.0955264998601,0.336123404011309,5.37142369567631));
#50808=CARTESIAN_POINT('Ctrl Pts',(65.8541007317118,1.9428641754081,5.48256158624435));
#50809=CARTESIAN_POINT('Ctrl Pts',(63.8309070567223,1.77128000596152,5.5936994768124));
#50810=CARTESIAN_POINT('Ctrl Pts',(62.8777970581406,-0.021578166361293,
5.70483736738043));
#50811=CARTESIAN_POINT('Ctrl Pts',(63.867164175545,-1.79468298474187,5.81597525794848));
#50812=CARTESIAN_POINT('Ctrl Pts',(65.8934273984406,-1.92509926646556,5.92711314851651));
#50813=CARTESIAN_POINT('Ctrl Pts',(67.1019290958798,-0.293440200112777,
6.03825103908457));
#50814=CARTESIAN_POINT('Ctrl Pts',(66.3865059227299,1.60678798501315,6.14938892965259));
#50815=CARTESIAN_POINT('Ctrl Pts',(64.4020086652382,2.03634438098787,6.26052682022066));
#50816=CARTESIAN_POINT('Ctrl Pts',(62.9648389371536,0.601933848826794,6.37166471078868));
#50817=CARTESIAN_POINT('Ctrl Pts',(63.3905160600216,-1.38328014168385,6.48280260135673));
#50818=CARTESIAN_POINT('Ctrl Pts',(65.2892915487438,-2.10266459070399,6.59394049192477));
#50819=CARTESIAN_POINT('Ctrl Pts',(66.9234340409675,-0.896859934344193,
6.70507838249281));
#50820=CARTESIAN_POINT('Ctrl Pts',(66.796721623453,1.12867407706946,6.81621627306086));
#50821=CARTESIAN_POINT('Ctrl Pts',(65.026077453603,2.12345182245079,6.92735416362889));
#50822=CARTESIAN_POINT('Ctrl Pts',(63.2302233816263,1.1698735661067,7.03849205419693));
#50823=CARTESIAN_POINT('Ctrl Pts',(63.1156124805061,-0.172339073385988,
7.1125839812423));
#50824=CARTESIAN_POINT('Ctrl Pts',(63.3548292594101,-0.719397484879846,
7.14962994476498));
#50825=CARTESIAN_POINT('Ctrl Pts',(63.5335096305347,1.24726608657096,-2.14962994476498));
#50826=CARTESIAN_POINT('Ctrl Pts',(63.1187639830495,0.759623149459721,-2.1125839812423));
#50827=CARTESIAN_POINT('Ctrl Pts',(62.8213796585631,-0.653743668596888,
-2.03849205419694));
#50828=CARTESIAN_POINT('Ctrl Pts',(64.370148361682,-2.18801657894401,-1.9273541636289));
#50829=CARTESIAN_POINT('Ctrl Pts',(66.4955154509718,-1.71429596249071,-1.81621627306085));
#50830=CARTESIAN_POINT('Ctrl Pts',(67.2519438360201,0.32595105536059,-1.70507838249281));
#50831=CARTESIAN_POINT('Ctrl Pts',(65.9471840861633,2.06915647107053,-1.59394049192477));
#50832=CARTESIAN_POINT('Ctrl Pts',(63.7754346567777,1.91777815848532,-1.48280260135673));
#50833=CARTESIAN_POINT('Ctrl Pts',(62.7245546213054,0.0113711599425766,
-1.37166471078869));
#50834=CARTESIAN_POINT('Ctrl Pts',(63.756410041869,-1.90561412409944,-1.26052682022064));
#50835=CARTESIAN_POINT('Ctrl Pts',(65.9265402466607,-2.07828288857812,-1.1493889296526));
#50836=CARTESIAN_POINT('Ctrl Pts',(67.2485962395932,-0.348719532119266,
-1.03825103908456));
#50837=CARTESIAN_POINT('Ctrl Pts',(66.5124873120909,1.70005297254209,-0.927113148516519));
#50838=CARTESIAN_POINT('Ctrl Pts',(64.3919812306068,2.19273644759078,-0.815975257948477));
#50839=CARTESIAN_POINT('Ctrl Pts',(62.8280018090199,0.67838909851215,-0.704837367380436));
#50840=CARTESIAN_POINT('Ctrl Pts',(63.2520768699961,-1.45689838417496,-0.593699476812394));
#50841=CARTESIAN_POINT('Ctrl Pts',(65.2760458422295,-2.25866878330876,-0.482561586244352));
#50842=CARTESIAN_POINT('Ctrl Pts',(67.0473469003682,-0.993054775781753,
-0.37142369567631));
#50843=CARTESIAN_POINT('Ctrl Pts',(66.9446881343466,1.18151390830904,-0.260285805108268));
#50844=CARTESIAN_POINT('Ctrl Pts',(65.0620342584853,2.27462932095962,-0.149147914540226));
#50845=CARTESIAN_POINT('Ctrl Pts',(63.1225997254656,1.28575081741976,-0.0380100239721848));
#50846=CARTESIAN_POINT('Ctrl Pts',(62.9015709532967,-0.879990040083925,
0.0731278665958575));
#50847=CARTESIAN_POINT('Ctrl Pts',(64.6012580861897,-2.24026600908807,0.184265757163899));
#50848=CARTESIAN_POINT('Ctrl Pts',(66.6659182144232,-1.55000110633351,0.295403647731941));
#50849=CARTESIAN_POINT('Ctrl Pts',(67.2057445084059,0.55899739370044,0.406541538299982));
#50850=CARTESIAN_POINT('Ctrl Pts',(65.7266278388951,2.1563392365499,0.517679428868024));
#50851=CARTESIAN_POINT('Ctrl Pts',(63.5824204679768,1.77995932329319,0.628817319436066));
#50852=CARTESIAN_POINT('Ctrl Pts',(62.7357397191377,-0.225637545526539,
0.739955210004107));
#50853=CARTESIAN_POINT('Ctrl Pts',(63.9615620838435,-2.02470580959537,0.85109310057215));
#50854=CARTESIAN_POINT('Ctrl Pts',(66.1378784498875,-1.97053788463238,0.96223099114019));
#50855=CARTESIAN_POINT('Ctrl Pts',(67.2726817663336,-0.112714286336053,
1.07336888170823));
#50856=CARTESIAN_POINT('Ctrl Pts',(66.3272736880886,1.84827797645493,1.18450677227627));
#50857=CARTESIAN_POINT('Ctrl Pts',(64.1669969508297,2.11752044652708,1.29564466284432));
#50858=CARTESIAN_POINT('Ctrl Pts',(62.7691773513729,0.448572437563489,1.40678255341236));
#50859=CARTESIAN_POINT('Ctrl Pts',(63.4132550214545,-1.63095901065213,1.5179204439804));
#50860=CARTESIAN_POINT('Ctrl Pts',(65.5096983653104,-2.21765518008835,1.62905833454844));
#50861=CARTESIAN_POINT('Ctrl Pts',(67.1396090150254,-0.774506413267543,
1.74019622511649));
#50862=CARTESIAN_POINT('Ctrl Pts',(66.8111112684709,1.37755685711622,1.85133411568452));
#50863=CARTESIAN_POINT('Ctrl Pts',(64.8248828384863,2.26872671362468,1.96247200625257));
#50864=CARTESIAN_POINT('Ctrl Pts',(62.9989411323989,1.08330528004136,2.07360989682061));
#50865=CARTESIAN_POINT('Ctrl Pts',(63.0045913013778,-1.09367776188116,2.18474778738865));
#50866=CARTESIAN_POINT('Ctrl Pts',(64.8366616816794,-2.26960514520451,2.29588567795669));
#50867=CARTESIAN_POINT('Ctrl Pts',(66.8182374771223,-1.36813720004918,2.40702356852474));
#50868=CARTESIAN_POINT('Ctrl Pts',(67.1355598895398,0.785602240042274,2.51816145909277));
#50869=CARTESIAN_POINT('Ctrl Pts',(65.4981801161651,2.2202710404877,2.62929934966082));
#50870=CARTESIAN_POINT('Ctrl Pts',(63.4048104327177,1.62270057798853,2.74043724022886));
#50871=CARTESIAN_POINT('Ctrl Pts',(62.771535850884,-0.460146126219659,2.8515751307969));
#50872=CARTESIAN_POINT('Ctrl Pts',(64.1779997772384,-2.12181586268713,2.96271302136494));
#50873=CARTESIAN_POINT('Ctrl Pts',(66.3368498296032,-1.84136347700833,3.07385091193299));
#50874=CARTESIAN_POINT('Ctrl Pts',(67.2720660720238,0.124509781657855,3.18498880250102));
#50875=CARTESIAN_POINT('Ctrl Pts',(66.1276344717396,1.97641782513656,3.29612669306907));
#50876=CARTESIAN_POINT('Ctrl Pts',(63.9510662512269,2.01928821916336,3.40726458363711));
#50877=CARTESIAN_POINT('Ctrl Pts',(62.734598986685,0.213881205907557,3.51840247420515));
#50878=CARTESIAN_POINT('Ctrl Pts',(63.5916789610234,-1.7872937007003,3.62954036477319));
#50879=CARTESIAN_POINT('Ctrl Pts',(65.7378111537875,-2.15253841375417,3.74067825534123));
#50880=CARTESIAN_POINT('Ctrl Pts',(67.2086164301352,-0.547540305280222,
3.85181614590928));
#50881=CARTESIAN_POINT('Ctrl Pts',(66.6578500405806,1.55862765419994,3.96295403647732));
#50882=CARTESIAN_POINT('Ctrl Pts',(64.589634707556,2.23816604564495,4.07409192704536));
#50883=CARTESIAN_POINT('Ctrl Pts',(62.8970313806202,0.869085673191056,4.1852298176134));
#50884=CARTESIAN_POINT('Ctrl Pts',(63.1292990801791,-1.295478672449,4.29636770818144));
#50885=CARTESIAN_POINT('Ctrl Pts',(65.0738405470579,-2.27427669665589,4.40750559874948));
#50886=CARTESIAN_POINT('Ctrl Pts',(66.9507949233791,-1.17140346996484,4.51864348931753));
#50887=CARTESIAN_POINT('Ctrl Pts',(67.0421645836536,1.00366864056437,4.62978137988557));
#50888=CARTESIAN_POINT('Ctrl Pts',(65.2643178391297,2.26007145577795,4.74091927045361));
#50889=CARTESIAN_POINT('Ctrl Pts',(63.2445379821525,1.44780524884725,4.85205716102165));
#50890=CARTESIAN_POINT('Ctrl Pts',(62.8315524119571,-0.689653545795988,
4.96319505158969));
#50891=CARTESIAN_POINT('Ctrl Pts',(64.4033715236759,-2.19586458103279,5.07433294215774));
#50892=CARTESIAN_POINT('Ctrl Pts',(66.5212914209443,-1.69217595655929,5.18547083272578));
#50893=CARTESIAN_POINT('Ctrl Pts',(67.2467560774014,0.360380697056169,5.29660872329382));
#50894=CARTESIAN_POINT('Ctrl Pts',(65.9157393188846,2.08307644592185,5.40774661386186));
#50895=CARTESIAN_POINT('Ctrl Pts',(63.7465361685802,1.89910942115946,5.5188845044299));
#50896=CARTESIAN_POINT('Ctrl Pts',(62.7246422999565,-0.0231354155696212,
5.63002239499795));
#50897=CARTESIAN_POINT('Ctrl Pts',(63.7854098845984,-1.92420134188085,5.74116028556599));
#50898=CARTESIAN_POINT('Ctrl Pts',(65.957904105387,-2.06402948224289,5.85229817613403));
#50899=CARTESIAN_POINT('Ctrl Pts',(67.2536207348131,-0.314617139416408,
5.96343606670207));
#50900=CARTESIAN_POINT('Ctrl Pts',(66.4865670314617,1.72274636978576,6.07457395727011));
#50901=CARTESIAN_POINT('Ctrl Pts',(64.3588529347165,2.18330291407536,6.18571184783816));
#50902=CARTESIAN_POINT('Ctrl Pts',(62.8179658015557,0.645374101990838,6.29684973840619));
#50903=CARTESIAN_POINT('Ctrl Pts',(63.2743631140587,-1.48310845283243,6.40798762897424));
#50904=CARTESIAN_POINT('Ctrl Pts',(65.3101690889255,-2.25440930869464,6.51912551954228));
#50905=CARTESIAN_POINT('Ctrl Pts',(67.0622440810523,-0.961584359921082,
6.63026341011032));
#50906=CARTESIAN_POINT('Ctrl Pts',(66.9263871047018,1.21012802378329,6.74140130067837));
#50907=CARTESIAN_POINT('Ctrl Pts',(65.0279594065595,2.27669670962353,6.8525391912464));
#50908=CARTESIAN_POINT('Ctrl Pts',(63.1025024626319,1.25430079009593,6.96367708181444));
#50909=CARTESIAN_POINT('Ctrl Pts',(62.979620342723,-0.184776408472784,7.03776900885981));
#50910=CARTESIAN_POINT('Ctrl Pts',(63.2361008748732,-0.771314832491493,
7.07481497238249));
#50911=CARTESIAN_POINT('Ctrl Pts',(63.4347998857283,1.33121980333219,-2.22444491714747));
#50912=CARTESIAN_POINT('Ctrl Pts',(62.9921376300776,0.810753527669827,-2.18739895362479));
#50913=CARTESIAN_POINT('Ctrl Pts',(62.6747363103277,-0.697747278876005,
-2.11330702657943));
#50914=CARTESIAN_POINT('Ctrl Pts',(64.3277529284907,-2.33529238970749,-2.00216913601138));
#50915=CARTESIAN_POINT('Ctrl Pts',(66.5961788795174,-1.82968554874614,-1.89103124544334));
#50916=CARTESIAN_POINT('Ctrl Pts',(67.4035226025776,0.347890882695266,-1.7798933548753));
#50917=CARTESIAN_POINT('Ctrl Pts',(66.0109392265833,2.20843178543789,-1.66875546430726));
#50918=CARTESIAN_POINT('Ctrl Pts',(63.6930089313552,2.04686416993215,-1.55761757373922));
#50919=CARTESIAN_POINT('Ctrl Pts',(62.5713939614548,0.0121365548742175,
-1.44647968317118));
#50920=CARTESIAN_POINT('Ctrl Pts',(63.67270376601,-2.03388137208553,-1.33534179260313));
#50921=CARTESIAN_POINT('Ctrl Pts',(65.9889058463299,-2.21817250383822,-1.22420390203509));
#50922=CARTESIAN_POINT('Ctrl Pts',(67.3999496788005,-0.372191909941336,
-1.11306601146705));
#50923=CARTESIAN_POINT('Ctrl Pts',(66.6142931198262,1.8144838604437,-1.00192812089901));
#50924=CARTESIAN_POINT('Ctrl Pts',(64.3510553719621,2.34032995360773,-0.890790230330967));
#50925=CARTESIAN_POINT('Ctrl Pts',(62.6818041989874,0.724051597351488,-0.779652339762924));
#50926=CARTESIAN_POINT('Ctrl Pts',(63.1344238327198,-1.55496249063293,-0.668514449194883));
#50927=CARTESIAN_POINT('Ctrl Pts',(65.2946265402067,-2.41070020734327,-0.55737655862684));
#50928=CARTESIAN_POINT('Ctrl Pts',(67.1851542083967,-1.05989748101682,-0.446238668058799));
#50929=CARTESIAN_POINT('Ctrl Pts',(67.0755854613707,1.26104183348523,-0.335100777490757));
#50930=CARTESIAN_POINT('Ctrl Pts',(65.0662097961853,2.42773505180943,-0.223962886922715));
#50931=CARTESIAN_POINT('Ctrl Pts',(62.9962315570428,1.3722949487109,-0.112824996354674));
#50932=CARTESIAN_POINT('Ctrl Pts',(62.7603252963136,-0.939222336522784,
-0.00168710578663132));
#50933=CARTESIAN_POINT('Ctrl Pts',(64.5744186923722,-2.39105873890072,0.10945078478141));
#50934=CARTESIAN_POINT('Ctrl Pts',(66.778051485284,-1.65433197467169,0.220588675349452));
#50935=CARTESIAN_POINT('Ctrl Pts',(67.3542135894627,0.596623614252954,0.331726565917493));
#50936=CARTESIAN_POINT('Ctrl Pts',(65.7755372964953,2.301482839391,0.442864456485536));
#50937=CARTESIAN_POINT('Ctrl Pts',(63.4870029209119,1.89976872281362,0.554002347053577));
#50938=CARTESIAN_POINT('Ctrl Pts',(62.5833319303427,-0.24082525149545,0.665140237621619));
#50939=CARTESIAN_POINT('Ctrl Pts',(63.8916646308255,-2.16098914151125,0.77627812818966));
#50940=CARTESIAN_POINT('Ctrl Pts',(66.2144692640843,-2.1031751632491,0.887416018757702));
#50941=CARTESIAN_POINT('Ctrl Pts',(67.4256564069122,-0.120301106319279,
0.998553909325744));
#50942=CARTESIAN_POINT('Ctrl Pts',(66.416612731677,1.97268591747247,1.10969179989378));
#50943=CARTESIAN_POINT('Ctrl Pts',(64.1109273576576,2.26005114925193,1.22082969046183));
#50944=CARTESIAN_POINT('Ctrl Pts',(62.6190202559434,0.478765933382519,1.33196758102987));
#50945=CARTESIAN_POINT('Ctrl Pts',(63.3064509161112,-1.74073917087913,1.44310547159791));
#50946=CARTESIAN_POINT('Ctrl Pts',(65.5440062589152,-2.36692597071416,1.55424336216595));
#50947=CARTESIAN_POINT('Ctrl Pts',(67.2836265034836,-0.82663858678633,1.665381252734));
#50948=CARTESIAN_POINT('Ctrl Pts',(66.9330175113275,1.4702804703452,1.77651914330204));
#50949=CARTESIAN_POINT('Ctrl Pts',(64.8130956691436,2.42143513885567,1.88765703387008));
#50950=CARTESIAN_POINT('Ctrl Pts',(62.864249480632,1.15622276382909,1.99879492443812));
#50951=CARTESIAN_POINT('Ctrl Pts',(62.8702799635561,-1.16729341938809,2.10993281500616));
#50952=CARTESIAN_POINT('Ctrl Pts',(64.8256673485052,-2.42237269783168,2.2210707055742));
#50953=CARTESIAN_POINT('Ctrl Pts',(66.9406233864343,-1.46022677437506,2.33220859614225));
#50954=CARTESIAN_POINT('Ctrl Pts',(67.279304830594,0.838481275764972,2.44334648671029));
#50955=CARTESIAN_POINT('Ctrl Pts',(65.5317127142361,2.36971790517293,2.55448437727833));
#50956=CARTESIAN_POINT('Ctrl Pts',(63.2974379205056,1.7319248615472,2.66562226784637));
#50957=CARTESIAN_POINT('Ctrl Pts',(62.6215375065036,-0.491118649216439,
2.77676015841441));
#50958=CARTESIAN_POINT('Ctrl Pts',(64.122670786398,-2.2646356906881,2.88789804898245));
#50959=CARTESIAN_POINT('Ctrl Pts',(66.4268334450924,-1.96530600175718,2.9990359395505));
#50960=CARTESIAN_POINT('Ctrl Pts',(67.4249992701018,0.132890558667548,3.11017383011854));
#50961=CARTESIAN_POINT('Ctrl Pts',(66.2035357618251,2.10945088366341,3.22131172068658));
#50962=CARTESIAN_POINT('Ctrl Pts',(63.8804623217255,2.15520689204012,3.33244961125462));
#50963=CARTESIAN_POINT('Ctrl Pts',(62.5821144149725,0.228277590427784,3.44358750182266));
#50964=CARTESIAN_POINT('Ctrl Pts',(63.4968846048806,-1.90759677855456,3.55472539239071));
#50965=CARTESIAN_POINT('Ctrl Pts',(65.7874733624335,-2.29742618249227,3.66586328295874));
#50966=CARTESIAN_POINT('Ctrl Pts',(67.3572788207879,-0.584395347038978,
3.77700117352679));
#50967=CARTESIAN_POINT('Ctrl Pts',(66.7694402411304,1.66353917711055,3.88813906409483));
#50968=CARTESIAN_POINT('Ctrl Pts',(64.5620129419189,2.3888174265201,3.99927695466288));
#50969=CARTESIAN_POINT('Ctrl Pts',(62.7554801641395,0.927583994626953,4.11041484523091));
#50970=CARTESIAN_POINT('Ctrl Pts',(63.0033818465923,-1.38267758750649,4.22155273579896));
#50971=CARTESIAN_POINT('Ctrl Pts',(65.0788107682801,-2.42735869229696,4.33269062636699));
#50972=CARTESIAN_POINT('Ctrl Pts',(67.0821032995307,-1.25025085961922,4.44382851693504));
#50973=CARTESIAN_POINT('Ctrl Pts',(67.1796230689615,1.07122576705028,4.55496640750307));
#50974=CARTESIAN_POINT('Ctrl Pts',(65.2821091229946,2.41219729396229,4.66610429807113));
#50975=CARTESIAN_POINT('Ctrl Pts',(63.1263775009061,1.54525729464231,4.77724218863916));
#50976=CARTESIAN_POINT('Ctrl Pts',(62.6855937936814,-0.736074256717675,
4.88838007920721));
#50977=CARTESIAN_POINT('Ctrl Pts',(64.3632123478174,-2.3436686423048,4.99951796977525));
#50978=CARTESIAN_POINT('Ctrl Pts',(66.6236898349158,-1.80607664102166,5.11065586034329));
#50979=CARTESIAN_POINT('Ctrl Pts',(67.3979856549427,0.384637990101029,5.22179375091133));
#50980=CARTESIAN_POINT('Ctrl Pts',(65.9773779060574,2.22328871643559,5.33293164147938));
#50981=CARTESIAN_POINT('Ctrl Pts',(63.6621652804381,2.02693883635741,5.44406953204741));
#50982=CARTESIAN_POINT('Ctrl Pts',(62.5714875417724,-0.0246926647779473,
5.55520742261546));
#50983=CARTESIAN_POINT('Ctrl Pts',(63.7036555936518,-2.05371969901983,5.66634531318349));
#50984=CARTESIAN_POINT('Ctrl Pts',(66.0223808123334,-2.20295969802021,5.77748320375154));
#50985=CARTESIAN_POINT('Ctrl Pts',(67.4053123737463,-0.335794078720041,
5.88862109431958));
#50986=CARTESIAN_POINT('Ctrl Pts',(66.5866281401934,1.83870475455837,5.99975898488763));
#50987=CARTESIAN_POINT('Ctrl Pts',(64.3156972041947,2.33026144716285,6.11089687545566));
#50988=CARTESIAN_POINT('Ctrl Pts',(62.6710926659578,0.688814355154883,6.22203476602371));
#50989=CARTESIAN_POINT('Ctrl Pts',(63.1582101680956,-1.58293676398101,6.33317265659174));
#50990=CARTESIAN_POINT('Ctrl Pts',(65.3310466291073,-2.4061540266853,6.4443105471598));
#50991=CARTESIAN_POINT('Ctrl Pts',(67.2010541211369,-1.02630878549797,6.55544843772783));
#50992=CARTESIAN_POINT('Ctrl Pts',(67.0560525859507,1.29158197049713,6.66658632829588));
#50993=CARTESIAN_POINT('Ctrl Pts',(65.029841359516,2.42994159679627,6.77772421886392));
#50994=CARTESIAN_POINT('Ctrl Pts',(62.9747815436376,1.33872801408516,6.88886210943195));
#50995=CARTESIAN_POINT('Ctrl Pts',(62.8436282049399,-0.197213743559581,
6.96295403647732));
#50996=CARTESIAN_POINT('Ctrl Pts',(63.1173724903363,-0.82323218010314,7.));
#50997=CARTESIAN_POINT('Ctrl Pts',(63.7309291201476,1.07935865304851,-2.));
#50998=CARTESIAN_POINT('Ctrl Pts',(63.6855968419854,1.03706844878193,-2.));
#50999=CARTESIAN_POINT('Ctrl Pts',(63.6429944057469,0.992209355215868,-2.));
#51000=CARTESIAN_POINT('Ctrl Pts',(63.6031204505518,0.945126337776206,-2.));
#51001=CARTESIAN_POINT('Ctrl Pts',(63.5606157477665,0.894936943402905,-2.));
#51002=CARTESIAN_POINT('Ctrl Pts',(63.5212107097528,0.842220257206834,-2.));
#51003=CARTESIAN_POINT('Ctrl Pts',(63.4849325153228,0.787339414500543,-2.));
#51004=CARTESIAN_POINT('Ctrl Pts',(63.4531890951965,0.739318677132538,-2.));
#51005=CARTESIAN_POINT('Ctrl Pts',(63.4238399078534,0.689639781931255,-2.));
#51006=CARTESIAN_POINT('Ctrl Pts',(63.3969260537536,0.638518448144012,-2.));
#51007=CARTESIAN_POINT('Ctrl Pts',(63.3834208986394,0.612866174787509,-2.));
#51008=CARTESIAN_POINT('Ctrl Pts',(63.3705293094211,0.586850346511891,-2.));
#51009=CARTESIAN_POINT('Ctrl Pts',(63.3582588228011,0.560496376489487,-2.));
#51010=CARTESIAN_POINT('Ctrl Pts',(63.3526556403243,0.548462126537112,-2.));
#51011=CARTESIAN_POINT('Ctrl Pts',(63.3471814026121,0.536355708793655,-2.));
#51012=CARTESIAN_POINT('Ctrl Pts',(63.3418453144691,0.524199442929296,-2.));
#51013=CARTESIAN_POINT('Ctrl Pts',(63.3149230085512,0.462867114893175,-2.));
#51014=CARTESIAN_POINT('Ctrl Pts',(63.2914620509973,0.400159371536742,-2.));
#51015=CARTESIAN_POINT('Ctrl Pts',(63.2714860817372,0.336433888030266,-2.));
#51016=CARTESIAN_POINT('Ctrl Pts',(63.2511562856396,0.271579658979292,-2.));
#51017=CARTESIAN_POINT('Ctrl Pts',(63.234435470153,0.205670475363271,-2.));
#51018=CARTESIAN_POINT('Ctrl Pts',(63.2213878692259,0.139046848385531,-2.));
#51019=CARTESIAN_POINT('Ctrl Pts',(63.2104743799268,0.0833204168257664,
-2.));
#51020=CARTESIAN_POINT('Ctrl Pts',(63.2021313216505,0.0270932010885611,
-2.));
#51021=CARTESIAN_POINT('Ctrl Pts',(63.1964211149777,-0.0294478216180754,
-2.));
#51022=CARTESIAN_POINT('Ctrl Pts',(63.1937898542026,-0.0555019005259951,
-2.));
#51023=CARTESIAN_POINT('Ctrl Pts',(63.1917179786585,-0.0816227252280235,
-2.));
#51024=CARTESIAN_POINT('Ctrl Pts',(63.1902134007643,-0.107792402833692,
-2.));
#51025=CARTESIAN_POINT('Ctrl Pts',(63.1895569069983,-0.119211040759237,
-2.));
#51026=CARTESIAN_POINT('Ctrl Pts',(63.1890085369681,-0.130638731934728,
-2.));
#51027=CARTESIAN_POINT('Ctrl Pts',(63.188569278878,-0.142059931589906,-2.));
#51028=CARTESIAN_POINT('Ctrl Pts',(63.1858723378449,-0.212183402721495,
-2.));
#51029=CARTESIAN_POINT('Ctrl Pts',(63.1872764272312,-0.282193469637118,
-2.));
#51030=CARTESIAN_POINT('Ctrl Pts',(63.1928363192141,-0.351729486371673,
-2.));
#51031=CARTESIAN_POINT('Ctrl Pts',(63.1978071231062,-0.413897942825674,
-2.));
#51032=CARTESIAN_POINT('Ctrl Pts',(63.2061000911913,-0.475688445032767,
-2.));
#51033=CARTESIAN_POINT('Ctrl Pts',(63.2177875010733,-0.536855401025573,
-2.));
#51034=CARTESIAN_POINT('Ctrl Pts',(63.2305203455448,-0.603493719122339,
-2.));
#51035=CARTESIAN_POINT('Ctrl Pts',(63.2472809681187,-0.669392782961396,
-2.));
#51036=CARTESIAN_POINT('Ctrl Pts',(63.2678240437401,-0.734338936172354,
-2.));
#51037=CARTESIAN_POINT('Ctrl Pts',(63.2757504472629,-0.759397959810863,
-2.));
#51038=CARTESIAN_POINT('Ctrl Pts',(63.2842405167726,-0.784315071865798,
-2.));
#51039=CARTESIAN_POINT('Ctrl Pts',(63.2932821667432,-0.809077679604566,
-2.));
#51040=CARTESIAN_POINT('Ctrl Pts',(63.2972485928295,-0.819940636434083,
-2.));
#51041=CARTESIAN_POINT('Ctrl Pts',(63.301321059107,-0.830773275870266,-2.));
#51042=CARTESIAN_POINT('Ctrl Pts',(63.305493469376,-0.84156202494396,-2.));
#51043=CARTESIAN_POINT('Ctrl Pts',(63.3307175500488,-0.906784824105441,
-2.));
#51044=CARTESIAN_POINT('Ctrl Pts',(63.3596326694677,-0.970522726147455,
-2.));
#51045=CARTESIAN_POINT('Ctrl Pts',(63.3919260622372,-1.03255684531855,-2.));
#51046=CARTESIAN_POINT('Ctrl Pts',(63.4249680867708,-1.0960290516056,-2.));
#51047=CARTESIAN_POINT('Ctrl Pts',(63.4615471340283,-1.15771838394187,-2.));
#51048=CARTESIAN_POINT('Ctrl Pts',(63.5013843211809,-1.21738667180208,-2.));
#51049=CARTESIAN_POINT('Ctrl Pts',(63.5318674685179,-1.26304444385366,-2.));
#51050=CARTESIAN_POINT('Ctrl Pts',(63.5642595400749,-1.30751888441863,-2.));
#51051=CARTESIAN_POINT('Ctrl Pts',(63.5984551101011,-1.35069719140617,-2.));
#51052=CARTESIAN_POINT('Ctrl Pts',(63.6197386625932,-1.37757165972414,-2.));
#51053=CARTESIAN_POINT('Ctrl Pts',(63.6417211957122,-1.40394389607449,-2.));
#51054=CARTESIAN_POINT('Ctrl Pts',(63.6643801907515,-1.42978501718758,-2.));
#51055=CARTESIAN_POINT('Ctrl Pts',(63.6770896558904,-1.44427934173145,-2.));
#51056=CARTESIAN_POINT('Ctrl Pts',(63.6900164428935,-1.45861113921514,-2.));
#51057=CARTESIAN_POINT('Ctrl Pts',(63.7031327806133,-1.4727497841485,-2.));
#51058=CARTESIAN_POINT('Ctrl Pts',(63.7540080482783,-1.52759034717556,-2.));
#51059=CARTESIAN_POINT('Ctrl Pts',(63.8077798406958,-1.57958602567074,-2.));
#51060=CARTESIAN_POINT('Ctrl Pts',(63.864163060535,-1.62847278877981,-2.));
#51061=CARTESIAN_POINT('Ctrl Pts',(63.9063355382314,-1.6650382054542,-2.));
#51062=CARTESIAN_POINT('Ctrl Pts',(63.9499701263758,-1.69986415254484,-2.));
#51063=CARTESIAN_POINT('Ctrl Pts',(63.9949639294552,-1.73283039560955,-2.));
#51064=CARTESIAN_POINT('Ctrl Pts',(64.0089991299538,-1.74311376352765,-2.));
#51065=CARTESIAN_POINT('Ctrl Pts',(64.0231666801194,-1.7532160976543,-2.));
#51066=CARTESIAN_POINT('Ctrl Pts',(64.0374636965982,-1.76313352319509,-2.));
#51067=CARTESIAN_POINT('Ctrl Pts',(64.0512649018476,-1.7727070188707,-2.));
#51068=CARTESIAN_POINT('Ctrl Pts',(64.0651797317906,-1.78210327692406,-2.));
#51069=CARTESIAN_POINT('Ctrl Pts',(64.0792001599556,-1.7913160321663,-2.));
#51070=CARTESIAN_POINT('Ctrl Pts',(64.1421565047859,-1.83268434054044,-2.));
#51071=CARTESIAN_POINT('Ctrl Pts',(64.2072699652678,-1.87037681376273,-2.));
#51072=CARTESIAN_POINT('Ctrl Pts',(64.2742791023333,-1.90411417796279,-2.));
#51073=CARTESIAN_POINT('Ctrl Pts',(64.3255634213005,-1.92993450370516,-2.));
#51074=CARTESIAN_POINT('Ctrl Pts',(64.3779590786631,-1.95343777834749,-2.));
#51075=CARTESIAN_POINT('Ctrl Pts',(64.4313627927198,-1.97448349564832,-2.));
#51076=CARTESIAN_POINT('Ctrl Pts',(64.4437562344803,-1.97936759175068,-2.));
#51077=CARTESIAN_POINT('Ctrl Pts',(64.4562040109557,-1.98411926473272,-2.));
#51078=CARTESIAN_POINT('Ctrl Pts',(64.4687042096542,-1.98873909628092,-2.));
#51079=CARTESIAN_POINT('Ctrl Pts',(66.6673159824367,-0.00130059074131283,
-0.871480363390211));
#51080=CARTESIAN_POINT('Ctrl Pts',(66.6680474999804,-0.0865457667101108,
-0.877193940366669));
#51081=CARTESIAN_POINT('Ctrl Pts',(66.6620744628598,-0.171688078253662,
-0.882907517343126));
#51082=CARTESIAN_POINT('Ctrl Pts',(66.6490403647761,-0.255735261203256,
-0.888621094319584));
#51083=CARTESIAN_POINT('Ctrl Pts',(66.5645292565598,-0.800684403669386,
-0.925667057842264));
#51084=CARTESIAN_POINT('Ctrl Pts',(66.1831691519411,-1.29959403086365,-0.962713021364943));
#51085=CARTESIAN_POINT('Ctrl Pts',(65.6794913573425,-1.52414483947233,-0.999758984887624));
#51086=CARTESIAN_POINT('Ctrl Pts',(65.1758135627439,-1.74869564808102,-1.0368049484103));
#51087=CARTESIAN_POINT('Ctrl Pts',(64.5498180781654,-1.69888763810414,-1.07385091193299));
#51088=CARTESIAN_POINT('Ctrl Pts',(64.0879958937795,-1.39749696674794,-1.11089687545567));
#51089=CARTESIAN_POINT('Ctrl Pts',(63.6261737093935,-1.09610629539174,-1.14794283897835));
#51090=CARTESIAN_POINT('Ctrl Pts',(63.3285248252001,-0.54313296265622,-1.18498880250103));
#51091=CARTESIAN_POINT('Ctrl Pts',(63.3312687442061,0.00831466463026731,
-1.22203476602371));
#51092=CARTESIAN_POINT('Ctrl Pts',(63.3340126632121,0.559762291916755,-1.25908072954639));
#51093=CARTESIAN_POINT('Ctrl Pts',(63.6371493854174,1.10968421375421,-1.29612669306907));
#51094=CARTESIAN_POINT('Ctrl Pts',(64.1019490294701,1.40647845913029,-1.33317265659175));
#51095=CARTESIAN_POINT('Ctrl Pts',(64.5667486735228,1.70327270450638,-1.37021862011443));
#51096=CARTESIAN_POINT('Ctrl Pts',(65.193211239423,1.7469392734211,-1.40726458363711));
#51097=CARTESIAN_POINT('Ctrl Pts',(65.6946279386367,1.51735015093769,-1.44431054715979));
#51098=CARTESIAN_POINT('Ctrl Pts',(66.1960446378505,1.28776102845429,-1.48135651068247));
#51099=CARTESIAN_POINT('Ctrl Pts',(66.5724154703778,0.784916214572762,-1.51840247420515));
#51100=CARTESIAN_POINT('Ctrl Pts',(66.6515012684707,0.239229109186819,-1.55544843772783));
#51101=CARTESIAN_POINT('Ctrl Pts',(66.6629095976148,0.160512345140362,-1.56079241294863));
#51102=CARTESIAN_POINT('Ctrl Pts',(66.6681317812815,0.0809040843243828,
-1.56613638816942));
#51103=CARTESIAN_POINT('Ctrl Pts',(66.6674675207825,0.00121113675536799,
-1.57148036339021));
#51104=CARTESIAN_POINT('Ctrl Pts',(65.5301702171886,-1.98517432567172,-2.));
#51105=CARTESIAN_POINT('Ctrl Pts',(66.1902879097456,-1.80888011517988,-1.96295403647732));
#51106=CARTESIAN_POINT('Ctrl Pts',(67.3093622463653,-0.748693059830632,
-1.88886210943196));
#51107=CARTESIAN_POINT('Ctrl Pts',(66.8811995093437,1.53837321455301,-1.77772421886392));
#51108=CARTESIAN_POINT('Ctrl Pts',(64.7278715623352,2.41277602144419,-1.66658632829587));
#51109=CARTESIAN_POINT('Ctrl Pts',(62.8252644286755,1.08095990301173,-1.55544843772783));
#51110=CARTESIAN_POINT('Ctrl Pts',(62.9123886677794,-1.24138962897177,-1.44431054715979));
#51111=CARTESIAN_POINT('Ctrl Pts',(64.9107473342681,-2.42691462884512,-1.33317265659175));
#51112=CARTESIAN_POINT('Ctrl Pts',(66.9905869477348,-1.39134438721222,-1.22203476602371));
#51113=CARTESIAN_POINT('Ctrl Pts',(67.24852778644,0.917884815202477,-1.11089687545567));
#51114=CARTESIAN_POINT('Ctrl Pts',(65.4483108550045,2.38688976599863,-0.999758984887625));
#51115=CARTESIAN_POINT('Ctrl Pts',(63.2377776981899,1.67118490708906,-0.888621094319582));
#51116=CARTESIAN_POINT('Ctrl Pts',(62.6402125087857,-0.574193448178934,
-0.777483203751542));
#51117=CARTESIAN_POINT('Ctrl Pts',(64.2025947176117,-2.29399639382145,-0.666345313183498));
#51118=CARTESIAN_POINT('Ctrl Pts',(66.4948474007694,-1.91408331059475,-0.555207422615458));
#51119=CARTESIAN_POINT('Ctrl Pts',(67.4188511430454,0.217814411897158,-0.444069532047416));
#51120=CARTESIAN_POINT('Ctrl Pts',(66.1288520704621,2.15034287637184,-0.332931641479373));
#51121=CARTESIAN_POINT('Ctrl Pts',(63.8056023683761,2.11463875683278,-0.221793750911332));
#51122=CARTESIAN_POINT('Ctrl Pts',(62.5755981242121,0.143381478345983,-0.110655860343291));
#51123=CARTESIAN_POINT('Ctrl Pts',(63.5646765331008,-1.95911432942998,0.00048203022475183));
#51124=CARTESIAN_POINT('Ctrl Pts',(65.8675227272721,-2.26841065672895,0.111619920792793));
#51125=CARTESIAN_POINT('Ctrl Pts',(67.3763155620569,-0.501404942245515,
0.222757811360835));
#51126=CARTESIAN_POINT('Ctrl Pts',(66.7100397977853,1.72454238081742,0.333895701928876));
#51127=CARTESIAN_POINT('Ctrl Pts',(64.4785452214709,2.37199651591817,0.445033592496919));
#51128=CARTESIAN_POINT('Ctrl Pts',(62.7243441135659,0.848335334231218,0.55617148306496));
#51129=CARTESIAN_POINT('Ctrl Pts',(63.0530766482751,-1.45181679686653,0.667309373633002));
#51130=CARTESIAN_POINT('Ctrl Pts',(65.1638502053818,-2.42310455048396,0.778447264201043));
#51131=CARTESIAN_POINT('Ctrl Pts',(67.1246498118468,-1.17649722845176,0.889585154769086));
#51132=CARTESIAN_POINT('Ctrl Pts',(67.1407333500909,1.14697134880473,1.00072304533713));
#51133=CARTESIAN_POINT('Ctrl Pts',(65.1973793755662,2.42060404314488,1.11186093590517));
#51134=CARTESIAN_POINT('Ctrl Pts',(63.0733618200821,1.47863040518407,1.22299882647321));
#51135=CARTESIAN_POINT('Ctrl Pts',(62.7128180402749,-0.816750411403602,
1.33413671704125));
#51136=CARTESIAN_POINT('Ctrl Pts',(64.4457578465939,-2.36455031387796,1.4452746076093));
#51137=CARTESIAN_POINT('Ctrl Pts',(66.686001781468,-1.74805049822322,1.55641249817733));
#51138=CARTESIAN_POINT('Ctrl Pts',(67.3830291651992,0.468459762690022,1.66755038874538));
#51139=CARTESIAN_POINT('Ctrl Pts',(65.898842928637,2.25618349012117,1.77868827931342));
#51140=CARTESIAN_POINT('Ctrl Pts',(63.5919355659201,1.97879688218179,1.88982616988146));
#51141=CARTESIAN_POINT('Ctrl Pts',(62.5738455482538,-0.109804953100732,
2.0009640604495));
#51142=CARTESIAN_POINT('Ctrl Pts',(63.7764422147334,-2.09790106953769,2.11210195101754));
#51143=CARTESIAN_POINT('Ctrl Pts',(66.0989751981566,-2.1657645452103,2.22323984158559));
#51144=CARTESIAN_POINT('Ctrl Pts',(67.4156037194807,-0.25127917121156,2.33437773215363));
#51145=CARTESIAN_POINT('Ctrl Pts',(66.5212027615546,1.89320487789679,2.44551562272167));
#51146=CARTESIAN_POINT('Ctrl Pts',(64.234427664365,2.30481703186258,2.55665351328971));
#51147=CARTESIAN_POINT('Ctrl Pts',(62.6483896081628,0.606804018161656,2.66779140385776));
#51148=CARTESIAN_POINT('Ctrl Pts',(63.214807212685,-1.64662359498827,2.77892929442579));
#51149=CARTESIAN_POINT('Ctrl Pts',(65.4152320208998,-2.39287795766375,2.89006718499384));
#51150=CARTESIAN_POINT('Ctrl Pts',(67.2355902513335,-0.948903988607909,
3.00120507556188));
#51151=CARTESIAN_POINT('Ctrl Pts',(67.009687371404,1.36361256252398,3.11234296612992));
#51152=CARTESIAN_POINT('Ctrl Pts',(64.9442948490232,2.42799907075925,3.22348085669796));
#51153=CARTESIAN_POINT('Ctrl Pts',(62.9298898830713,1.27001049414665,3.334618747266));
#51154=CARTESIAN_POINT('Ctrl Pts',(62.8102801837889,-1.05043309065764,3.44575663783405));
#51155=CARTESIAN_POINT('Ctrl Pts',(64.6949458653977,-2.40940335486022,3.55689452840209));
#51156=CARTESIAN_POINT('Ctrl Pts',(66.8588310559543,-1.56301940386928,3.66803241897013));
#51157=CARTESIAN_POINT('Ctrl Pts',(67.3213071004237,0.714013933333857,3.77917030953817));
#51158=CARTESIAN_POINT('Ctrl Pts',(65.6590644304509,2.33750221987791,3.89030820010621));
#51159=CARTESIAN_POINT('Ctrl Pts',(63.39357261301,1.82144821550899,4.00144609067426));
#51160=CARTESIAN_POINT('Ctrl Pts',(62.5984620009619,-0.361797997181331,
4.1125839812423));
#51161=CARTESIAN_POINT('Ctrl Pts',(64.0015063548152,-2.21388639990766,4.22372187181034));
#51162=CARTESIAN_POINT('Ctrl Pts',(66.3184832656195,-2.03957947376811,4.33485976237838));
#51163=CARTESIAN_POINT('Ctrl Pts',(67.4286374911296,0.00157767540964959,
4.44599765294642));
#51164=CARTESIAN_POINT('Ctrl Pts',(66.3158322777071,2.04129075981349,4.55713554351446));
#51165=CARTESIAN_POINT('Ctrl Pts',(63.9986308592856,2.21258726309085,4.66827343408251));
#51166=CARTESIAN_POINT('Ctrl Pts',(62.5979939690176,0.358677549762036,4.77941132465055));
#51167=CARTESIAN_POINT('Ctrl Pts',(63.3959404447162,-1.82353378810157,4.89054921521859));
#51168=CARTESIAN_POINT('Ctrl Pts',(65.6621008123707,-2.33664397819607,5.00168710578663));
#51169=CARTESIAN_POINT('Ctrl Pts',(67.3222328179754,-0.710997418429188,
5.11282499635466));
#51170=CARTESIAN_POINT('Ctrl Pts',(66.8567987494513,1.56543310762405,5.22396288692272));
#51171=CARTESIAN_POINT('Ctrl Pts',(64.6918158067503,2.4090050242139,5.33510077749075));
#51172=CARTESIAN_POINT('Ctrl Pts',(62.8089171959401,1.04758718972752,5.4462386680588));
#51173=CARTESIAN_POINT('Ctrl Pts',(62.931541830362,-1.27269881881276,5.55737655862684));
#51174=CARTESIAN_POINT('Ctrl Pts',(64.9474490817621,-2.42806968006158,5.66851444919488));
#51175=CARTESIAN_POINT('Ctrl Pts',(67.0114579748176,-1.36099981154567,5.77965233976292));
#51176=CARTESIAN_POINT('Ctrl Pts',(67.234354225073,0.951806616989214,5.89079023033096));
#51177=CARTESIAN_POINT('Ctrl Pts',(65.4121253417219,2.39341760299657,6.001928120899));
#51178=CARTESIAN_POINT('Ctrl Pts',(63.2126643336617,1.64429852840487,6.11306601146706));
#51179=CARTESIAN_POINT('Ctrl Pts',(62.649189925264,-0.609850285121809,6.22420390203508));
#51180=CARTESIAN_POINT('Ctrl Pts',(64.2374031554985,-2.30582648807954,6.33534179260314));
#51181=CARTESIAN_POINT('Ctrl Pts',(66.5236998933488,-1.89119386508314,6.44647968317117));
#51182=CARTESIAN_POINT('Ctrl Pts',(67.4151988715152,0.25435224605703,6.55761757373922));
#51183=CARTESIAN_POINT('Ctrl Pts',(66.0963109962835,2.16731896239629,6.66875546430726));
#51184=CARTESIAN_POINT('Ctrl Pts',(63.7734206371606,2.09605634078856,6.77989335487529));
#51185=CARTESIAN_POINT('Ctrl Pts',(62.5742917867301,0.107152602938506,6.89103124544335));
#51186=CARTESIAN_POINT('Ctrl Pts',(63.5933356141608,-1.98161526205798,7.00216913601138));
#51187=CARTESIAN_POINT('Ctrl Pts',(65.9042541560964,-2.25300237548895,7.11330702657943));
#51188=CARTESIAN_POINT('Ctrl Pts',(66.8857543436368,-1.06431345694511,7.18739895362479));
#51189=CARTESIAN_POINT('Ctrl Pts',(67.0166758614465,-0.393720754290184,
7.22444491714747));
#51190=CARTESIAN_POINT('Ctrl Pts',(65.4967348970877,-1.85997880000276,-2.07481497238249));
#51191=CARTESIAN_POINT('Ctrl Pts',(66.1152220988337,-1.69480262890398,-2.03776900885981));
#51192=CARTESIAN_POINT('Ctrl Pts',(67.1637217267118,-0.701476540869014,
-1.96367708181445));
#51193=CARTESIAN_POINT('Ctrl Pts',(66.7625611820115,1.4413553150263,-1.8525391912464));
#51194=CARTESIAN_POINT('Ctrl Pts',(64.7450334117317,2.26061368566345,-1.74140130067836));
#51195=CARTESIAN_POINT('Ctrl Pts',(62.962414682697,1.01278889075625,-1.63026341011032));
#51196=CARTESIAN_POINT('Ctrl Pts',(63.0440444094189,-1.16310107509048,-1.51912551954228));
#51197=CARTESIAN_POINT('Ctrl Pts',(64.9163760764189,-2.27386063817902,-1.40798762897424));
#51198=CARTESIAN_POINT('Ctrl Pts',(66.8650500736736,-1.30359889821863,-1.2968497384062));
#51199=CARTESIAN_POINT('Ctrl Pts',(67.1067238075328,0.859998174993211,-1.18571184783815));
#51200=CARTESIAN_POINT('Ctrl Pts',(65.4200380164786,2.2363599535264,-1.07457395727011));
#51201=CARTESIAN_POINT('Ctrl Pts',(63.3489126975537,1.56579120426538,-0.963436066702071));
#51202=CARTESIAN_POINT('Ctrl Pts',(62.7890331093795,-0.53798179177636,-0.85229817613403));
#51203=CARTESIAN_POINT('Ctrl Pts',(64.2528832853252,-2.1493249255815,-0.741160285565987));
#51204=CARTESIAN_POINT('Ctrl Pts',(66.4005744678012,-1.79337115794136,-0.630022394997947));
#51205=CARTESIAN_POINT('Ctrl Pts',(67.2663056781698,0.204077890402244,-0.518884504429904));
#51206=CARTESIAN_POINT('Ctrl Pts',(66.0576607264394,2.014730953885,-0.407746613861862));
#51207=CARTESIAN_POINT('Ctrl Pts',(63.8809273599474,1.98127852376002,-0.296608723293821));
#51208=CARTESIAN_POINT('Ctrl Pts',(62.7284936474651,0.134339088808407,-0.185470832725779));
#51209=CARTESIAN_POINT('Ctrl Pts',(63.6551955739828,-1.83556228407719,-0.0743329421577371));
#51210=CARTESIAN_POINT('Ctrl Pts',(65.8128121849957,-2.12535275953085,0.0368049484103043));
#51211=CARTESIAN_POINT('Ctrl Pts',(67.2264526144558,-0.469783711552737,
0.147942838978346));
#51212=CARTESIAN_POINT('Ctrl Pts',(66.6021957013601,1.61578367529074,0.259080729546388));
#51213=CARTESIAN_POINT('Ctrl Pts',(64.5114309002076,2.22240595006455,0.37021862011443));
#51214=CARTESIAN_POINT('Ctrl Pts',(62.8678589330251,0.794834849795578,0.481356510682471));
#51215=CARTESIAN_POINT('Ctrl Pts',(63.1758598665065,-1.36025759991931,0.592494401250513));
#51216=CARTESIAN_POINT('Ctrl Pts',(65.153516950348,-2.27029084338243,0.703632291818555));
#51217=CARTESIAN_POINT('Ctrl Pts',(66.9906582290337,-1.10230113037647,0.814770182386596));
#51218=CARTESIAN_POINT('Ctrl Pts',(67.0057274548323,1.07463730786742,0.925908072954638));
#51219=CARTESIAN_POINT('Ctrl Pts',(65.1849315948547,2.26794803117707,1.03704596352268));
#51220=CARTESIAN_POINT('Ctrl Pts',(63.1948657487746,1.38538020118272,1.14818385409072));
#51221=CARTESIAN_POINT('Ctrl Pts',(62.8570597544889,-0.765241838189804,
1.25932174465876));
#51222=CARTESIAN_POINT('Ctrl Pts',(64.480711269498,-2.21542934465704,1.37045963522681));
#51223=CARTESIAN_POINT('Ctrl Pts',(66.5796736486789,-1.63780924727066,1.48159752579485));
#51224=CARTESIAN_POINT('Ctrl Pts',(67.232742822502,0.438916228156908,1.59273541636289));
#51225=CARTESIAN_POINT('Ctrl Pts',(65.8421571698655,2.11389670230683,1.70387330693093));
#51226=CARTESIAN_POINT('Ctrl Pts',(63.680735508938,1.8540035516147,1.81501119749897));
#51227=CARTESIAN_POINT('Ctrl Pts',(62.7268515981571,-0.102880075699926,
1.92614908806701));
#51228=CARTESIAN_POINT('Ctrl Pts',(63.8536061988389,-1.96559640298738,2.03728697863505));
#51229=CARTESIAN_POINT('Ctrl Pts',(66.0296680467136,-2.02918005124096,2.1484248692031));
#51230=CARTESIAN_POINT('Ctrl Pts',(67.2632630542012,-0.23543218612684,2.25956275977114));
#51231=CARTESIAN_POINT('Ctrl Pts',(66.42526772103,1.77380942893181,2.37070065033918));
#51232=CARTESIAN_POINT('Ctrl Pts',(64.2827086791644,2.15946315732203,2.48183854090722));
#51233=CARTESIAN_POINT('Ctrl Pts',(62.7966945178967,0.568535767837554,2.59297643147526));
#51234=CARTESIAN_POINT('Ctrl Pts',(63.3273908515816,-1.54277885758279,2.7041143220433));
#51235=CARTESIAN_POINT('Ctrl Pts',(65.3890453074919,-2.24197049835535,2.81525221261135));
#51236=CARTESIAN_POINT('Ctrl Pts',(67.0946021813807,-0.889061116308551,
2.92639010317939));
#51237=CARTESIAN_POINT('Ctrl Pts',(66.8829459242478,1.27761598813437,3.03752799374744));
#51238=CARTESIAN_POINT('Ctrl Pts',(64.9478079085913,2.27487668948697,3.14866588431547));
#51239=CARTESIAN_POINT('Ctrl Pts',(63.0604419061002,1.18991695809612,3.25980377488352));
#51240=CARTESIAN_POINT('Ctrl Pts',(62.9483754230397,-0.98418725961686,3.37094166545155));
#51241=CARTESIAN_POINT('Ctrl Pts',(64.7141841822776,-2.25745371715865,3.4820795560196));
#51242=CARTESIAN_POINT('Ctrl Pts',(66.7416034008459,-1.46444718612111,3.59321744658764));
#51243=CARTESIAN_POINT('Ctrl Pts',(67.1749132754993,0.668984462338435,3.70435533715568));
#51244=CARTESIAN_POINT('Ctrl Pts',(65.6175003638835,2.19008704561056,3.81549322772372));
#51245=CARTESIAN_POINT('Ctrl Pts',(63.4948823662959,1.70657811877717,3.92663111829177));
#51246=CARTESIAN_POINT('Ctrl Pts',(62.7499156079905,-0.338981114121067,
4.0377690088598));
#51247=CARTESIAN_POINT('Ctrl Pts',(64.0644766114669,-2.07426708888619,4.14890689942785));
#51248=CARTESIAN_POINT('Ctrl Pts',(66.2353327818609,-1.91095287354467,4.26004478999589));
#51249=CARTESIAN_POINT('Ctrl Pts',(67.2754748477136,0.00147817890715481,
4.37118268056393));
#51250=CARTESIAN_POINT('Ctrl Pts',(66.2328489791779,1.9125562368987,4.48232057113198));
#51251=CARTESIAN_POINT('Ctrl Pts',(64.061782459797,2.0730498824644,4.59345846170001));
#51252=CARTESIAN_POINT('Ctrl Pts',(62.7494770926002,0.336057458514928,4.70459635226806));
#51253=CARTESIAN_POINT('Ctrl Pts',(63.4971008700911,-1.70853216420175,4.8157342428361));
#51254=CARTESIAN_POINT('Ctrl Pts',(65.6203452556023,-2.18928292915949,4.92687213340414));
#51255=CARTESIAN_POINT('Ctrl Pts',(67.1757806124374,-0.666158184716354,
5.03801002397218));
#51256=CARTESIAN_POINT('Ctrl Pts',(66.7396992622713,1.46670866903236,5.14914791454023));
#51257=CARTESIAN_POINT('Ctrl Pts',(64.7112515215779,2.25708050733624,5.26028580510827));
#51258=CARTESIAN_POINT('Ctrl Pts',(62.9470983923676,0.981520836155458,5.3714236956763));
#51259=CARTESIAN_POINT('Ctrl Pts',(63.0619896729133,-1.19243574288082,5.48256158624435));
#51260=CARTESIAN_POINT('Ctrl Pts',(64.9507632188372,-2.27494284579562,5.59369947681239));
#51261=CARTESIAN_POINT('Ctrl Pts',(66.8846048641049,-1.27516801096354,5.70483736738043));
#51262=CARTESIAN_POINT('Ctrl Pts',(67.093444105432,0.891780689689939,5.81597525794848));
#51263=CARTESIAN_POINT('Ctrl Pts',(65.3861345518294,2.24247611081748,5.92711314851652));
#51264=CARTESIAN_POINT('Ctrl Pts',(63.3253831137711,1.54060042191708,6.03825103908456));
#51265=CARTESIAN_POINT('Ctrl Pts',(62.7974443627954,-0.571389921194146,
6.1493889296526));
#51266=CARTESIAN_POINT('Ctrl Pts',(64.2854965201902,-2.16040895192495,6.26052682022064));
#51267=CARTESIAN_POINT('Ctrl Pts',(66.4276073705699,-1.77192524115467,6.37166471078868));
#51268=CARTESIAN_POINT('Ctrl Pts',(67.2628837380762,0.238311456722616,6.48280260135673));
#51269=CARTESIAN_POINT('Ctrl Pts',(66.0271718634116,2.03063643871027,6.59394049192476));
#51270=CARTESIAN_POINT('Ctrl Pts',(63.8507751778273,1.96386801252778,6.70507838249281));
#51271=CARTESIAN_POINT('Ctrl Pts',(62.7272696944899,0.100394996677835,6.81621627306085));
#51272=CARTESIAN_POINT('Ctrl Pts',(63.6820472627792,-1.85664418964446,6.92735416362889));
#51273=CARTESIAN_POINT('Ctrl Pts',(65.8472271368835,-2.11091620548103,7.03849205419694));
#51274=CARTESIAN_POINT('Ctrl Pts',(66.7668287645171,-0.997192257060707,
7.1125839812423));
#51275=CARTESIAN_POINT('Ctrl Pts',(66.8894936833815,-0.368890654402881,
7.14962994476498));
#51276=CARTESIAN_POINT('Ctrl Pts',(65.4632995769868,-1.7347832743338,-2.14962994476498));
#51277=CARTESIAN_POINT('Ctrl Pts',(66.0401562879218,-1.58072514262809,-2.1125839812423));
#51278=CARTESIAN_POINT('Ctrl Pts',(67.0180812070583,-0.654260021907395,
-2.03849205419694));
#51279=CARTESIAN_POINT('Ctrl Pts',(66.6439228546792,1.3443374154996,-1.92735416362889));
#51280=CARTESIAN_POINT('Ctrl Pts',(64.7621952611282,2.10845134988271,-1.81621627306085));
#51281=CARTESIAN_POINT('Ctrl Pts',(63.0995649367186,0.944617878500777,-1.70507838249281));
#51282=CARTESIAN_POINT('Ctrl Pts',(63.1757001510583,-1.08481252120918,-1.59394049192477));
#51283=CARTESIAN_POINT('Ctrl Pts',(64.9220048185698,-2.12080664751291,-1.48280260135673));
#51284=CARTESIAN_POINT('Ctrl Pts',(66.7395131996123,-1.21585340922504,-1.37166471078869));
#51285=CARTESIAN_POINT('Ctrl Pts',(66.9649198286257,0.802111534783946,-1.26052682022064));
#51286=CARTESIAN_POINT('Ctrl Pts',(65.3917651779528,2.08583014105416,-1.1493889296526));
#51287=CARTESIAN_POINT('Ctrl Pts',(63.4600476969176,1.4603975014417,-1.03825103908456));
#51288=CARTESIAN_POINT('Ctrl Pts',(62.9378537099731,-0.501770135373788,
-0.927113148516519));
#51289=CARTESIAN_POINT('Ctrl Pts',(64.3031718530388,-2.00465345734156,-0.815975257948477));
#51290=CARTESIAN_POINT('Ctrl Pts',(66.306301534833,-1.67265900528796,-0.704837367380435));
#51291=CARTESIAN_POINT('Ctrl Pts',(67.1137602132943,0.190341368907332,-0.593699476812392));
#51292=CARTESIAN_POINT('Ctrl Pts',(65.9864693824166,1.87911903139815,-0.482561586244352));
#51293=CARTESIAN_POINT('Ctrl Pts',(63.9562523515188,1.84791829068726,-0.371423695676309));
#51294=CARTESIAN_POINT('Ctrl Pts',(62.8813891707182,0.125296699270833,-0.260285805108269));
#51295=CARTESIAN_POINT('Ctrl Pts',(63.7457146148648,-1.71201023872441,-0.149147914540226));
#51296=CARTESIAN_POINT('Ctrl Pts',(65.7581016427195,-1.98229486233275,-0.0380100239721847));
#51297=CARTESIAN_POINT('Ctrl Pts',(67.0765896668548,-0.438162480859964,
0.0731278665958569));
#51298=CARTESIAN_POINT('Ctrl Pts',(66.4943516049349,1.50702496976408,0.184265757163899));
#51299=CARTESIAN_POINT('Ctrl Pts',(64.5443165789444,2.07281538421093,0.295403647731941));
#51300=CARTESIAN_POINT('Ctrl Pts',(63.0113737524843,0.741334365359939,0.406541538299983));
#51301=CARTESIAN_POINT('Ctrl Pts',(63.298643084738,-1.2686984029721,0.517679428868024));
#51302=CARTESIAN_POINT('Ctrl Pts',(65.1431836953141,-2.11747713628089,0.628817319436066));
#51303=CARTESIAN_POINT('Ctrl Pts',(66.8566666462206,-1.02810503230118,0.739955210004107));
#51304=CARTESIAN_POINT('Ctrl Pts',(66.8707215595737,1.0023032669301,0.851093100572149));
#51305=CARTESIAN_POINT('Ctrl Pts',(65.1724838141431,2.11529201920926,0.96223099114019));
#51306=CARTESIAN_POINT('Ctrl Pts',(63.3163696774672,1.29212999718137,1.07336888170823));
#51307=CARTESIAN_POINT('Ctrl Pts',(63.0013014687028,-0.713733264976008,
1.18450677227627));
#51308=CARTESIAN_POINT('Ctrl Pts',(64.5156646924021,-2.06630837543612,1.29564466284432));
#51309=CARTESIAN_POINT('Ctrl Pts',(66.4733455158896,-1.52756799631811,1.40678255341236));
#51310=CARTESIAN_POINT('Ctrl Pts',(67.0824564798048,0.409372693623795,1.5179204439804));
#51311=CARTESIAN_POINT('Ctrl Pts',(65.7854714110939,1.97160991449248,1.62905833454844));
#51312=CARTESIAN_POINT('Ctrl Pts',(63.7695354519561,1.72921022104761,1.74019622511648));
#51313=CARTESIAN_POINT('Ctrl Pts',(62.8798576480604,-0.095955198299122,
1.85133411568453));
#51314=CARTESIAN_POINT('Ctrl Pts',(63.9307701829444,-1.83329173643707,1.96247200625256));
#51315=CARTESIAN_POINT('Ctrl Pts',(65.9603608952703,-1.89259555727162,2.07360989682061));
#51316=CARTESIAN_POINT('Ctrl Pts',(67.110922388922,-0.219585201042117,2.18474778738865));
#51317=CARTESIAN_POINT('Ctrl Pts',(66.3293326805052,1.65441397996683,2.29588567795669));
#51318=CARTESIAN_POINT('Ctrl Pts',(64.330989693964,2.01410928278149,2.40702356852474));
#51319=CARTESIAN_POINT('Ctrl Pts',(62.9449994276305,0.530267517513453,2.51816145909277));
#51320=CARTESIAN_POINT('Ctrl Pts',(63.4399744904782,-1.43893412017732,2.62929934966082));
#51321=CARTESIAN_POINT('Ctrl Pts',(65.362858594084,-2.09106303904695,2.74043724022886));
#51322=CARTESIAN_POINT('Ctrl Pts',(66.953614111428,-0.829218244009191,2.8515751307969));
#51323=CARTESIAN_POINT('Ctrl Pts',(66.7562044770915,1.19161941374475,2.96271302136494));
#51324=CARTESIAN_POINT('Ctrl Pts',(64.9513209681592,2.12175430821469,3.07385091193298));
#51325=CARTESIAN_POINT('Ctrl Pts',(63.1909939291292,1.10982342204558,3.18498880250103));
#51326=CARTESIAN_POINT('Ctrl Pts',(63.0864706622905,-0.917941428576071,
3.29612669306907));
#51327=CARTESIAN_POINT('Ctrl Pts',(64.7334224991575,-2.10550407945708,3.40726458363711));
#51328=CARTESIAN_POINT('Ctrl Pts',(66.6243757457373,-1.36587496837293,3.51840247420515));
#51329=CARTESIAN_POINT('Ctrl Pts',(67.0285194505751,0.623954991343011,3.6295403647732));
#51330=CARTESIAN_POINT('Ctrl Pts',(65.5759362973161,2.0426718713432,3.74067825534123));
#51331=CARTESIAN_POINT('Ctrl Pts',(63.5961921195818,1.59170802204535,3.85181614590928));
#51332=CARTESIAN_POINT('Ctrl Pts',(62.9013692150191,-0.316164231060802,
3.96295403647732));
#51333=CARTESIAN_POINT('Ctrl Pts',(64.1274468681187,-1.93464777786472,4.07409192704536));
#51334=CARTESIAN_POINT('Ctrl Pts',(66.1521822981021,-1.78232627332123,4.1852298176134));
#51335=CARTESIAN_POINT('Ctrl Pts',(67.1223122042977,0.00137868240466034,
4.29636770818144));
#51336=CARTESIAN_POINT('Ctrl Pts',(66.1498656806486,1.78382171398391,4.40750559874948));
#51337=CARTESIAN_POINT('Ctrl Pts',(64.1249340603086,1.93351250183796,4.51864348931753));
#51338=CARTESIAN_POINT('Ctrl Pts',(62.9009602161829,0.31343736726782,4.62978137988557));
#51339=CARTESIAN_POINT('Ctrl Pts',(63.5982612954659,-1.59353054030193,4.74091927045361));
#51340=CARTESIAN_POINT('Ctrl Pts',(65.578589698834,-2.04192188012291,4.85205716102165));
#51341=CARTESIAN_POINT('Ctrl Pts',(67.0293284068993,-0.621318951003518,
4.96319505158969));
#51342=CARTESIAN_POINT('Ctrl Pts',(66.6225997750914,1.36798423044066,5.07433294215773));
#51343=CARTESIAN_POINT('Ctrl Pts',(64.7306872364055,2.10515599045857,5.18547083272578));
#51344=CARTESIAN_POINT('Ctrl Pts',(63.0852795887951,0.915454482583398,5.29660872329381));
#51345=CARTESIAN_POINT('Ctrl Pts',(63.1924375154646,-1.11217266694888,5.40774661386187));
#51346=CARTESIAN_POINT('Ctrl Pts',(64.9540773559123,-2.12181601152966,5.5188845044299));
#51347=CARTESIAN_POINT('Ctrl Pts',(66.7577517533922,-1.18933621038142,5.63002239499795));
#51348=CARTESIAN_POINT('Ctrl Pts',(66.9525339857911,0.831754762390664,5.74116028556598));
#51349=CARTESIAN_POINT('Ctrl Pts',(65.360143761937,2.0915346186384,5.85229817613403));
#51350=CARTESIAN_POINT('Ctrl Pts',(63.4381018938805,1.43690231542928,5.96343606670207));
#51351=CARTESIAN_POINT('Ctrl Pts',(62.9456988003269,-0.532929557266482,
6.0745739572701));
#51352=CARTESIAN_POINT('Ctrl Pts',(64.3335898848817,-2.01499141577036,6.18571184783816));
#51353=CARTESIAN_POINT('Ctrl Pts',(66.3315148477911,-1.6526566172262,6.29684973840619));
#51354=CARTESIAN_POINT('Ctrl Pts',(67.1105686046372,0.2222706673882,6.40798762897424));
#51355=CARTESIAN_POINT('Ctrl Pts',(65.9580327305397,1.89395391502425,6.51912551954227));
#51356=CARTESIAN_POINT('Ctrl Pts',(63.9281297184939,1.83167968426699,6.63026341011033));
#51357=CARTESIAN_POINT('Ctrl Pts',(62.8802476022497,0.0936373904171628,
6.74140130067836));
#51358=CARTESIAN_POINT('Ctrl Pts',(63.7707589113974,-1.73167311723094,6.85253919124641));
#51359=CARTESIAN_POINT('Ctrl Pts',(65.7902001176707,-1.96883003547311,6.96367708181445));
#51360=CARTESIAN_POINT('Ctrl Pts',(66.6479031853974,-0.930071057176307,
7.03776900885981));
#51361=CARTESIAN_POINT('Ctrl Pts',(66.7623115053165,-0.344060554515578,
7.07481497238249));
#51362=CARTESIAN_POINT('Ctrl Pts',(65.4298642568859,-1.60958774866484,-2.22444491714747));
#51363=CARTESIAN_POINT('Ctrl Pts',(65.9650904770099,-1.4666476563522,-2.18739895362479));
#51364=CARTESIAN_POINT('Ctrl Pts',(66.8724406874047,-0.607043502945776,
-2.11330702657942));
#51365=CARTESIAN_POINT('Ctrl Pts',(66.5252845273471,1.2473195159729,-2.00216913601139));
#51366=CARTESIAN_POINT('Ctrl Pts',(64.7793571105247,1.95628901410197,-1.89103124544334));
#51367=CARTESIAN_POINT('Ctrl Pts',(63.2367151907402,0.876446866245303,-1.7798933548753));
#51368=CARTESIAN_POINT('Ctrl Pts',(63.3073558926977,-1.00652396732789,-1.66875546430726));
#51369=CARTESIAN_POINT('Ctrl Pts',(64.9276335607206,-1.9677526568468,-1.55761757373922));
#51370=CARTESIAN_POINT('Ctrl Pts',(66.6139763255511,-1.12810792023144,-1.44647968317117));
#51371=CARTESIAN_POINT('Ctrl Pts',(66.8231158497185,0.74422489457468,-1.33534179260313));
#51372=CARTESIAN_POINT('Ctrl Pts',(65.363492339427,1.93530032858193,-1.22420390203509));
#51373=CARTESIAN_POINT('Ctrl Pts',(63.5711826962814,1.35500379861802,-1.11306601146705));
#51374=CARTESIAN_POINT('Ctrl Pts',(63.0866743105668,-0.465558478971215,
-1.00192812089901));
#51375=CARTESIAN_POINT('Ctrl Pts',(64.3534604207524,-1.85998198910161,-0.890790230330965));
#51376=CARTESIAN_POINT('Ctrl Pts',(66.2120286018649,-1.55194685263456,-0.779652339762925));
#51377=CARTESIAN_POINT('Ctrl Pts',(66.9612147484188,0.176604847412417,-0.668514449194881));
#51378=CARTESIAN_POINT('Ctrl Pts',(65.915278038394,1.7435071089113,-0.55737655862684));
#51379=CARTESIAN_POINT('Ctrl Pts',(64.0315773430901,1.7145580576145,-0.446238668058799));
#51380=CARTESIAN_POINT('Ctrl Pts',(63.0342846939712,0.116254309733256,-0.335100777490757));
#51381=CARTESIAN_POINT('Ctrl Pts',(63.8362336557469,-1.58845819337162,-0.223962886922715));
#51382=CARTESIAN_POINT('Ctrl Pts',(65.703391100443,-1.83923696513465,-0.112824996354674));
#51383=CARTESIAN_POINT('Ctrl Pts',(66.9267267192538,-0.406541250167187,
-0.00168710578663183));
#51384=CARTESIAN_POINT('Ctrl Pts',(66.3865075085097,1.39826626423741,0.10945078478141));
#51385=CARTESIAN_POINT('Ctrl Pts',(64.5772022576811,1.92322481835731,0.220588675349452));
#51386=CARTESIAN_POINT('Ctrl Pts',(63.1548885719436,0.687833880924302,0.331726565917493));
#51387=CARTESIAN_POINT('Ctrl Pts',(63.4214263029693,-1.17713920602489,0.442864456485535));
#51388=CARTESIAN_POINT('Ctrl Pts',(65.1328504402804,-1.96466342917936,0.554002347053577));
#51389=CARTESIAN_POINT('Ctrl Pts',(66.7226750634076,-0.953908934225886,
0.665140237621619));
#51390=CARTESIAN_POINT('Ctrl Pts',(66.7357156643151,0.929969225992789,0.77627812818966));
#51391=CARTESIAN_POINT('Ctrl Pts',(65.1600360334315,1.96263600724145,0.887416018757702));
#51392=CARTESIAN_POINT('Ctrl Pts',(63.4378736061597,1.19887979318003,0.998553909325744));
#51393=CARTESIAN_POINT('Ctrl Pts',(63.1455431829167,-0.66222469176221,1.10969179989378));
#51394=CARTESIAN_POINT('Ctrl Pts',(64.5506181153062,-1.9171874062152,1.22082969046183));
#51395=CARTESIAN_POINT('Ctrl Pts',(66.3670173831005,-1.41732674536556,1.33196758102987));
#51396=CARTESIAN_POINT('Ctrl Pts',(66.9321701371076,0.379829159090682,1.44310547159791));
#51397=CARTESIAN_POINT('Ctrl Pts',(65.7287856523224,1.82932312667812,1.55424336216595));
#51398=CARTESIAN_POINT('Ctrl Pts',(63.858335394974,1.60441689048052,1.66538125273399));
#51399=CARTESIAN_POINT('Ctrl Pts',(63.0328636979636,-0.0890303208983184,
1.77651914330204));
#51400=CARTESIAN_POINT('Ctrl Pts',(64.00793416705,-1.70098706988675,1.88765703387008));
#51401=CARTESIAN_POINT('Ctrl Pts',(65.8910537438272,-1.75601106330228,1.99879492443812));
#51402=CARTESIAN_POINT('Ctrl Pts',(66.9585817236427,-0.203738215957396,
2.10993281500616));
#51403=CARTESIAN_POINT('Ctrl Pts',(66.2333976399805,1.53501853100185,2.2210707055742));
#51404=CARTESIAN_POINT('Ctrl Pts',(64.3792707087636,1.86875540824094,2.33220859614224));
#51405=CARTESIAN_POINT('Ctrl Pts',(63.0933043373643,0.491999267189351,2.44334648671029));
#51406=CARTESIAN_POINT('Ctrl Pts',(63.5525581293749,-1.33508938277185,2.55448437727833));
#51407=CARTESIAN_POINT('Ctrl Pts',(65.336671880676,-1.94015557973856,2.66562226784637));
#51408=CARTESIAN_POINT('Ctrl Pts',(66.8126260414754,-0.76937537170983,2.77676015841441));
#51409=CARTESIAN_POINT('Ctrl Pts',(66.6294630299351,1.10562283935513,2.88789804898245));
#51410=CARTESIAN_POINT('Ctrl Pts',(64.9548340277273,1.96863192694241,2.9990359395505));
#51411=CARTESIAN_POINT('Ctrl Pts',(63.3215459521581,1.02972988599504,3.11017383011853));
#51412=CARTESIAN_POINT('Ctrl Pts',(63.2245659015414,-0.851695597535288,
3.22131172068658));
#51413=CARTESIAN_POINT('Ctrl Pts',(64.7526608160373,-1.95355444175551,3.33244961125462));
#51414=CARTESIAN_POINT('Ctrl Pts',(66.507148090629,-1.26730275062476,3.44358750182267));
#51415=CARTESIAN_POINT('Ctrl Pts',(66.8821256256507,0.578925520347588,3.5547253923907));
#51416=CARTESIAN_POINT('Ctrl Pts',(65.5343722307488,1.89525669707585,3.66586328295875));
#51417=CARTESIAN_POINT('Ctrl Pts',(63.6975018728676,1.47683792531353,3.77700117352679));
#51418=CARTESIAN_POINT('Ctrl Pts',(63.0528228220477,-0.293347348000536,
3.88813906409483));
#51419=CARTESIAN_POINT('Ctrl Pts',(64.1904171247705,-1.79502846684324,3.99927695466287));
#51420=CARTESIAN_POINT('Ctrl Pts',(66.0690318143434,-1.65369967309779,4.11041484523092));
#51421=CARTESIAN_POINT('Ctrl Pts',(66.9691495608818,0.00127918590216747,
4.22155273579895));
#51422=CARTESIAN_POINT('Ctrl Pts',(66.0668823821194,1.65508719106912,4.332690626367));
#51423=CARTESIAN_POINT('Ctrl Pts',(64.18808566082,1.79397512121151,4.44382851693503));
#51424=CARTESIAN_POINT('Ctrl Pts',(63.0524433397656,0.290817276020709,4.55496640750308));
#51425=CARTESIAN_POINT('Ctrl Pts',(63.6994217208406,-1.4785289164021,4.66610429807112));
#51426=CARTESIAN_POINT('Ctrl Pts',(65.5368341420657,-1.89456083108634,4.77724218863916));
#51427=CARTESIAN_POINT('Ctrl Pts',(66.8828762013613,-0.576479717290682,
4.88838007920721));
#51428=CARTESIAN_POINT('Ctrl Pts',(66.5055002879113,1.26925979184897,4.99951796977524));
#51429=CARTESIAN_POINT('Ctrl Pts',(64.750122951233,1.9532314735809,5.11065586034329));
#51430=CARTESIAN_POINT('Ctrl Pts',(63.2234607852226,0.849388129011338,5.22179375091133));
#51431=CARTESIAN_POINT('Ctrl Pts',(63.3228853580158,-1.03190959101694,5.33293164147937));
#51432=CARTESIAN_POINT('Ctrl Pts',(64.9573914929873,-1.9686891772637,5.44406953204742));
#51433=CARTESIAN_POINT('Ctrl Pts',(66.6308986426796,-1.10350440979929,5.55520742261545));
#51434=CARTESIAN_POINT('Ctrl Pts',(66.8116238661501,0.771728835091389,5.6663453131835));
#51435=CARTESIAN_POINT('Ctrl Pts',(65.3341529720446,1.94059312645932,5.77748320375153));
#51436=CARTESIAN_POINT('Ctrl Pts',(63.5508206739898,1.33320420894149,5.88862109431959));
#51437=CARTESIAN_POINT('Ctrl Pts',(63.0939532378584,-0.494469193338818,
5.99975898488762));
#51438=CARTESIAN_POINT('Ctrl Pts',(64.3816832495733,-1.86957387961577,6.11089687545566));
#51439=CARTESIAN_POINT('Ctrl Pts',(66.2354223250123,-1.53338799329773,6.22203476602371));
#51440=CARTESIAN_POINT('Ctrl Pts',(66.9582534711982,0.206229878053785,6.33317265659175));
#51441=CARTESIAN_POINT('Ctrl Pts',(65.8888935976679,1.75727139133823,6.44431054715979));
#51442=CARTESIAN_POINT('Ctrl Pts',(64.0054842591604,1.6994913560062,6.55544843772783));
#51443=CARTESIAN_POINT('Ctrl Pts',(63.0332255100096,0.0868797841564908,
6.66658632829588));
#51444=CARTESIAN_POINT('Ctrl Pts',(63.8594705600156,-1.60670204481742,6.77772421886391));
#51445=CARTESIAN_POINT('Ctrl Pts',(65.7331730984579,-1.82674386546519,6.88886210943197));
#51446=CARTESIAN_POINT('Ctrl Pts',(66.5289776062776,-0.862949857291908,
6.96295403647732));
#51447=CARTESIAN_POINT('Ctrl Pts',(66.6351293272515,-0.319230454628274,
7.));
#51448=CARTESIAN_POINT('Ctrl Pts',(66.6638321395092,0.000941642735149761,
-1.3785196366098));
#51449=CARTESIAN_POINT('Ctrl Pts',(66.664949390616,0.216825623511906,-1.36412702194091));
#51450=CARTESIAN_POINT('Ctrl Pts',(66.625958965974,0.432322760104845,-1.34973440727202));
#51451=CARTESIAN_POINT('Ctrl Pts',(66.5449886773087,0.630681997774868,-1.33534179260313));
#51452=CARTESIAN_POINT('Ctrl Pts',(66.3365746796213,1.14125003924376,-1.29829582908045));
#51453=CARTESIAN_POINT('Ctrl Pts',(65.8500335095242,1.53827518391285,-1.26124986555777));
#51454=CARTESIAN_POINT('Ctrl Pts',(65.308044650618,1.64007166792007,-1.22420390203509));
#51455=CARTESIAN_POINT('Ctrl Pts',(64.7660557917118,1.74186815192729,-1.18715793851241));
#51456=CARTESIAN_POINT('Ctrl Pts',(64.1686192439966,1.54843597527265,-1.15011197498973));
#51457=CARTESIAN_POINT('Ctrl Pts',(63.7891495725199,1.14829284068046,-1.11306601146705));
#51458=CARTESIAN_POINT('Ctrl Pts',(63.4096799010432,0.748149706088272,-1.07602004794437));
#51459=CARTESIAN_POINT('Ctrl Pts',(63.248177105805,0.141295613558526,-1.03897408442169));
#51460=CARTESIAN_POINT('Ctrl Pts',(63.3785567265502,-0.394535351061412,
-1.00192812089901));
#51461=CARTESIAN_POINT('Ctrl Pts',(63.5089363472953,-0.93036631568135,-0.964882157376327));
#51462=CARTESIAN_POINT('Ctrl Pts',(63.9311983840238,-1.39517415239148,-0.927836193853646));
#51463=CARTESIAN_POINT('Ctrl Pts',(64.4520907659069,-1.57623888133537,-0.890790230330965));
#51464=CARTESIAN_POINT('Ctrl Pts',(64.9729831477899,-1.75730361027926,-0.853744266808285));
#51465=CARTESIAN_POINT('Ctrl Pts',(65.5925058748274,-1.65462523145691,-0.816698303285605));
#51466=CARTESIAN_POINT('Ctrl Pts',(66.0271315961051,-1.31519409203791,-0.779652339762925));
#51467=CARTESIAN_POINT('Ctrl Pts',(66.422630141453,-1.0063202373306,-0.745941438711882));
#51468=CARTESIAN_POINT('Ctrl Pts',(66.6650238854461,-0.501402189087533,
-0.712230537660838));
#51469=CARTESIAN_POINT('Ctrl Pts',(66.6681941903091,0.000864019930038266,
-0.678519636609795));
#51470=CARTESIAN_POINT('Ctrl Pts',(65.5301702171886,-1.98517432567172,-2.));
#51471=CARTESIAN_POINT('Ctrl Pts',(65.5988381452814,-1.95974913772664,-2.));
#51472=CARTESIAN_POINT('Ctrl Pts',(65.6658026948309,-1.93043476164875,-2.));
#51473=CARTESIAN_POINT('Ctrl Pts',(65.730874875774,-1.89752507621399,-2.));
#51474=CARTESIAN_POINT('Ctrl Pts',(65.7977553584727,-1.8637008580083,-2.));
#51475=CARTESIAN_POINT('Ctrl Pts',(65.8626376079646,-1.82607804419433,-2.));
#51476=CARTESIAN_POINT('Ctrl Pts',(65.9252852210981,-1.78493106183395,-2.));
#51477=CARTESIAN_POINT('Ctrl Pts',(65.9782205027354,-1.75016314345963,-2.));
#51478=CARTESIAN_POINT('Ctrl Pts',(66.0295599817184,-1.71287801549895,-2.));
#51479=CARTESIAN_POINT('Ctrl Pts',(66.0791382962118,-1.67322322119488,-2.));
#51480=CARTESIAN_POINT('Ctrl Pts',(66.1011632204631,-1.65560677235685,-2.));
#51481=CARTESIAN_POINT('Ctrl Pts',(66.1228402691625,-1.63752248214469,-2.));
#51482=CARTESIAN_POINT('Ctrl Pts',(66.1441533920278,-1.61898256263396,-2.));
#51483=CARTESIAN_POINT('Ctrl Pts',(66.1558656059004,-1.60879430895284,-2.));
#51484=CARTESIAN_POINT('Ctrl Pts',(66.167467902359,-1.59846845594872,-2.));
#51485=CARTESIAN_POINT('Ctrl Pts',(66.1789574836609,-1.58800698854278,-2.));
#51486=CARTESIAN_POINT('Ctrl Pts',(66.1895512887021,-1.57836114129822,-2.));
#51487=CARTESIAN_POINT('Ctrl Pts',(66.2000507028277,-1.56859848611489,-2.));
#51488=CARTESIAN_POINT('Ctrl Pts',(66.210437644616,-1.5587360337551,-2.));
#51489=CARTESIAN_POINT('Ctrl Pts',(66.2635229555623,-1.50833126968861,-2.));
#51490=CARTESIAN_POINT('Ctrl Pts',(66.3137682961291,-1.45523826476737,-2.));
#51491=CARTESIAN_POINT('Ctrl Pts',(66.3609549723778,-1.39971629736155,-2.));
#51492=CARTESIAN_POINT('Ctrl Pts',(66.4077748713701,-1.34462589658626,-2.));
#51493=CARTESIAN_POINT('Ctrl Pts',(66.4515839789298,-1.28714326375553,-2.));
#51494=CARTESIAN_POINT('Ctrl Pts',(66.4921238713265,-1.22749743717743,-2.));
#51495=CARTESIAN_POINT('Ctrl Pts',(66.5258166843524,-1.17792563113991,-2.));
#51496=CARTESIAN_POINT('Ctrl Pts',(66.5572507035796,-1.12685898699336,-2.));
#51497=CARTESIAN_POINT('Ctrl Pts',(66.5862499617206,-1.07442250689085,-2.));
#51498=CARTESIAN_POINT('Ctrl Pts',(66.5983545270528,-1.05253502286947,-2.));
#51499=CARTESIAN_POINT('Ctrl Pts',(66.6100345605391,-1.03040883225682,-2.));
#51500=CARTESIAN_POINT('Ctrl Pts',(66.6212758238085,-1.00805294268962,-2.));
#51501=CARTESIAN_POINT('Ctrl Pts',(66.6264792884302,-0.997704632392041,
-2.));
#51502=CARTESIAN_POINT('Ctrl Pts',(66.6315887267379,-0.987307105267063,
-2.));
#51503=CARTESIAN_POINT('Ctrl Pts',(66.6366026612151,-0.976861256677832,
-2.));
#51504=CARTESIAN_POINT('Ctrl Pts',(66.6418315207929,-0.965967640956889,
-2.));
#51505=CARTESIAN_POINT('Ctrl Pts',(66.6469528966202,-0.955028940819226,
-2.));
#51506=CARTESIAN_POINT('Ctrl Pts',(66.6519637514069,-0.944050420232592,
-2.));
#51507=CARTESIAN_POINT('Ctrl Pts',(66.6805038460038,-0.881520566661746,
-2.));
#51508=CARTESIAN_POINT('Ctrl Pts',(66.705483022792,-0.817657226321086,-2.));
#51509=CARTESIAN_POINT('Ctrl Pts',(66.726677809183,-0.752664675176916,-2.));
#51510=CARTESIAN_POINT('Ctrl Pts',(66.7458885398579,-0.693756112813037,
-2.));
#51511=CARTESIAN_POINT('Ctrl Pts',(66.7619899159167,-0.633919258272544,
-2.));
#51512=CARTESIAN_POINT('Ctrl Pts',(66.7747787781587,-0.573301385906257,
-2.));
#51513=CARTESIAN_POINT('Ctrl Pts',(66.7899084885612,-0.50158813755264,-2.));
#51514=CARTESIAN_POINT('Ctrl Pts',(66.8004026737972,-0.42878027311813,-2.));
#51515=CARTESIAN_POINT('Ctrl Pts',(66.8063365292405,-0.355301138761089,
-2.));
#51516=CARTESIAN_POINT('Ctrl Pts',(66.8076429326892,-0.339123900294128,
-2.));
#51517=CARTESIAN_POINT('Ctrl Pts',(66.8087280690516,-0.32291420665931,-2.));
#51518=CARTESIAN_POINT('Ctrl Pts',(66.809592371063,-0.306676740190648,-2.));
#51519=CARTESIAN_POINT('Ctrl Pts',(66.8104842013171,-0.289922106213089,
-2.));
#51520=CARTESIAN_POINT('Ctrl Pts',(66.8111409153901,-0.27313175447349,-2.));
#51521=CARTESIAN_POINT('Ctrl Pts',(66.8115624311269,-0.256344928177872,
-2.));
#51522=CARTESIAN_POINT('Ctrl Pts',(66.8132840454952,-0.187781790856896,
-2.));
#51523=CARTESIAN_POINT('Ctrl Pts',(66.8110938642257,-0.119190445643793,
-2.));
#51524=CARTESIAN_POINT('Ctrl Pts',(66.8051125395855,-0.0509093849216768,
-2.));
#51525=CARTESIAN_POINT('Ctrl Pts',(66.7991324434512,0.0173576515338734,
-2.));
#51526=CARTESIAN_POINT('Ctrl Pts',(66.7893623073071,0.0853156029745438,
-2.));
#51527=CARTESIAN_POINT('Ctrl Pts',(66.7758731021479,0.152611158122592,-2.));
#51528=CARTESIAN_POINT('Ctrl Pts',(66.7661100689037,0.201317418746942,-2.));
#51529=CARTESIAN_POINT('Ctrl Pts',(66.7543977966752,0.249676426140225,-2.));
#51530=CARTESIAN_POINT('Ctrl Pts',(66.7407489756663,0.29754456718097,-2.));
#51531=CARTESIAN_POINT('Ctrl Pts',(66.7305106872339,0.333451539247104,-2.));
#51532=CARTESIAN_POINT('Ctrl Pts',(66.7191824845939,0.369082153610466,-2.));
#51533=CARTESIAN_POINT('Ctrl Pts',(66.7067658074173,0.404371614546108,-2.));
#51534=CARTESIAN_POINT('Ctrl Pts',(66.7026385144614,0.4161018014119,-2.));
#51535=CARTESIAN_POINT('Ctrl Pts',(66.6983941580482,0.427785082937903,-2.));
#51536=CARTESIAN_POINT('Ctrl Pts',(66.6940333669607,0.439418945593974,-2.));
#51537=CARTESIAN_POINT('Ctrl Pts',(66.6709086373959,0.501111863762935,-2.));
#51538=CARTESIAN_POINT('Ctrl Pts',(66.6445114918184,0.561421289076099,-2.));
#51539=CARTESIAN_POINT('Ctrl Pts',(66.6148919774249,0.620012996701175,-2.));
#51540=CARTESIAN_POINT('Ctrl Pts',(66.5940505456268,0.661240380181596,-2.));
#51541=CARTESIAN_POINT('Ctrl Pts',(66.5716128408677,0.701616780460216,-2.));
#51542=CARTESIAN_POINT('Ctrl Pts',(66.5475858840223,0.741014396509355,-2.));
#51543=CARTESIAN_POINT('Ctrl Pts',(66.5398732603013,0.753660983009995,-2.));
#51544=CARTESIAN_POINT('Ctrl Pts',(66.5319957124855,0.766208337049959,-2.));
#51545=CARTESIAN_POINT('Ctrl Pts',(66.5239568319111,0.778646543700854,-2.));
#51546=CARTESIAN_POINT('Ctrl Pts',(66.4897115300548,0.831632794381773,-2.));
#51547=CARTESIAN_POINT('Ctrl Pts',(66.4526108600522,0.882535056499814,-2.));
#51548=CARTESIAN_POINT('Ctrl Pts',(66.4126890994678,0.931037995712848,-2.));
#51549=CARTESIAN_POINT('Ctrl Pts',(66.3758798548356,0.975759383966769,-2.));
#51550=CARTESIAN_POINT('Ctrl Pts',(66.336671680953,1.01844109085503,-2.));
#51551=CARTESIAN_POINT('Ctrl Pts',(66.295069969863,1.05880296618532,-2.));
#51552=CARTESIAN_POINT('Ctrl Pts',(66.2872852045854,1.0663557258525,-2.));
#51553=CARTESIAN_POINT('Ctrl Pts',(66.279416574172,1.07382715133634,-2.));
#51554=CARTESIAN_POINT('Ctrl Pts',(66.2714656498818,1.0812165860621,-2.));
#51555=CARTESIAN_POINT('Origin',(65.,0.,3.));
#51556=CARTESIAN_POINT('Origin',(65.,0.,8.));
#51557=CARTESIAN_POINT('Origin',(65.,0.,13.));
#51558=CARTESIAN_POINT('Ctrl Pts',(63.3648706727485,-0.319230454628301,
13.));
#51559=CARTESIAN_POINT('Ctrl Pts',(63.3697100624573,-0.381552584102801,
13.));
#51560=CARTESIAN_POINT('Ctrl Pts',(63.3783265672582,-0.443390469668827,
13.));
#51561=CARTESIAN_POINT('Ctrl Pts',(63.3904636088659,-0.504524999056366,
13.));
#51562=CARTESIAN_POINT('Ctrl Pts',(63.3981627172741,-0.543305567208763,
13.));
#51563=CARTESIAN_POINT('Ctrl Pts',(63.4072795438865,-0.581803401471875,
13.));
#51564=CARTESIAN_POINT('Ctrl Pts',(63.4177589835331,-0.619964019296847,
13.));
#51565=CARTESIAN_POINT('Ctrl Pts',(63.4249317271173,-0.646083385971169,
13.));
#51566=CARTESIAN_POINT('Ctrl Pts',(63.4327429984653,-0.672044791713898,
13.));
#51567=CARTESIAN_POINT('Ctrl Pts',(63.4411771706464,-0.69783074874542,13.));
#51568=CARTESIAN_POINT('Ctrl Pts',(63.445633981408,-0.711456642114301,13.));
#51569=CARTESIAN_POINT('Ctrl Pts',(63.4502647769864,-0.725033238750576,
13.));
#51570=CARTESIAN_POINT('Ctrl Pts',(63.4550623359318,-0.738544708545356,
13.));
#51571=CARTESIAN_POINT('Ctrl Pts',(63.4771367982206,-0.800713497682774,
13.));
#51572=CARTESIAN_POINT('Ctrl Pts',(63.5027603465155,-0.861575212002685,
13.));
#51573=CARTESIAN_POINT('Ctrl Pts',(63.5316785435928,-0.920885280767066,
13.));
#51574=CARTESIAN_POINT('Ctrl Pts',(63.552535208242,-0.963661468066429,13.));
#51575=CARTESIAN_POINT('Ctrl Pts',(63.5751068652181,-1.00563072000056,13.));
#51576=CARTESIAN_POINT('Ctrl Pts',(63.5993147001858,-1.04669965515685,13.));
#51577=CARTESIAN_POINT('Ctrl Pts',(63.6059727893565,-1.05799519780992,13.));
#51578=CARTESIAN_POINT('Ctrl Pts',(63.6127547257886,-1.06922261674128,13.));
#51579=CARTESIAN_POINT('Ctrl Pts',(63.6196590403468,-1.08037991992191,13.));
#51580=CARTESIAN_POINT('Ctrl Pts',(63.6266559377188,-1.09168683600231,13.));
#51581=CARTESIAN_POINT('Ctrl Pts',(63.6337742041172,-1.10291470718646,13.));
#51582=CARTESIAN_POINT('Ctrl Pts',(63.6410091869952,-1.11405768751354,13.));
#51583=CARTESIAN_POINT('Ctrl Pts',(63.6779597277015,-1.1709671723197,13.));
#51584=CARTESIAN_POINT('Ctrl Pts',(63.7179710366331,-1.2256961535147,13.));
#51585=CARTESIAN_POINT('Ctrl Pts',(63.7607845671631,-1.27799720826047,13.));
#51586=CARTESIAN_POINT('Ctrl Pts',(63.8042168531726,-1.33105413536263,13.));
#51587=CARTESIAN_POINT('Ctrl Pts',(63.8505333121816,-1.3816134481406,13.));
#51588=CARTESIAN_POINT('Ctrl Pts',(63.899515178467,-1.42940352766181,13.));
#51589=CARTESIAN_POINT('Ctrl Pts',(63.9298610021707,-1.45901100156839,13.));
#51590=CARTESIAN_POINT('Ctrl Pts',(63.9612308493175,-1.48755527136839,13.));
#51591=CARTESIAN_POINT('Ctrl Pts',(63.9935813335733,-1.51496662410822,13.));
#51592=CARTESIAN_POINT('Ctrl Pts',(64.0200865948567,-1.53742517714731,13.));
#51593=CARTESIAN_POINT('Ctrl Pts',(64.0472502674124,-1.55912317450051,13.));
#51594=CARTESIAN_POINT('Ctrl Pts',(64.0750513948299,-1.58001951679719,13.));
#51595=CARTESIAN_POINT('Ctrl Pts',(64.0864069562603,-1.58855477132336,13.));
#51596=CARTESIAN_POINT('Ctrl Pts',(64.0978710430034,-1.59695761736653,13.));
#51597=CARTESIAN_POINT('Ctrl Pts',(64.109422488797,-1.60521141817007,13.));
#51598=CARTESIAN_POINT('Ctrl Pts',(64.1667717342953,-1.64618890765761,13.));
#51599=CARTESIAN_POINT('Ctrl Pts',(64.2263690235154,-1.6835708134358,13.));
#51600=CARTESIAN_POINT('Ctrl Pts',(64.2879736625821,-1.71708519917631,13.));
#51601=CARTESIAN_POINT('Ctrl Pts',(64.2948173903715,-1.7208083495187,13.));
#51602=CARTESIAN_POINT('Ctrl Pts',(64.3016859372404,-1.7244837434876,13.));
#51603=CARTESIAN_POINT('Ctrl Pts',(64.3085790067212,-1.72811098684768,13.));
#51604=CARTESIAN_POINT('Ctrl Pts',(64.3682468605421,-1.75950916543644,13.));
#51605=CARTESIAN_POINT('Ctrl Pts',(64.4297493247371,-1.78730275834966,13.));
#51606=CARTESIAN_POINT('Ctrl Pts',(64.4927553331735,-1.81157421874288,13.));
#51607=CARTESIAN_POINT('Ctrl Pts',(64.5605395057602,-1.837686345206,13.));
#51608=CARTESIAN_POINT('Ctrl Pts',(64.630064551517,-1.85972265026457,13.));
#51609=CARTESIAN_POINT('Ctrl Pts',(64.7009535899412,-1.87773216280799,13.));
#51610=CARTESIAN_POINT('Ctrl Pts',(64.7139243245219,-1.88102740580073,13.));
#51611=CARTESIAN_POINT('Ctrl Pts',(64.7269407961053,-1.88418768246609,13.));
#51612=CARTESIAN_POINT('Ctrl Pts',(64.7400007816474,-1.88721308481341,13.));
#51613=CARTESIAN_POINT('Ctrl Pts',(64.7512396230459,-1.88981661121387,13.));
#51614=CARTESIAN_POINT('Ctrl Pts',(64.7625015972973,-1.89231813894598,13.));
#51615=CARTESIAN_POINT('Ctrl Pts',(64.7737835813128,-1.89471786802249,13.));
#51616=CARTESIAN_POINT('Ctrl Pts',(64.843296940848,-1.90950367430022,13.));
#51617=CARTESIAN_POINT('Ctrl Pts',(64.913585486576,-1.92043263344677,13.));
#51618=CARTESIAN_POINT('Ctrl Pts',(64.9842819831785,-1.92760569490766,13.));
#51619=CARTESIAN_POINT('Ctrl Pts',(65.05646946371,-1.93493003570874,13.));
#51620=CARTESIAN_POINT('Ctrl Pts',(65.1290831839004,-1.93833864552727,13.));
#51621=CARTESIAN_POINT('Ctrl Pts',(65.201759677652,-1.93789121633581,13.));
#51622=CARTESIAN_POINT('Ctrl Pts',(65.2748769215823,-1.93744107368796,13.));
#51623=CARTESIAN_POINT('Ctrl Pts',(65.3480587639425,-1.93308814116639,13.));
#51624=CARTESIAN_POINT('Ctrl Pts',(65.4209476367097,-1.9248423197926,13.));
#51625=CARTESIAN_POINT('Ctrl Pts',(65.4389597307297,-1.92280463551765,13.));
#51626=CARTESIAN_POINT('Ctrl Pts',(65.456953949934,-1.92052897608509,13.));
#51627=CARTESIAN_POINT('Ctrl Pts',(65.4749248972257,-1.91801499804223,13.));
#51628=CARTESIAN_POINT('Ctrl Pts',(65.4889862933804,-1.91604793194321,13.));
#51629=CARTESIAN_POINT('Ctrl Pts',(65.5030350340934,-1.91393458313286,13.));
#51630=CARTESIAN_POINT('Ctrl Pts',(65.5170472633766,-1.91167847471352,13.));
#51631=CARTESIAN_POINT('Ctrl Pts',(65.5914320406422,-1.89970178500425,13.));
#51632=CARTESIAN_POINT('Ctrl Pts',(65.6649215575059,-1.88368854669915,13.));
#51633=CARTESIAN_POINT('Ctrl Pts',(65.7371322844938,-1.86371341403934,13.));
#51634=CARTESIAN_POINT('Ctrl Pts',(65.8094217307119,-1.84371650584657,13.));
#51635=CARTESIAN_POINT('Ctrl Pts',(65.8804307229118,-1.81974914158094,13.));
#51636=CARTESIAN_POINT('Ctrl Pts',(65.9497816755116,-1.7918347663575,13.));
#51637=CARTESIAN_POINT('Ctrl Pts',(66.0175539940295,-1.76455580539227,13.));
#51638=CARTESIAN_POINT('Ctrl Pts',(66.0837439310439,-1.73350736821287,13.));
#51639=CARTESIAN_POINT('Ctrl Pts',(66.1479900592074,-1.69866277513519,13.));
#51640=CARTESIAN_POINT('Ctrl Pts',(66.161806917563,-1.69116905028708,13.));
#51641=CARTESIAN_POINT('Ctrl Pts',(66.1755338057728,-1.68349956906395,13.));
#51642=CARTESIAN_POINT('Ctrl Pts',(66.1891670016328,-1.67565377050185,13.));
#51643=CARTESIAN_POINT('Ctrl Pts',(66.2007100870974,-1.66901081427423,13.));
#51644=CARTESIAN_POINT('Ctrl Pts',(66.2121860050345,-1.66224145688859,13.));
#51645=CARTESIAN_POINT('Ctrl Pts',(66.2235939546713,-1.65534738192938,13.));
#51646=CARTESIAN_POINT('Ctrl Pts',(66.8826275096638,-0.823232180103057,
13.));
#51647=CARTESIAN_POINT('Ctrl Pts',(66.9060091418344,-0.75234056523854,13.));
#51648=CARTESIAN_POINT('Ctrl Pts',(66.9251542481804,-0.680227462783449,
13.));
#51649=CARTESIAN_POINT('Ctrl Pts',(66.9401506980288,-0.607243329607971,
13.));
#51650=CARTESIAN_POINT('Ctrl Pts',(66.9547542267031,-0.536171449771447,
13.));
#51651=CARTESIAN_POINT('Ctrl Pts',(66.9654231894067,-0.464272677050615,
13.));
#51652=CARTESIAN_POINT('Ctrl Pts',(66.9721930205229,-0.391873748622197,
13.));
#51653=CARTESIAN_POINT('Ctrl Pts',(66.973704025792,-0.375714532763298,13.));
#51654=CARTESIAN_POINT('Ctrl Pts',(66.9750207650907,-0.359528284183379,
13.));
#51655=CARTESIAN_POINT('Ctrl Pts',(66.9761428768562,-0.343325629457175,
13.));
#51656=CARTESIAN_POINT('Ctrl Pts',(66.9812921188373,-0.268973508318639,
13.));
#51657=CARTESIAN_POINT('Ctrl Pts',(66.982338009526,-0.194422973994401,13.));
#51658=CARTESIAN_POINT('Ctrl Pts',(66.9793427332316,-0.120028700216811,
13.));
#51659=CARTESIAN_POINT('Ctrl Pts',(66.9772398551,-0.0677990973105729,13.));
#51660=CARTESIAN_POINT('Ctrl Pts',(66.9731439809986,-0.0156465385725868,
13.));
#51661=CARTESIAN_POINT('Ctrl Pts',(66.9670620462467,0.036301425843876,13.));
#51662=CARTESIAN_POINT('Ctrl Pts',(66.9647496285227,0.0560526067661498,
13.));
#51663=CARTESIAN_POINT('Ctrl Pts',(66.9621499863883,0.0757741531518394,
13.));
#51664=CARTESIAN_POINT('Ctrl Pts',(66.959263072388,0.0954588091203112,13.));
#51665=CARTESIAN_POINT('Ctrl Pts',(66.9565142386985,0.114201953351662,13.));
#51666=CARTESIAN_POINT('Ctrl Pts',(66.9535037847261,0.132917493687503,13.));
#51667=CARTESIAN_POINT('Ctrl Pts',(66.9502376703079,0.151566178089532,13.));
#51668=CARTESIAN_POINT('Ctrl Pts',(66.9377139254721,0.223073582629113,13.));
#51669=CARTESIAN_POINT('Ctrl Pts',(66.9214263256521,0.293675712348292,13.));
#51670=CARTESIAN_POINT('Ctrl Pts',(66.9014303057997,0.363043772415116,13.));
#51671=CARTESIAN_POINT('Ctrl Pts',(66.8818637674727,0.430921920965692,13.));
#51672=CARTESIAN_POINT('Ctrl Pts',(66.8587459438609,0.497619260733484,13.));
#51673=CARTESIAN_POINT('Ctrl Pts',(66.832085679365,0.562804370291326,13.));
#51674=CARTESIAN_POINT('Ctrl Pts',(66.806010072774,0.626559974542009,13.));
#51675=CARTESIAN_POINT('Ctrl Pts',(66.7765453046617,0.688869612373866,13.));
#51676=CARTESIAN_POINT('Ctrl Pts',(66.7436641146812,0.749389827201452,13.));
#51677=CARTESIAN_POINT('Ctrl Pts',(66.7329788263453,0.769056875321275,13.));
#51678=CARTESIAN_POINT('Ctrl Pts',(66.7219324918104,0.78853464586851,13.));
#51679=CARTESIAN_POINT('Ctrl Pts',(66.7105234437382,0.807810393806577,13.));
#51680=CARTESIAN_POINT('Ctrl Pts',(66.7040881271314,0.818682952150557,13.));
#51681=CARTESIAN_POINT('Ctrl Pts',(66.6975366290266,0.829492290259307,13.));
#51682=CARTESIAN_POINT('Ctrl Pts',(66.6908782714334,0.840221024252215,13.));
#51683=CARTESIAN_POINT('Ctrl Pts',(66.6548614911017,0.898255524510526,13.));
#51684=CARTESIAN_POINT('Ctrl Pts',(66.6156613534594,0.95403757007839,13.));
#51685=CARTESIAN_POINT('Ctrl Pts',(66.5732918040599,1.00726408484869,13.));
#51686=CARTESIAN_POINT('Ctrl Pts',(66.5671762929795,1.01494666220588,13.));
#51687=CARTESIAN_POINT('Ctrl Pts',(66.5609946872862,1.02257593937887,13.));
#51688=CARTESIAN_POINT('Ctrl Pts',(66.5547469639699,1.0301509410887,13.));
#51689=CARTESIAN_POINT('Ctrl Pts',(66.5106056086045,1.0836697711388,13.));
#51690=CARTESIAN_POINT('Ctrl Pts',(66.4631661110399,1.13448299232108,13.));
#51691=CARTESIAN_POINT('Ctrl Pts',(66.4127666235202,1.18244447913167,13.));
#51692=CARTESIAN_POINT('Ctrl Pts',(66.365747970858,1.22718867397352,13.));
#51693=CARTESIAN_POINT('Ctrl Pts',(66.3161520834383,1.26945072111514,13.));
#51694=CARTESIAN_POINT('Ctrl Pts',(66.2642393874426,1.30907445582191,13.));
#51695=CARTESIAN_POINT('Ctrl Pts',(66.252782589871,1.31781915880565,13.));
#51696=CARTESIAN_POINT('Ctrl Pts',(66.2412129249471,1.32643521269063,13.));
#51697=CARTESIAN_POINT('Ctrl Pts',(66.2295331629191,1.33492068208728,13.));
#51698=CARTESIAN_POINT('Ctrl Pts',(66.220402595367,1.34155413500801,13.));
#51699=CARTESIAN_POINT('Ctrl Pts',(66.2112052676163,1.34810730470407,13.));
#51700=CARTESIAN_POINT('Ctrl Pts',(66.2019533412583,1.3545719924638,13.));
#51701=CARTESIAN_POINT('Ctrl Pts',(66.1459049969294,1.39373519280896,13.));
#51702=CARTESIAN_POINT('Ctrl Pts',(66.0877532410082,1.42972959280653,13.));
#51703=CARTESIAN_POINT('Ctrl Pts',(66.0278290561594,1.46243222395895,13.));
#51704=CARTESIAN_POINT('Ctrl Pts',(65.9681817043714,1.49498377805451,13.));
#51705=CARTESIAN_POINT('Ctrl Pts',(65.9067771564088,1.52427416708808,13.));
#51706=CARTESIAN_POINT('Ctrl Pts',(65.8439279085686,1.55013292120153,13.));
#51707=CARTESIAN_POINT('Ctrl Pts',(65.782425269513,1.57543762532004,13.));
#51708=CARTESIAN_POINT('Ctrl Pts',(65.71953820698,1.59745625939185,13.));
#51709=CARTESIAN_POINT('Ctrl Pts',(65.6555614668715,1.61597952404088,13.));
#51710=CARTESIAN_POINT('Ctrl Pts',(65.6420830163666,1.61988195647707,13.));
#51711=CARTESIAN_POINT('Ctrl Pts',(65.6285562363675,1.6236290658509,13.));
#51712=CARTESIAN_POINT('Ctrl Pts',(65.6149839550191,1.62721860069977,13.));
#51713=CARTESIAN_POINT('Ctrl Pts',(65.6021159145385,1.63062188114732,13.));
#51714=CARTESIAN_POINT('Ctrl Pts',(65.5892052052993,1.63388381687885,13.));
#51715=CARTESIAN_POINT('Ctrl Pts',(65.5762752295761,1.63699772300991,13.));
#51716=CARTESIAN_POINT('Ctrl Pts',(65.5127465219567,1.65229724378163,13.));
#51717=CARTESIAN_POINT('Ctrl Pts',(65.4486405341705,1.66405837364474,13.));
#51718=CARTESIAN_POINT('Ctrl Pts',(65.3842420392997,1.67213585465472,13.));
#51719=CARTESIAN_POINT('Ctrl Pts',(65.3210685723957,1.68005968082915,13.));
#51720=CARTESIAN_POINT('Ctrl Pts',(65.2576127399634,1.68443871292823,13.));
#51721=CARTESIAN_POINT('Ctrl Pts',(65.1941497362031,1.68508652435148,13.));
#51722=CARTESIAN_POINT('Ctrl Pts',(65.1327484538298,1.68571329033744,13.));
#51723=CARTESIAN_POINT('Ctrl Pts',(65.0713397979654,1.68284723930067,13.));
#51724=CARTESIAN_POINT('Ctrl Pts',(65.0101900871468,1.6762734709127,13.));
#51725=CARTESIAN_POINT('Ctrl Pts',(65.0000071662403,1.67517877786091,13.));
#51726=CARTESIAN_POINT('Ctrl Pts',(64.9898314781273,1.67398116343416,13.));
#51727=CARTESIAN_POINT('Ctrl Pts',(64.9796643197989,1.67267950846503,13.));
#51728=CARTESIAN_POINT('Ctrl Pts',(64.9689074729785,1.6713023583643,13.));
#51729=CARTESIAN_POINT('Ctrl Pts',(64.9581601737451,1.66980874798799,13.));
#51730=CARTESIAN_POINT('Ctrl Pts',(64.9474239513002,1.66819938802347,13.));
#51731=CARTESIAN_POINT('Origin',(65.,0.,23.5459252805377));
#51732=CARTESIAN_POINT('Ctrl Pts',(62.9434348764936,0.00149614206266632,
21.7959252805377));
#51733=CARTESIAN_POINT('Ctrl Pts',(62.9426160796481,0.0997858054225766,
21.7905813053169));
#51734=CARTESIAN_POINT('Ctrl Pts',(62.9937092272654,0.87861806824978,21.7481913665734));
#51735=CARTESIAN_POINT('Ctrl Pts',(63.9890540527047,2.20843040890228,21.6687554643073));
#51736=CARTESIAN_POINT('Ctrl Pts',(66.3069967286646,2.04687460564975,21.5576175737392));
#51737=CARTESIAN_POINT('Ctrl Pts',(67.428612079538,0.0121339679509602,21.4464796831712));
#51738=CARTESIAN_POINT('Ctrl Pts',(66.3273005244664,-2.03388573489,21.3353417926031));
#51739=CARTESIAN_POINT('Ctrl Pts',(64.0110910734901,-2.21817972145311,21.2242039020351));
#51740=CARTESIAN_POINT('Ctrl Pts',(62.9978510382059,-0.892619747709225,
21.1443983980133));
#51741=CARTESIAN_POINT('Ctrl Pts',(62.942718846502,-0.10674080247177,21.1016388575141));
#51742=CARTESIAN_POINT('Ctrl Pts',(62.9436210622307,-0.00160392935065416,
21.0959252805377));
#51743=CARTESIAN_POINT('Ctrl Pts',(62.9473239618077,-0.00235074752840471,
21.8540747194623));
#51744=CARTESIAN_POINT('Ctrl Pts',(62.9508762982104,0.467866578479434,21.8286245525962));
#51745=CARTESIAN_POINT('Ctrl Pts',(63.3434621334709,1.62957520615004,21.7661284222074));
#51746=CARTESIAN_POINT('Ctrl Pts',(65.2721300366129,2.41280623887489,21.6665863282959));
#51747=CARTESIAN_POINT('Ctrl Pts',(67.1747422685441,1.08094901338605,21.5554484377278));
#51748=CARTESIAN_POINT('Ctrl Pts',(67.0876157148515,-1.24138505016237,21.4443105471598));
#51749=CARTESIAN_POINT('Ctrl Pts',(65.0892538486775,-2.42692553227054,21.3331726565917));
#51750=CARTESIAN_POINT('Ctrl Pts',(63.2787520820962,-1.52545559952441,21.2364273806926));
#51751=CARTESIAN_POINT('Ctrl Pts',(62.9500869585733,-0.417919283968019,
21.1767280683161));
#51752=CARTESIAN_POINT('Ctrl Pts',(62.9479182248742,0.00116161895481415,
21.1540747194623));
#51753=CARTESIAN_POINT('Ctrl Pts',(66.2690708798524,1.07935865304855,22.));
#51754=CARTESIAN_POINT('Ctrl Pts',(66.6279833110066,0.657362393039556,21.9629540364773));
#51755=CARTESIAN_POINT('Ctrl Pts',(66.8852826717605,-0.565789777391214,
21.8888621094319));
#51756=CARTESIAN_POINT('Ctrl Pts',(65.5450879211412,-1.89344353213327,21.7777242188639));
#51757=CARTESIAN_POINT('Ctrl Pts',(63.7057951684468,-1.4835378033008,21.6665863282959));
#51758=CARTESIAN_POINT('Ctrl Pts',(63.0512142972679,0.282082603662779,21.5554484377278));
#51759=CARTESIAN_POINT('Ctrl Pts',(64.180320745495,1.79060472623492,21.4443105471598));
#51760=CARTESIAN_POINT('Ctrl Pts',(66.0597184815454,1.65961459691567,21.3331726565917));
#51761=CARTESIAN_POINT('Ctrl Pts',(66.9691289570557,0.009838272590972,21.2220347660237));
#51762=CARTESIAN_POINT('Ctrl Pts',(66.0761808851496,-1.6490831655076,21.1108968754557));
#51763=CARTESIAN_POINT('Ctrl Pts',(64.1981884552545,-1.79850951013062,20.9997589848876));
#51764=CARTESIAN_POINT('Ctrl Pts',(63.0541051349916,-0.301775268334271,
20.8886210943196));
#51765=CARTESIAN_POINT('Ctrl Pts',(63.6911204902705,1.47119522218438,20.7774832037516));
#51766=CARTESIAN_POINT('Ctrl Pts',(65.5261685894954,1.89755500871053,20.6663453131835));
#51767=CARTESIAN_POINT('Ctrl Pts',(66.8796083671824,0.587065728133533,20.5552074226155));
#51768=CARTESIAN_POINT('Ctrl Pts',(66.5126214133544,-1.26077376527147,20.4440695320474));
#51769=CARTESIAN_POINT('Ctrl Pts',(64.7611148635138,-1.95461157704262,20.3329316414794));
#51770=CARTESIAN_POINT('Ctrl Pts',(63.2282626195245,-0.859371828191345,
20.2217937509113));
#51771=CARTESIAN_POINT('Ctrl Pts',(63.3171016769871,1.02246099457515,20.1106558603433));
#51772=CARTESIAN_POINT('Ctrl Pts',(64.9463166628138,1.96842352553115,19.9995179697752));
#51773=CARTESIAN_POINT('Ctrl Pts',(66.6246686119733,1.11266575470347,19.8883800792072));
#51774=CARTESIAN_POINT('Ctrl Pts',(66.8159429576165,-0.761527637475687,
19.7772421886392));
#51775=CARTESIAN_POINT('Ctrl Pts',(65.3450641189423,-1.93868612782189,19.6661042980711));
#51776=CARTESIAN_POINT('Ctrl Pts',(63.5583441794198,-1.34134322872204,19.5549664075031));
#51777=CARTESIAN_POINT('Ctrl Pts',(63.0911881617047,0.483746344304433,19.443828516935));
#51778=CARTESIAN_POINT('Ctrl Pts',(64.3711892671104,1.86605739990808,19.332690626367));
#51779=CARTESIAN_POINT('Ctrl Pts',(66.2267479674628,1.54034495606735,19.221552735799));
#51780=CARTESIAN_POINT('Ctrl Pts',(66.9594503409616,-0.19526269537746,19.1104148452309));
#51781=CARTESIAN_POINT('Ctrl Pts',(65.8986455956832,-1.7521441870034,18.9992769546629));
#51782=CARTESIAN_POINT('Ctrl Pts',(64.0153003453502,-1.70526823375495,18.8881390640948));
#51783=CARTESIAN_POINT('Ctrl Pts',(63.0332618561676,-0.0975409270146879,
18.7770011735268));
#51784=CARTESIAN_POINT('Ctrl Pts',(63.8514010943644,1.59946669637175,18.6658632829587));
#51785=CARTESIAN_POINT('Ctrl Pts',(65.720865936886,1.83246431340309,18.5547253923907));
#51786=CARTESIAN_POINT('Ctrl Pts',(66.9305140122006,0.388186562807746,18.4435875018227));
#51787=CARTESIAN_POINT('Ctrl Pts',(66.3731407186298,-1.41140275105548,18.3324496112546));
#51788=CARTESIAN_POINT('Ctrl Pts',(64.5589161528223,-1.91911912048434,18.2213117206866));
#51789=CARTESIAN_POINT('Ctrl Pts',(63.1484206345677,-0.670243994641488,
18.1101738301185));
#51790=CARTESIAN_POINT('Ctrl Pts',(63.4326967078313,1.19211306057994,17.9990359395505));
#51791=CARTESIAN_POINT('Ctrl Pts',(65.1515432588453,1.96331551197126,17.8878980489824));
#51792=CARTESIAN_POINT('Ctrl Pts',(66.7316805464207,0.937473009742852,17.7767601584144));
#51793=CARTESIAN_POINT('Ctrl Pts',(66.7267909912641,-0.946449169970139,
17.6656222678463));
#51794=CARTESIAN_POINT('Ctrl Pts',(65.1413500586618,-1.96407569094589,17.5544843772784));
#51795=CARTESIAN_POINT('Ctrl Pts',(63.4265298143476,-1.18396145786556,17.4433464867103));
#51796=CARTESIAN_POINT('Ctrl Pts',(63.1519246753265,0.679846124635256,17.3322085961423));
#51797=CARTESIAN_POINT('Ctrl Pts',(64.5688838395789,1.921382839278,17.2210707055742));
#51798=CARTESIAN_POINT('Ctrl Pts',(66.3804485146544,1.40425605116615,17.1099328150062));
#51799=CARTESIAN_POINT('Ctrl Pts',(66.9284730089157,-0.398202225924797,
16.9987949244381));
#51800=CARTESIAN_POINT('Ctrl Pts',(65.7113442877452,-1.83618148970648,16.8876570338701));
#51801=CARTESIAN_POINT('Ctrl Pts',(63.8431140728085,-1.59348301224526,16.776519143302));
#51802=CARTESIAN_POINT('Ctrl Pts',(63.033794667009,0.107748537650188,16.665381252734));
#51803=CARTESIAN_POINT('Ctrl Pts',(64.024165300781,1.71035662908353,16.5542433621659));
#51804=CARTESIAN_POINT('Ctrl Pts',(65.9077285014668,1.74745590115203,16.4431054715979));
#51805=CARTESIAN_POINT('Ctrl Pts',(66.9604375104179,0.18508896940079,16.3319675810299));
#51806=CARTESIAN_POINT('Ctrl Pts',(66.2187358332113,-1.54669199509962,16.2208296904618));
#51807=CARTESIAN_POINT('Ctrl Pts',(64.3615114264595,-1.8627682357953,16.1096917998938));
#51808=CARTESIAN_POINT('Ctrl Pts',(63.0887028520271,-0.473831585058415,
15.9985539093257));
#51809=CARTESIAN_POINT('Ctrl Pts',(63.5653262327086,1.34880848913673,15.8874160187577));
#51810=CARTESIAN_POINT('Ctrl Pts',(65.3551227829179,1.9368688566197,15.7762781281897));
#51811=CARTESIAN_POINT('Ctrl Pts',(66.819871422519,0.752091194204021,15.6651402376216));
#51812=CARTESIAN_POINT('Ctrl Pts',(66.6188711104164,-1.12108406786278,15.5540023470536));
#51813=CARTESIAN_POINT('Ctrl Pts',(64.9360997115566,-1.96811836805763,15.4428644564855));
#51814=CARTESIAN_POINT('Ctrl Pts',(63.3118169716773,-1.01371160717774,15.3317265659175));
#51815=CARTESIAN_POINT('Ctrl Pts',(63.2327473023447,0.868556886382306,15.2205886753495));
#51816=CARTESIAN_POINT('Ctrl Pts',(64.771264070325,1.955825407051,15.1094507847814));
#51817=CARTESIAN_POINT('Ctrl Pts',(66.5191454265163,1.25290476136479,14.9983128942134));
#51818=CARTESIAN_POINT('Ctrl Pts',(66.8765357500253,-0.59681383973413,14.8871750036453));
#51819=CARTESIAN_POINT('Ctrl Pts',(65.516311611266,-1.90026192842665,14.7760371130773));
#51820=CARTESIAN_POINT('Ctrl Pts',(63.6835016170176,-1.46437879615621,14.6648992225092));
#51821=CARTESIAN_POINT('Ctrl Pts',(63.0556974877489,0.311866999404039,14.5537613319412));
#51822=CARTESIAN_POINT('Ctrl Pts',(64.2075355674246,1.80265710789545,14.4426234413732));
#51823=CARTESIAN_POINT('Ctrl Pts',(66.0847251913073,1.64345528891984,14.3314855508051));
#51824=CARTESIAN_POINT('Ctrl Pts',(66.969053819969,-0.0200209189642787,
14.2203476602371));
#51825=CARTESIAN_POINT('Ctrl Pts',(66.0510846129266,-1.66516952053625,14.109209769669));
#51826=CARTESIAN_POINT('Ctrl Pts',(64.1710468184079,-1.78617400482042,13.998071879101));
#51827=CARTESIAN_POINT('Ctrl Pts',(63.049757131241,-0.272264377212424,13.8869339885329));
#51828=CARTESIAN_POINT('Ctrl Pts',(63.7135511069036,1.49083448335769,13.7757960979649));
#51829=CARTESIAN_POINT('Ctrl Pts',(65.5548379149366,1.88939023827019,13.6646582073969));
#51830=CARTESIAN_POINT('Ctrl Pts',(66.8882920122399,0.558497016674507,13.5535203168288));
#51831=CARTESIAN_POINT('Ctrl Pts',(66.4933378285089,-1.28345860874756,13.4423824262608));
#51832=CARTESIAN_POINT('Ctrl Pts',(64.7315804519141,-1.95092037563962,13.3312445356927));
#51833=CARTESIAN_POINT('Ctrl Pts',(63.2153798048402,-0.832146062593809,
13.2201066451247));
#51834=CARTESIAN_POINT('Ctrl Pts',(63.3329222496525,1.04723556764185,13.1089687545567));
#51835=CARTESIAN_POINT('Ctrl Pts',(64.9758366741791,1.97019425053385,12.9978308639886));
#51836=CARTESIAN_POINT('Ctrl Pts',(66.6419915114447,1.08548270413877,12.8866929734206));
#51837=CARTESIAN_POINT('Ctrl Pts',(66.7483953817108,-0.159901738299113,
12.8126010463752));
#51838=CARTESIAN_POINT('Ctrl Pts',(66.526442356053,-0.667480137268131,12.7755550828525));
#51839=CARTESIAN_POINT('Ctrl Pts',(66.3677806246588,1.16331236980977,22.0748149723825));
#51840=CARTESIAN_POINT('Ctrl Pts',(66.7546096639785,0.708492771249666,22.0377690088598));
#51841=CARTESIAN_POINT('Ctrl Pts',(67.0319220552433,-0.6097975356867,21.9636770818144));
#51842=CARTESIAN_POINT('Ctrl Pts',(65.5874854660279,-2.04071767641435,21.8525391912464));
#51843=CARTESIAN_POINT('Ctrl Pts',(63.605130476917,-1.59892902399571,21.7414013006783));
#51844=CARTESIAN_POINT('Ctrl Pts',(62.8996355773925,0.304023302377046,21.6302634101103));
#51845=CARTESIAN_POINT('Ctrl Pts',(64.1165651812316,1.92987995379071,21.5191255195423));
#51846=CARTESIAN_POINT('Ctrl Pts',(66.1421445639184,1.7887012664937,21.4079876289742));
#51847=CARTESIAN_POINT('Ctrl Pts',(67.1222899978831,0.0106035043776343,
21.2968497384062));
#51848=CARTESIAN_POINT('Ctrl Pts',(66.1598874315886,-1.77735068863506,21.1857118478382));
#51849=CARTESIAN_POINT('Ctrl Pts',(64.135822661333,-1.93839958057145,21.0745739572701));
#51850=CARTESIAN_POINT('Ctrl Pts',(62.9027512676903,-0.325247684413694,
20.9634360667021));
#51851=CARTESIAN_POINT('Ctrl Pts',(63.5893143859473,1.58562642318962,20.852298176134));
#51852=CARTESIAN_POINT('Ctrl Pts',(65.56709456772,2.04514894821357,20.741160285566));
#51853=CARTESIAN_POINT('Ctrl Pts',(67.0258063969427,0.632728353546081,20.630022394998));
#51854=CARTESIAN_POINT('Ctrl Pts',(66.6302747895932,-1.35883815127573,20.5188845044299));
#51855=CARTESIAN_POINT('Ctrl Pts',(64.7425341118513,-2.10664343990283,20.4077466138619));
#51856=CARTESIAN_POINT('Ctrl Pts',(63.0904549151108,-0.926214724991942,
20.2966087232938));
#51857=CARTESIAN_POINT('Ctrl Pts',(63.1862039732913,1.1019891481648,20.1854708327258));
#51858=CARTESIAN_POINT('Ctrl Pts',(64.9421411131277,2.12152969710983,20.0743329421577));
#51859=CARTESIAN_POINT('Ctrl Pts',(66.7510371439672,1.19921013488374,19.9631950515897));
#51860=CARTESIAN_POINT('Ctrl Pts',(66.9571890209963,-0.820760104276143,
19.8520571610216));
#51861=CARTESIAN_POINT('Ctrl Pts',(65.3719035899786,-2.08947929152552,19.7409192704536));
#51862=CARTESIAN_POINT('Ctrl Pts',(63.4462105859322,-1.44567439722258,19.6297813798856));
#51863=CARTESIAN_POINT('Ctrl Pts',(62.942718653474,0.521372673105626,19.5186434893175));
#51864=CARTESIAN_POINT('Ctrl Pts',(64.3222796687888,2.01120142035911,19.4075055987495));
#51865=CARTESIAN_POINT('Ctrl Pts',(66.3221657890618,1.66015470029928,19.2963677081814));
#51866=CARTESIAN_POINT('Ctrl Pts',(67.1118585682622,-0.210450445042923,
19.1852298176134));
#51867=CARTESIAN_POINT('Ctrl Pts',(65.9685432498092,-1.88842791103253,19.0740919270454));
#51868=CARTESIAN_POINT('Ctrl Pts',(63.9387093107874,-1.83790589399349,18.9629540364773));
#51869=CARTESIAN_POINT('Ctrl Pts',(62.8802867754523,-0.105127768826806,
18.8518161459093));
#51870=CARTESIAN_POINT('Ctrl Pts',(63.762061793731,1.72387499533424,18.7406782553413));
#51871=CARTESIAN_POINT('Ctrl Pts',(65.7769356913807,1.9749954262153,18.6295403647732));
#51872=CARTESIAN_POINT('Ctrl Pts',(67.0806715396602,0.418380145499126,18.5184024742052));
#51873=CARTESIAN_POINT('Ctrl Pts',(66.4799451312683,-1.52118322714048,18.4072645836371));
#51874=CARTESIAN_POINT('Ctrl Pts',(64.5246081605074,-2.06839034059004,18.296126693069));
#51875=CARTESIAN_POINT('Ctrl Pts',(63.0044027317441,-0.722376318154269,
18.184988802501));
#51876=CARTESIAN_POINT('Ctrl Pts',(63.3107901142278,1.28483694059204,18.073850911933));
#51877=CARTESIAN_POINT('Ctrl Pts',(65.1633304621018,2.11602437657287,17.962713021365));
#51878=CARTESIAN_POINT('Ctrl Pts',(66.8663725857206,1.01039070332779,17.8515751307969));
#51879=CARTESIAN_POINT('Ctrl Pts',(66.8611027155246,-1.02006503928304,17.7404372402289));
#51880=CARTESIAN_POINT('Ctrl Pts',(65.1523444234686,-2.1168436831138,17.6292993496608));
#51881=CARTESIAN_POINT('Ctrl Pts',(63.3041435529085,-1.27605129715033,17.5181614590928));
#51882=CARTESIAN_POINT('Ctrl Pts',(63.0081793206914,0.732725312500794,17.4070235685247));
#51883=CARTESIAN_POINT('Ctrl Pts',(64.5353511450282,2.07083013394974,17.2958856779567));
#51884=CARTESIAN_POINT('Ctrl Pts',(66.4878213357972,1.51348064898345,17.1847477873886));
#51885=CARTESIAN_POINT('Ctrl Pts',(67.0784717848694,-0.429174838035294,
17.0736098968206));
#51886=CARTESIAN_POINT('Ctrl Pts',(65.7666734377774,-1.97900172862672,16.9624720062526));
#51887=CARTESIAN_POINT('Ctrl Pts',(63.7531301984196,-1.71742589359987,16.8513341156845));
#51888=CARTESIAN_POINT('Ctrl Pts',(62.8808610289137,0.11612933877294,16.7401962251165));
#51889=CARTESIAN_POINT('Ctrl Pts',(63.9482637923134,1.84339007037129,16.6290583345485));
#51890=CARTESIAN_POINT('Ctrl Pts',(65.9783326341088,1.88337496509218,16.5179204439804));
#51891=CARTESIAN_POINT('Ctrl Pts',(67.1129225208572,0.199485395342077,16.4067825534124));
#51892=CARTESIAN_POINT('Ctrl Pts',(66.3135304620949,-1.66699541908821,16.2956446628443));
#51893=CARTESIAN_POINT('Ctrl Pts',(64.3118490749262,-2.00765642140262,16.1845067722763));
#51894=CARTESIAN_POINT('Ctrl Pts',(62.9400400336448,-0.510686732855825,
16.0733688817082));
#51895=CARTESIAN_POINT('Ctrl Pts',(63.4537357110932,1.45372031389702,15.9622309911402));
#51896=CARTESIAN_POINT('Ctrl Pts',(65.3827446280278,2.08752067094762,15.8510931005722));
#51897=CARTESIAN_POINT('Ctrl Pts',(66.9614230462693,0.81058968394928,15.7399552100041));
#51898=CARTESIAN_POINT('Ctrl Pts',(66.7447887062896,-1.20828323380548,15.6288173194361));
#51899=CARTESIAN_POINT('Ctrl Pts',(64.931129476036,-2.12120080414854,15.517679428868));
#51900=CARTESIAN_POINT('Ctrl Pts',(63.1805082177236,-1.09255922368241,15.4065415383));
#51901=CARTESIAN_POINT('Ctrl Pts',(63.0952884215498,0.936114207226868,15.2954036477319));
#51902=CARTESIAN_POINT('Ctrl Pts',(64.7534727352587,2.10795168295958,15.1842657571639));
#51903=CARTESIAN_POINT('Ctrl Pts',(66.6373062477565,1.35035708749135,15.0731278665959));
#51904=CARTESIAN_POINT('Ctrl Pts',(67.022494788205,-0.643234684111208,14.9619899760278));
#51905=CARTESIAN_POINT('Ctrl Pts',(65.5564709027586,-2.04806641515651,14.8508520854598));
#51906=CARTESIAN_POINT('Ctrl Pts',(63.5811029082571,-1.57827980796208,14.7397141948917));
#51907=CARTESIAN_POINT('Ctrl Pts',(62.9044674754165,0.336124361552561,14.6285763043237));
#51908=CARTESIAN_POINT('Ctrl Pts',(64.1458968022858,1.9428697831044,14.5174384137556));
#51909=CARTESIAN_POINT('Ctrl Pts',(66.1690963233843,1.77128506954561,14.4063005231876));
#51910=CARTESIAN_POINT('Ctrl Pts',(67.1222090165502,-0.0215781683134909,
14.2951626326196));
#51911=CARTESIAN_POINT('Ctrl Pts',(66.1328391433939,-1.79468825825303,14.1840247420515));
#51912=CARTESIAN_POINT('Ctrl Pts',(64.1065699177788,-1.92510460593565,14.0728868514835));
#51913=CARTESIAN_POINT('Ctrl Pts',(62.8980650713711,-0.293441403351145,
13.9617489609155));
#51914=CARTESIAN_POINT('Ctrl Pts',(63.613489680895,1.60679324794459,13.8506110703474));
#51915=CARTESIAN_POINT('Ctrl Pts',(65.5979938251871,2.03634911284552,13.7394731797794));
#51916=CARTESIAN_POINT('Ctrl Pts',(67.0351654655728,0.601937535928652,13.6283352892113));
#51917=CARTESIAN_POINT('Ctrl Pts',(66.6094913060666,-1.38328744711302,13.5171973986433));
#51918=CARTESIAN_POINT('Ctrl Pts',(64.7107024808619,-2.10266513274845,13.4060595080752));
#51919=CARTESIAN_POINT('Ctrl Pts',(63.0765700607689,-0.896871309059063,
13.2949216175072));
#51920=CARTESIAN_POINT('Ctrl Pts',(63.2032550876981,1.12869071508499,13.1837837269391));
#51921=CARTESIAN_POINT('Ctrl Pts',(64.9739572238164,2.12343815107307,13.0726458363711));
#51922=CARTESIAN_POINT('Ctrl Pts',(66.7697074378301,1.16991275640646,12.9615079458031));
#51923=CARTESIAN_POINT('Ctrl Pts',(66.8843875194939,-0.172339073385905,
12.8874160187577));
#51924=CARTESIAN_POINT('Ctrl Pts',(66.6451707405899,-0.719397484879773,
12.850370055235));
#51925=CARTESIAN_POINT('Ctrl Pts',(66.4664903694652,1.247266086571,22.149629944765));
#51926=CARTESIAN_POINT('Ctrl Pts',(66.8812360169505,0.759623149459774,22.1125839812423));
#51927=CARTESIAN_POINT('Ctrl Pts',(67.1785614387261,-0.653805293982184,
22.0384920541969));
#51928=CARTESIAN_POINT('Ctrl Pts',(65.6298830109146,-2.18799182069543,21.9273541636289));
#51929=CARTESIAN_POINT('Ctrl Pts',(63.5044657853871,-1.71432024469062,21.8162162730608));
#51930=CARTESIAN_POINT('Ctrl Pts',(62.7480568575172,0.325964001091311,21.7050783824928));
#51931=CARTESIAN_POINT('Ctrl Pts',(64.0528096169681,2.06915518134649,21.5939404919247));
#51932=CARTESIAN_POINT('Ctrl Pts',(66.2245706462915,1.91778793607172,21.4828026013567));
#51933=CARTESIAN_POINT('Ctrl Pts',(67.2754510387106,0.0113687361642993,
21.3716647107886));
#51934=CARTESIAN_POINT('Ctrl Pts',(66.2435939780275,-1.90561821176253,21.2605268202207));
#51935=CARTESIAN_POINT('Ctrl Pts',(64.0734568674116,-2.07828965101228,21.1493889296526));
#51936=CARTESIAN_POINT('Ctrl Pts',(62.751397400389,-0.348720100493116,21.0382510390846));
#51937=CARTESIAN_POINT('Ctrl Pts',(63.4875082816241,1.70005762419486,20.9271131485165));
#51938=CARTESIAN_POINT('Ctrl Pts',(65.6080205459445,2.19274288771662,20.8159752579485));
#51939=CARTESIAN_POINT('Ctrl Pts',(67.172004426703,0.678390978958629,20.7048373673804));
#51940=CARTESIAN_POINT('Ctrl Pts',(66.7479281658321,-1.45690253727999,20.5936994768124));
#51941=CARTESIAN_POINT('Ctrl Pts',(64.7239533601888,-2.25867530276304,20.4825615862443));
#51942=CARTESIAN_POINT('Ctrl Pts',(62.9526472106971,-0.993057621792541,
20.3714236956763));
#51943=CARTESIAN_POINT('Ctrl Pts',(63.0553062695956,1.18151730175446,20.2602858051083));
#51944=CARTESIAN_POINT('Ctrl Pts',(64.9379655634416,2.2746358686885,20.1491479145402));
#51945=CARTESIAN_POINT('Ctrl Pts',(66.8774056759608,1.285754515064,20.0380100239722));
#51946=CARTESIAN_POINT('Ctrl Pts',(67.0984350843764,-0.879992571076597,
19.9268721334041));
#51947=CARTESIAN_POINT('Ctrl Pts',(65.3987430610147,-2.24027245522916,19.8157342428361));
#51948=CARTESIAN_POINT('Ctrl Pts',(63.3340769924447,-1.55000556572312,19.7045963522681));
#51949=CARTESIAN_POINT('Ctrl Pts',(62.7942491452433,0.558999001906815,19.5934584617));
#51950=CARTESIAN_POINT('Ctrl Pts',(64.2733700704672,2.15634544081014,19.482320571132));
#51951=CARTESIAN_POINT('Ctrl Pts',(66.4175836106607,1.77996444453121,19.3711826805639));
#51952=CARTESIAN_POINT('Ctrl Pts',(67.2642667955629,-0.225638194708385,
19.2600447899959));
#51953=CARTESIAN_POINT('Ctrl Pts',(66.0384409039352,-2.02471163506166,19.1489068994278));
#51954=CARTESIAN_POINT('Ctrl Pts',(63.8621182762245,-1.97054355423203,19.0377690088598));
#51955=CARTESIAN_POINT('Ctrl Pts',(62.727311694737,-0.112714610638923,18.9266311182918));
#51956=CARTESIAN_POINT('Ctrl Pts',(63.6727224930976,1.84828329429673,18.8154932277237));
#51957=CARTESIAN_POINT('Ctrl Pts',(65.8330054458753,2.11752653902752,18.7043553371557));
#51958=CARTESIAN_POINT('Ctrl Pts',(67.2308290671198,0.448573728190504,18.5932174465877));
#51959=CARTESIAN_POINT('Ctrl Pts',(66.5867495439068,-1.63096370322548,18.4820795560196));
#51960=CARTESIAN_POINT('Ctrl Pts',(64.4903001681923,-2.21766156069574,18.3709416654516));
#51961=CARTESIAN_POINT('Ctrl Pts',(62.8603848289206,-0.774508641667049,
18.2598037748835));
#51962=CARTESIAN_POINT('Ctrl Pts',(63.1888835206242,1.37756082060413,18.1486658843155));
#51963=CARTESIAN_POINT('Ctrl Pts',(65.1751176653583,2.26873324117447,18.0375279937474));
#51964=CARTESIAN_POINT('Ctrl Pts',(67.0010646250206,1.08330839691273,17.9263901031794));
#51965=CARTESIAN_POINT('Ctrl Pts',(66.9954144397851,-1.09368090859595,17.8152522126113));
#51966=CARTESIAN_POINT('Ctrl Pts',(65.1633387882755,-2.26961167528171,17.7041143220433));
#51967=CARTESIAN_POINT('Ctrl Pts',(63.1817572914694,-1.36814113643509,17.5929764314753));
#51968=CARTESIAN_POINT('Ctrl Pts',(62.8644339660562,0.785604500366333,17.4818385409072));
#51969=CARTESIAN_POINT('Ctrl Pts',(64.5018184504777,2.22027742862147,17.3707006503392));
#51970=CARTESIAN_POINT('Ctrl Pts',(66.5951941569401,1.62270524680075,17.2595627597711));
#51971=CARTESIAN_POINT('Ctrl Pts',(67.2284705608229,-0.460147450145792,
17.1484248692031));
#51972=CARTESIAN_POINT('Ctrl Pts',(65.8220025878096,-2.12182196754697,17.0372869786351));
#51973=CARTESIAN_POINT('Ctrl Pts',(63.6631463240307,-1.84136877495448,16.926149088067));
#51974=CARTESIAN_POINT('Ctrl Pts',(62.7279273908184,0.124510139895692,16.815011197499));
#51975=CARTESIAN_POINT('Ctrl Pts',(63.8723622838458,1.97642351165905,16.7038733069309));
#51976=CARTESIAN_POINT('Ctrl Pts',(66.0489367667509,2.01929402903232,16.5927354163629));
#51977=CARTESIAN_POINT('Ctrl Pts',(67.2654075312964,0.213881821283365,16.4815975257949));
#51978=CARTESIAN_POINT('Ctrl Pts',(66.4083250909786,-1.7872988430768,16.3704596352268));
#51979=CARTESIAN_POINT('Ctrl Pts',(64.2621867233928,-2.15254460700995,16.2593217446588));
#51980=CARTESIAN_POINT('Ctrl Pts',(62.7913772152625,-0.547541880653236,
16.1481838540907));
#51981=CARTESIAN_POINT('Ctrl Pts',(63.3421451894777,1.5586321386573,16.0370459635227));
#51982=CARTESIAN_POINT('Ctrl Pts',(65.4103664731376,2.23817248527553,15.9259080729546));
#51983=CARTESIAN_POINT('Ctrl Pts',(67.1029746700197,0.869088173694541,15.8147701823866));
#51984=CARTESIAN_POINT('Ctrl Pts',(66.8707063021627,-1.29548239974819,15.7036322918186));
#51985=CARTESIAN_POINT('Ctrl Pts',(64.9261592405154,-2.27428324023946,15.5924944012505));
#51986=CARTESIAN_POINT('Ctrl Pts',(63.0491994637699,-1.17140684018708,15.4813565106825));
#51987=CARTESIAN_POINT('Ctrl Pts',(62.9578295407548,1.00367152807143,15.3702186201144));
#51988=CARTESIAN_POINT('Ctrl Pts',(64.7356814001924,2.26007795886816,15.2590807295464));
#51989=CARTESIAN_POINT('Ctrl Pts',(66.7554670689966,1.44780941361792,15.1479428389783));
#51990=CARTESIAN_POINT('Ctrl Pts',(67.1684538263848,-0.689655528488287,
15.0368049484103));
#51991=CARTESIAN_POINT('Ctrl Pts',(65.5966301942511,-2.19587090188638,14.9256670578423));
#51992=CARTESIAN_POINT('Ctrl Pts',(63.4787041994968,-1.69218081976795,14.8145291672742));
#51993=CARTESIAN_POINT('Ctrl Pts',(62.753237463084,0.360381723701083,14.7033912767062));
#51994=CARTESIAN_POINT('Ctrl Pts',(64.084258037147,2.08308245831336,14.5922533861381));
#51995=CARTESIAN_POINT('Ctrl Pts',(66.2534674554613,1.89911485017137,14.4811154955701));
#51996=CARTESIAN_POINT('Ctrl Pts',(67.2753642131315,-0.0231354176627016,
14.3699776050021));
#51997=CARTESIAN_POINT('Ctrl Pts',(66.214593673861,-1.92420699596982,14.258839714434));
#51998=CARTESIAN_POINT('Ctrl Pts',(64.0420930171499,-2.06403520705088,14.147701823866));
#51999=CARTESIAN_POINT('Ctrl Pts',(62.746373011501,-0.314618429489868,14.0365639332979));
#52000=CARTESIAN_POINT('Ctrl Pts',(63.5134282548864,1.72275201253148,13.9254260427299));
#52001=CARTESIAN_POINT('Ctrl Pts',(65.6411497354375,2.18330798742086,13.8142881521618));
#52002=CARTESIAN_POINT('Ctrl Pts',(67.1820389189058,0.645378055182796,13.7031502615938));
#52003=CARTESIAN_POINT('Ctrl Pts',(66.7256447836243,-1.48311628547849,13.5920123710258));
#52004=CARTESIAN_POINT('Ctrl Pts',(64.6898245098097,-2.25440988985727,13.4808744804577));
#52005=CARTESIAN_POINT('Ctrl Pts',(62.9377603166977,-0.961596555524317,
13.3697365898897));
#52006=CARTESIAN_POINT('Ctrl Pts',(63.0735879257438,1.21014586252812,13.2585986993216));
#52007=CARTESIAN_POINT('Ctrl Pts',(64.9720777734537,2.2766820516123,13.1474608087536));
#52008=CARTESIAN_POINT('Ctrl Pts',(66.8974233642155,1.25434280867416,13.0363229181856));
#52009=CARTESIAN_POINT('Ctrl Pts',(67.020379657277,-0.184776408472694,12.9622309911402));
#52010=CARTESIAN_POINT('Ctrl Pts',(66.7638991251268,-0.771314832491415,
12.9251850276175));
#52011=CARTESIAN_POINT('Ctrl Pts',(66.5652001142717,1.33121980333223,22.2244449171475));
#52012=CARTESIAN_POINT('Ctrl Pts',(67.0078623699224,0.810753527669884,22.1873989536248));
#52013=CARTESIAN_POINT('Ctrl Pts',(67.3252008222088,-0.697813052277671,
22.1133070265794));
#52014=CARTESIAN_POINT('Ctrl Pts',(65.6722805558013,-2.3352659649765,22.0021691360114));
#52015=CARTESIAN_POINT('Ctrl Pts',(63.4038010938572,-1.82971146538554,21.8910312454434));
#52016=CARTESIAN_POINT('Ctrl Pts',(62.5964781376417,0.34790469980558,21.7798933548753));
#52017=CARTESIAN_POINT('Ctrl Pts',(63.9890540527047,2.20843040890228,21.6687554643073));
#52018=CARTESIAN_POINT('Ctrl Pts',(66.3069967286646,2.04687460564975,21.5576175737392));
#52019=CARTESIAN_POINT('Ctrl Pts',(67.428612079538,0.0121339679509602,21.4464796831712));
#52020=CARTESIAN_POINT('Ctrl Pts',(66.3273005244664,-2.03388573489,21.3353417926031));
#52021=CARTESIAN_POINT('Ctrl Pts',(64.0110910734901,-2.21817972145311,21.2242039020351));
#52022=CARTESIAN_POINT('Ctrl Pts',(62.6000435330876,-0.372192516572535,
21.1130660114671));
#52023=CARTESIAN_POINT('Ctrl Pts',(63.385702177301,1.8144888252001,21.001928120899));
#52024=CARTESIAN_POINT('Ctrl Pts',(65.6489465241691,2.34033682721966,20.8907902303309));
#52025=CARTESIAN_POINT('Ctrl Pts',(67.3182024564633,0.724053604371175,20.7796523397629));
#52026=CARTESIAN_POINT('Ctrl Pts',(66.865581542071,-1.55496692328425,20.6685144491949));
#52027=CARTESIAN_POINT('Ctrl Pts',(64.7053726085262,-2.41070716562325,20.5573765586268));
#52028=CARTESIAN_POINT('Ctrl Pts',(62.8148395062834,-1.05990051859314,20.4462386680588));
#52029=CARTESIAN_POINT('Ctrl Pts',(62.9244085658998,1.26104545534411,20.3351007774907));
#52030=CARTESIAN_POINT('Ctrl Pts',(64.9337900137556,2.42774204026718,20.2239628869227));
#52031=CARTESIAN_POINT('Ctrl Pts',(67.0037742079544,1.37229889524427,20.1128249963547));
#52032=CARTESIAN_POINT('Ctrl Pts',(67.2396811477566,-0.939225037877053,
20.0016871057866));
#52033=CARTESIAN_POINT('Ctrl Pts',(65.4255825320509,-2.39106561893279,19.8905492152186));
#52034=CARTESIAN_POINT('Ctrl Pts',(63.2219433989572,-1.65433673422366,19.7794113246505));
#52035=CARTESIAN_POINT('Ctrl Pts',(62.6457796370125,0.596625330708006,19.6682734340825));
#52036=CARTESIAN_POINT('Ctrl Pts',(64.2244604721458,2.30148946126118,19.5571355435145));
#52037=CARTESIAN_POINT('Ctrl Pts',(66.5130014322595,1.89977418876314,19.4459976529464));
#52038=CARTESIAN_POINT('Ctrl Pts',(67.4166750228635,-0.240825944373849,
19.3348597623784));
#52039=CARTESIAN_POINT('Ctrl Pts',(66.1083385580613,-2.16099535909078,19.2237218718103));
#52040=CARTESIAN_POINT('Ctrl Pts',(63.7855272416616,-2.10318121447058,19.1125839812423));
#52041=CARTESIAN_POINT('Ctrl Pts',(62.5743366140218,-0.12030145245104,19.0014460906743));
#52042=CARTESIAN_POINT('Ctrl Pts',(63.5833831924642,1.97269159325921,18.8903082001062));
#52043=CARTESIAN_POINT('Ctrl Pts',(65.88907520037,2.26005765183973,18.7791703095382));
#52044=CARTESIAN_POINT('Ctrl Pts',(67.3809865945794,0.478767310881884,18.6680324189701));
#52045=CARTESIAN_POINT('Ctrl Pts',(66.6935539565454,-1.74074417931048,18.5568945284021));
#52046=CARTESIAN_POINT('Ctrl Pts',(64.4559921758773,-2.36693278080144,18.445756637834));
#52047=CARTESIAN_POINT('Ctrl Pts',(62.7163669260972,-0.826640965179831,
18.334618747266));
#52048=CARTESIAN_POINT('Ctrl Pts',(63.0669769270206,1.47028470061623,18.2234808566979));
#52049=CARTESIAN_POINT('Ctrl Pts',(65.1869048686148,2.42144210577608,18.1123429661299));
#52050=CARTESIAN_POINT('Ctrl Pts',(67.1357566643205,1.15622609049767,18.0012050755618));
#52051=CARTESIAN_POINT('Ctrl Pts',(67.1297261640456,-1.16729677790885,17.8900671849939));
#52052=CARTESIAN_POINT('Ctrl Pts',(65.1743331530824,-2.42237966744962,17.7789292944258));
#52053=CARTESIAN_POINT('Ctrl Pts',(63.0593710300304,-1.46023097571985,17.6677914038578));
#52054=CARTESIAN_POINT('Ctrl Pts',(62.720688611421,0.838483688231869,17.5566535132897));
#52055=CARTESIAN_POINT('Ctrl Pts',(64.4682857559272,2.3697247232932,17.4455156227217));
#52056=CARTESIAN_POINT('Ctrl Pts',(66.7025669780829,1.73192984461804,17.3343777321536));
#52057=CARTESIAN_POINT('Ctrl Pts',(67.3784693367765,-0.491120062256288,
17.2232398415856));
#52058=CARTESIAN_POINT('Ctrl Pts',(65.8773317378418,-2.26464220646722,17.1121019510175));
#52059=CARTESIAN_POINT('Ctrl Pts',(63.5731624496418,-1.96531165630909,17.0009640604495));
#52060=CARTESIAN_POINT('Ctrl Pts',(62.5749937527231,0.132890941018443,16.8898261698815));
#52061=CARTESIAN_POINT('Ctrl Pts',(63.7964607753782,2.1094569529468,16.7786882793134));
#52062=CARTESIAN_POINT('Ctrl Pts',(66.119540899393,2.15521309297247,16.6675503887454));
#52063=CARTESIAN_POINT('Ctrl Pts',(67.4178925417354,0.228278247224652,16.5564124981773));
#52064=CARTESIAN_POINT('Ctrl Pts',(66.5031197198625,-1.90760226706539,16.4452746076093));
#52065=CARTESIAN_POINT('Ctrl Pts',(64.2125243718594,-2.29743279261728,16.3341367170413));
#52066=CARTESIAN_POINT('Ctrl Pts',(62.6427143968803,-0.584397028450647,
16.2229988264732));
#52067=CARTESIAN_POINT('Ctrl Pts',(63.2305546678621,1.66354396341759,16.1118609359052));
#52068=CARTESIAN_POINT('Ctrl Pts',(65.4379883182475,2.38882429960344,16.0007230453371));
#52069=CARTESIAN_POINT('Ctrl Pts',(67.24452629377,0.927586663439804,15.8895851547691));
#52070=CARTESIAN_POINT('Ctrl Pts',(66.996623898036,-1.3826815656909,15.7784472642011));
#52071=CARTESIAN_POINT('Ctrl Pts',(64.9211890049946,-2.42736567633038,15.667309373633));
#52072=CARTESIAN_POINT('Ctrl Pts',(62.9178907098163,-1.25025445669175,15.556171483065));
#52073=CARTESIAN_POINT('Ctrl Pts',(62.8203706599597,1.07122884891599,15.4450335924969));
#52074=CARTESIAN_POINT('Ctrl Pts',(64.7178900651262,2.41220423477674,15.3338957019289));
#52075=CARTESIAN_POINT('Ctrl Pts',(66.8736278902366,1.54526173974448,15.2227578113608));
#52076=CARTESIAN_POINT('Ctrl Pts',(67.3144128645646,-0.736076372865367,
15.1116199207928));
#52077=CARTESIAN_POINT('Ctrl Pts',(65.6367894857436,-2.34367538861624,15.0004820302248));
#52078=CARTESIAN_POINT('Ctrl Pts',(63.3763054907363,-1.80608183157382,14.8893441396567));
#52079=CARTESIAN_POINT('Ctrl Pts',(62.6020074507516,0.384639085849608,14.7782062490887));
#52080=CARTESIAN_POINT('Ctrl Pts',(64.0226192720082,2.22329513352231,14.6670683585206));
#52081=CARTESIAN_POINT('Ctrl Pts',(66.3378385875382,2.02694463079714,14.5559304679526));
#52082=CARTESIAN_POINT('Ctrl Pts',(67.4285194097127,-0.0246926670119161,
14.4447925773845));
#52083=CARTESIAN_POINT('Ctrl Pts',(66.2963482043283,-2.05372573368659,14.3336546868165));
#52084=CARTESIAN_POINT('Ctrl Pts',(63.9776161165208,-2.20296580816612,14.2225167962485));
#52085=CARTESIAN_POINT('Ctrl Pts',(62.5946809516312,-0.335795455628588,
14.1113789056804));
#52086=CARTESIAN_POINT('Ctrl Pts',(63.4133668288776,1.83871077711838,14.0002410151124));
#52087=CARTESIAN_POINT('Ctrl Pts',(65.684305645688,2.3302668619962,13.8891031245443));
#52088=CARTESIAN_POINT('Ctrl Pts',(67.3289123722387,0.688818574436941,13.7779652339763));
#52089=CARTESIAN_POINT('Ctrl Pts',(66.8417982611818,-1.58294512384396,13.6668273434083));
#52090=CARTESIAN_POINT('Ctrl Pts',(64.6689465387577,-2.4061546469661,13.5556894528402));
#52091=CARTESIAN_POINT('Ctrl Pts',(62.7989505726263,-1.02632180198957,13.4445515622722));
#52092=CARTESIAN_POINT('Ctrl Pts',(62.9439207637896,1.29160100997125,13.3334136717041));
#52093=CARTESIAN_POINT('Ctrl Pts',(64.970198323091,2.42992595215152,13.2222757811361));
#52094=CARTESIAN_POINT('Ctrl Pts',(67.0251392906009,1.33877286094185,13.111137890568));
#52095=CARTESIAN_POINT('Ctrl Pts',(67.1563717950601,-0.197213743559485,
13.0370459635227));
#52096=CARTESIAN_POINT('Ctrl Pts',(66.8826275096638,-0.823232180103057,
13.));
#52097=CARTESIAN_POINT('Ctrl Pts',(66.2690708798524,1.07935865304855,22.));
#52098=CARTESIAN_POINT('Ctrl Pts',(66.3144013959112,1.03707009263743,22.));
#52099=CARTESIAN_POINT('Ctrl Pts',(66.3570019677251,0.99221251338095,22.));
#52100=CARTESIAN_POINT('Ctrl Pts',(66.396874028036,0.945130914769627,22.));
#52101=CARTESIAN_POINT('Ctrl Pts',(66.439378556838,0.894940853142022,22.));
#52102=CARTESIAN_POINT('Ctrl Pts',(66.4787831170335,0.842223171997003,22.));
#52103=CARTESIAN_POINT('Ctrl Pts',(66.5150606107881,0.787341095409856,22.));
#52104=CARTESIAN_POINT('Ctrl Pts',(66.5468034178233,0.739319278396103,22.));
#52105=CARTESIAN_POINT('Ctrl Pts',(66.5761518212751,0.689639120405576,22.));
#52106=CARTESIAN_POINT('Ctrl Pts',(66.6030647719507,0.638516396532125,22.));
#52107=CARTESIAN_POINT('Ctrl Pts',(66.6165687845836,0.612864734723027,22.));
#52108=CARTESIAN_POINT('Ctrl Pts',(66.629459263796,0.586849522997877,22.));
#52109=CARTESIAN_POINT('Ctrl Pts',(66.6417286804043,0.560496177531073,22.));
#52110=CARTESIAN_POINT('Ctrl Pts',(66.647332630197,0.548459515187504,22.));
#52111=CARTESIAN_POINT('Ctrl Pts',(66.6528075873728,0.536350650701833,22.));
#52112=CARTESIAN_POINT('Ctrl Pts',(66.6581443433919,0.524191916046412,22.));
#52113=CARTESIAN_POINT('Ctrl Pts',(66.6850645452224,0.46285960297952,22.));
#52114=CARTESIAN_POINT('Ctrl Pts',(66.7085235016562,0.400151855797127,22.));
#52115=CARTESIAN_POINT('Ctrl Pts',(66.7284976532585,0.3364264028118,22.));
#52116=CARTESIAN_POINT('Ctrl Pts',(66.7488259022683,0.271571238880423,22.));
#52117=CARTESIAN_POINT('Ctrl Pts',(66.7655452530524,0.205661124541036,22.));
#52118=CARTESIAN_POINT('Ctrl Pts',(66.7785915546243,0.139036642052964,22.));
#52119=CARTESIAN_POINT('Ctrl Pts',(66.7895042319112,0.0833080914905487,
22.));
#52120=CARTESIAN_POINT('Ctrl Pts',(66.7978464644136,0.0270787841007689,
22.));
#52121=CARTESIAN_POINT('Ctrl Pts',(66.8035558761527,-0.0294642473876453,
22.));
#52122=CARTESIAN_POINT('Ctrl Pts',(66.8061865906747,-0.0555174698305799,
22.));
#52123=CARTESIAN_POINT('Ctrl Pts',(66.8082580030076,-0.081637411350437,
22.));
#52124=CARTESIAN_POINT('Ctrl Pts',(66.8097622067312,-0.107806177273391,
22.));
#52125=CARTESIAN_POINT('Ctrl Pts',(66.8104186759515,-0.119226830666176,
22.));
#52126=CARTESIAN_POINT('Ctrl Pts',(66.8109669930221,-0.130656542116141,
22.));
#52127=CARTESIAN_POINT('Ctrl Pts',(66.8114061694317,-0.14207975450712,22.));
#52128=CARTESIAN_POINT('Ctrl Pts',(66.8141021938362,-0.212204785620605,
22.));
#52129=CARTESIAN_POINT('Ctrl Pts',(66.8126973724661,-0.282216215137578,
22.));
#52130=CARTESIAN_POINT('Ctrl Pts',(66.80713701542,-0.351753309319936,22.));
#52131=CARTESIAN_POINT('Ctrl Pts',(66.80216566698,-0.413924339312757,22.));
#52132=CARTESIAN_POINT('Ctrl Pts',(66.7938721956305,-0.475717167669398,
22.));
#52133=CARTESIAN_POINT('Ctrl Pts',(66.7821843766151,-0.536886120776803,
22.));
#52134=CARTESIAN_POINT('Ctrl Pts',(66.7694512323358,-0.603525850935124,
22.));
#52135=CARTESIAN_POINT('Ctrl Pts',(66.7526905137876,-0.66942595359814,22.));
#52136=CARTESIAN_POINT('Ctrl Pts',(66.7321474941548,-0.734372824653469,
22.));
#52137=CARTESIAN_POINT('Ctrl Pts',(66.7242214209376,-0.759431149301895,
22.));
#52138=CARTESIAN_POINT('Ctrl Pts',(66.71573174826,-0.784347525586081,22.));
#52139=CARTESIAN_POINT('Ctrl Pts',(66.7066905572876,-0.80910936507284,22.));
#52140=CARTESIAN_POINT('Ctrl Pts',(66.7027243122815,-0.819972040411269,
22.));
#52141=CARTESIAN_POINT('Ctrl Pts',(66.6986520383784,-0.830804390701535,
22.));
#52142=CARTESIAN_POINT('Ctrl Pts',(66.6944798306678,-0.841592845083872,
22.));
#52143=CARTESIAN_POINT('Ctrl Pts',(66.6692560535682,-0.906816244172474,
22.));
#52144=CARTESIAN_POINT('Ctrl Pts',(66.6403413434903,-0.970554427372129,
22.));
#52145=CARTESIAN_POINT('Ctrl Pts',(66.6080484131008,-1.03258856567894,22.));
#52146=CARTESIAN_POINT('Ctrl Pts',(66.5750071922106,-1.09606015657544,22.));
#52147=CARTESIAN_POINT('Ctrl Pts',(66.5384290748914,-1.15774863483118,22.));
#52148=CARTESIAN_POINT('Ctrl Pts',(66.4985928798088,-1.21741589247309,22.));
#52149=CARTESIAN_POINT('Ctrl Pts',(66.4681126351482,-1.26306966556535,22.));
#52150=CARTESIAN_POINT('Ctrl Pts',(66.4357237709963,-1.30754017026296,22.));
#52151=CARTESIAN_POINT('Ctrl Pts',(66.4015316630724,-1.35071465500183,22.));
#52152=CARTESIAN_POINT('Ctrl Pts',(66.3802494925797,-1.37758772018966,22.));
#52153=CARTESIAN_POINT('Ctrl Pts',(66.3582683894734,-1.40395856097014,22.));
#52154=CARTESIAN_POINT('Ctrl Pts',(66.3356108635762,-1.42979830341358,22.));
#52155=CARTESIAN_POINT('Ctrl Pts',(66.3229007387176,-1.4442935468157,22.));
#52156=CARTESIAN_POINT('Ctrl Pts',(66.3099732536077,-1.45862623051675,22.));
#52157=CARTESIAN_POINT('Ctrl Pts',(66.2968561826132,-1.47276572508009,22.));
#52158=CARTESIAN_POINT('Ctrl Pts',(66.2459827546045,-1.52760453467751,22.));
#52159=CARTESIAN_POINT('Ctrl Pts',(66.1922128066828,-1.57959843575484,22.));
#52160=CARTESIAN_POINT('Ctrl Pts',(66.1358313615534,-1.62848347080716,22.));
#52161=CARTESIAN_POINT('Ctrl Pts',(66.0936603481041,-1.66504747632229,22.));
#52162=CARTESIAN_POINT('Ctrl Pts',(66.0500271947279,-1.69987205106308,22.));
#52163=CARTESIAN_POINT('Ctrl Pts',(66.00503476506,-1.73283699198631,22.));
#52164=CARTESIAN_POINT('Ctrl Pts',(65.9909996372083,-1.74312021438386,22.));
#52165=CARTESIAN_POINT('Ctrl Pts',(65.9768321470098,-1.75322240064489,22.));
#52166=CARTESIAN_POINT('Ctrl Pts',(65.9625351770669,-1.76313967663704,22.));
#52167=CARTESIAN_POINT('Ctrl Pts',(65.9487346475682,-1.77271259036793,22.));
#52168=CARTESIAN_POINT('Ctrl Pts',(65.9348204929495,-1.78210828001308,22.));
#52169=CARTESIAN_POINT('Ctrl Pts',(65.9208007360916,-1.79132048320785,22.));
#52170=CARTESIAN_POINT('Ctrl Pts',(65.8578459988918,-1.83268723707061,22.));
#52171=CARTESIAN_POINT('Ctrl Pts',(65.792733983974,-1.8703783102438,22.));
#52172=CARTESIAN_POINT('Ctrl Pts',(65.7257260555984,-1.90411450232551,22.));
#52173=CARTESIAN_POINT('Ctrl Pts',(65.6744429845571,-1.92993376845009,22.));
#52174=CARTESIAN_POINT('Ctrl Pts',(65.622048450405,-1.95343614609329,22.));
#52175=CARTESIAN_POINT('Ctrl Pts',(65.5686456989049,-1.97448116510364,22.));
#52176=CARTESIAN_POINT('Ctrl Pts',(65.5562524015237,-1.97936513028632,22.));
#52177=CARTESIAN_POINT('Ctrl Pts',(65.54380476008,-1.98411668136773,22.));
#52178=CARTESIAN_POINT('Ctrl Pts',(65.531304687333,-1.9887363997513,22.));
#52179=CARTESIAN_POINT('Ctrl Pts',(63.3326792503596,-0.00130047270866476,
20.8714803633902));
#52180=CARTESIAN_POINT('Ctrl Pts',(63.3319477300267,-0.086545894594441,
20.8771939403667));
#52181=CARTESIAN_POINT('Ctrl Pts',(63.3379207823453,-0.171688456696973,
20.8829075173431));
#52182=CARTESIAN_POINT('Ctrl Pts',(63.3509549142486,-0.25573589354722,20.8886210943196));
#52183=CARTESIAN_POINT('Ctrl Pts',(63.4354662417459,-0.800686682266386,
20.9256670578423));
#52184=CARTESIAN_POINT('Ctrl Pts',(63.8168273485002,-1.2995980961985,20.9627130213649));
#52185=CARTESIAN_POINT('Ctrl Pts',(64.3205066401932,-1.52414941239406,20.9997589848876));
#52186=CARTESIAN_POINT('Ctrl Pts',(64.8241859318862,-1.74870072858961,21.0368049484103));
#52187=CARTESIAN_POINT('Ctrl Pts',(65.4501834085179,-1.6988919470486,21.073850911933));
#52188=CARTESIAN_POINT('Ctrl Pts',(65.9120068254848,-1.39750064992834,21.1108968754557));
#52189=CARTESIAN_POINT('Ctrl Pts',(66.3738302424517,-1.09610935280807,21.1479428389783));
#52190=CARTESIAN_POINT('Ctrl Pts',(66.6714795997537,-0.543135540108549,
21.184988802501));
#52191=CARTESIAN_POINT('Ctrl Pts',(66.6687358658197,0.00831408696199361,
21.2220347660237));
#52192=CARTESIAN_POINT('Ctrl Pts',(66.6659921318856,0.559763714032539,21.2590807295464));
#52193=CARTESIAN_POINT('Ctrl Pts',(66.3628553067155,1.10968915547411,21.2961266930691));
#52194=CARTESIAN_POINT('Ctrl Pts',(65.898053938122,1.40648356441476,21.3331726565917));
#52195=CARTESIAN_POINT('Ctrl Pts',(65.4332525695286,1.70327797335542,21.3702186201144));
#52196=CARTESIAN_POINT('Ctrl Pts',(64.8067866575118,1.74694134979517,21.4072645836371));
#52197=CARTESIAN_POINT('Ctrl Pts',(64.3053692934656,1.51735268425302,21.4443105471598));
#52198=CARTESIAN_POINT('Ctrl Pts',(63.8039519294193,1.28776401871087,21.4813565106825));
#52199=CARTESIAN_POINT('Ctrl Pts',(63.4275831133436,0.784923311186826,21.5184024742051));
#52200=CARTESIAN_POINT('Ctrl Pts',(63.3484955171689,0.23923288959754,21.5554484377278));
#52201=CARTESIAN_POINT('Ctrl Pts',(63.337086928647,0.160515647180261,21.5607924129486));
#52202=CARTESIAN_POINT('Ctrl Pts',(63.3318644062264,0.0809067535388596,
21.5661363881694));
#52203=CARTESIAN_POINT('Ctrl Pts',(63.3325282901756,0.00121307831918299,
21.5714803633902));
#52204=CARTESIAN_POINT('Ctrl Pts',(64.4698297828114,-1.98517432567172,22.));
#52205=CARTESIAN_POINT('Ctrl Pts',(63.8097120902545,-1.80888011517989,21.9629540364773));
#52206=CARTESIAN_POINT('Ctrl Pts',(62.6906509614045,-0.748610048502898,
21.888862109432));
#52207=CARTESIAN_POINT('Ctrl Pts',(63.1187889329781,1.53833553624066,21.7777242188639));
#52208=CARTESIAN_POINT('Ctrl Pts',(65.2721300366129,2.41280623887489,21.6665863282959));
#52209=CARTESIAN_POINT('Ctrl Pts',(67.1747422685441,1.08094901338605,21.5554484377278));
#52210=CARTESIAN_POINT('Ctrl Pts',(67.0876157148515,-1.24138505016237,21.4443105471598));
#52211=CARTESIAN_POINT('Ctrl Pts',(65.0892538486775,-2.42692553227054,21.3331726565917));
#52212=CARTESIAN_POINT('Ctrl Pts',(63.0094071033202,-1.39134559511318,21.2220347660237));
#52213=CARTESIAN_POINT('Ctrl Pts',(62.7514666617416,0.917885875238371,21.1108968754557));
#52214=CARTESIAN_POINT('Ctrl Pts',(64.5516876929394,2.3868968681091,20.9997589848876));
#52215=CARTESIAN_POINT('Ctrl Pts',(66.7622271403759,1.67118893435552,20.8886210943196));
#52216=CARTESIAN_POINT('Ctrl Pts',(67.3597936726881,-0.574194749175797,
20.7774832037516));
#52217=CARTESIAN_POINT('Ctrl Pts',(65.7974074532359,-2.2940026123021,20.6663453131835));
#52218=CARTESIAN_POINT('Ctrl Pts',(63.5051485972519,-1.91408833219884,20.5552074226155));
#52219=CARTESIAN_POINT('Ctrl Pts',(62.5811424445442,0.217814955653713,20.4440695320474));
#52220=CARTESIAN_POINT('Ctrl Pts',(63.8711449203827,2.15034861017487,20.3329316414794));
#52221=CARTESIAN_POINT('Ctrl Pts',(66.1944008109328,2.11464436694832,20.2217937509113));
#52222=CARTESIAN_POINT('Ctrl Pts',(67.4244083164919,0.143381864737545,20.1106558603433));
#52223=CARTESIAN_POINT('Ctrl Pts',(66.4353272830534,-1.95911953903995,19.9995179697752));
#52224=CARTESIAN_POINT('Ctrl Pts',(64.132474966303,-2.26841668404625,19.8883800792072));
#52225=CARTESIAN_POINT('Ctrl Pts',(62.6236781227743,-0.50140627563105,19.7772421886392));
#52226=CARTESIAN_POINT('Ctrl Pts',(63.2899556571721,1.72454696459255,19.6661042980711));
#52227=CARTESIAN_POINT('Ctrl Pts',(65.5214561645339,2.37200281981328,19.5549664075031));
#52228=CARTESIAN_POINT('Ctrl Pts',(67.2756619344365,0.848337588988218,19.443828516935));
#52229=CARTESIAN_POINT('Ctrl Pts',(66.9469285261459,-1.45182065545646,19.332690626367));
#52230=CARTESIAN_POINT('Ctrl Pts',(64.8361493591312,-2.42311099039749,19.221552735799));
#52231=CARTESIAN_POINT('Ctrl Pts',(62.8753445414284,-1.17650035527426,19.1104148452309));
#52232=CARTESIAN_POINT('Ctrl Pts',(62.8592609604237,1.14697439714762,18.9992769546629));
#52233=CARTESIAN_POINT('Ctrl Pts',(64.8026200998564,2.42061047643986,18.8881390640948));
#52234=CARTESIAN_POINT('Ctrl Pts',(66.9266433003906,1.47863433497921,18.7770011735268));
#52235=CARTESIAN_POINT('Ctrl Pts',(67.2871880384261,-0.816752582102671,
18.6658632829587));
#52236=CARTESIAN_POINT('Ctrl Pts',(65.5542436264288,-2.36455659820143,18.5547253923907));
#52237=CARTESIAN_POINT('Ctrl Pts',(63.3139937376034,-1.7480551440608,18.4435875018227));
#52238=CARTESIAN_POINT('Ctrl Pts',(62.6169645013648,0.468461007727324,18.3324496112546));
#52239=CARTESIAN_POINT('Ctrl Pts',(64.1011546824859,2.25618948643599,18.2213117206866));
#52240=CARTESIAN_POINT('Ctrl Pts',(66.4080681763277,1.97880214127948,18.1101738301185));
#52241=CARTESIAN_POINT('Ctrl Pts',(67.4261608997972,-0.109805244932086,
17.9990359395505));
#52242=CARTESIAN_POINT('Ctrl Pts',(66.2235610371465,-2.09790664518147,17.8878980489825));
#52243=CARTESIAN_POINT('Ctrl Pts',(63.9010218810697,-2.16577030121656,17.7767601584144));
#52244=CARTESIAN_POINT('Ctrl Pts',(62.5843898605093,-0.251279839042475,
17.6656222678464));
#52245=CARTESIAN_POINT('Ctrl Pts',(63.478793195507,1.89320990951442,17.5544843772783));
#52246=CARTESIAN_POINT('Ctrl Pts',(65.7655743703156,2.30482315743208,17.4433464867103));
#52247=CARTESIAN_POINT('Ctrl Pts',(67.3516166417705,0.606805630879791,17.3322085961422));
#52248=CARTESIAN_POINT('Ctrl Pts',(66.7851975318663,-1.64662797126069,17.2210707055742));
#52249=CARTESIAN_POINT('Ctrl Pts',(64.5847668755277,-2.39288431727495,17.1099328150062));
#52250=CARTESIAN_POINT('Ctrl Pts',(62.7644038070828,-0.94890651053363,16.9987949244381));
#52251=CARTESIAN_POINT('Ctrl Pts',(62.9903072873999,1.36361618663094,16.8876570338701));
#52252=CARTESIAN_POINT('Ctrl Pts',(65.0557052990257,2.42800552371272,16.776519143302));
#52253=CARTESIAN_POINT('Ctrl Pts',(67.0701156187118,1.27001386948508,16.665381252734));
#52254=CARTESIAN_POINT('Ctrl Pts',(67.1897256358837,-1.05043588241968,16.5542433621659));
#52255=CARTESIAN_POINT('Ctrl Pts',(65.3050549453524,-2.40940975839149,16.4431054715979));
#52256=CARTESIAN_POINT('Ctrl Pts',(63.141164003784,-1.56302355794458,16.3319675810298));
#52257=CARTESIAN_POINT('Ctrl Pts',(62.6786867301813,0.714015830985959,16.2208296904619));
#52258=CARTESIAN_POINT('Ctrl Pts',(64.3409338179361,2.33750843231645,16.1096917998938));
#52259=CARTESIAN_POINT('Ctrl Pts',(66.6064316564341,1.82145305641563,15.9985539093258));
#52260=CARTESIAN_POINT('Ctrl Pts',(67.401544381661,-0.361798958737837,15.8874160187577));
#52261=CARTESIAN_POINT('Ctrl Pts',(65.9984962989145,-2.2138922838142,15.7762781281897));
#52262=CARTESIAN_POINT('Ctrl Pts',(63.6815132301988,-2.03958489439843,15.6651402376216));
#52263=CARTESIAN_POINT('Ctrl Pts',(62.5713560542506,0.00157767958230164,
15.5540023470536));
#52264=CARTESIAN_POINT('Ctrl Pts',(63.6841642251148,2.04129618504104,15.4428644564855));
#52265=CARTESIAN_POINT('Ctrl Pts',(66.0013718021885,2.21259314346663,15.3317265659175));
#52266=CARTESIAN_POINT('Ctrl Pts',(67.4020124146433,0.358678503164372,15.2205886753494));
#52267=CARTESIAN_POINT('Ctrl Pts',(66.6040638188323,-1.82353863480769,15.1094507847814));
#52268=CARTESIAN_POINT('Ctrl Pts',(64.3378974271891,-2.33665018787605,14.9983128942134));
#52269=CARTESIAN_POINT('Ctrl Pts',(62.6777610116057,-0.710999308952887,
14.8871750036453));
#52270=CARTESIAN_POINT('Ctrl Pts',(63.1431963129712,1.56543726976266,14.7760371130773));
#52271=CARTESIAN_POINT('Ctrl Pts',(65.308185017446,2.40901142364104,14.6648992225093));
#52272=CARTESIAN_POINT('Ctrl Pts',(67.1910886177016,1.04758997952522,14.5537613319412));
#52273=CARTESIAN_POINT('Ctrl Pts',(67.068463685159,-1.27270221153156,14.4426234413732));
#52274=CARTESIAN_POINT('Ctrl Pts',(65.0525510239567,-2.42807611461693,14.3314855508051));
#52275=CARTESIAN_POINT('Ctrl Pts',(62.9885367426501,-1.36100346218851,14.2203476602371));
#52276=CARTESIAN_POINT('Ctrl Pts',(62.7656397187534,0.951809206360665,14.109209769669));
#52277=CARTESIAN_POINT('Ctrl Pts',(64.5878737813476,2.39342385873018,13.998071879101));
#52278=CARTESIAN_POINT('Ctrl Pts',(66.7873400138256,1.64430308142019,13.8869339885329));
#52279=CARTESIAN_POINT('Ctrl Pts',(67.3508170614469,-0.609852217558742,
13.7757960979649));
#52280=CARTESIAN_POINT('Ctrl Pts',(65.7625975239189,-2.30583209920716,13.6646582073969));
#52281=CARTESIAN_POINT('Ctrl Pts',(63.4762984963492,-1.89119971793714,13.5535203168288));
#52282=CARTESIAN_POINT('Ctrl Pts',(62.5847903309572,0.254354168931206,13.4423824262608));
#52283=CARTESIAN_POINT('Ctrl Pts',(63.9036938704104,2.16732302296764,13.3312445356927));
#52284=CARTESIAN_POINT('Ctrl Pts',(66.2265689546786,2.09606376419022,13.2201066451247));
#52285=CARTESIAN_POINT('Ctrl Pts',(67.4257384694328,0.107152139943104,13.1089687545567));
#52286=CARTESIAN_POINT('Ctrl Pts',(66.4066260077932,-1.98162422647333,12.9978308639886));
#52287=CARTESIAN_POINT('Ctrl Pts',(64.0958295620755,-2.2529948526272,12.8866929734206));
#52288=CARTESIAN_POINT('Ctrl Pts',(63.1142456563632,-1.06431345694514,12.8126010463752));
#52289=CARTESIAN_POINT('Ctrl Pts',(62.9833241385535,-0.393720754290216,
12.7755550828525));
#52290=CARTESIAN_POINT('Ctrl Pts',(64.5032651029123,-1.85997880000276,22.0748149723825));
#52291=CARTESIAN_POINT('Ctrl Pts',(63.8847779011663,-1.694802628904,22.0377690088598));
#52292=CARTESIAN_POINT('Ctrl Pts',(62.8362906481067,-0.701398764671857,
21.9636770818144));
#52293=CARTESIAN_POINT('Ctrl Pts',(63.2374279891983,1.44132001290635,21.8525391912464));
#52294=CARTESIAN_POINT('Ctrl Pts',(65.2549680863783,2.26064199742416,21.7414013006783));
#52295=CARTESIAN_POINT('Ctrl Pts',(67.0375915921608,1.0127786878876,21.6302634101104));
#52296=CARTESIAN_POINT('Ctrl Pts',(66.9559596968202,-1.16309678504486,21.5191255195423));
#52297=CARTESIAN_POINT('Ctrl Pts',(65.0836250319239,-2.27387085397712,21.4079876289743));
#52298=CARTESIAN_POINT('Ctrl Pts',(63.1349443525531,-1.30360002994301,21.2968497384062));
#52299=CARTESIAN_POINT('Ctrl Pts',(62.8932709907757,0.859999168177673,21.1857118478382));
#52300=CARTESIAN_POINT('Ctrl Pts',(64.5799606230396,2.23636660774046,21.0745739572701));
#52301=CARTESIAN_POINT('Ctrl Pts',(66.6510918358667,1.56579497755125,20.9634360667021));
#52302=CARTESIAN_POINT('Ctrl Pts',(67.2109726822582,-0.537983010725524,
20.8522981761341));
#52303=CARTESIAN_POINT('Ctrl Pts',(65.7471187486173,-2.14933075189209,20.741160285566));
#52304=CARTESIAN_POINT('Ctrl Pts',(63.5994217826059,-1.7933758628567,20.630022394998));
#52305=CARTESIAN_POINT('Ctrl Pts',(62.73368831382,0.204078399866653,20.5188845044299));
#52306=CARTESIAN_POINT('Ctrl Pts',(63.9423364541786,2.01473632608427,20.4077466138619));
#52307=CARTESIAN_POINT('Ctrl Pts',(66.1190756188575,1.98128378007219,20.2966087232938));
#52308=CARTESIAN_POINT('Ctrl Pts',(67.2715123870543,0.134339450832088,20.1854708327258));
#52309=CARTESIAN_POINT('Ctrl Pts',(66.3448080015046,-1.83556716514178,20.0743329421578));
#52310=CARTESIAN_POINT('Ctrl Pts',(64.1871856540346,-2.12535840673385,19.9631950515897));
#52311=CARTESIAN_POINT('Ctrl Pts',(62.7735414686431,-0.469784960847975,
19.8520571610217));
#52312=CARTESIAN_POINT('Ctrl Pts',(63.3978000402315,1.61578796998894,19.7409192704536));
#52313=CARTESIAN_POINT('Ctrl Pts',(65.4885703983884,2.22241185640291,19.6297813798856));
#52314=CARTESIAN_POINT('Ctrl Pts',(67.1321467335585,0.794836962355754,19.5186434893175));
#52315=CARTESIAN_POINT('Ctrl Pts',(66.8241449815883,-1.36026121516629,19.4075055987495));
#52316=CARTESIAN_POINT('Ctrl Pts',(64.8464826416291,-2.27029687716116,19.2963677081814));
#52317=CARTESIAN_POINT('Ctrl Pts',(63.0093364803535,-1.10230406000511,19.1852298176134));
#52318=CARTESIAN_POINT('Ctrl Pts',(62.9942672144912,1.07464016396579,19.0740919270454));
#52319=CARTESIAN_POINT('Ctrl Pts',(64.8150679136506,2.26795405875467,18.9629540364773));
#52320=CARTESIAN_POINT('Ctrl Pts',(66.8051390487741,1.38538388314433,18.8518161459093));
#52321=CARTESIAN_POINT('Ctrl Pts',(67.1429459408574,-0.765243871993183,
18.7406782553413));
#52322=CARTESIAN_POINT('Ctrl Pts',(65.5192901106281,-2.21543523265805,18.6295403647732));
#52323=CARTESIAN_POINT('Ctrl Pts',(63.4203221529835,-1.63781360011732,18.5184024742052));
#52324=CARTESIAN_POINT('Ctrl Pts',(62.7672512434818,0.438917394675616,18.4072645836371));
#52325=CARTESIAN_POINT('Ctrl Pts',(64.1578405919126,2.11390232046252,18.2961266930691));
#52326=CARTESIAN_POINT('Ctrl Pts',(66.3192679973039,1.85400847904606,18.184988802501));
#52327=CARTESIAN_POINT('Ctrl Pts',(67.2731544432459,-0.102880349126863,
18.073850911933));
#52328=CARTESIAN_POINT('Ctrl Pts',(66.1463968479604,-1.96560162700175,17.9627130213649));
#52329=CARTESIAN_POINT('Ctrl Pts',(63.9703292167121,-2.02918544424321,17.8515751307969));
#52330=CARTESIAN_POINT('Ctrl Pts',(62.7367309306682,-0.235432811840826,
17.7404372402289));
#52331=CARTESIAN_POINT('Ctrl Pts',(63.5747284910006,1.77381414322919,17.6292993496608));
#52332=CARTESIAN_POINT('Ctrl Pts',(65.7172932271985,2.15946889658093,17.5181614590928));
#52333=CARTESIAN_POINT('Ctrl Pts',(67.2033113378831,0.568537278849208,17.4070235685247));
#52334=CARTESIAN_POINT('Ctrl Pts',(66.6726135937532,-1.54278295786448,17.2958856779567));
#52335=CARTESIAN_POINT('Ctrl Pts',(64.6109536585329,-2.24197645689605,17.1847477873887));
#52336=CARTESIAN_POINT('Ctrl Pts',(62.9053922517429,-0.889063479188381,
17.0736098968206));
#52337=CARTESIAN_POINT('Ctrl Pts',(63.1170490714002,1.27761938368609,16.9624720062526));
#52338=CARTESIAN_POINT('Ctrl Pts',(65.0521922301209,2.27488273548329,16.8513341156845));
#52339=CARTESIAN_POINT('Ctrl Pts',(66.9395632487115,1.18992012056796,16.7401962251165));
#52340=CARTESIAN_POINT('Ctrl Pts',(67.0516300296139,-0.984189875315707,
16.6290583345485));
#52341=CARTESIAN_POINT('Ctrl Pts',(65.2858165773424,-2.25745971684959,16.5179204439804));
#52342=CARTESIAN_POINT('Ctrl Pts',(63.2583919704513,-1.46445107821859,16.4067825534124));
#52343=CARTESIAN_POINT('Ctrl Pts',(62.8250809441801,0.66898624031462,16.2956446628443));
#52344=CARTESIAN_POINT('Ctrl Pts',(64.3824979949693,2.19009286626007,16.1845067722763));
#52345=CARTESIAN_POINT('Ctrl Pts',(66.5051216338947,1.70658265439079,16.0733688817082));
#52346=CARTESIAN_POINT('Ctrl Pts',(67.2500903721106,-0.338982015036762,
15.9622309911402));
#52347=CARTESIAN_POINT('Ctrl Pts',(65.9355258749046,-2.07427260172266,15.8510931005721));
#52348=CARTESIAN_POINT('Ctrl Pts',(63.7646639349497,-1.91095795232155,15.7399552100041));
#52349=CARTESIAN_POINT('Ctrl Pts',(62.7245191047287,0.00147818281665529,
15.6288173194361));
#52350=CARTESIAN_POINT('Ctrl Pts',(63.7671477441945,1.91256131998289,15.517679428868));
#52351=CARTESIAN_POINT('Ctrl Pts',(65.9382200338304,2.07305539199278,15.4065415383));
#52352=CARTESIAN_POINT('Ctrl Pts',(67.2505288884734,0.336058351790703,15.2954036477319));
#52353=CARTESIAN_POINT('Ctrl Pts',(66.5029031245757,-1.7085367052491,15.1842657571639));
#52354=CARTESIAN_POINT('Ctrl Pts',(64.3796530949801,-2.18928874722442,15.0731278665959));
#52355=CARTESIAN_POINT('Ctrl Pts',(62.8242136062828,-0.666159956013692,
14.9619899760278));
#52356=CARTESIAN_POINT('Ctrl Pts',(63.2602961115408,1.46671256868464,14.8508520854598));
#52357=CARTESIAN_POINT('Ctrl Pts',(65.2887492506402,2.25708650318186,14.7397141948917));
#52358=CARTESIAN_POINT('Ctrl Pts',(67.0529070546353,0.981523450013854,14.6285763043237));
#52359=CARTESIAN_POINT('Ctrl Pts',(66.93801549477,-1.19243892163694,14.5174384137556));
#52360=CARTESIAN_POINT('Ctrl Pts',(65.0492368802144,-2.27494887455409,14.4063005231876));
#52361=CARTESIAN_POINT('Ctrl Pts',(63.115390186507,-1.27517143137766,14.2951626326196));
#52362=CARTESIAN_POINT('Ctrl Pts',(62.9065502203286,0.891783115762019,14.1840247420515));
#52363=CARTESIAN_POINT('Ctrl Pts',(64.6138646265439,2.24248197203166,14.0728868514835));
#52364=CARTESIAN_POINT('Ctrl Pts',(66.6746209595408,1.54060468779532,13.9617489609154));
#52365=CARTESIAN_POINT('Ctrl Pts',(67.2025621832966,-0.571391731761448,
13.8506110703474));
#52366=CARTESIAN_POINT('Ctrl Pts',(65.7145041163797,-2.16041420918537,13.7394731797794));
#52367=CARTESIAN_POINT('Ctrl Pts',(63.5723911206821,-1.77193072489694,13.6283352892113));
#52368=CARTESIAN_POINT('Ctrl Pts',(62.7371061453451,0.23831325833024,13.5171973986433));
#52369=CARTESIAN_POINT('Ctrl Pts',(63.9728326963629,2.03064024320065,13.4060595080752));
#52370=CARTESIAN_POINT('Ctrl Pts',(66.1492150704054,1.96387496777071,13.2949216175072));
#52371=CARTESIAN_POINT('Ctrl Pts',(67.2727586535603,0.100394562881356,13.1837837269391));
#52372=CARTESIAN_POINT('Ctrl Pts',(66.3179167794963,-1.85665258871666,13.0726458363711));
#52373=CARTESIAN_POINT('Ctrl Pts',(64.1528513015804,-2.11090915705047,12.9615079458031));
#52374=CARTESIAN_POINT('Ctrl Pts',(63.2331712354829,-0.997192257060735,
12.8874160187577));
#52375=CARTESIAN_POINT('Ctrl Pts',(63.1105063166185,-0.368890654402911,
12.850370055235));
#52376=CARTESIAN_POINT('Ctrl Pts',(64.5367004230132,-1.7347832743338,22.149629944765));
#52377=CARTESIAN_POINT('Ctrl Pts',(63.9598437120782,-1.5807251426281,22.1125839812423));
#52378=CARTESIAN_POINT('Ctrl Pts',(62.9819303348089,-0.654187480840814,
22.0384920541969));
#52379=CARTESIAN_POINT('Ctrl Pts',(63.3560670454183,1.34430448957203,21.9273541636289));
#52380=CARTESIAN_POINT('Ctrl Pts',(65.2378061361438,2.10847775597344,21.8162162730608));
#52381=CARTESIAN_POINT('Ctrl Pts',(66.9004409157773,0.944608362389151,21.7050783824928));
#52382=CARTESIAN_POINT('Ctrl Pts',(66.8243036787891,-1.08480851992735,21.5939404919248));
#52383=CARTESIAN_POINT('Ctrl Pts',(65.0779962151703,-2.12081617568371,21.4828026013567));
#52384=CARTESIAN_POINT('Ctrl Pts',(63.260481601786,-1.21585446477283,21.3716647107887));
#52385=CARTESIAN_POINT('Ctrl Pts',(63.0350753198097,0.802112461116973,21.2605268202206));
#52386=CARTESIAN_POINT('Ctrl Pts',(64.6082335531397,2.08583634737181,21.1493889296526));
#52387=CARTESIAN_POINT('Ctrl Pts',(66.5399565313575,1.46040102074698,21.0382510390845));
#52388=CARTESIAN_POINT('Ctrl Pts',(67.0621516918282,-0.501771272275252,
20.9271131485165));
#52389=CARTESIAN_POINT('Ctrl Pts',(65.6968300439987,-2.00465889148207,20.8159752579485));
#52390=CARTESIAN_POINT('Ctrl Pts',(63.6936949679598,-1.67266339351456,20.7048373673804));
#52391=CARTESIAN_POINT('Ctrl Pts',(62.8862341830958,0.190341844079594,20.5936994768124));
#52392=CARTESIAN_POINT('Ctrl Pts',(64.0135279879744,1.87912404199367,20.4825615862443));
#52393=CARTESIAN_POINT('Ctrl Pts',(66.0437504267822,1.84792319319607,20.3714236956763));
#52394=CARTESIAN_POINT('Ctrl Pts',(67.1186164576166,0.125297036926629,20.2602858051083));
#52395=CARTESIAN_POINT('Ctrl Pts',(66.2542887199559,-1.71201479124362,20.1491479145402));
#52396=CARTESIAN_POINT('Ctrl Pts',(64.2418963417663,-1.98230012942144,20.0380100239722));
#52397=CARTESIAN_POINT('Ctrl Pts',(62.9234048145118,-0.438163646064901,
19.9268721334041));
#52398=CARTESIAN_POINT('Ctrl Pts',(63.505644423291,1.50702897538532,19.8157342428361));
#52399=CARTESIAN_POINT('Ctrl Pts',(65.4556846322429,2.07282089299253,19.7045963522681));
#52400=CARTESIAN_POINT('Ctrl Pts',(66.9886315326805,0.741336335723289,19.5934584617));
#52401=CARTESIAN_POINT('Ctrl Pts',(66.7013614370307,-1.26870177487612,19.482320571132));
#52402=CARTESIAN_POINT('Ctrl Pts',(64.856815924127,-2.11748276392483,19.3711826805639));
#52403=CARTESIAN_POINT('Ctrl Pts',(63.1433284192787,-1.02810776473596,19.2600447899959));
#52404=CARTESIAN_POINT('Ctrl Pts',(63.1292734685587,1.00230593078395,19.1489068994279));
#52405=CARTESIAN_POINT('Ctrl Pts',(64.8275157274446,2.11529764106946,19.0377690088598));
#52406=CARTESIAN_POINT('Ctrl Pts',(66.6836347971578,1.29213343130945,18.9266311182918));
#52407=CARTESIAN_POINT('Ctrl Pts',(66.9987038432886,-0.713735161883696,
18.8154932277237));
#52408=CARTESIAN_POINT('Ctrl Pts',(65.4843365948275,-2.06631386711466,18.7043553371557));
#52409=CARTESIAN_POINT('Ctrl Pts',(63.5266505683636,-1.52757205617383,18.5932174465876));
#52410=CARTESIAN_POINT('Ctrl Pts',(62.9175379855987,0.409373781623907,18.4820795560196));
#52411=CARTESIAN_POINT('Ctrl Pts',(64.2145265013393,1.97161515448904,18.3709416654516));
#52412=CARTESIAN_POINT('Ctrl Pts',(66.2304678182801,1.72921481681263,18.2598037748835));
#52413=CARTESIAN_POINT('Ctrl Pts',(67.1201479866946,-0.0959554533216394,
18.1486658843155));
#52414=CARTESIAN_POINT('Ctrl Pts',(66.0692326587742,-1.83329660882204,18.0375279937474));
#52415=CARTESIAN_POINT('Ctrl Pts',(64.0396365523547,-1.89260058726987,17.9263901031794));
#52416=CARTESIAN_POINT('Ctrl Pts',(62.8890720008271,-0.219585784639178,
17.8152522126113));
#52417=CARTESIAN_POINT('Ctrl Pts',(63.6706637864943,1.65441837694396,17.7041143220433));
#52418=CARTESIAN_POINT('Ctrl Pts',(65.6690120840812,2.01411463572978,17.5929764314753));
#52419=CARTESIAN_POINT('Ctrl Pts',(67.0550060339956,0.530268926818625,17.4818385409072));
#52420=CARTESIAN_POINT('Ctrl Pts',(66.5600296556403,-1.43893794446826,17.3707006503392));
#52421=CARTESIAN_POINT('Ctrl Pts',(64.6371404415378,-2.09106859651715,17.2595627597711));
#52422=CARTESIAN_POINT('Ctrl Pts',(63.0463806964032,-0.829220447843132,
17.1484248692031));
#52423=CARTESIAN_POINT('Ctrl Pts',(63.2437908554003,1.19162258074125,17.0372869786351));
#52424=CARTESIAN_POINT('Ctrl Pts',(65.0486791612162,2.12175994725385,16.926149088067));
#52425=CARTESIAN_POINT('Ctrl Pts',(66.8090108787112,1.10982637165085,16.815011197499));
#52426=CARTESIAN_POINT('Ctrl Pts',(66.9135344233438,-0.917943868211739,
16.7038733069309));
#52427=CARTESIAN_POINT('Ctrl Pts',(65.2665782093324,-2.10550967530768,16.5927354163629));
#52428=CARTESIAN_POINT('Ctrl Pts',(63.3756199371186,-1.3658785984926,16.4815975257949));
#52429=CARTESIAN_POINT('Ctrl Pts',(62.9714751581789,0.623956649643286,16.3704596352268));
#52430=CARTESIAN_POINT('Ctrl Pts',(64.4240621720026,2.04267730020369,16.2593217446588));
#52431=CARTESIAN_POINT('Ctrl Pts',(66.4038116113553,1.59171225236596,16.1481838540907));
#52432=CARTESIAN_POINT('Ctrl Pts',(67.0986363625603,-0.316165071335693,
16.0370459635227));
#52433=CARTESIAN_POINT('Ctrl Pts',(65.8725554508947,-1.93465291963112,15.9259080729547));
#52434=CARTESIAN_POINT('Ctrl Pts',(63.8478146397005,-1.78233101024467,15.8147701823866));
#52435=CARTESIAN_POINT('Ctrl Pts',(62.8776821552069,0.00137868605101399,
15.7036322918186));
#52436=CARTESIAN_POINT('Ctrl Pts',(63.8501312632742,1.78382645492474,15.5924944012505));
#52437=CARTESIAN_POINT('Ctrl Pts',(65.8750682654724,1.93351764051894,15.4813565106825));
#52438=CARTESIAN_POINT('Ctrl Pts',(67.0990453623036,0.313438200417032,15.3702186201144));
#52439=CARTESIAN_POINT('Ctrl Pts',(66.401742430319,-1.59353477569052,15.2590807295464));
#52440=CARTESIAN_POINT('Ctrl Pts',(64.4214087627711,-2.04192730657279,15.1479428389783));
#52441=CARTESIAN_POINT('Ctrl Pts',(62.9706662009597,-0.621320603074498,
15.0368049484103));
#52442=CARTESIAN_POINT('Ctrl Pts',(63.3773959101104,1.36798786760661,14.9256670578422));
#52443=CARTESIAN_POINT('Ctrl Pts',(65.2693134838344,2.10516158272269,14.8145291672742));
#52444=CARTESIAN_POINT('Ctrl Pts',(66.914725491569,0.91545692050249,14.7033912767062));
#52445=CARTESIAN_POINT('Ctrl Pts',(66.8075673043809,-1.11217563174233,14.5922533861381));
#52446=CARTESIAN_POINT('Ctrl Pts',(65.0459227364722,-2.12182163449126,14.4811154955701));
#52447=CARTESIAN_POINT('Ctrl Pts',(63.2422436303638,-1.18933940056681,14.3699776050021));
#52448=CARTESIAN_POINT('Ctrl Pts',(63.0474607219038,0.831757025163371,14.258839714434));
#52449=CARTESIAN_POINT('Ctrl Pts',(64.6398554717402,2.09154008533314,14.147701823866));
#52450=CARTESIAN_POINT('Ctrl Pts',(66.5619019052561,1.43690629417045,14.0365639332979));
#52451=CARTESIAN_POINT('Ctrl Pts',(67.0543073051464,-0.532931245964157,
13.9254260427299));
#52452=CARTESIAN_POINT('Ctrl Pts',(65.6664107088405,-2.01499631916359,13.8142881521618));
#52453=CARTESIAN_POINT('Ctrl Pts',(63.668483745015,-1.65266173185674,13.7031502615938));
#52454=CARTESIAN_POINT('Ctrl Pts',(62.889421959733,0.222272347729275,13.5920123710258));
#52455=CARTESIAN_POINT('Ctrl Pts',(64.0419715223154,1.89395746343366,13.4808744804577));
#52456=CARTESIAN_POINT('Ctrl Pts',(66.0718611861322,1.8316861713512,13.3697365898897));
#52457=CARTESIAN_POINT('Ctrl Pts',(67.1197788376878,0.093636985819607,13.2585986993216));
#52458=CARTESIAN_POINT('Ctrl Pts',(66.2292075511993,-1.73168095096,13.1474608087536));
#52459=CARTESIAN_POINT('Ctrl Pts',(64.2098730410853,-1.96882346147375,13.0363229181856));
#52460=CARTESIAN_POINT('Ctrl Pts',(63.3520968146026,-0.930071057176334,
12.9622309911402));
#52461=CARTESIAN_POINT('Ctrl Pts',(63.2376884946835,-0.344060554515606,
12.9251850276175));
#52462=CARTESIAN_POINT('Ctrl Pts',(64.5701357431142,-1.60958774866485,22.2244449171475));
#52463=CARTESIAN_POINT('Ctrl Pts',(64.0349095229901,-1.46664765635221,22.1873989536248));
#52464=CARTESIAN_POINT('Ctrl Pts',(63.1275700215111,-0.606976197009772,
22.1133070265794));
#52465=CARTESIAN_POINT('Ctrl Pts',(63.4747061016384,1.24728896623771,22.0021691360114));
#52466=CARTESIAN_POINT('Ctrl Pts',(65.2206441859093,1.95631351452272,21.8910312454434));
#52467=CARTESIAN_POINT('Ctrl Pts',(66.7632902393938,0.8764380368907,21.7798933548753));
#52468=CARTESIAN_POINT('Ctrl Pts',(66.692647660758,-1.00652025480984,21.6687554643073));
#52469=CARTESIAN_POINT('Ctrl Pts',(65.0723673984167,-1.9677614973903,21.5576175737392));
#52470=CARTESIAN_POINT('Ctrl Pts',(63.3860188510191,-1.12810889960266,21.4464796831712));
#52471=CARTESIAN_POINT('Ctrl Pts',(63.1768796488437,0.744225754056273,21.3353417926031));
#52472=CARTESIAN_POINT('Ctrl Pts',(64.6365064832399,1.93530608700317,21.2242039020351));
#52473=CARTESIAN_POINT('Ctrl Pts',(66.4288212268481,1.35500706394271,21.113066011467));
#52474=CARTESIAN_POINT('Ctrl Pts',(66.9133307013985,-0.46555953382498,21.001928120899));
#52475=CARTESIAN_POINT('Ctrl Pts',(65.6465413393799,-1.85998703107205,20.890790230331));
#52476=CARTESIAN_POINT('Ctrl Pts',(63.7879681533139,-1.55195092417241,20.7796523397629));
#52477=CARTESIAN_POINT('Ctrl Pts',(63.0387800523716,0.176605288292535,20.6685144491949));
#52478=CARTESIAN_POINT('Ctrl Pts',(64.0847195217704,1.74351175790307,20.5573765586268));
#52479=CARTESIAN_POINT('Ctrl Pts',(65.9684252347068,1.71456260631994,20.4462386680588));
#52480=CARTESIAN_POINT('Ctrl Pts',(66.965720528179,0.11625462302117,20.3351007774908));
#52481=CARTESIAN_POINT('Ctrl Pts',(66.163769438407,-1.58846241734545,20.2239628869227));
#52482=CARTESIAN_POINT('Ctrl Pts',(64.296607029498,-1.83924185210904,20.1128249963547));
#52483=CARTESIAN_POINT('Ctrl Pts',(63.0732681603805,-0.406542331281825,
20.0016871057866));
#52484=CARTESIAN_POINT('Ctrl Pts',(63.6134888063506,1.3982699807817,19.8905492152186));
#52485=CARTESIAN_POINT('Ctrl Pts',(65.4227988660973,1.92322992958215,19.7794113246506));
#52486=CARTESIAN_POINT('Ctrl Pts',(66.8451163318026,0.687835709090824,19.6682734340825));
#52487=CARTESIAN_POINT('Ctrl Pts',(66.5785778924731,-1.17714233458594,19.5571355435145));
#52488=CARTESIAN_POINT('Ctrl Pts',(64.8671492066249,-1.96466865068851,19.4459976529464));
#52489=CARTESIAN_POINT('Ctrl Pts',(63.277320358204,-0.953911469466806,19.3348597623784));
#52490=CARTESIAN_POINT('Ctrl Pts',(63.2642797226261,0.929971697602112,19.2237218718103));
#52491=CARTESIAN_POINT('Ctrl Pts',(64.8399635412389,1.96264122338426,19.1125839812423));
#52492=CARTESIAN_POINT('Ctrl Pts',(66.5621305455413,1.19888297947457,19.0014460906742));
#52493=CARTESIAN_POINT('Ctrl Pts',(66.8544617457199,-0.662226451774208,
18.8903082001062));
#52494=CARTESIAN_POINT('Ctrl Pts',(65.4493830790269,-1.91719250157128,18.7791703095382));
#52495=CARTESIAN_POINT('Ctrl Pts',(63.6329789837436,-1.41733051223035,18.6680324189701));
#52496=CARTESIAN_POINT('Ctrl Pts',(63.0678247277157,0.379830168572198,18.5568945284021));
#52497=CARTESIAN_POINT('Ctrl Pts',(64.271212410766,1.82932798851557,18.445756637834));
#52498=CARTESIAN_POINT('Ctrl Pts',(66.1416676392564,1.6044211545792,18.334618747266));
#52499=CARTESIAN_POINT('Ctrl Pts',(66.9671415301433,-0.089030557516416,
18.223480856698));
#52500=CARTESIAN_POINT('Ctrl Pts',(65.9920684695881,-1.70099159064233,18.1123429661299));
#52501=CARTESIAN_POINT('Ctrl Pts',(64.1089438879971,-1.75601573029652,18.0012050755619));
#52502=CARTESIAN_POINT('Ctrl Pts',(63.0414130709861,-0.203738757437529,
17.8900671849938));
#52503=CARTESIAN_POINT('Ctrl Pts',(63.7665990819878,1.53502261065873,17.7789292944258));
#52504=CARTESIAN_POINT('Ctrl Pts',(65.6207309409642,1.86876037487862,17.6677914038578));
#52505=CARTESIAN_POINT('Ctrl Pts',(66.906700730108,0.492000574788043,17.5566535132897));
#52506=CARTESIAN_POINT('Ctrl Pts',(66.4474457175273,-1.33509293107205,17.4455156227217));
#52507=CARTESIAN_POINT('Ctrl Pts',(64.6633272245428,-1.94016073613825,17.3343777321536));
#52508=CARTESIAN_POINT('Ctrl Pts',(63.1873691410633,-0.769377416497885,
17.2232398415856));
#52509=CARTESIAN_POINT('Ctrl Pts',(63.3705326394006,1.1056257777964,17.1121019510176));
#52510=CARTESIAN_POINT('Ctrl Pts',(65.0451660923113,1.96863715902441,17.0009640604495));
#52511=CARTESIAN_POINT('Ctrl Pts',(66.6784585087109,1.02973262273374,16.8898261698815));
#52512=CARTESIAN_POINT('Ctrl Pts',(66.7754388170738,-0.851697861107768,
16.7786882793134));
#52513=CARTESIAN_POINT('Ctrl Pts',(65.2473398413224,-1.95355963376578,16.6675503887454));
#52514=CARTESIAN_POINT('Ctrl Pts',(63.4928479037859,-1.2673061187666,16.5564124981773));
#52515=CARTESIAN_POINT('Ctrl Pts',(63.1178693721777,0.578927058971946,16.4452746076093));
#52516=CARTESIAN_POINT('Ctrl Pts',(64.4656263490358,1.89526173414732,16.3341367170413));
#52517=CARTESIAN_POINT('Ctrl Pts',(66.3025015888158,1.47684185034113,16.2229988264732));
#52518=CARTESIAN_POINT('Ctrl Pts',(66.9471823530099,-0.29334812763462,16.1118609359052));
#52519=CARTESIAN_POINT('Ctrl Pts',(65.8095850268849,-1.79503323753958,16.0007230453371));
#52520=CARTESIAN_POINT('Ctrl Pts',(63.9309653444512,-1.6537040681678,15.8895851547691));
#52521=CARTESIAN_POINT('Ctrl Pts',(63.0308452056851,0.00127918928536937,
15.778447264201));
#52522=CARTESIAN_POINT('Ctrl Pts',(63.9331147823537,1.65509158986659,15.667309373633));
#52523=CARTESIAN_POINT('Ctrl Pts',(65.8119164971145,1.79397988904509,15.556171483065));
#52524=CARTESIAN_POINT('Ctrl Pts',(66.9475618361337,0.290818049043361,15.4450335924969));
#52525=CARTESIAN_POINT('Ctrl Pts',(66.3005817360626,-1.47853284613194,15.3338957019289));
#52526=CARTESIAN_POINT('Ctrl Pts',(64.4631644305619,-1.89456586592116,15.2227578113608));
#52527=CARTESIAN_POINT('Ctrl Pts',(63.1171187956369,-0.5764812501353,15.1116199207928));
#52528=CARTESIAN_POINT('Ctrl Pts',(63.4944957086799,1.26926316652858,15.0004820302248));
#52529=CARTESIAN_POINT('Ctrl Pts',(65.2498777170288,1.95323666226352,14.8893441396567));
#52530=CARTESIAN_POINT('Ctrl Pts',(66.7765439285027,0.849390390991124,14.7782062490887));
#52531=CARTESIAN_POINT('Ctrl Pts',(66.6771191139918,-1.03191234184771,14.6670683585206));
#52532=CARTESIAN_POINT('Ctrl Pts',(65.0426085927299,-1.96869439442842,14.5559304679526));
#52533=CARTESIAN_POINT('Ctrl Pts',(63.3690970742208,-1.10350736975596,14.4447925773845));
#52534=CARTESIAN_POINT('Ctrl Pts',(63.1883712234789,0.771730934564724,14.3336546868165));
#52535=CARTESIAN_POINT('Ctrl Pts',(64.6658463169365,1.94059819863462,14.2225167962484));
#52536=CARTESIAN_POINT('Ctrl Pts',(66.4491828509713,1.33320790054559,14.1113789056804));
#52537=CARTESIAN_POINT('Ctrl Pts',(66.9060524269962,-0.494470760166863,
14.0002410151124));
#52538=CARTESIAN_POINT('Ctrl Pts',(65.6183173013013,-1.86957842914181,13.8891031245443));
#52539=CARTESIAN_POINT('Ctrl Pts',(63.764576369348,-1.53339273881653,13.7779652339763));
#52540=CARTESIAN_POINT('Ctrl Pts',(63.0417377741208,0.206231437128308,13.6668273434082));
#52541=CARTESIAN_POINT('Ctrl Pts',(64.111110348268,1.75727468366667,13.5556894528402));
#52542=CARTESIAN_POINT('Ctrl Pts',(65.9945073018589,1.69949737493169,13.4445515622722));
#52543=CARTESIAN_POINT('Ctrl Pts',(66.9667990218154,0.0868794087578594,
13.3334136717041));
#52544=CARTESIAN_POINT('Ctrl Pts',(66.1404983229023,-1.60670931320334,13.2222757811361));
#52545=CARTESIAN_POINT('Ctrl Pts',(64.2668947805903,-1.82673776589702,13.111137890568));
#52546=CARTESIAN_POINT('Ctrl Pts',(63.4710223937224,-0.862949857291932,
13.0370459635227));
#52547=CARTESIAN_POINT('Ctrl Pts',(63.3648706727485,-0.319230454628301,
13.));
#52548=CARTESIAN_POINT('Ctrl Pts',(63.3361634080255,0.000941845566869666,
21.3785196366098));
#52549=CARTESIAN_POINT('Ctrl Pts',(63.3350462116423,0.216826197428607,21.3641270219409));
#52550=CARTESIAN_POINT('Ctrl Pts',(63.3740367968513,0.432323693321034,21.349734407272));
#52551=CARTESIAN_POINT('Ctrl Pts',(63.4550073216056,0.630683367270934,21.3353417926031));
#52552=CARTESIAN_POINT('Ctrl Pts',(63.6634219269757,1.14125253170524,21.2982958290804));
#52553=CARTESIAN_POINT('Ctrl Pts',(64.1499642051078,1.5382793093542,21.2612498655578));
#52554=CARTESIAN_POINT('Ctrl Pts',(64.6919544681085,1.64007619433528,21.2242039020351));
#52555=CARTESIAN_POINT('Ctrl Pts',(65.2339447311093,1.74187307931635,21.1871579385124));
#52556=CARTESIAN_POINT('Ctrl Pts',(65.8313829789787,1.54844007162953,21.1501119749897));
#52557=CARTESIAN_POINT('Ctrl Pts',(66.2108536820051,1.14829580149151,21.113066011467));
#52558=CARTESIAN_POINT('Ctrl Pts',(66.5903243850316,0.748151531353484,21.0760200479444));
#52559=CARTESIAN_POINT('Ctrl Pts',(66.751827543215,0.141295998764253,21.0389740844217));
#52560=CARTESIAN_POINT('Ctrl Pts',(66.6214475619703,-0.394536350404874,
21.001928120899));
#52561=CARTESIAN_POINT('Ctrl Pts',(66.4910675807256,-0.930368699574004,
20.9648821573763));
#52562=CARTESIAN_POINT('Ctrl Pts',(66.0688044600528,-1.39517786532303,20.9278361938536));
#52563=CARTESIAN_POINT('Ctrl Pts',(65.5479107020387,-1.5762430970476,20.890790230331));
#52564=CARTESIAN_POINT('Ctrl Pts',(65.0270169440246,-1.75730832877217,20.8537442668083));
#52565=CARTESIAN_POINT('Ctrl Pts',(64.4074925486692,-1.65462962647229,20.8166983032856));
#52566=CARTESIAN_POINT('Ctrl Pts',(63.9728656675012,-1.31519757324486,20.7796523397629));
#52567=CARTESIAN_POINT('Ctrl Pts',(63.5773660666821,-1.00632288699472,20.7459414387119));
#52568=CARTESIAN_POINT('Ctrl Pts',(63.3349716882235,-0.501403518382676,
20.7122305376608));
#52569=CARTESIAN_POINT('Ctrl Pts',(63.3318013787731,0.000864016794202189,
20.6785196366098));
#52570=CARTESIAN_POINT('Ctrl Pts',(64.4698297828114,-1.98517432567172,22.));
#52571=CARTESIAN_POINT('Ctrl Pts',(64.4011635904062,-1.95974978038744,22.));
#52572=CARTESIAN_POINT('Ctrl Pts',(64.3342007656389,-1.93043577138037,22.));
#52573=CARTESIAN_POINT('Ctrl Pts',(64.2691302660868,-1.89752626078973,22.));
#52574=CARTESIAN_POINT('Ctrl Pts',(64.2022499741928,-1.86370144478953,22.));
#52575=CARTESIAN_POINT('Ctrl Pts',(64.1373679615241,-1.82607765547926,22.));
#52576=CARTESIAN_POINT('Ctrl Pts',(64.0747206099686,-1.78492942875554,22.));
#52577=CARTESIAN_POINT('Ctrl Pts',(64.0217852175793,-1.75016024101401,22.));
#52578=CARTESIAN_POINT('Ctrl Pts',(63.9704456655164,-1.71287362002848,22.));
#52579=CARTESIAN_POINT('Ctrl Pts',(63.9208673056513,-1.67321717698663,22.));
#52580=CARTESIAN_POINT('Ctrl Pts',(63.8988414814123,-1.65559929195053,22.));
#52581=CARTESIAN_POINT('Ctrl Pts',(63.8771635659827,-1.63751349743213,22.));
#52582=CARTESIAN_POINT('Ctrl Pts',(63.8558496107185,-1.61897201296707,22.));
#52583=CARTESIAN_POINT('Ctrl Pts',(63.8441378985453,-1.60878373366242,22.));
#52584=CARTESIAN_POINT('Ctrl Pts',(63.8325360961551,-1.59845785925709,22.));
#52585=CARTESIAN_POINT('Ctrl Pts',(63.8210470007987,-1.58799637542554,22.));
#52586=CARTESIAN_POINT('Ctrl Pts',(63.8104526359386,-1.57834959530466,22.));
#52587=CARTESIAN_POINT('Ctrl Pts',(63.7999526722266,-1.56858598843039,22.));
#52588=CARTESIAN_POINT('Ctrl Pts',(63.7895651937366,-1.55872256958869,22.));
#52589=CARTESIAN_POINT('Ctrl Pts',(63.7364801435476,-1.50831571822926,22.));
#52590=CARTESIAN_POINT('Ctrl Pts',(63.6862350752836,-1.45522053846986,22.));
#52591=CARTESIAN_POINT('Ctrl Pts',(63.6390486652555,-1.39969641403709,22.));
#52592=CARTESIAN_POINT('Ctrl Pts',(63.5922286928545,-1.34460347579517,22.));
#52593=CARTESIAN_POINT('Ctrl Pts',(63.5484195492904,-1.28711828832214,22.));
#52594=CARTESIAN_POINT('Ctrl Pts',(63.5078796466367,-1.22746999892659,22.));
#52595=CARTESIAN_POINT('Ctrl Pts',(63.474187130903,-1.17789659599779,22.));
#52596=CARTESIAN_POINT('Ctrl Pts',(63.4427533858128,-1.12682844545585,22.));
#52597=CARTESIAN_POINT('Ctrl Pts',(63.413754367488,-1.07439061084553,22.));
#52598=CARTESIAN_POINT('Ctrl Pts',(63.4016500392299,-1.05250280912221,22.));
#52599=CARTESIAN_POINT('Ctrl Pts',(63.3899702272242,-1.03037633270796,22.));
#52600=CARTESIAN_POINT('Ctrl Pts',(63.3787291685042,-1.0080201935721,22.));
#52601=CARTESIAN_POINT('Ctrl Pts',(63.3735259415771,-0.997672052170427,
22.));
#52602=CARTESIAN_POINT('Ctrl Pts',(63.3684167321672,-0.987274704411429,
22.));
#52603=CARTESIAN_POINT('Ctrl Pts',(63.3634030175311,-0.976829046022845,
22.));
#52604=CARTESIAN_POINT('Ctrl Pts',(63.358174016723,-0.965934856760109,22.));
#52605=CARTESIAN_POINT('Ctrl Pts',(63.3530525039999,-0.954995586455951,
22.));
#52606=CARTESIAN_POINT('Ctrl Pts',(63.3480415178783,-0.944016502304618,
22.));
#52607=CARTESIAN_POINT('Ctrl Pts',(63.3195013216542,-0.881484855151525,
22.));
#52608=CARTESIAN_POINT('Ctrl Pts',(63.2945220500079,-0.817619969382916,
22.));
#52609=CARTESIAN_POINT('Ctrl Pts',(63.273327165114,-0.752626219153232,22.));
#52610=CARTESIAN_POINT('Ctrl Pts',(63.2541166188605,-0.693717409257717,
22.));
#52611=CARTESIAN_POINT('Ctrl Pts',(63.2380153357376,-0.633880618069508,
22.));
#52612=CARTESIAN_POINT('Ctrl Pts',(63.2252264587662,-0.573263190512459,
22.));
#52613=CARTESIAN_POINT('Ctrl Pts',(63.2100966383573,-0.501550029564712,
22.));
#52614=CARTESIAN_POINT('Ctrl Pts',(63.199602249042,-0.428742773422565,22.));
#52615=CARTESIAN_POINT('Ctrl Pts',(63.1936681155555,-0.355264662039538,
22.));
#52616=CARTESIAN_POINT('Ctrl Pts',(63.1923616383022,-0.339087492895166,
22.));
#52617=CARTESIAN_POINT('Ctrl Pts',(63.1912764288138,-0.322877888063042,
22.));
#52618=CARTESIAN_POINT('Ctrl Pts',(63.1904120545576,-0.30664052888322,22.));
#52619=CARTESIAN_POINT('Ctrl Pts',(63.1895201663096,-0.289886316543617,
22.));
#52620=CARTESIAN_POINT('Ctrl Pts',(63.1888633864282,-0.273096407549196,
22.));
#52621=CARTESIAN_POINT('Ctrl Pts',(63.188441797465,-0.256310042477455,22.));
#52622=CARTESIAN_POINT('Ctrl Pts',(63.1867198704084,-0.187748247168369,
22.));
#52623=CARTESIAN_POINT('Ctrl Pts',(63.188909677006,-0.119158552195863,22.));
#52624=CARTESIAN_POINT('Ctrl Pts',(63.1948905827395,-0.050879356588759,
22.));
#52625=CARTESIAN_POINT('Ctrl Pts',(63.2008702728731,0.0173859614913684,
22.));
#52626=CARTESIAN_POINT('Ctrl Pts',(63.210639974989,0.085341978217158,22.));
#52627=CARTESIAN_POINT('Ctrl Pts',(63.2241287349543,0.152635471609117,22.));
#52628=CARTESIAN_POINT('Ctrl Pts',(63.2338917748096,0.201341880477173,22.));
#52629=CARTESIAN_POINT('Ctrl Pts',(63.2456041790461,0.24970094617825,22.));
#52630=CARTESIAN_POINT('Ctrl Pts',(63.2592532629239,0.297569075157063,22.));
#52631=CARTESIAN_POINT('Ctrl Pts',(63.2694917264659,0.333475960759386,22.));
#52632=CARTESIAN_POINT('Ctrl Pts',(63.2808201731862,0.369106450237582,22.));
#52633=CARTESIAN_POINT('Ctrl Pts',(63.2932371663357,0.404395756317229,22.));
#52634=CARTESIAN_POINT('Ctrl Pts',(63.2973637241668,0.416123503977368,22.));
#52635=CARTESIAN_POINT('Ctrl Pts',(63.3016073023584,0.427804353006757,22.));
#52636=CARTESIAN_POINT('Ctrl Pts',(63.3059672772102,0.439435804940296,22.));
#52637=CARTESIAN_POINT('Ctrl Pts',(63.3290918712259,0.501127124940676,22.));
#52638=CARTESIAN_POINT('Ctrl Pts',(63.3554889558721,0.561434936807572,22.));
#52639=CARTESIAN_POINT('Ctrl Pts',(63.3851084989831,0.620025088710617,22.));
#52640=CARTESIAN_POINT('Ctrl Pts',(63.4059501828543,0.66125183617762,22.));
#52641=CARTESIAN_POINT('Ctrl Pts',(63.4283882196152,0.701627610099956,22.));
#52642=CARTESIAN_POINT('Ctrl Pts',(63.4524155940489,0.741024631059141,22.));
#52643=CARTESIAN_POINT('Ctrl Pts',(63.4601281158537,0.753670639636949,22.));
#52644=CARTESIAN_POINT('Ctrl Pts',(63.4680055619147,0.766217427182377,22.));
#52645=CARTESIAN_POINT('Ctrl Pts',(63.4760443363961,0.778655072840915,22.));
#52646=CARTESIAN_POINT('Ctrl Pts',(63.510290079392,0.831640315514542,22.));
#52647=CARTESIAN_POINT('Ctrl Pts',(63.547391322875,0.882541662758466,22.));
#52648=CARTESIAN_POINT('Ctrl Pts',(63.5873138038049,0.931043840582933,22.));
#52649=CARTESIAN_POINT('Ctrl Pts',(63.6241208989844,0.975761108498468,22.));
#52650=CARTESIAN_POINT('Ctrl Pts',(63.6633266817943,1.01843913679488,22.));
#52651=CARTESIAN_POINT('Ctrl Pts',(63.7049257741094,1.05879788933142,22.));
#52652=CARTESIAN_POINT('Ctrl Pts',(63.7127105119291,1.06635051343316,22.));
#52653=CARTESIAN_POINT('Ctrl Pts',(63.7205791168681,1.07382181318669,22.));
#52654=CARTESIAN_POINT('Ctrl Pts',(63.7285300176229,1.08121113172718,22.));
#52655=CARTESIAN_POINT('Origin',(65.,0.,17.));
#52656=CARTESIAN_POINT('Origin',(65.,0.,12.));
#52657=CARTESIAN_POINT('Origin',(0.,0.,-2.));
#52658=CARTESIAN_POINT('',(-60.,-7.34788079488412E-15,22.));
#52659=CARTESIAN_POINT('Origin',(0.,0.,22.));
#52660=CARTESIAN_POINT('',(-60.,-7.34788079488412E-15,-2.));
#52661=CARTESIAN_POINT('',(-60.,-7.34788079488412E-15,-2.));
#52662=CARTESIAN_POINT('Origin',(0.,0.,-2.));
#52663=CARTESIAN_POINT('Origin',(0.,0.,-2.));
#52664=CARTESIAN_POINT('',(-70.,-8.57252759403147E-15,22.));
#52665=CARTESIAN_POINT('Origin',(0.,0.,22.));
#52666=CARTESIAN_POINT('',(-70.,-8.57252759403147E-15,-2.));
#52667=CARTESIAN_POINT('',(-70.,-8.57252759403147E-15,-2.));
#52668=CARTESIAN_POINT('Origin',(0.,0.,-2.));
#52669=CARTESIAN_POINT('Origin',(0.,0.,22.));
#52670=CARTESIAN_POINT('Origin',(0.,0.,-2.));
#99492=UNCERTAINTY_MEASURE_WITH_UNIT(LENGTH_MEASURE(0.01),#99527,
'DISTANCE_ACCURACY_VALUE',
'Maximum model space distance between geometric entities at asserted c
onnectivities');
#99508=UNCERTAINTY_MEASURE_WITH_UNIT(LENGTH_MEASURE(0.01),#99527,
'DISTANCE_ACCURACY_VALUE',
'Maximum model space distance between geometric entities at asserted c
onnectivities');
#99510=(
GEOMETRIC_REPRESENTATION_CONTEXT(3)
GLOBAL_UNCERTAINTY_ASSIGNED_CONTEXT((#99492))
GLOBAL_UNIT_ASSIGNED_CONTEXT((#99527,#99529,#99530))
REPRESENTATION_CONTEXT('','3D')
);
#99526=(
GEOMETRIC_REPRESENTATION_CONTEXT(3)
GLOBAL_UNCERTAINTY_ASSIGNED_CONTEXT((#99508))
GLOBAL_UNIT_ASSIGNED_CONTEXT((#99527,#99529,#99530))
REPRESENTATION_CONTEXT('','3D')
);
#99527=(
LENGTH_UNIT()
NAMED_UNIT(*)
SI_UNIT(.MILLI.,.METRE.)
);
#99529=(
NAMED_UNIT(*)
PLANE_ANGLE_UNIT()
SI_UNIT($,.RADIAN.)
);
#99530=(
NAMED_UNIT(*)
SI_UNIT($,.STERADIAN.)
SOLID_ANGLE_UNIT()
);
#99532=SHAPE_DEFINITION_REPRESENTATION(#99549,#99625);
#99549=PRODUCT_DEFINITION_SHAPE('',$,#99643);
#99625=SHAPE_REPRESENTATION('',(#18464),#99510);
#99641=PRODUCT_DEFINITION_CONTEXT('part definition',#99694,'design');
#99643=PRODUCT_DEFINITION('Outer race','Outer race',#99660,#99641);
#99660=PRODUCT_DEFINITION_FORMATION('',$,#99697);
#99694=APPLICATION_CONTEXT(
'Core Data for Automotive Mechanical Design Process');
#99695=PRODUCT_CONTEXT('part definition',#99694,'mechanical');
#99697=PRODUCT('Outer race','Outer race',$,(#99695));
#99714=PRESENTATION_STYLE_ASSIGNMENT((#99727));
#99727=SURFACE_STYLE_USAGE(.BOTH.,#99740);
#99740=SURFACE_SIDE_STYLE('',(#99753));
#99753=SURFACE_STYLE_FILL_AREA(#99766);
#99766=FILL_AREA_STYLE('Dark blue',(#99779));
#99779=FILL_AREA_STYLE_COLOUR('Dark blue',#99792);
#99792=COLOUR_RGB('Dark blue',0.0901960784313725,0.270588235294118,0.513725490196078);
ENDSEC;
END-ISO-10303-21;
